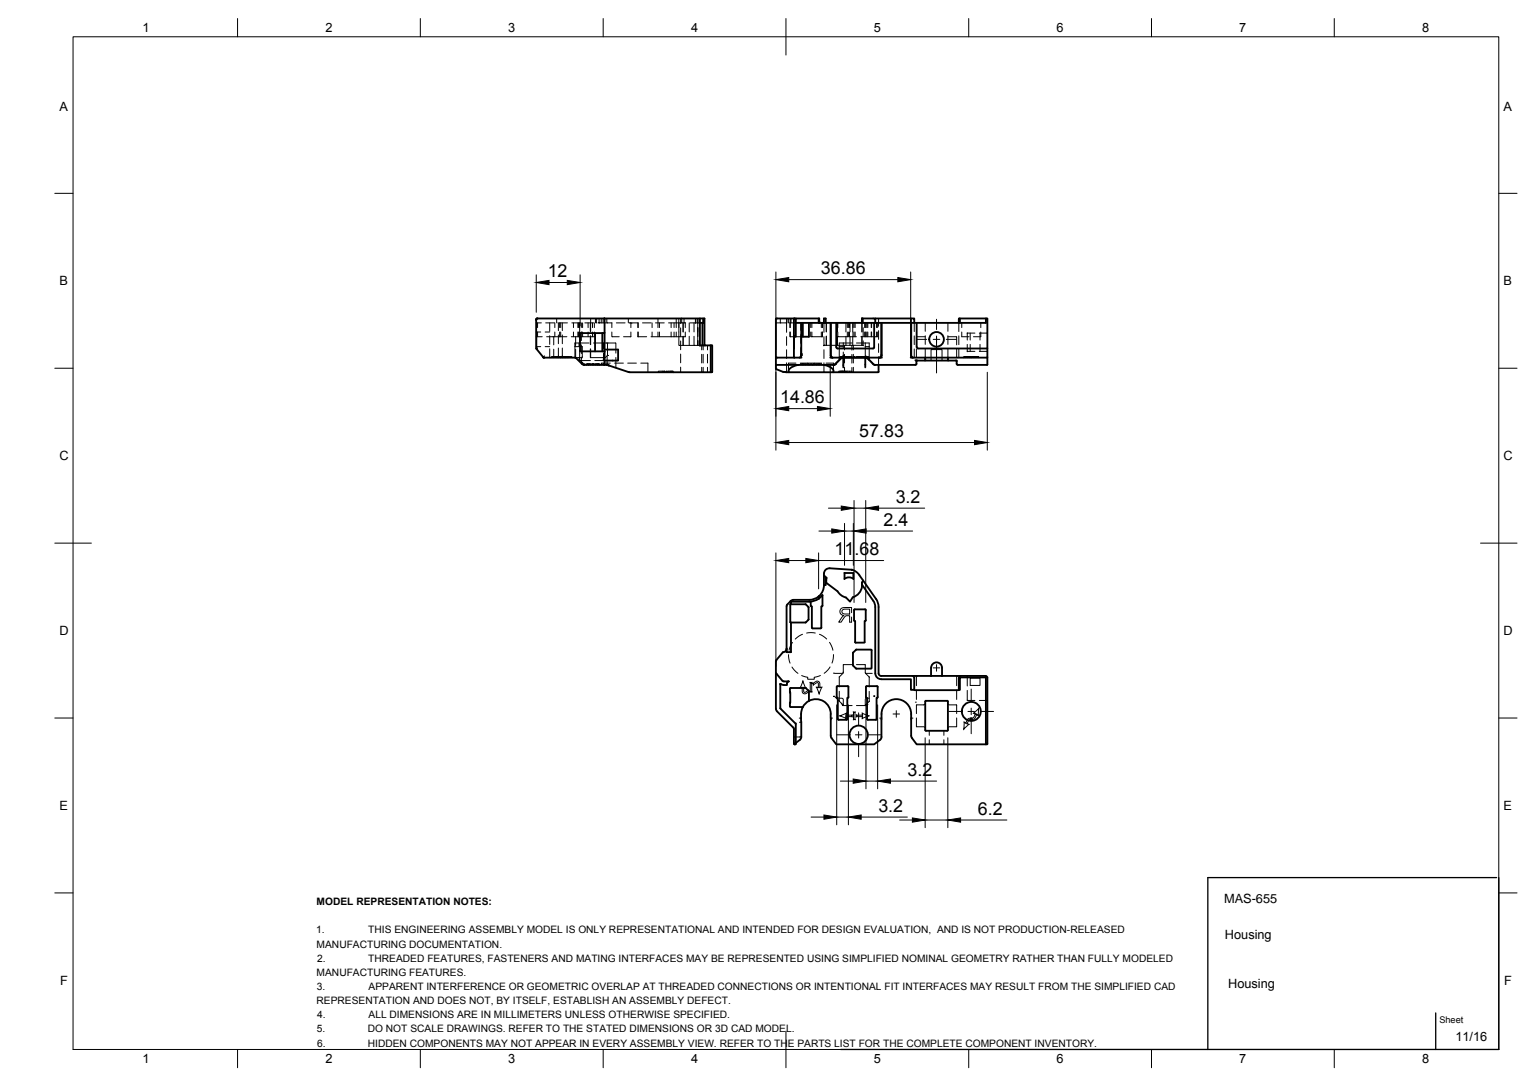
ISO-10303-21;
HEADER;
FILE_DESCRIPTION((''),'2;1');
FILE_NAME('Housing.step','2026-10-09T11:34:15-07:00',(''),(''),'','','');
FILE_SCHEMA (('AUTOMOTIVE_DESIGN { 1 0 10303 214 3 1 1 }'));
ENDSEC;
DATA;
#10=MECHANICAL_DESIGN_GEOMETRIC_PRESENTATION_REPRESENTATION('',(#643),#117170);
#97=(
BOUNDED_SURFACE()
B_SPLINE_SURFACE(2,2,((#90419,#90420,#90421),(#90422,#90423,#90424),(#90425,
#90426,#90427)),.UNSPECIFIED.,.F.,.F.,.F.)
B_SPLINE_SURFACE_WITH_KNOTS((3,3),(3,3),(-1.57079632679569,0.),(-3.14159265358917,
-1.57079632679587),.UNSPECIFIED.)
GEOMETRIC_REPRESENTATION_ITEM()
RATIONAL_B_SPLINE_SURFACE(((1.,0.707106781187113,1.),(0.707106781186163,
0.500000000000127,0.707106781186163),(1.,0.707106781187113,1.)))
REPRESENTATION_ITEM('')
SURFACE()
) ;
#98=(
BOUNDED_SURFACE()
B_SPLINE_SURFACE(2,2,((#90597,#90598,#90599),(#90600,#90601,#90602),(#90603,
#90604,#90605)),.UNSPECIFIED.,.F.,.F.,.F.)
B_SPLINE_SURFACE_WITH_KNOTS((3,3),(3,3),(-1.570796326795,2.27222014866972E-13),
(-1.57079632679441,-7.1054273575954E-13),.UNSPECIFIED.)
GEOMETRIC_REPRESENTATION_ITEM()
RATIONAL_B_SPLINE_SURFACE(((1.,0.707106781186971,1.),(0.70710678118641,
0.500000000000203,0.70710678118641),(1.,0.707106781186971,1.)))
REPRESENTATION_ITEM('')
SURFACE()
) ;
#99=(
BOUNDED_SURFACE()
B_SPLINE_SURFACE(2,2,((#92757,#92758,#92759),(#92760,#92761,#92762),(#92763,
#92764,#92765)),.UNSPECIFIED.,.F.,.F.,.F.)
B_SPLINE_SURFACE_WITH_KNOTS((3,3),(3,3),(-1.57079632680452,-1.25635394189736E-12),
(-2.44346095281043,-1.64859272029811),.UNSPECIFIED.)
GEOMETRIC_REPRESENTATION_ITEM()
RATIONAL_B_SPLINE_SURFACE(((1.,0.922057163080232,1.),(0.707106781183326,
0.651992872652692,0.707106781183326),(1.,0.922057163080232,1.)))
REPRESENTATION_ITEM('')
SURFACE()
) ;
#100=(
BOUNDED_SURFACE()
B_SPLINE_SURFACE(2,2,((#92794,#92795,#92796,#92797,#92798),(#92799,#92800,
#92801,#92802,#92803),(#92804,#92805,#92806,#92807,#92808)),
 .UNSPECIFIED.,.F.,.F.,.F.)
B_SPLINE_SURFACE_WITH_KNOTS((3,3),(3,2,3),(-3.14159265358979,-1.57079632679397),
(-0.795304873266846,0.,0.795304873266846),.UNSPECIFIED.)
GEOMETRIC_REPRESENTATION_ITEM()
RATIONAL_B_SPLINE_SURFACE(((1.,0.921972639390714,1.,0.921972639390714,1.),
(0.707106781186466,0.651933105381558,0.707106781186466,0.651933105381558,
0.707106781186466),(1.,0.921972639390714,1.,0.921972639390714,1.)))
REPRESENTATION_ITEM('')
SURFACE()
) ;
#101=(
BOUNDED_SURFACE()
B_SPLINE_SURFACE(2,2,((#97993,#97994,#97995),(#97996,#97997,#97998),(#97999,
#98000,#98001)),.UNSPECIFIED.,.F.,.F.,.F.)
B_SPLINE_SURFACE_WITH_KNOTS((3,3),(3,3),(-1.57079632673965,5.57007752630405E-11),
(4.19220214067588E-12,0.187132086721036),.UNSPECIFIED.)
GEOMETRIC_REPRESENTATION_ITEM()
RATIONAL_B_SPLINE_SURFACE(((1.,0.99562589029583,1.),(0.70710678118639,0.704013818552918,
0.70710678118639),(1.,0.99562589029583,1.)))
REPRESENTATION_ITEM('')
SURFACE()
) ;
#102=(
BOUNDED_SURFACE()
B_SPLINE_SURFACE(2,2,((#98044,#98045,#98046),(#98047,#98048,#98049),(#98050,
#98051,#98052)),.UNSPECIFIED.,.F.,.F.,.F.)
B_SPLINE_SURFACE_WITH_KNOTS((3,3),(3,3),(-1.57079632677152,2.35301000695734E-11),
(3.55271367856584E-13,0.187132086725463),.UNSPECIFIED.)
GEOMETRIC_REPRESENTATION_ITEM()
RATIONAL_B_SPLINE_SURFACE(((1.,0.995625890295444,1.),(0.707106781186499,
0.704013818552754,0.707106781186499),(1.,0.995625890295444,1.)))
REPRESENTATION_ITEM('')
SURFACE()
) ;
#395=ELLIPSE('',#52555,0.105759245252314,0.090533850109107) ;
#396=ELLIPSE('',#52556,0.105759245244956,0.0905338500956946) ;
#397=ELLIPSE('',#52573,0.634821045649877,0.44) ;
#398=ELLIPSE('',#52575,0.499397396869427,0.2) ;
#399=ELLIPSE('',#52590,0.335751501918208,0.111374721424487) ;
#400=ELLIPSE('',#52593,0.784766199683495,0.4) ;
#401=ELLIPSE('',#52594,24.8257930386904,0.4) ;
#402=ELLIPSE('',#52595,0.424264068711929,0.3) ;
#403=ELLIPSE('',#52596,6.4346717087976,4.55) ;
#404=ELLIPSE('',#52598,0.354400902933385,0.100000000000016) ;
#405=ELLIPSE('',#52599,0.354400902933385,0.100000000000016) ;
#406=ELLIPSE('',#52600,0.354400902933389,0.100000000000016) ;
#407=ELLIPSE('',#52601,0.354400902933389,0.100000000000016) ;
#408=ELLIPSE('',#52605,0.76367532368147,0.54) ;
#409=ELLIPSE('',#52606,0.617737808459213,0.299999999999998) ;
#410=ELLIPSE('',#52614,0.354400902933389,0.100000000000016) ;
#411=ELLIPSE('',#52615,0.354400902933389,0.100000000000016) ;
#412=ELLIPSE('',#52616,0.354400902933385,0.0999999999999801) ;
#413=ELLIPSE('',#52617,0.354400902933385,0.0999999999999801) ;
#414=ELLIPSE('',#52621,0.617737808459213,0.300000000000002) ;
#415=ELLIPSE('',#52622,0.76367532368147,0.54) ;
#416=ELLIPSE('',#52628,0.141421356237298,0.1) ;
#417=ELLIPSE('',#52631,0.277848879788995,0.239999999999938) ;
#418=ELLIPSE('',#52632,0.277848879788997,0.240000000000009) ;
#419=ELLIPSE('',#52639,0.141421356237298,0.1) ;
#420=ELLIPSE('',#52640,0.141421356237298,0.1) ;
#421=ELLIPSE('',#52647,0.339411254969547,0.24) ;
#422=ELLIPSE('',#52650,0.243578652595007,0.24) ;
#423=ELLIPSE('',#52652,0.0577110041499885,0.04) ;
#424=ELLIPSE('',#52655,0.577110041499878,0.399999999999996) ;
#425=ELLIPSE('',#52668,0.424264068711929,0.3) ;
#426=ELLIPSE('',#52700,0.344580851516853,0.222253203953467) ;
#427=ELLIPSE('',#52708,0.141421356237297,0.1) ;
#428=ELLIPSE('',#52747,0.141421356237322,0.1) ;
#429=ELLIPSE('',#52767,1.13357840487546,0.749999999999993) ;
#430=ELLIPSE('',#52768,1.20208152801713,0.85) ;
#431=ELLIPSE('',#52771,0.223606797749978,0.100000000000016) ;
#432=ELLIPSE('',#52772,0.282842712474619,0.2) ;
#433=ELLIPSE('',#52774,0.10069443430648,0.100017256319563) ;
#434=ELLIPSE('',#52805,0.282842712474618,0.2) ;
#435=ELLIPSE('',#52806,0.223606797749975,0.100000000000016) ;
#436=ELLIPSE('',#52810,0.70710678118655,0.5) ;
#437=ELLIPSE('',#52811,0.640312423743287,0.399999999999992) ;
#438=ELLIPSE('',#52813,0.846312901686476,0.400595643005874) ;
#439=ELLIPSE('',#52814,0.862858514657635,0.518233232113999) ;
#440=ELLIPSE('',#52815,0.640312423743287,0.399999999999992) ;
#441=ELLIPSE('',#52816,0.70710678118655,0.5) ;
#442=ELLIPSE('',#52818,0.412310562561758,0.4) ;
#443=ELLIPSE('',#52820,1.34350288425444,0.95) ;
#444=ELLIPSE('',#52825,0.141421356237322,0.1) ;
#445=ELLIPSE('',#52829,0.141421356237322,0.1) ;
#446=ELLIPSE('',#52836,0.223606797749974,0.0999999999999979) ;
#447=ELLIPSE('',#52837,0.223606797749986,0.0999999999999979) ;
#448=ELLIPSE('',#52967,0.258478364700829,0.0999999999999979) ;
#449=ELLIPSE('',#52969,0.311144765372046,0.199999999999998) ;
#450=ELLIPSE('',#52993,0.624999999999997,0.4) ;
#451=ELLIPSE('',#53004,0.51747248987523,0.4999999999999) ;
#452=ELLIPSE('',#53007,0.202758751010048,0.200000000000102) ;
#453=ELLIPSE('',#53010,1.06510302057801,0.999999999999996) ;
#454=ELLIPSE('',#53041,0.499999999999995,0.4) ;
#455=ELLIPSE('',#53084,0.499999999999995,0.4) ;
#456=ELLIPSE('',#53153,0.110950450383119,0.1) ;
#457=ELLIPSE('',#53155,0.693271231193088,0.499999999999992) ;
#458=ELLIPSE('',#53183,0.421637021355679,0.399999999999901) ;
#459=ELLIPSE('',#53187,0.105409255339058,0.100000000000106) ;
#460=ELLIPSE('',#53189,1.1595018087284,1.1) ;
#461=ELLIPSE('',#53225,0.141421356237293,0.1) ;
#462=ELLIPSE('',#53250,0.10597392847322,0.1) ;
#463=ELLIPSE('',#53279,0.800390529679108,0.5) ;
#464=ELLIPSE('',#53281,0.883883476483187,0.5) ;
#465=ELLIPSE('',#53287,0.210818510677909,0.200000000000016) ;
#466=ELLIPSE('',#53289,0.120185042515483,0.0999999999999979) ;
#467=ELLIPSE('',#53291,0.21081851067789,0.199999999999998) ;
#468=ELLIPSE('',#53293,0.120185042515479,0.0999999999999979) ;
#469=ELLIPSE('',#53311,0.316227766016838,0.3) ;
#470=ELLIPSE('',#53317,6.48266920334518,6.15) ;
#471=ELLIPSE('',#53320,1.21037184369102,0.749999999999993) ;
#472=ELLIPSE('',#53322,0.141421356237311,0.1) ;
#473=ELLIPSE('',#53323,0.112603250061041,0.1) ;
#474=ELLIPSE('',#53325,0.17320508075689,0.1) ;
#475=ELLIPSE('',#53326,0.173205080756888,0.1) ;
#476=ELLIPSE('',#53334,0.704171845621267,0.200000000000013) ;
#477=ELLIPSE('',#53337,24.8233760798141,0.2) ;
#478=ELLIPSE('',#53340,0.860232526704269,0.5) ;
#479=ELLIPSE('',#53341,0.18370348154524,0.0706876553262425) ;
#480=ELLIPSE('',#53343,0.989949493661167,0.7) ;
#481=ELLIPSE('',#53347,0.777817459305202,0.55) ;
#482=ELLIPSE('',#53348,0.930053761886906,0.75) ;
#483=ELLIPSE('',#53349,0.930053761886906,0.75) ;
#484=ELLIPSE('',#53358,0.675321117625136,0.479717269382621) ;
#485=ELLIPSE('',#53360,6.4346717087976,4.55) ;
#486=ELLIPSE('',#53363,0.461579895576042,0.2) ;
#487=ELLIPSE('',#53367,0.282842712474621,0.2) ;
#488=ELLIPSE('',#53373,0.565685424949227,0.399999999999992) ;
#489=ELLIPSE('',#53379,6.48266920334518,6.15) ;
#490=ELLIPSE('',#53401,0.100694440756805,0.100017263171969) ;
#491=ELLIPSE('',#53406,0.108636037740531,0.1) ;
#492=ELLIPSE('',#53416,0.179117445565849,0.1) ;
#493=ELLIPSE('',#53419,0.179117445565765,0.1) ;
#494=ELLIPSE('',#53421,0.265520995084799,0.1) ;
#495=ELLIPSE('',#53429,0.179117445565772,0.1) ;
#496=ELLIPSE('',#53431,0.265520995084877,0.1) ;
#497=ELLIPSE('',#53433,0.179117445565864,0.1) ;
#498=ELLIPSE('',#53440,0.179117445565776,0.1) ;
#499=ELLIPSE('',#53441,0.141421356237291,0.1) ;
#500=ELLIPSE('',#53443,0.265520995084917,0.1) ;
#501=ELLIPSE('',#53445,0.179117445565779,0.1) ;
#502=ELLIPSE('',#53447,0.141421356237298,0.1) ;
#503=ELLIPSE('',#53449,0.14142135623732,0.1) ;
#504=ELLIPSE('',#53451,0.141421356237322,0.1) ;
#505=ELLIPSE('',#53459,0.141421356237284,0.1) ;
#506=ELLIPSE('',#53460,0.141421356237347,0.1) ;
#507=ELLIPSE('',#53462,0.141421356237322,0.1) ;
#508=ELLIPSE('',#53464,0.141421356237297,0.1) ;
#509=ELLIPSE('',#53470,0.141421356237321,0.1) ;
#510=ELLIPSE('',#53471,0.17911744556577,0.1) ;
#511=ELLIPSE('',#53473,0.141421356237297,0.1) ;
#512=ELLIPSE('',#53475,0.141421356237325,0.1) ;
#513=ELLIPSE('',#53477,0.141421356237269,0.1) ;
#514=ELLIPSE('',#53479,0.17911744556575,0.1) ;
#515=ELLIPSE('',#53481,0.265520995084842,0.1) ;
#516=ELLIPSE('',#53489,0.141421356237322,0.1) ;
#517=ELLIPSE('',#53490,0.141421356237297,0.1) ;
#518=ELLIPSE('',#53492,0.141421356237297,0.1) ;
#519=ELLIPSE('',#53494,0.141421356237322,0.1) ;
#520=ELLIPSE('',#53500,0.179117445565841,0.1) ;
#521=ELLIPSE('',#53501,0.265520995084931,0.1) ;
#522=ELLIPSE('',#53503,0.141421356237301,0.1) ;
#523=ELLIPSE('',#53511,0.141421356237312,0.1) ;
#524=ELLIPSE('',#53513,0.141421356237306,0.1) ;
#525=ELLIPSE('',#53521,0.141421356237327,0.1) ;
#526=ELLIPSE('',#53523,0.179117445565764,0.1) ;
#527=ELLIPSE('',#53534,0.141421356237301,0.1) ;
#528=ELLIPSE('',#53535,0.179117445565841,0.1) ;
#529=ELLIPSE('',#53543,0.141421356237313,0.1) ;
#530=ELLIPSE('',#53545,0.141421356237306,0.1) ;
#531=ELLIPSE('',#53553,0.141421356237327,0.1) ;
#532=ELLIPSE('',#53555,0.179117445565764,0.1) ;
#533=ELLIPSE('',#53557,0.265520995084931,0.1) ;
#534=ELLIPSE('',#53569,0.179117445565845,0.1) ;
#535=ELLIPSE('',#53571,0.265520995084763,0.1) ;
#536=ELLIPSE('',#53573,0.179117445565757,0.1) ;
#537=ELLIPSE('',#53577,0.179117445565837,0.1) ;
#538=ELLIPSE('',#53579,0.179117445565763,0.1) ;
#539=ELLIPSE('',#53580,0.265520995084739,0.1) ;
#540=ELLIPSE('',#53587,0.179117445565766,0.1) ;
#541=ELLIPSE('',#53588,0.265520995084941,0.1) ;
#542=ELLIPSE('',#53590,0.179117445565779,0.1) ;
#543=ELLIPSE('',#53592,0.141421356237327,0.1) ;
#544=ELLIPSE('',#53594,0.141421356237297,0.1) ;
#545=ELLIPSE('',#53596,0.141421356237347,0.1) ;
#546=ELLIPSE('',#53598,0.141421356237294,0.1) ;
#547=ELLIPSE('',#53610,0.14142135623731,0.1) ;
#548=ELLIPSE('',#53611,0.141421356237284,0.1) ;
#549=ELLIPSE('',#53613,0.141421356237322,0.1) ;
#550=ELLIPSE('',#53615,0.141421356237297,0.1) ;
#551=ELLIPSE('',#53619,0.141421356237325,0.1) ;
#552=ELLIPSE('',#53620,0.141421356237319,0.1) ;
#553=ELLIPSE('',#53622,0.141421356237303,0.1) ;
#554=ELLIPSE('',#53624,0.179117445565787,0.1) ;
#555=ELLIPSE('',#53626,0.265520995084743,0.1) ;
#556=ELLIPSE('',#53628,0.179117445565783,0.1) ;
#557=ELLIPSE('',#53630,0.141421356237323,0.1) ;
#558=ELLIPSE('',#53635,0.141421356237297,0.1) ;
#559=ELLIPSE('',#53636,0.141421356237322,0.1) ;
#560=ELLIPSE('',#53638,0.141421356237322,0.1) ;
#561=ELLIPSE('',#53640,0.141421356237322,0.1) ;
#562=ELLIPSE('',#53644,0.141421356237324,0.1) ;
#563=ELLIPSE('',#53646,0.179117445565837,0.1) ;
#564=ELLIPSE('',#53648,0.265520995084907,0.1) ;
#565=ELLIPSE('',#53650,0.17911744556577,0.1) ;
#566=ELLIPSE('',#53652,0.141421356237293,0.1) ;
#567=ELLIPSE('',#53669,0.141421356237314,0.1) ;
#568=ELLIPSE('',#53670,0.141421356237323,0.1) ;
#569=ELLIPSE('',#53673,0.141421356237324,0.1) ;
#570=ELLIPSE('',#53675,0.179117445565837,0.1) ;
#571=ELLIPSE('',#53677,0.265520995084885,0.1) ;
#572=ELLIPSE('',#53679,0.179117445565777,0.1) ;
#573=ELLIPSE('',#53681,0.141421356237293,0.1) ;
#574=ELLIPSE('',#53750,0.554752251915545,0.5) ;
#575=ELLIPSE('',#53770,1.17924764150709,0.999999999999996) ;
#576=ELLIPSE('',#53781,6.09138736249799,4.05) ;
#577=ELLIPSE('',#53794,6.09138736249799,4.05) ;
#578=ELLIPSE('',#53808,1.04166666666667,0.5) ;
#579=ELLIPSE('',#53810,1.17924764150709,0.999999999999997) ;
#580=ELLIPSE('',#53811,0.800390529679107,0.5) ;
#581=ELLIPSE('',#53814,1.17924764150709,0.999999999999997) ;
#582=ELLIPSE('',#53815,0.800390529679107,0.5) ;
#583=ELLIPSE('',#53817,0.883883476483178,0.5) ;
#584=ELLIPSE('',#53821,1.17924764150709,0.999999999999996) ;
#585=ELLIPSE('',#53822,0.800390529679108,0.5) ;
#601=SHAPE_REPRESENTATION_RELATIONSHIP('SRR','None',#117256,#622) ;
#622=ADVANCED_BREP_SHAPE_REPRESENTATION('',(#664),#117164) ;
#643=STYLED_ITEM('',(#117355),#664) ;
#664=MANIFOLD_SOLID_BREP('Body1',#49072) ;
#738=FACE_BOUND('',#15575,.T.) ;
#739=FACE_BOUND('',#15577,.T.) ;
#740=FACE_BOUND('',#15578,.T.) ;
#741=FACE_BOUND('',#15718,.T.) ;
#742=FACE_BOUND('',#15719,.T.) ;
#743=FACE_BOUND('',#15720,.T.) ;
#744=FACE_BOUND('',#15721,.T.) ;
#745=FACE_BOUND('',#15722,.T.) ;
#746=FACE_BOUND('',#15723,.T.) ;
#747=FACE_BOUND('',#15724,.T.) ;
#748=FACE_BOUND('',#15886,.T.) ;
#749=FACE_BOUND('',#15887,.T.) ;
#750=FACE_BOUND('',#15891,.T.) ;
#751=FACE_BOUND('',#15930,.T.) ;
#752=FACE_BOUND('',#15931,.T.) ;
#753=FACE_BOUND('',#15932,.T.) ;
#754=FACE_BOUND('',#15963,.T.) ;
#755=FACE_BOUND('',#15973,.T.) ;
#756=FACE_BOUND('',#15976,.T.) ;
#757=FACE_BOUND('',#16106,.T.) ;
#758=FACE_BOUND('',#16107,.T.) ;
#759=FACE_BOUND('',#16108,.T.) ;
#760=FACE_BOUND('',#16262,.T.) ;
#1149=B_SPLINE_CURVE_WITH_KNOTS('',3,(#89080,#89081,#89082,#89083,#89084,
#89085,#89086,#89087,#89088,#89089,#89090,#89091,#89092),.UNSPECIFIED.,
 .F.,.F.,(4,1,1,1,1,1,1,1,1,1,4),(0.,0.1,0.2,0.3,0.4,0.5,0.6,0.7,0.8,0.9,
1.),.UNSPECIFIED.) ;
#1150=B_SPLINE_CURVE_WITH_KNOTS('',3,(#89094,#89095,#89096,#89097,#89098,
#89099),.UNSPECIFIED.,.F.,.F.,(4,1,1,4),(0.,0.333333333333333,0.666666666666667,
1.),.UNSPECIFIED.) ;
#1151=B_SPLINE_CURVE_WITH_KNOTS('',3,(#89101,#89102,#89103,#89104,#89105,
#89106,#89107,#89108,#89109,#89110,#89111,#89112,#89113,#89114,#89115,#89116,
#89117,#89118,#89119,#89120,#89121,#89122,#89123,#89124,#89125,#89126,#89127,
#89128,#89129,#89130,#89131,#89132,#89133,#89134,#89135,#89136,#89137,#89138,
#89139,#89140,#89141,#89142,#89143,#89144,#89145,#89146,#89147,#89148,#89149,
#89150,#89151,#89152,#89153,#89154,#89155,#89156,#89157,#89158,#89159,#89160,
#89161,#89162,#89163,#89164),.UNSPECIFIED.,.F.,.F.,(4,3,3,3,3,3,3,3,3,3,
3,3,3,3,3,3,3,3,3,3,3,4),(0.50000000000002,0.540931884362004,0.549999476969566,
0.57785534140829,0.599999449142665,0.630623423732254,0.650001938995543,
0.670121368703304,0.699999961337087,0.726319366023772,0.749998804879715,
0.764743070246695,0.800000000093043,0.800090168326521,0.850000141966713,
0.856761721866945,0.899999993071106,0.902358829665644,0.942091717824869,
0.950000243206862,0.977692918008602,1.),.UNSPECIFIED.) ;
#1152=B_SPLINE_CURVE_WITH_KNOTS('',3,(#89245,#89246,#89247,#89248,#89249,
#89250,#89251,#89252,#89253,#89254,#89255,#89256,#89257),.UNSPECIFIED.,
 .F.,.F.,(4,1,1,1,1,1,1,1,1,1,4),(0.,0.1,0.2,0.3,0.4,0.5,0.6,0.7,0.8,0.9,
1.),.UNSPECIFIED.) ;
#1153=B_SPLINE_CURVE_WITH_KNOTS('',3,(#89260,#89261,#89262,#89263,#89264,
#89265,#89266,#89267,#89268,#89269,#89270,#89271,#89272,#89273,#89274,#89275,
#89276,#89277,#89278,#89279,#89280,#89281,#89282,#89283,#89284,#89285,#89286,
#89287,#89288,#89289,#89290,#89291,#89292,#89293,#89294,#89295,#89296,#89297,
#89298,#89299,#89300,#89301,#89302,#89303,#89304,#89305,#89306,#89307,#89308,
#89309,#89310,#89311,#89312,#89313,#89314,#89315,#89316,#89317,#89318,#89319,
#89320,#89321,#89322,#89323,#89324,#89325,#89326),.UNSPECIFIED.,.F.,.F.,
(4,3,3,3,3,3,3,3,3,3,3,3,3,3,3,3,3,3,3,3,3,3,4),(0.,0.029211291026702,0.0500008174088028,
0.060544943773545,0.0938972400757973,0.100000166665901,0.130378684246365,
0.15000088015134,0.174071006839537,0.199999777732466,0.221649421518731,
0.249999425571877,0.25898085613298,0.293770381915345,0.299999713862244,
0.331057161559401,0.350001769846541,0.368733440803518,0.400000309272562,
0.412905090819267,0.450000017037755,0.479639534628252,0.50000000000002),
 .UNSPECIFIED.) ;
#1154=B_SPLINE_CURVE_WITH_KNOTS('',3,(#89406,#89407,#89408,#89409,#89410,
#89411),.UNSPECIFIED.,.F.,.F.,(4,1,1,4),(0.,0.333333333333333,0.666666666666667,
0.999999901148969),.UNSPECIFIED.) ;
#1155=B_SPLINE_CURVE_WITH_KNOTS('',3,(#89413,#89414,#89415,#89416,#89417,
#89418,#89419,#89420,#89421,#89422,#89423,#89424,#89425,#89426,#89427,#89428,
#89429,#89430,#89431,#89432,#89433,#89434,#89435,#89436,#89437,#89438,#89439,
#89440,#89441,#89442,#89443,#89444,#89445,#89446,#89447,#89448,#89449,#89450,
#89451,#89452,#89453,#89454,#89455),.UNSPECIFIED.,.F.,.F.,(4,3,3,3,3,3,
3,3,3,3,3,3,3,3,4),(0.740046669567313,0.763099290859212,0.784481908360721,
0.811421669815631,0.819140541376942,0.832121780979733,0.85502513103706,
0.889660371947781,0.913260537792704,0.914933018320988,0.935388557500039,
0.955946024091937,0.975439020158076,0.993845115294604,0.999999999999939),
 .UNSPECIFIED.) ;
#1156=B_SPLINE_CURVE_WITH_KNOTS('',3,(#89457,#89458,#89459,#89460,#89461,
#89462,#89463,#89464,#89465,#89466,#89467,#89468,#89469,#89470,#89471,#89472,
#89473,#89474,#89475,#89476,#89477,#89478,#89479,#89480,#89481,#89482,#89483,
#89484,#89485,#89486,#89487,#89488,#89489,#89490,#89491,#89492,#89493,#89494,
#89495,#89496,#89497,#89498,#89499,#89500,#89501,#89502,#89503,#89504,#89505,
#89506,#89507,#89508,#89509,#89510,#89511,#89512,#89513,#89514,#89515,#89516,
#89517,#89518,#89519,#89520,#89521,#89522,#89523,#89524,#89525,#89526,#89527,
#89528,#89529,#89530,#89531,#89532,#89533,#89534,#89535,#89536,#89537,#89538,
#89539,#89540,#89541,#89542,#89543,#89544,#89545,#89546,#89547,#89548,#89549,
#89550,#89551,#89552,#89553,#89554,#89555,#89556),.UNSPECIFIED.,.F.,.F.,
(4,3,3,3,3,3,3,3,3,3,3,3,3,3,3,3,3,3,3,3,3,3,3,3,3,3,3,3,3,3,3,3,3,4),(9.43012544827459E-8,
0.031864058797589,0.0647840362122895,0.0990069909892971,0.125039338268755,
0.134916637559053,0.176959063913584,0.215046371604815,0.260170220267245,
0.265136830208005,0.318040825054938,0.360663273489004,0.363657546998835,
0.400621818895941,0.438082955214945,0.468825159061875,0.473202770514011,
0.511546102075598,0.546372378738656,0.578100024548857,0.583032295575111,
0.622265622394134,0.665621014897703,0.680754237084197,0.720780686822075,
0.771027763058629,0.790928228827376,0.813100495945339,0.85149915167859,
0.888624363758942,0.922410481952504,0.955205742315633,0.986814689647663,
1.),.UNSPECIFIED.) ;
#1157=B_SPLINE_CURVE_WITH_KNOTS('',3,(#89625,#89626,#89627,#89628,#89629,
#89630,#89631,#89632,#89633,#89634,#89635),.UNSPECIFIED.,.F.,.F.,(4,1,1,
1,1,1,1,1,4),(0.,0.125,0.25,0.375,0.5,0.625,0.75,0.875,1.),
 .UNSPECIFIED.) ;
#1158=B_SPLINE_CURVE_WITH_KNOTS('',3,(#89638,#89639,#89640,#89641,#89642,
#89643,#89644,#89645,#89646,#89647,#89648,#89649,#89650,#89651,#89652,#89653,
#89654,#89655,#89656,#89657,#89658,#89659,#89660,#89661,#89662,#89663,#89664,
#89665,#89666,#89667,#89668,#89669,#89670,#89671,#89672,#89673,#89674,#89675,
#89676,#89677,#89678,#89679,#89680,#89681,#89682,#89683,#89684,#89685,#89686,
#89687,#89688,#89689,#89690,#89691,#89692,#89693,#89694,#89695,#89696,#89697,
#89698,#89699,#89700,#89701,#89702,#89703,#89704,#89705,#89706,#89707,#89708,
#89709,#89710,#89711,#89712,#89713,#89714,#89715,#89716,#89717,#89718,#89719,
#89720,#89721,#89722,#89723,#89724,#89725,#89726,#89727,#89728,#89729,#89730,
#89731,#89732,#89733,#89734,#89735,#89736,#89737),.UNSPECIFIED.,.F.,.F.,
(4,3,3,3,3,3,3,3,3,3,3,3,3,3,3,3,3,3,3,3,3,3,3,3,3,3,3,3,3,3,3,3,3,4),(0.,
0.0234163840184272,0.0478392774354898,0.0735929525966121,0.101260672275236,
0.13215515581021,0.161611085696521,0.205091291829831,0.208484168145554,
0.238318416362703,0.265116005993426,0.265187074007494,0.29019218665116,
0.318308090975454,0.345050056035187,0.357100347629798,0.373722767756927,
0.405591170427141,0.433846469730387,0.445335557423208,0.48217444472529,
0.505617857135101,0.514408471114612,0.542613244205269,0.568369687650452,
0.581008652375286,0.593348553719565,0.615767486536519,0.638648003192484,
0.659516414041665,0.663954602269109,0.699207373791262,0.730123470459489,
0.740046655839865),.UNSPECIFIED.) ;
#1159=B_SPLINE_CURVE_WITH_KNOTS('',3,(#89805,#89806,#89807,#89808,#89809,
#89810),.UNSPECIFIED.,.F.,.F.,(4,1,1,4),(0.,0.333333333333333,0.666666666666667,
1.),.UNSPECIFIED.) ;
#1160=B_SPLINE_CURVE_WITH_KNOTS('',3,(#89812,#89813,#89814,#89815,#89816,
#89817,#89818,#89819,#89820,#89821,#89822,#89823,#89824,#89825,#89826,#89827,
#89828,#89829,#89830,#89831,#89832,#89833,#89834,#89835,#89836,#89837,#89838,
#89839,#89840,#89841,#89842,#89843,#89844,#89845,#89846,#89847,#89848,#89849,
#89850,#89851,#89852,#89853,#89854,#89855,#89856,#89857,#89858,#89859,#89860,
#89861,#89862,#89863,#89864,#89865,#89866,#89867,#89868,#89869,#89870,#89871,
#89872),.UNSPECIFIED.,.F.,.F.,(4,3,3,3,3,3,3,3,3,3,3,3,3,3,3,3,3,3,3,3,
4),(0.499999999999957,0.543426929556171,0.562498466595099,0.582529420733352,
0.623146114415814,0.624999981287924,0.663596929285891,0.687501639134093,
0.717594346195301,0.749999793833349,0.754935239198527,0.789630090278152,
0.812500138729425,0.825709594031802,0.866465848423957,0.875000628872866,
0.911531406767164,0.937498440919157,0.946944182542892,0.977771956059037,
1.),.UNSPECIFIED.) ;
#1161=B_SPLINE_CURVE_WITH_KNOTS('',3,(#89894,#89895,#89896,#89897,#89898),
 .UNSPECIFIED.,.F.,.F.,(4,1,4),(0.,0.0298071351389365,0.0685496713495228),
 .UNSPECIFIED.) ;
#1162=B_SPLINE_CURVE_WITH_KNOTS('',3,(#89901,#89902,#89903,#89904,#89905),
 .UNSPECIFIED.,.F.,.F.,(4,1,4),(0.,0.0298071351389365,0.0685496713495228),
 .UNSPECIFIED.) ;
#1163=B_SPLINE_CURVE_WITH_KNOTS('',3,(#89917,#89918,#89919,#89920,#89921),
 .UNSPECIFIED.,.F.,.F.,(4,1,4),(0.,0.0263673128827931,0.0523427870633456),
 .UNSPECIFIED.) ;
#1164=B_SPLINE_CURVE_WITH_KNOTS('',3,(#89924,#89925,#89926,#89927,#89928),
 .UNSPECIFIED.,.F.,.F.,(4,1,4),(0.,0.0263673128827931,0.0523427870633456),
 .UNSPECIFIED.) ;
#1165=B_SPLINE_CURVE_WITH_KNOTS('',3,(#89940,#89941,#89942,#89943,#89944),
 .UNSPECIFIED.,.F.,.F.,(4,1,4),(0.,0.0190758281807941,0.0379545209982657),
 .UNSPECIFIED.) ;
#1166=B_SPLINE_CURVE_WITH_KNOTS('',3,(#89947,#89948,#89949,#89950,#89951),
 .UNSPECIFIED.,.F.,.F.,(4,1,4),(0.,0.0190758281807941,0.0379545209982657),
 .UNSPECIFIED.) ;
#1167=B_SPLINE_CURVE_WITH_KNOTS('',3,(#89963,#89964,#89965,#89966,#89967),
 .UNSPECIFIED.,.F.,.F.,(4,1,4),(0.,0.0205128997765721,0.0398218276255599),
 .UNSPECIFIED.) ;
#1168=B_SPLINE_CURVE_WITH_KNOTS('',3,(#89970,#89971,#89972,#89973,#89974),
 .UNSPECIFIED.,.F.,.F.,(4,1,4),(0.,0.0205128997765721,0.0398218276255599),
 .UNSPECIFIED.) ;
#1169=B_SPLINE_CURVE_WITH_KNOTS('',3,(#89986,#89987,#89988,#89989,#89990),
 .UNSPECIFIED.,.F.,.F.,(4,1,4),(0.,0.0323852950215525,0.0574227556854303),
 .UNSPECIFIED.) ;
#1170=B_SPLINE_CURVE_WITH_KNOTS('',3,(#89993,#89994,#89995,#89996,#89997),
 .UNSPECIFIED.,.F.,.F.,(4,1,4),(0.,0.0323852950215525,0.0574227556854303),
 .UNSPECIFIED.) ;
#1171=B_SPLINE_CURVE_WITH_KNOTS('',3,(#90033,#90034,#90035,#90036,#90037),
 .UNSPECIFIED.,.F.,.F.,(4,1,4),(0.,0.011955158932918,0.0295605475166918),
 .UNSPECIFIED.) ;
#1172=B_SPLINE_CURVE_WITH_KNOTS('',3,(#90040,#90041,#90042,#90043,#90044),
 .UNSPECIFIED.,.F.,.F.,(4,1,4),(0.,0.011955158932918,0.0295605475166918),
 .UNSPECIFIED.) ;
#1173=B_SPLINE_CURVE_WITH_KNOTS('',3,(#90056,#90057,#90058,#90059,#90060),
 .UNSPECIFIED.,.F.,.F.,(4,1,4),(0.,0.0135228484064754,0.0263579081616444),
 .UNSPECIFIED.) ;
#1174=B_SPLINE_CURVE_WITH_KNOTS('',3,(#90063,#90064,#90065,#90066,#90067),
 .UNSPECIFIED.,.F.,.F.,(4,1,4),(0.,0.0135228484064754,0.0263579081616444),
 .UNSPECIFIED.) ;
#1175=B_SPLINE_CURVE_WITH_KNOTS('',3,(#90079,#90080,#90081,#90082,#90083),
 .UNSPECIFIED.,.F.,.F.,(4,1,4),(0.,0.0216058216755205,0.0381303842659523),
 .UNSPECIFIED.) ;
#1176=B_SPLINE_CURVE_WITH_KNOTS('',3,(#90086,#90087,#90088,#90089,#90090),
 .UNSPECIFIED.,.F.,.F.,(4,1,4),(0.,0.0216058216755205,0.0381303842659523),
 .UNSPECIFIED.) ;
#1177=B_SPLINE_CURVE_WITH_KNOTS('',3,(#90102,#90103,#90104,#90105,#90106),
 .UNSPECIFIED.,.F.,.F.,(4,1,4),(0.,0.0381782469542568,0.0670753371474822),
 .UNSPECIFIED.) ;
#1178=B_SPLINE_CURVE_WITH_KNOTS('',3,(#90109,#90110,#90111,#90112,#90113),
 .UNSPECIFIED.,.F.,.F.,(4,1,4),(0.,0.0381782469542568,0.0670753371474822),
 .UNSPECIFIED.) ;
#1179=B_SPLINE_CURVE_WITH_KNOTS('',3,(#90143,#90144,#90145,#90146,#90147),
 .UNSPECIFIED.,.F.,.F.,(4,1,4),(0.,0.0329095469988702,0.0691336974954879),
 .UNSPECIFIED.) ;
#1180=B_SPLINE_CURVE_WITH_KNOTS('',3,(#90150,#90151,#90152,#90153,#90154),
 .UNSPECIFIED.,.F.,.F.,(4,1,4),(0.,0.0329095469988702,0.0691336974954879),
 .UNSPECIFIED.) ;
#1181=B_SPLINE_CURVE_WITH_KNOTS('',3,(#90166,#90167,#90168,#90169,#90170),
 .UNSPECIFIED.,.F.,.F.,(4,1,4),(0.,0.0210301296927785,0.0377156586265697),
 .UNSPECIFIED.) ;
#1182=B_SPLINE_CURVE_WITH_KNOTS('',3,(#90173,#90174,#90175,#90176,#90177),
 .UNSPECIFIED.,.F.,.F.,(4,1,4),(0.,0.0210301296927785,0.0377156586265697),
 .UNSPECIFIED.) ;
#1183=B_SPLINE_CURVE_WITH_KNOTS('',3,(#90189,#90190,#90191,#90192,#90193),
 .UNSPECIFIED.,.F.,.F.,(4,1,4),(0.,0.0424180496051088,0.0942055476140892),
 .UNSPECIFIED.) ;
#1184=B_SPLINE_CURVE_WITH_KNOTS('',3,(#90196,#90197,#90198,#90199,#90200),
 .UNSPECIFIED.,.F.,.F.,(4,1,4),(0.,0.0424180496051088,0.0942055476140892),
 .UNSPECIFIED.) ;
#1185=B_SPLINE_CURVE_WITH_KNOTS('',3,(#90212,#90213,#90214,#90215,#90216),
 .UNSPECIFIED.,.F.,.F.,(4,1,4),(0.,0.0398228695438388,0.0783699334705556),
 .UNSPECIFIED.) ;
#1186=B_SPLINE_CURVE_WITH_KNOTS('',3,(#90219,#90220,#90221,#90222,#90223),
 .UNSPECIFIED.,.F.,.F.,(4,1,4),(0.,0.0398228695438388,0.0783699334705556),
 .UNSPECIFIED.) ;
#1187=B_SPLINE_CURVE_WITH_KNOTS('',3,(#90235,#90236,#90237,#90238,#90239),
 .UNSPECIFIED.,.F.,.F.,(4,1,4),(0.,0.0313133324080373,0.063168759987351),
 .UNSPECIFIED.) ;
#1188=B_SPLINE_CURVE_WITH_KNOTS('',3,(#90242,#90243,#90244,#90245,#90246),
 .UNSPECIFIED.,.F.,.F.,(4,1,4),(0.,0.0313133324080373,0.063168759987351),
 .UNSPECIFIED.) ;
#1189=B_SPLINE_CURVE_WITH_KNOTS('',3,(#90258,#90259,#90260,#90261,#90262),
 .UNSPECIFIED.,.F.,.F.,(4,1,4),(0.,0.0290828541577381,0.0592932101613289),
 .UNSPECIFIED.) ;
#1190=B_SPLINE_CURVE_WITH_KNOTS('',3,(#90265,#90266,#90267,#90268,#90269),
 .UNSPECIFIED.,.F.,.F.,(4,1,4),(0.,0.0290828541577381,0.0592932101613289),
 .UNSPECIFIED.) ;
#1191=B_SPLINE_CURVE_WITH_KNOTS('',3,(#90281,#90282,#90283,#90284,#90285),
 .UNSPECIFIED.,.F.,.F.,(4,1,4),(0.,0.0471458586470647,0.0823534588635132),
 .UNSPECIFIED.) ;
#1192=B_SPLINE_CURVE_WITH_KNOTS('',3,(#90288,#90289,#90290,#90291,#90292),
 .UNSPECIFIED.,.F.,.F.,(4,1,4),(0.,0.0471458586470647,0.0823534588635132),
 .UNSPECIFIED.) ;
#1193=B_SPLINE_CURVE_WITH_KNOTS('',3,(#90383,#90384,#90385,#90386,#90387,
#90388),.UNSPECIFIED.,.F.,.F.,(4,2,4),(-0.0646894582084791,-0.0581995466601206,
-0.0505532240038533),.UNSPECIFIED.) ;
#1194=B_SPLINE_CURVE_WITH_KNOTS('',3,(#90391,#90392,#90393,#90394,#90395,
#90396),.UNSPECIFIED.,.F.,.F.,(4,2,4),(-0.0279464003917075,-0.0162728575198495,
-0.00636479267613269),.UNSPECIFIED.) ;
#1195=B_SPLINE_CURVE_WITH_KNOTS('',3,(#90404,#90405,#90406,#90407,#90408,
#90409,#90410,#90411),.UNSPECIFIED.,.F.,.F.,(4,2,2,4),(-0.0463941724255825,
-0.0363335959367585,-0.0244739336232673,6.93889390390723E-18),
 .UNSPECIFIED.) ;
#1196=B_SPLINE_CURVE_WITH_KNOTS('',3,(#90438,#90439,#90440,#90441),
 .UNSPECIFIED.,.F.,.F.,(4,4),(-0.00233157716846821,0.),.UNSPECIFIED.) ;
#1197=B_SPLINE_CURVE_WITH_KNOTS('',3,(#90466,#90467,#90468,#90469,#90470,
#90471,#90472,#90473,#90474,#90475,#90476,#90477,#90478,#90479,#90480,#90481,
#90482,#90483,#90484,#90485,#90486,#90487,#90488,#90489,#90490,#90491,#90492,
#90493),.UNSPECIFIED.,.F.,.F.,(4,3,3,3,3,3,3,3,3,4),(3.21026029059551E-8,
0.00464707931025668,0.00929415862051336,0.0137678334300167,0.0156388310171345,
0.0187179653523303,0.0232666593299545,0.0251479586559353,0.0296888345732088,
0.0316724821582484),.UNSPECIFIED.) ;
#1198=B_SPLINE_CURVE_WITH_KNOTS('',3,(#90495,#90496,#90497,#90498),
 .UNSPECIFIED.,.F.,.F.,(4,4),(0.000498023522427242,0.00742046561384795),
 .UNSPECIFIED.) ;
#1199=B_SPLINE_CURVE_WITH_KNOTS('',3,(#90499,#90500,#90501,#90502,#90503,
#90504,#90505),.UNSPECIFIED.,.F.,.F.,(4,3,4),(0.00742046561384795,0.0146643599521495,
0.0162549092688308),.UNSPECIFIED.) ;
#1200=B_SPLINE_CURVE_WITH_KNOTS('',3,(#90552,#90553,#90554,#90555,#90556,
#90557),.UNSPECIFIED.,.F.,.F.,(4,2,4),(0.,0.00166959259478934,0.00333900921077541),
 .UNSPECIFIED.) ;
#1201=B_SPLINE_CURVE_WITH_KNOTS('',3,(#90565,#90566,#90567,#90568,#90569,
#90570,#90571,#90572,#90573,#90574,#90575,#90576,#90577),.UNSPECIFIED.,
 .F.,.F.,(4,3,3,3,4),(-0.0247314244030886,-0.0245013764734994,-0.0199768571653589,
-0.0156201260570807,-0.0140088579916689),.UNSPECIFIED.) ;
#1202=B_SPLINE_CURVE_WITH_KNOTS('',3,(#90579,#90580,#90581,#90582,#90583,
#90584),.UNSPECIFIED.,.F.,.F.,(4,2,4),(-0.00524067245577225,-0.00262950955895225,
0.),.UNSPECIFIED.) ;
#1203=B_SPLINE_CURVE_WITH_KNOTS('',3,(#90585,#90586,#90587,#90588,#90589,
#90590),.UNSPECIFIED.,.F.,.F.,(4,2,4),(-0.0208077196740842,-0.0103104127273635,
-0.000111699617630046),.UNSPECIFIED.) ;
#1204=B_SPLINE_CURVE_WITH_KNOTS('',3,(#90620,#90621,#90622,#90623,#90624,
#90625),.UNSPECIFIED.,.F.,.F.,(4,2,4),(-0.167893988576184,-0.139678911984281,
-0.12132773760924),.UNSPECIFIED.) ;
#1205=B_SPLINE_CURVE_WITH_KNOTS('',3,(#90711,#90712,#90713,#90714,#90715,
#90716,#90717,#90718,#90719,#90720,#90721,#90722),.UNSPECIFIED.,.F.,.F.,
(4,2,2,2,2,4),(-0.103468456759814,-0.102439814165996,-0.0469583320002097,
-0.0291854860033449,-0.010865621464627,0.),.UNSPECIFIED.) ;
#1206=B_SPLINE_CURVE_WITH_KNOTS('',3,(#90724,#90725,#90726,#90727,#90728,
#90729,#90730,#90731,#90732,#90733,#90734,#90735,#90736,#90737,#90738,#90739,
#90740,#90741,#90742,#90743,#90744,#90745,#90746,#90747,#90748,#90749,#90750,
#90751),.UNSPECIFIED.,.F.,.F.,(4,3,3,3,3,3,3,3,3,4),(-0.0929261016547975,
-0.0912735545557092,-0.0896210074566209,-0.0863159132584443,-0.0797057248620911,
-0.073095536465738,-0.0532649712766785,-0.0268242176912658,-0.0234862530524168,
-0.00123315546009042),.UNSPECIFIED.) ;
#1207=B_SPLINE_CURVE_WITH_KNOTS('',3,(#90757,#90758,#90759,#90760,#90761,
#90762),.UNSPECIFIED.,.F.,.F.,(4,2,4),(-0.0160009459236279,-0.00787429008612065,
-7.73645268326029E-6),.UNSPECIFIED.) ;
#1208=B_SPLINE_CURVE_WITH_KNOTS('',3,(#90764,#90765,#90766,#90767,#90768,
#90769,#90770,#90771),.UNSPECIFIED.,.F.,.F.,(4,2,2,4),(2.69755551674642E-5,
0.0275748103794202,0.0564582935792714,0.0567967509721843),.UNSPECIFIED.) ;
#1209=B_SPLINE_CURVE_WITH_KNOTS('',3,(#90777,#90778,#90779,#90780,#90781),
 .UNSPECIFIED.,.F.,.F.,(4,1,4),(-0.0267801877362277,-0.0114772233155261,
0.),.UNSPECIFIED.) ;
#1210=B_SPLINE_CURVE_WITH_KNOTS('',3,(#90890,#90891,#90892,#90893,#90894,
#90895),.UNSPECIFIED.,.F.,.F.,(4,2,4),(0.,0.0518624644373431,0.0522283064773341),
 .UNSPECIFIED.) ;
#1211=B_SPLINE_CURVE_WITH_KNOTS('',3,(#90896,#90897,#90898,#90899,#90900,
#90901),.UNSPECIFIED.,.F.,.F.,(4,2,4),(-0.0522283064773341,-0.0518624644373431,
0.),.UNSPECIFIED.) ;
#1212=B_SPLINE_CURVE_WITH_KNOTS('',3,(#91009,#91010,#91011,#91012),
 .UNSPECIFIED.,.F.,.F.,(4,4),(-0.051862464436985,-0.00040498540622502),
 .UNSPECIFIED.) ;
#1213=B_SPLINE_CURVE_WITH_KNOTS('',3,(#91013,#91014,#91015,#91016,#91017,
#91018),.UNSPECIFIED.,.F.,.F.,(4,2,4),(-0.00040498540622502,0.,0.000365842040355155),
 .UNSPECIFIED.) ;
#1214=B_SPLINE_CURVE_WITH_KNOTS('',3,(#91020,#91021,#91022,#91023,#91024,
#91025),.UNSPECIFIED.,.F.,.F.,(4,2,4),(-0.000365842040355155,0.,0.000404915206456683),
 .UNSPECIFIED.) ;
#1215=B_SPLINE_CURVE_WITH_KNOTS('',3,(#91026,#91027,#91028,#91029),
 .UNSPECIFIED.,.F.,.F.,(4,4),(0.000404915206456683,0.051862464436985),
 .UNSPECIFIED.) ;
#1216=B_SPLINE_CURVE_WITH_KNOTS('',3,(#91099,#91100,#91101,#91102,#91103,
#91104,#91105,#91106,#91107,#91108),.UNSPECIFIED.,.F.,.F.,(4,2,2,2,4),(-0.0248690759606685,
-0.024715611553566,-0.0142883199095518,-0.00605736591428742,0.),
 .UNSPECIFIED.) ;
#1217=B_SPLINE_CURVE_WITH_KNOTS('',3,(#91148,#91149,#91150,#91151,#91152,
#91153),.UNSPECIFIED.,.F.,.F.,(4,2,4),(-0.0617997712808834,-0.0284087068830499,
0.),.UNSPECIFIED.) ;
#1218=B_SPLINE_CURVE_WITH_KNOTS('',3,(#91310,#91311,#91312,#91313,#91314),
 .UNSPECIFIED.,.F.,.F.,(4,1,4),(0.0402140666257685,0.0595744748887569,0.0856917518795941),
 .UNSPECIFIED.) ;
#1219=B_SPLINE_CURVE_WITH_KNOTS('',3,(#91315,#91316,#91317,#91318),
 .UNSPECIFIED.,.F.,.F.,(4,4),(-0.00119196920320868,0.00853666604048891),
 .UNSPECIFIED.) ;
#1220=B_SPLINE_CURVE_WITH_KNOTS('',3,(#91335,#91336,#91337,#91338,#91339,
#91340,#91341,#91342,#91343,#91344,#91345,#91346,#91347,#91348,#91349,#91350),
 .UNSPECIFIED.,.F.,.F.,(4,2,2,2,2,2,2,4),(0.0209336302119049,0.0225603262737206,
0.0248958150254002,0.0295087749195171,0.0344155207767142,0.0391677058630032,
0.0437345723765867,0.0438833919350602),.UNSPECIFIED.) ;
#1221=B_SPLINE_CURVE_WITH_KNOTS('',3,(#91398,#91399,#91400,#91401,#91402,
#91403),.UNSPECIFIED.,.F.,.F.,(4,2,4),(-0.0194026045695604,-0.0117562819132907,
0.),.UNSPECIFIED.) ;
#1222=B_SPLINE_CURVE_WITH_KNOTS('',3,(#91489,#91490,#91491,#91492,#91493,
#91494,#91495,#91496,#91497,#91498,#91499,#91500),.UNSPECIFIED.,.F.,.F.,
(4,2,2,2,2,4),(-0.029993636019315,-0.0220228924152891,-0.0132531560003494,
-0.00562260137335941,1.54323775980458E-12,7.5349547761283E-5),
 .UNSPECIFIED.) ;
#1223=B_SPLINE_CURVE_WITH_KNOTS('',3,(#91501,#91502,#91503,#91504,#91505,
#91506),.UNSPECIFIED.,.F.,.F.,(4,1,1,4),(-0.184560397797916,-0.166722152241299,
-0.156528869066089,-0.148883906684682),.UNSPECIFIED.) ;
#1224=B_SPLINE_CURVE_WITH_KNOTS('',3,(#91507,#91508,#91509,#91510,#91511),
 .UNSPECIFIED.,.F.,.F.,(4,1,4),(0.148883906684682,0.156528869066089,0.159545911357215),
 .UNSPECIFIED.) ;
#1225=B_SPLINE_CURVE_WITH_KNOTS('',3,(#91555,#91556,#91557,#91558,#91559,
#91560),.UNSPECIFIED.,.F.,.F.,(4,2,4),(-0.0663145530984604,0.,0.000424263177439857),
 .UNSPECIFIED.) ;
#1226=B_SPLINE_CURVE_WITH_KNOTS('',3,(#91562,#91563,#91564,#91565,#91566,
#91567),.UNSPECIFIED.,.F.,.F.,(4,2,4),(-0.000424263177439857,0.,0.00584465807886479),
 .UNSPECIFIED.) ;
#1227=B_SPLINE_CURVE_WITH_KNOTS('',3,(#91568,#91569,#91570,#91571),
 .UNSPECIFIED.,.F.,.F.,(4,4),(0.00584465807886479,0.0663145530984604),
 .UNSPECIFIED.) ;
#1228=B_SPLINE_CURVE_WITH_KNOTS('',3,(#91617,#91618,#91619,#91620),
 .UNSPECIFIED.,.F.,.F.,(4,4),(-0.0254449718282482,0.),.UNSPECIFIED.) ;
#1229=B_SPLINE_CURVE_WITH_KNOTS('',3,(#91623,#91624,#91625,#91626),
 .UNSPECIFIED.,.F.,.F.,(4,4),(0.,0.0254449718282482),.UNSPECIFIED.) ;
#1230=B_SPLINE_CURVE_WITH_KNOTS('',3,(#91685,#91686,#91687,#91688,#91689,
#91690,#91691,#91692,#91693,#91694),.UNSPECIFIED.,.F.,.F.,(4,2,2,2,4),(0.,
0.00873255283564249,0.0137119265240959,0.0174485463463235,0.0174926355298175),
 .UNSPECIFIED.) ;
#1231=B_SPLINE_CURVE_WITH_KNOTS('',3,(#91698,#91699,#91700,#91701,#91702,
#91703),.UNSPECIFIED.,.F.,.F.,(4,2,4),(-0.00554349508612338,-0.00278303954230401,
-7.86527024303811E-6),.UNSPECIFIED.) ;
#1232=B_SPLINE_CURVE_WITH_KNOTS('',3,(#91793,#91794,#91795,#91796,#91797,
#91798,#91799,#91800,#91801,#91802,#91803,#91804,#91805,#91806,#91807,#91808,
#91809,#91810,#91811),.UNSPECIFIED.,.F.,.F.,(4,3,3,3,3,3,4),(0.,0.00467491259865511,
0.00948510350195526,0.0145483091112081,0.0197594621886094,0.025280122058927,
0.0297379259389668),.UNSPECIFIED.) ;
#1233=B_SPLINE_CURVE_WITH_KNOTS('',3,(#91813,#91814,#91815,#91816,#91817,
#91818,#91819),.UNSPECIFIED.,.F.,.F.,(4,3,4),(0.0297379259389668,0.0299720828361244,
0.0300731157523127),.UNSPECIFIED.) ;
#1234=B_SPLINE_CURVE_WITH_KNOTS('',3,(#91821,#91822,#91823,#91824,#91825,
#91826),.UNSPECIFIED.,.F.,.F.,(4,2,4),(-0.0300731157523127,-0.0299720828361244,
-0.0297216886550733),.UNSPECIFIED.) ;
#1235=B_SPLINE_CURVE_WITH_KNOTS('',3,(#91827,#91828,#91829,#91830),
 .UNSPECIFIED.,.F.,.F.,(4,4),(-0.0297216886550733,0.),.UNSPECIFIED.) ;
#1236=B_SPLINE_CURVE_WITH_KNOTS('',3,(#91931,#91932,#91933,#91934,#91935,
#91936,#91937,#91938,#91939,#91940),.UNSPECIFIED.,.F.,.F.,(4,2,2,2,4),(-0.0174676169376883,
-0.0173982625003064,-0.00856749914223533,-0.00158802779347854,0.),
 .UNSPECIFIED.) ;
#1237=B_SPLINE_CURVE_WITH_KNOTS('',3,(#91946,#91947,#91948,#91949),
 .UNSPECIFIED.,.F.,.F.,(4,4),(1.33431567541952E-15,0.0171168860941288),
 .UNSPECIFIED.) ;
#1238=B_SPLINE_CURVE_WITH_KNOTS('',3,(#91961,#91962,#91963,#91964,#91965,
#91966,#91967,#91968),.UNSPECIFIED.,.F.,.F.,(4,2,2,4),(-0.0256452708673575,
-0.0124292433503726,-0.00476507154092581,-9.48509615022065E-6),
 .UNSPECIFIED.) ;
#1239=B_SPLINE_CURVE_WITH_KNOTS('',3,(#91983,#91984,#91985,#91986,#91987,
#91988,#91989,#91990,#91991,#91992,#91993,#91994,#91995,#91996),
 .UNSPECIFIED.,.F.,.F.,(4,2,2,2,2,2,4),(0.0354537163355204,0.0383240848475325,
0.0418682032589909,0.0476210418726295,0.057789083784607,0.0709074326710473,
0.0712608101152448),.UNSPECIFIED.) ;
#1240=B_SPLINE_CURVE_WITH_KNOTS('',3,(#92000,#92001,#92002,#92003,#92004,
#92005,#92006,#92007,#92008,#92009,#92010,#92011,#92012,#92013),
 .UNSPECIFIED.,.F.,.F.,(4,2,2,2,2,2,4),(-0.0354537163167348,-0.0325833478064478,
-0.0290392293972437,-0.0232863907872553,-0.013118348881858,0.,0.000353377444176431),
 .UNSPECIFIED.) ;
#1241=B_SPLINE_CURVE_WITH_KNOTS('',3,(#92066,#92067,#92068,#92069,#92070,
#92071,#92072,#92073,#92074,#92075,#92076,#92077,#92078,#92079,#92080,#92081,
#92082,#92083,#92084,#92085,#92086,#92087),.UNSPECIFIED.,.F.,.F.,(4,3,3,
3,3,3,3,4),(-0.0477209576750425,-0.0468497353395086,-0.0434194841369138,
-0.0391915106912518,-0.0334700977178844,-0.0309360218424187,-0.0293311245511305,
-0.0287682560648015),.UNSPECIFIED.) ;
#1242=B_SPLINE_CURVE_WITH_KNOTS('',3,(#92227,#92228,#92229,#92230,#92231,
#92232),.UNSPECIFIED.,.F.,.F.,(4,2,4),(0.,0.0117562819132905,0.0194026045695574),
 .UNSPECIFIED.) ;
#1243=B_SPLINE_CURVE_WITH_KNOTS('',3,(#92236,#92237,#92238,#92239,#92240,
#92241),.UNSPECIFIED.,.F.,.F.,(4,2,4),(0.0505532240038504,0.0581995466601177,
0.0699558285734079),.UNSPECIFIED.) ;
#1244=B_SPLINE_CURVE_WITH_KNOTS('',3,(#92268,#92269,#92270,#92271,#92272,
#92273,#92274),.UNSPECIFIED.,.F.,.F.,(4,3,4),(-0.129427938726121,-0.00760184093280492,
-9.99999994838463E-7),.UNSPECIFIED.) ;
#1245=B_SPLINE_CURVE_WITH_KNOTS('',3,(#92411,#92412,#92413,#92414,#92415,
#92416),.UNSPECIFIED.,.F.,.F.,(4,2,4),(-0.0699558285734104,-0.0581995466601188,
-0.0505532240038526),.UNSPECIFIED.) ;
#1246=B_SPLINE_CURVE_WITH_KNOTS('',3,(#92435,#92436,#92437,#92438,#92439,
#92440),.UNSPECIFIED.,.F.,.F.,(4,2,4),(-0.0194026045695577,-0.0117562819132915,
0.),.UNSPECIFIED.) ;
#1247=B_SPLINE_CURVE_WITH_KNOTS('',3,(#92443,#92444,#92445,#92446,#92447,
#92448),.UNSPECIFIED.,.F.,.F.,(4,2,4),(-0.0194026045695576,-0.01175628191329,
0.),.UNSPECIFIED.) ;
#1248=B_SPLINE_CURVE_WITH_KNOTS('',3,(#92558,#92559,#92560,#92561,#92562,
#92563,#92564,#92565),.UNSPECIFIED.,.F.,.F.,(4,1,1,1,1,4),(-0.0400607966507765,
-0.0286148547505547,-0.0171689128503328,-0.0114459419002219,-0.00572297095011093,
-9.19824141439016E-31),.UNSPECIFIED.) ;
#1249=B_SPLINE_CURVE_WITH_KNOTS('',3,(#92568,#92569,#92570,#92571,#92572,
#92573,#92574,#92575),.UNSPECIFIED.,.F.,.F.,(4,1,1,1,1,4),(9.19824141439016E-31,
0.00572297095011093,0.0114459419002219,0.0171689128503328,0.0286148547505547,
0.0400607966507765),.UNSPECIFIED.) ;
#1250=B_SPLINE_CURVE_WITH_KNOTS('',3,(#92582,#92583,#92584,#92585,#92586,
#92587,#92588,#92589,#92590,#92591,#92592,#92593,#92594,#92595,#92596,#92597,
#92598,#92599,#92600),.UNSPECIFIED.,.F.,.F.,(4,3,3,3,3,3,4),(0.0252869589686981,
0.0279002827276299,0.0312075970894694,0.0359392781305207,0.0430930520183015,
0.0490510238207101,0.049573752749312),.UNSPECIFIED.) ;
#1251=B_SPLINE_CURVE_WITH_KNOTS('',3,(#92669,#92670,#92671,#92672,#92673,
#92674,#92675,#92676,#92677,#92678,#92679,#92680,#92681,#92682),
 .UNSPECIFIED.,.F.,.F.,(4,2,2,2,2,2,4),(-0.0293717278535513,-0.0114851593454505,
-0.00300187054344729,-0.00150093527172364,-0.00075046763586182,-0.000375233817930908,
3.46944695195361E-18),.UNSPECIFIED.) ;
#1252=B_SPLINE_CURVE_WITH_KNOTS('',3,(#92810,#92811,#92812,#92813,#92814,
#92815,#92816,#92817,#92818,#92819,#92820,#92821,#92822,#92823,#92824,#92825,
#92826,#92827,#92828,#92829,#92830,#92831,#92832,#92833,#92834),
 .UNSPECIFIED.,.F.,.F.,(4,3,3,3,3,3,3,3,4),(6.85291849789822E-5,0.00224825149847016,
0.00410846025809801,0.00699382185291758,0.00799199065054034,0.0109464436869959,
0.0118449474474184,0.014171090431278,0.0157080392133692),.UNSPECIFIED.) ;
#1253=B_SPLINE_CURVE_WITH_KNOTS('',3,(#92835,#92836,#92837,#92838),
 .UNSPECIFIED.,.F.,.F.,(4,4),(-7.29056287534871E-5,6.85291849789822E-5),
 .UNSPECIFIED.) ;
#1254=B_SPLINE_CURVE_WITH_KNOTS('',3,(#92897,#92898,#92899,#92900),
 .UNSPECIFIED.,.F.,.F.,(4,4),(2.15310365171961E-15,0.0294983491188769),
 .UNSPECIFIED.) ;
#1255=B_SPLINE_CURVE_WITH_KNOTS('',3,(#92936,#92937,#92938,#92939,#92940,
#92941,#92942,#92943,#92944,#92945,#92946,#92947,#92948,#92949,#92950,#92951,
#92952,#92953,#92954,#92955,#92956,#92957,#92958,#92959,#92960),
 .UNSPECIFIED.,.F.,.F.,(4,3,3,3,3,3,3,3,4),(8.270742692011E-19,0.0056026191517687,
0.0117794878631444,0.0162039536314463,0.0221619695143852,0.0231485051877804,
0.0273176591774019,0.0314713233612342,0.0324079072628925),.UNSPECIFIED.) ;
#1256=B_SPLINE_CURVE_WITH_KNOTS('',3,(#92963,#92964,#92965,#92966,#92967,
#92968),.UNSPECIFIED.,.F.,.F.,(4,1,1,4),(-0.0324079072628925,-0.0231485051877804,
-0.0162039536314463,-8.270742692011E-19),.UNSPECIFIED.) ;
#1257=B_SPLINE_CURVE_WITH_KNOTS('',3,(#93034,#93035,#93036,#93037,#93038,
#93039,#93040,#93041,#93042,#93043,#93044,#93045,#93046,#93047,#93048,#93049,
#93050,#93051,#93052,#93053,#93054,#93055,#93056,#93057,#93058),
 .UNSPECIFIED.,.F.,.F.,(4,3,3,3,3,3,3,3,4),(0.,0.00415188905280238,0.00832027739506051,
0.00925932038092611,0.0152172958024042,0.0162038106666207,0.0224596241657163,
0.0281435224497628,0.032407621333235),.UNSPECIFIED.) ;
#1258=B_SPLINE_CURVE_WITH_KNOTS('',3,(#93062,#93063,#93064,#93065,#93066,
#93067),.UNSPECIFIED.,.F.,.F.,(4,1,1,4),(-0.0324076213332414,-0.0162038106666207,
-0.00925932038092611,0.),.UNSPECIFIED.) ;
#1259=B_SPLINE_CURVE_WITH_KNOTS('',3,(#93111,#93112,#93113,#93114,#93115),
 .UNSPECIFIED.,.F.,.F.,(4,1,4),(-0.0294932405228361,-0.0126399602240726,
0.),.UNSPECIFIED.) ;
#1260=B_SPLINE_CURVE_WITH_KNOTS('',3,(#93116,#93117,#93118,#93119,#93120),
 .UNSPECIFIED.,.F.,.F.,(4,1,4),(0.,0.0126399602240726,0.0294932405228361),
 .UNSPECIFIED.) ;
#1261=B_SPLINE_CURVE_WITH_KNOTS('',3,(#93255,#93256,#93257,#93258,#93259),
 .UNSPECIFIED.,.F.,.F.,(4,1,4),(-0.0294932405474481,-0.0168532803128275,
0.),.UNSPECIFIED.) ;
#1262=B_SPLINE_CURVE_WITH_KNOTS('',3,(#93261,#93262,#93263,#93264,#93265),
 .UNSPECIFIED.,.F.,.F.,(4,1,4),(0.,0.0168532803128275,0.0294932405474481),
 .UNSPECIFIED.) ;
#1263=B_SPLINE_CURVE_WITH_KNOTS('',3,(#93300,#93301,#93302,#93303),
 .UNSPECIFIED.,.F.,.F.,(4,4),(0.,0.0936141811972385),.UNSPECIFIED.) ;
#1264=B_SPLINE_CURVE_WITH_KNOTS('',3,(#93679,#93680,#93681,#93682),
 .UNSPECIFIED.,.F.,.F.,(4,4),(-0.0294983491188769,-2.15310365171961E-15),
 .UNSPECIFIED.) ;
#1265=B_SPLINE_CURVE_WITH_KNOTS('',3,(#93820,#93821,#93822,#93823,#93824,
#93825,#93826,#93827,#93828,#93829,#93830,#93831,#93832,#93833,#93834,#93835,
#93836,#93837,#93838,#93839,#93840,#93841,#93842),.UNSPECIFIED.,.F.,.F.,
(4,2,1,1,1,1,1,1,1,1,1,1,1,1,1,1,1,1,1,4),(-0.158000078699635,-0.148000078699544,
-0.12685721031389,-0.116285776121063,-0.105714341928236,-0.105053627291185,
-0.104392912654133,-0.100428624831823,-0.0951429077354094,-0.0845714735425825,
-0.079285756446169,-0.0766428978979623,-0.0759821832609106,-0.0753214686238589,
-0.0746607539868073,-0.0740000393497556,-0.0634286051569287,-0.0422857367712749,
-0.0211428683856211,-0.0100909341248642),.UNSPECIFIED.) ;
#1266=B_SPLINE_CURVE_WITH_KNOTS('',3,(#93846,#93847,#93848,#93849,#93850,
#93851,#93852,#93853,#93854,#93855,#93856),.UNSPECIFIED.,.F.,.F.,(4,1,1,
1,1,1,2,4),(-0.208459662581221,-0.179372878146882,-0.155976415779898,-0.124781132623918,
-0.0935858494679386,-0.062390566311959,0.,0.0100000000000179),
 .UNSPECIFIED.) ;
#1267=B_SPLINE_CURVE_WITH_KNOTS('',3,(#93872,#93873,#93874,#93875,#93876,
#93877,#93878,#93879,#93880,#93881,#93882,#93883,#93884,#93885,#93886,#93887),
 .UNSPECIFIED.,.F.,.F.,(4,2,1,1,1,1,1,1,1,1,1,1,4),(-0.168369812149447,
-0.158369812149344,-0.135745553270846,-0.113121294392348,-0.107465229672724,
-0.101809164953099,-0.0961531002334749,-0.0904970355138505,-0.084840970794226,
-0.0791849060746015,-0.0678727766353526,-0.0226242588783568,-0.0102825850151437),
 .UNSPECIFIED.) ;
#1268=B_SPLINE_CURVE_WITH_KNOTS('',3,(#93891,#93892,#93893,#93894,#93895,
#93896,#93897,#93898,#93899,#93900,#93901),.UNSPECIFIED.,.F.,.F.,(4,1,1,
1,1,1,2,4),(-0.206302611384505,-0.177449514196477,-0.154303925388241,-0.123443140310593,
-0.0925823552329445,-0.0617215701552963,0.,0.0100000000001109),
 .UNSPECIFIED.) ;
#1269=B_SPLINE_CURVE_WITH_KNOTS('',3,(#94047,#94048,#94049,#94050,#94051),
 .UNSPECIFIED.,.F.,.F.,(4,1,4),(-0.045647970439003,-0.0195634159024299,
0.),.UNSPECIFIED.) ;
#1270=B_SPLINE_CURVE_WITH_KNOTS('',3,(#94052,#94053,#94054,#94055,#94056,
#94057,#94058,#94059,#94060,#94061,#94062,#94063,#94064,#94065,#94066,#94067,
#94068,#94069,#94070,#94071,#94072,#94073,#94074,#94075,#94076,#94077,#94078,
#94079),.UNSPECIFIED.,.F.,.F.,(4,3,3,3,3,3,3,3,3,4),(0.,0.00537990329643797,
0.0110107587247129,0.017075331585266,0.0195634159024299,0.0256456020000555,
0.0315029066657429,0.0371776636413155,0.0425892624415814,0.045647970439003),
 .UNSPECIFIED.) ;
#1271=B_SPLINE_CURVE_WITH_KNOTS('',3,(#94152,#94153,#94154,#94155),
 .UNSPECIFIED.,.F.,.F.,(4,4),(-0.0171168860941288,-1.33431567541952E-15),
 .UNSPECIFIED.) ;
#1272=B_SPLINE_CURVE_WITH_KNOTS('',3,(#94179,#94180,#94181,#94182,#94183,
#94184,#94185,#94186,#94187,#94188,#94189,#94190,#94191),.UNSPECIFIED.,
 .F.,.F.,(4,3,3,3,4),(0.530502305869095,0.542967004358727,0.555197283003313,
0.567168185545784,0.569716944924395),.UNSPECIFIED.) ;
#1273=B_SPLINE_CURVE_WITH_KNOTS('',3,(#94243,#94244,#94245,#94246),
 .UNSPECIFIED.,.F.,.F.,(4,4),(0.0564440131838686,0.109806780005479),
 .UNSPECIFIED.) ;
#1274=B_SPLINE_CURVE_WITH_KNOTS('',3,(#94317,#94318,#94319,#94320,#94321,
#94322,#94323,#94324,#94325,#94326,#94327,#94328,#94329,#94330,#94331,#94332,
#94333,#94334,#94335,#94336,#94337,#94338,#94339,#94340,#94341,#94342,#94343,
#94344),.UNSPECIFIED.,.F.,.F.,(4,3,3,3,3,3,3,3,3,4),(1.1236943236576E-6,
0.00317388582283794,0.00628350468964704,0.00935335072246934,0.0114772233155261,
0.0148928133883393,0.0183304301194573,0.0217988007428664,0.0253473022429601,
0.0267801877362277),.UNSPECIFIED.) ;
#1275=B_SPLINE_CURVE_WITH_KNOTS('',3,(#94412,#94413,#94414,#94415,#94416,
#94417,#94418,#94419,#94420,#94421,#94422,#94423),.UNSPECIFIED.,.F.,.F.,
(4,2,2,2,2,4),(0.,0.00818348889632409,0.0162723371528994,0.0205125633057343,
0.0248544226127729,0.0249813220785652),.UNSPECIFIED.) ;
#1276=B_SPLINE_CURVE_WITH_KNOTS('',3,(#94424,#94425,#94426,#94427,#94428),
 .UNSPECIFIED.,.F.,.F.,(4,1,4),(-0.0856917518795941,-0.0595744748887569,
-0.0334715043589776),.UNSPECIFIED.) ;
#1277=B_SPLINE_CURVE_WITH_KNOTS('',3,(#94433,#94434,#94435,#94436),
 .UNSPECIFIED.,.F.,.F.,(4,4),(0.,0.0936131112963941),.UNSPECIFIED.) ;
#1278=B_SPLINE_CURVE_WITH_KNOTS('',3,(#94440,#94441,#94442,#94443),
 .UNSPECIFIED.,.F.,.F.,(4,4),(0.,0.0936141814749616),.UNSPECIFIED.) ;
#1279=B_SPLINE_CURVE_WITH_KNOTS('',3,(#94541,#94542,#94543,#94544,#94545,
#94546,#94547,#94548,#94549,#94550,#94551,#94552,#94553,#94554,#94555,#94556,
#94557,#94558),.UNSPECIFIED.,.F.,.F.,(4,2,2,2,2,2,2,2,4),(-0.0223129172590684,
-0.0168544066118854,-0.0114714787709719,-0.0065572365263978,-0.00563951438992895,
-0.0049148380277049,-0.00389243501027995,-0.00207747054762647,-9.5473990429501E-7),
 .UNSPECIFIED.) ;
#1280=B_SPLINE_CURVE_WITH_KNOTS('',3,(#94673,#94674,#94675,#94676,#94677,
#94678,#94679,#94680,#94681,#94682),.UNSPECIFIED.,.F.,.F.,(4,2,2,2,4),(-0.0146631250948371,
-0.00714591699534451,-0.00307413779860312,-0.00137081844245783,-2.36480237567184E-5),
 .UNSPECIFIED.) ;
#1281=B_SPLINE_CURVE_WITH_KNOTS('',3,(#94794,#94795,#94796,#94797),
 .UNSPECIFIED.,.F.,.F.,(4,4),(-0.341768486244514,-0.318230893672861),
 .UNSPECIFIED.) ;
#1282=B_SPLINE_CURVE_WITH_KNOTS('',3,(#94800,#94801,#94802,#94803),
 .UNSPECIFIED.,.F.,.F.,(4,4),(0.318228890765255,0.341768504405115),
 .UNSPECIFIED.) ;
#1283=B_SPLINE_CURVE_WITH_KNOTS('',3,(#94810,#94811,#94812,#94813,#94814,
#94815,#94816,#94817,#94818,#94819,#94820,#94821,#94822),.UNSPECIFIED.,
 .F.,.F.,(4,3,3,3,4),(0.110165078811181,0.122187579457333,0.134390211284239,
0.146912945246986,0.149379717866476),.UNSPECIFIED.) ;
#1284=B_SPLINE_CURVE_WITH_KNOTS('',3,(#94880,#94881,#94882,#94883,#94884,
#94885,#94886),.UNSPECIFIED.,.F.,.F.,(4,3,4),(-0.143004044169051,-0.0211094711173082,
-9.99999994338863E-7),.UNSPECIFIED.) ;
#1285=B_SPLINE_CURVE_WITH_KNOTS('',3,(#94957,#94958,#94959,#94960,#94961,
#94962,#94963,#94964,#94965,#94966,#94967,#94968,#94969,#94970),
 .UNSPECIFIED.,.F.,.F.,(4,2,2,2,2,2,4),(-0.000104155204377971,-3.86217593415514E-11,
0.00490122913929789,0.009484123212302,0.014276465079669,0.0171575682197624,
0.0199062496531735),.UNSPECIFIED.) ;
#1286=B_SPLINE_CURVE_WITH_KNOTS('',3,(#95025,#95026,#95027,#95028,#95029,
#95030,#95031,#95032,#95033,#95034),.UNSPECIFIED.,.F.,.F.,(4,1,1,1,1,1,
1,4),(-0.0100926828333812,0.0417412101282966,0.0676581566091356,0.0935751030899745,
0.106533576330394,0.119492049570813,0.132450522811233,0.161355759040101),
 .UNSPECIFIED.) ;
#1287=B_SPLINE_CURVE_WITH_KNOTS('',3,(#95036,#95037,#95038,#95039,#95040,
#95041,#95042,#95043,#95044,#95045,#95046,#95047,#95048,#95049),
 .UNSPECIFIED.,.F.,.F.,(4,2,2,2,2,2,4),(-0.00010162007045407,0.,0.00486299775130735,
0.00944029817878617,0.014181595291943,0.0169882395959943,0.0196725193024137),
 .UNSPECIFIED.) ;
#1288=B_SPLINE_CURVE_WITH_KNOTS('',3,(#95050,#95051,#95052,#95053,#95054,
#95055,#95056,#95057,#95058,#95059,#95060,#95061,#95062,#95063,#95064,#95065,
#95066,#95067,#95068,#95069,#95070,#95071,#95072,#95073,#95074,#95075,#95076,
#95077,#95078,#95079,#95080,#95081,#95082,#95083,#95084,#95085,#95086,#95087,
#95088,#95089,#95090,#95091,#95092,#95093,#95094,#95095,#95096,#95097,#95098,
#95099,#95100,#95101,#95102,#95103,#95104,#95105,#95106,#95107,#95108,#95109,
#95110,#95111,#95112,#95113,#95114,#95115,#95116,#95117,#95118,#95119,#95120,
#95121,#95122,#95123,#95124,#95125,#95126,#95127,#95128,#95129,#95130,#95131,
#95132,#95133,#95134,#95135,#95136,#95137,#95138,#95139,#95140,#95141,#95142,
#95143,#95144,#95145,#95146,#95147,#95148,#95149,#95150,#95151,#95152,#95153,
#95154,#95155),.UNSPECIFIED.,.F.,.F.,(4,3,3,3,3,3,3,3,3,3,3,3,3,3,3,3,3,
3,3,3,3,3,3,3,3,3,3,3,3,3,3,3,3,3,3,4),(-0.171325942532491,-0.165652411514985,
-0.160023962991389,-0.154439365331305,-0.148893369077348,-0.143356525209383,
-0.137846834510568,-0.132450522811233,-0.128972714613851,-0.125830929486734,
-0.12198716027631,-0.119492049570813,-0.114252996717646,-0.109668825471125,
-0.107349770539937,-0.105445902026418,-0.101635560910071,-0.097921982835525,
-0.0947866325002212,-0.0930504505530208,-0.0883568045689103,-0.0833681805307477,
-0.0778844727423146,-0.0775796267454788,-0.0727306918766619,-0.068184815437146,
-0.0667474756601821,-0.0611266349681567,-0.0551249595064378,-0.0486421623061817,
-0.04256147562346,-0.0393563002552848,-0.0299724411047558,-0.0185906216435956,
-0.000936915493295949,3.33115559203421E-6),.UNSPECIFIED.) ;
#1289=B_SPLINE_CURVE_WITH_KNOTS('',3,(#95160,#95161,#95162,#95163,#95164,
#95165,#95166,#95167,#95168,#95169,#95170,#95171,#95172,#95173),
 .UNSPECIFIED.,.F.,.F.,(4,2,2,2,2,2,4),(-0.0178788923403474,-0.0177845502863682,
-0.0133934732125181,-0.00931791430816039,-0.00505589452225569,-0.00246766909513425,
0.),.UNSPECIFIED.) ;
#1290=B_SPLINE_CURVE_WITH_KNOTS('',3,(#95231,#95232,#95233,#95234,#95235,
#95236,#95237,#95238,#95239,#95240,#95241),.UNSPECIFIED.,.F.,.F.,(4,1,1,
1,1,1,1,1,4),(-0.195028884511668,-0.161022259696524,-0.146383872451384,
-0.117107097961104,-0.0878303234708248,-0.073191936225685,-0.0585535489805452,
-0.0292767744902657,1.38391897109284E-14),.UNSPECIFIED.) ;
#1291=B_SPLINE_CURVE_WITH_KNOTS('',3,(#95243,#95244,#95245,#95246,#95247,
#95248,#95249,#95250,#95251,#95252,#95253),.UNSPECIFIED.,.F.,.F.,(4,1,1,
1,1,1,1,1,4),(0.0100076242561881,0.0292767744902657,0.0585535489805452,
0.073191936225685,0.0878303234708248,0.117107097961104,0.146383872451384,
0.161022259696524,0.204937421431943),.UNSPECIFIED.) ;
#1292=B_SPLINE_CURVE_WITH_KNOTS('',3,(#95254,#95255,#95256,#95257,#95258,
#95259,#95260,#95261,#95262,#95263,#95264,#95265,#95266,#95267),
 .UNSPECIFIED.,.F.,.F.,(4,2,2,2,2,2,4),(-0.017736256622245,-0.0176440568681958,
-0.0132953764850671,-0.00922540700529897,-0.00498067116082595,-0.0024336851353481,
0.),.UNSPECIFIED.) ;
#1293=B_SPLINE_CURVE_WITH_KNOTS('',3,(#95384,#95385,#95386,#95387,#95388,
#95389,#95390,#95391,#95392,#95393,#95394,#95395,#95396,#95397,#95398,#95399),
 .UNSPECIFIED.,.F.,.F.,(4,1,1,1,1,1,1,1,1,1,1,1,1,4),(0.01000334021752,
0.0295575519591679,0.059115103918338,0.088672655877508,0.118230207836678,
0.119153881335402,0.120077554834126,0.121924901831574,0.125619595826471,
0.133008983816263,0.140398371806056,0.144093065800952,0.147787759795848,
0.206902863714188),.UNSPECIFIED.) ;
#1294=B_SPLINE_CURVE_WITH_KNOTS('',3,(#95401,#95402,#95403,#95404,#95405,
#95406,#95407,#95408,#95409,#95410,#95411,#95412,#95413,#95414),
 .UNSPECIFIED.,.F.,.F.,(4,2,2,2,2,2,4),(-0.0176827121873784,-0.0175909062599249,
-0.0132508379959276,-0.00918624532464143,-0.00495893130814665,-0.0024252092698044,
0.),.UNSPECIFIED.) ;
#1295=B_SPLINE_CURVE_WITH_KNOTS('',3,(#95416,#95417,#95418,#95419,#95420,
#95421,#95422,#95423,#95424,#95425,#95426,#95427,#95428,#95429,#95430,#95431,
#95432,#95433,#95434,#95435,#95436,#95437,#95438,#95439,#95440,#95441,#95442,
#95443,#95444,#95445,#95446,#95447,#95448,#95449,#95450,#95451,#95452,#95453,
#95454,#95455,#95456,#95457,#95458,#95459,#95460,#95461,#95462,#95463,#95464,
#95465,#95466,#95467,#95468,#95469,#95470,#95471,#95472,#95473,#95474,#95475,
#95476,#95477,#95478,#95479,#95480,#95481,#95482,#95483,#95484,#95485,#95486,
#95487,#95488,#95489,#95490,#95491,#95492,#95493,#95494,#95495,#95496,#95497,
#95498,#95499,#95500,#95501,#95502,#95503,#95504,#95505,#95506,#95507,#95508,
#95509,#95510,#95511,#95512,#95513,#95514,#95515,#95516,#95517,#95518,#95519,
#95520,#95521),.UNSPECIFIED.,.F.,.F.,(4,3,3,3,3,3,3,3,3,3,3,3,3,3,3,3,3,
3,3,3,3,3,3,3,3,3,3,3,3,3,3,3,3,3,3,4),(-0.197162523347665,-0.185428221805325,
-0.172815072988371,-0.162883491013023,-0.154392034322415,-0.147787759795848,
-0.144093065800952,-0.140386955559284,-0.137815595832713,-0.133734101190473,
-0.130078332958677,-0.123836669195403,-0.121279913284718,-0.119931182187908,
-0.118936648793649,-0.117861366913671,-0.111884404652618,-0.105224027606823,
-0.0981642867190361,-0.0928694810531958,-0.0898789028134254,-0.0874314612044946,
-0.0809167123108539,-0.0769850640556748,-0.0673619310487152,-0.0631518103581704,
-0.0595014740038858,-0.0579656444507446,-0.0507199388944013,-0.0432381492298856,
-0.0354523555092146,-0.0296634974360258,-0.0257462330660413,-0.0158461536836325,
-0.00541231684862231,2.12204013797473E-15),.UNSPECIFIED.) ;
#1296=B_SPLINE_CURVE_WITH_KNOTS('',3,(#95522,#95523,#95524,#95525,#95526,
#95527,#95528,#95529,#95530,#95531,#95532,#95533,#95534,#95535),
 .UNSPECIFIED.,.F.,.F.,(4,2,2,2,2,2,4),(-0.0178405879764861,-0.0177469544214278,
-0.0133665397468608,-0.00928874858233894,-0.00503211426553545,-0.00245657296492195,
0.),.UNSPECIFIED.) ;
#1297=B_SPLINE_CURVE_WITH_KNOTS('',3,(#95559,#95560,#95561,#95562,#95563,
#95564,#95565,#95566,#95567,#95568,#95569,#95570,#95571,#95572),
 .UNSPECIFIED.,.F.,.F.,(4,2,2,2,2,2,4),(-0.000105117782515234,0.,0.00493324992095991,
0.00954507006010922,0.0143873118328074,0.0173002157143566,0.0200732442869903),
 .UNSPECIFIED.) ;
#1298=B_SPLINE_CURVE_WITH_KNOTS('',3,(#95639,#95640,#95641,#95642,#95643,
#95644,#95645,#95646,#95647,#95648,#95649,#95650,#95651,#95652,#95653,#95654,
#95655,#95656,#95657,#95658,#95659,#95660,#95661,#95662,#95663,#95664,#95665,
#95666,#95667,#95668,#95669,#95670,#95671,#95672,#95673,#95674,#95675,#95676,
#95677,#95678,#95679,#95680,#95681,#95682,#95683,#95684,#95685,#95686,#95687,
#95688,#95689,#95690,#95691,#95692,#95693,#95694,#95695,#95696,#95697,#95698,
#95699,#95700,#95701,#95702,#95703,#95704,#95705,#95706,#95707,#95708,#95709,
#95710,#95711,#95712,#95713,#95714,#95715,#95716,#95717,#95718,#95719,#95720,
#95721,#95722,#95723,#95724,#95725,#95726,#95727,#95728,#95729,#95730,#95731,
#95732,#95733,#95734,#95735,#95736,#95737,#95738,#95739,#95740,#95741,#95742,
#95743,#95744,#95745,#95746,#95747,#95748,#95749,#95750,#95751,#95752,#95753),
 .UNSPECIFIED.,.F.,.F.,(4,3,3,3,3,3,3,3,3,3,3,3,3,3,3,3,3,3,3,3,3,3,3,3,
3,3,3,3,3,3,3,3,3,3,3,3,3,3,4),(-0.177215824581903,-0.17030695155021,-0.163618926693659,
-0.157169053165717,-0.152969641660887,-0.150909770118349,-0.149305581657313,
-0.143934851050869,-0.138734177892587,-0.133779971680493,-0.131601954446486,
-0.126404873939755,-0.124975937434575,-0.123838209813924,-0.123095140176218,
-0.119886853024125,-0.116610406055776,-0.113180338591535,-0.109502458713641,
-0.105676366361172,-0.102113043504167,-0.0987197845521641,-0.0967028274534084,
-0.0925150665588207,-0.0881219492072544,-0.0833340779411559,-0.0809205515762085,
-0.080118735865623,-0.0767815667188522,-0.0723071648618782,-0.0689908285233252,
-0.0628516389877999,-0.0566815075547967,-0.0496779741197332,-0.0422255974286259,
-0.0327088895574629,-0.0209856075626229,-0.00903256831842716,8.12739771206159E-6),
 .UNSPECIFIED.) ;
#1299=B_SPLINE_CURVE_WITH_KNOTS('',3,(#95755,#95756,#95757,#95758,#95759,
#95760,#95761,#95762,#95763,#95764,#95765,#95766,#95767),.UNSPECIFIED.,
 .F.,.F.,(4,1,1,1,1,1,1,1,1,1,4),(-0.010282001904707,0.043288805662896,
0.0566815075547967,0.0633778585007471,0.0700742094466975,0.0767705603926478,
0.080118735865623,0.0968596132304989,0.1236450170143,0.150430420798102,
0.167188433543675),.UNSPECIFIED.) ;
#1300=B_SPLINE_CURVE_WITH_KNOTS('',3,(#95768,#95769,#95770,#95771,#95772,
#95773,#95774,#95775,#95776,#95777,#95778,#95779,#95780,#95781),
 .UNSPECIFIED.,.F.,.F.,(4,2,2,2,2,2,4),(-0.000101449588089462,0.,0.00483514941605568,
0.00939524326714808,0.0141515681069081,0.0169776746522734,0.0196788154735788),
 .UNSPECIFIED.) ;
#1301=B_SPLINE_CURVE_WITH_KNOTS('',3,(#95813,#95814,#95815,#95816,#95817,
#95818,#95819,#95820,#95821,#95822,#95823,#95824,#95825,#95826,#95827,#95828,
#95829,#95830,#95831,#95832,#95833,#95834,#95835,#95836,#95837,#95838,#95839,
#95840,#95841,#95842,#95843,#95844,#95845,#95846,#95847,#95848,#95849,#95850,
#95851,#95852,#95853,#95854,#95855,#95856,#95857,#95858,#95859,#95860,#95861,
#95862,#95863,#95864,#95865,#95866,#95867,#95868,#95869,#95870,#95871,#95872,
#95873,#95874,#95875,#95876,#95877,#95878,#95879,#95880,#95881,#95882,#95883,
#95884,#95885,#95886,#95887,#95888,#95889,#95890,#95891,#95892,#95893,#95894,
#95895,#95896,#95897,#95898,#95899,#95900,#95901,#95902,#95903,#95904,#95905,
#95906,#95907,#95908,#95909,#95910,#95911,#95912,#95913,#95914,#95915,#95916,
#95917,#95918,#95919,#95920,#95921,#95922,#95923,#95924,#95925,#95926,#95927,
#95928,#95929,#95930,#95931,#95932,#95933,#95934,#95935,#95936,#95937,#95938,
#95939,#95940,#95941,#95942,#95943,#95944,#95945,#95946,#95947,#95948,#95949,
#95950,#95951,#95952,#95953,#95954,#95955,#95956,#95957,#95958,#95959,#95960,
#95961,#95962,#95963),.UNSPECIFIED.,.F.,.F.,(4,3,3,3,3,3,3,3,3,3,3,3,3,
3,3,3,3,3,3,3,3,3,3,3,3,3,3,3,3,3,3,3,3,3,3,3,3,3,3,3,3,3,3,3,3,3,3,3,3,
3,4),(-1.41081590854242E-13,0.0103491921525447,0.0211841901626651,0.0241620336586163,
0.0346906689700701,0.043243695236957,0.0509049151551453,0.0579592044052852,
0.0640311579531103,0.0672167264441228,0.0701609156160853,0.074589955199646,
0.0784184868981158,0.080000656512071,0.0822470185965856,0.0846286186319091,
0.0882902149729238,0.0901096689174299,0.0910088738799008,0.0929106796275256,
0.094767296982211,0.0956149406062722,0.0964897141933299,0.0980072157210099,
0.0995495458830169,0.101158309464652,0.101720958003161,0.102190952996405,
0.103858756677589,0.10544844525405,0.106942574357921,0.107537144758825,
0.109524324640222,0.111493613001422,0.11271545936729,0.113638792421966,
0.117087933645678,0.117401478085021,0.120526599485897,0.123807081707708,
0.127250293897731,0.13085310602188,0.134301105123365,0.135464756099362,
0.136301990452286,0.142360570616147,0.148621853955712,0.153529476394735,
0.155984145694832,0.157726358513963,0.158437098833759),.UNSPECIFIED.) ;
#1302=B_SPLINE_CURVE_WITH_KNOTS('',3,(#95990,#95991,#95992,#95993,#95994,
#95995,#95996,#95997,#95998,#95999,#96000,#96001,#96002,#96003,#96004,#96005,
#96006,#96007,#96008,#96009,#96010,#96011,#96012,#96013,#96014,#96015,#96016,
#96017,#96018,#96019,#96020,#96021,#96022,#96023,#96024,#96025,#96026,#96027,
#96028,#96029,#96030,#96031,#96032,#96033,#96034,#96035,#96036,#96037,#96038,
#96039,#96040,#96041,#96042,#96043,#96044,#96045,#96046,#96047,#96048,#96049,
#96050,#96051,#96052,#96053,#96054,#96055,#96056,#96057,#96058,#96059,#96060,
#96061,#96062,#96063,#96064,#96065,#96066,#96067,#96068,#96069,#96070,#96071,
#96072,#96073,#96074),.UNSPECIFIED.,.F.,.F.,(4,3,3,3,3,3,3,3,3,3,3,3,3,
3,3,3,3,3,3,3,3,3,3,3,3,3,3,3,4),(7.39226184629487E-5,0.0136598058106041,
0.0271262719666971,0.0405296849046172,0.0524208783693001,0.0614937185449666,
0.0634789335509413,0.0767258083011943,0.0880944587633485,0.0913698481542741,
0.0927499368255514,0.100385237169618,0.108120428760434,0.115978104732835,
0.121432471043905,0.126347332023278,0.134910688538487,0.143620005971135,
0.151284213182461,0.153901104284404,0.155875512280353,0.15796612950932,
0.16550652664177,0.171821397754491,0.177387753248743,0.180427948441218,
0.190045700231785,0.202346657648098,0.216025495543537),.UNSPECIFIED.) ;
#1303=B_SPLINE_CURVE_WITH_KNOTS('',3,(#96592,#96593,#96594,#96595,#96596,
#96597,#96598,#96599,#96600,#96601,#96602,#96603,#96604,#96605),
 .UNSPECIFIED.,.F.,.F.,(4,2,2,2,2,2,4),(-0.0176214355467283,-0.017530501859727,
-0.0132488502937593,-0.00923793408389468,-0.00503892175603895,-0.00245939376250771,
0.),.UNSPECIFIED.) ;
#1304=B_SPLINE_CURVE_WITH_KNOTS('',3,(#96607,#96608,#96609,#96610,#96611,
#96612,#96613,#96614,#96615,#96616,#96617,#96618,#96619,#96620,#96621,#96622,
#96623,#96624,#96625,#96626,#96627,#96628,#96629,#96630,#96631,#96632,#96633,
#96634,#96635,#96636,#96637,#96638,#96639,#96640,#96641,#96642,#96643,#96644,
#96645,#96646,#96647,#96648,#96649,#96650,#96651,#96652,#96653,#96654,#96655,
#96656,#96657,#96658,#96659,#96660,#96661,#96662,#96663,#96664,#96665,#96666,
#96667,#96668,#96669,#96670,#96671,#96672,#96673,#96674,#96675,#96676,#96677,
#96678,#96679,#96680,#96681,#96682,#96683,#96684,#96685,#96686,#96687,#96688,
#96689,#96690,#96691,#96692,#96693,#96694,#96695,#96696,#96697,#96698,#96699,
#96700,#96701,#96702,#96703,#96704,#96705,#96706,#96707,#96708,#96709,#96710,
#96711,#96712,#96713,#96714,#96715,#96716,#96717,#96718,#96719,#96720,#96721,
#96722,#96723,#96724,#96725,#96726,#96727,#96728,#96729,#96730,#96731,#96732,
#96733,#96734,#96735,#96736,#96737,#96738,#96739,#96740,#96741,#96742),
 .UNSPECIFIED.,.F.,.F.,(4,3,3,3,3,3,3,3,3,3,3,3,3,3,3,3,3,3,3,3,3,3,3,3,
3,3,3,3,3,3,3,3,3,3,3,3,3,3,3,3,3,3,3,3,3,4),(-3.27226604903845E-14,0.0160117966439575,
0.0211428683856211,0.031714302578448,0.0407823893134045,0.0422857367712749,
0.0492754087599505,0.0557982959251203,0.0617950682355224,0.0634286051569287,
0.0681480760224011,0.0725110490107089,0.0740000393497556,0.0746607539868073,
0.0766428978979623,0.0778912092473952,0.079285756446169,0.0837839956329802,
0.0845714735425825,0.088007436305928,0.091295323036963,0.0942668433925865,
0.0951429077354094,0.0974554089650903,0.0994724153333818,0.100919062094076,
0.103024026638316,0.104392912654133,0.105053627291185,0.105714341928236,
0.107788014864766,0.110048891466238,0.112101300019925,0.114621057440101,
0.116285776121063,0.118457056421753,0.120715341329924,0.123028442844287,
0.125415872099653,0.12685721031389,0.131314440274099,0.135828076616338,
0.140391856397832,0.145055869455185,0.148000078699544,0.148109584576875),
 .UNSPECIFIED.) ;
#1305=B_SPLINE_CURVE_WITH_KNOTS('',3,(#96743,#96744,#96745,#96746,#96747,
#96748,#96749,#96750,#96751,#96752,#96753,#96754,#96755,#96756),
 .UNSPECIFIED.,.F.,.F.,(4,2,2,2,2,2,4),(-0.0175852662160816,-0.0174945942492549,
-0.0132202758144662,-0.00921513953873651,-0.00502788279858528,-0.00245503564383476,
0.),.UNSPECIFIED.) ;
#1306=B_SPLINE_CURVE_WITH_KNOTS('',3,(#96760,#96761,#96762,#96763,#96764,
#96765,#96766,#96767,#96768,#96769,#96770,#96771,#96772,#96773),
 .UNSPECIFIED.,.F.,.F.,(4,2,2,2,2,2,4),(-0.0199785618144753,-0.0171739150053981,
-0.0142340627298171,-0.00945030384531014,-0.0048741475451923,0.,0.000102743923195659),
 .UNSPECIFIED.) ;
#1307=B_SPLINE_CURVE_WITH_KNOTS('',3,(#96781,#96782,#96783,#96784,#96785,
#96786,#96787,#96788,#96789,#96790,#96791,#96792,#96793,#96794),
 .UNSPECIFIED.,.F.,.F.,(4,2,2,2,2,2,4),(-0.000102391965205721,0.,0.00486346247839452,
0.00942960119761456,0.0141914129216922,0.0171211331600819,0.019918128305216),
 .UNSPECIFIED.) ;
#1308=B_SPLINE_CURVE_WITH_KNOTS('',3,(#96872,#96873,#96874,#96875,#96876,
#96877,#96878,#96879,#96880),.UNSPECIFIED.,.F.,.F.,(4,1,1,1,1,1,4),(0.000114312075647494,
0.062390566311959,0.0935858494679386,0.124781132623918,0.155976415779898,
0.179372878146882,0.218366982091857),.UNSPECIFIED.) ;
#1309=B_SPLINE_CURVE_WITH_KNOTS('',3,(#97020,#97021,#97022,#97023,#97024,
#97025,#97026,#97027,#97028,#97029,#97030,#97031,#97032,#97033),
 .UNSPECIFIED.,.F.,.F.,(4,2,2,2,2,2,4),(-0.0176806146939217,-0.0175891900945432,
-0.0132974964292661,-0.00928060348132365,-0.00506273387556004,-0.00246851070493003,
0.),.UNSPECIFIED.) ;
#1310=B_SPLINE_CURVE_WITH_KNOTS('',3,(#97034,#97035,#97036,#97037,#97038,
#97039,#97040,#97041,#97042,#97043,#97044,#97045,#97046,#97047),
 .UNSPECIFIED.,.F.,.F.,(4,2,2,2,2,2,4),(-0.0175931989203968,-0.0175024032743514,
-0.0132245503122902,-0.00921679814022863,-0.00502740345754487,-0.00245476268172447,
0.),.UNSPECIFIED.) ;
#1311=B_SPLINE_CURVE_WITH_KNOTS('',3,(#97058,#97059,#97060,#97061,#97062,
#97063,#97064,#97065,#97066,#97067,#97068,#97069,#97070,#97071),
 .UNSPECIFIED.,.F.,.F.,(4,2,2,2,2,2,4),(-0.000101340840706905,0.,0.00484233032281562,
0.0094210889116318,0.0145740257047924,0.0180441794667034,0.02136133766618),
 .UNSPECIFIED.) ;
#1312=B_SPLINE_CURVE_WITH_KNOTS('',3,(#97173,#97174,#97175,#97176,#97177,
#97178,#97179,#97180,#97181,#97182,#97183,#97184,#97185,#97186),
 .UNSPECIFIED.,.F.,.F.,(4,2,2,2,2,2,4),(-0.000102734018361801,0.,0.00489034565378813,
0.00951254000304755,0.0146727528261873,0.0181007070879955,0.0213700605851311),
 .UNSPECIFIED.) ;
#1313=B_SPLINE_CURVE_WITH_KNOTS('',3,(#97247,#97248,#97249,#97250,#97251,
#97252,#97253,#97254,#97255,#97256,#97257,#97258,#97259,#97260,#97261,#97262,
#97263,#97264,#97265,#97266,#97267,#97268,#97269,#97270,#97271,#97272,#97273,
#97274,#97275,#97276,#97277,#97278,#97279,#97280,#97281,#97282,#97283,#97284,
#97285,#97286,#97287,#97288,#97289,#97290,#97291,#97292,#97293,#97294,#97295),
 .UNSPECIFIED.,.F.,.F.,(4,3,3,3,3,3,3,3,3,3,3,3,3,3,3,3,4),(0.,0.032673883783352,
0.0500024738644771,0.0672069534204982,0.104457829903168,0.14643552926833,
0.209150107398444,0.250248878590514,0.289222712534637,0.299999453075335,
0.329665056211051,0.350002030405379,0.370262793003315,0.400000667676969,
0.418641417258019,0.450001086263869,0.499999999999957),.UNSPECIFIED.) ;
#1314=B_SPLINE_CURVE_WITH_KNOTS('',3,(#97573,#97574,#97575,#97576,#97577,
#97578,#97579,#97580,#97581,#97582,#97583,#97584,#97585,#97586,#97587,#97588),
 .UNSPECIFIED.,.F.,.F.,(4,3,3,3,3,4),(-0.0789300037689148,-0.0785665817449109,
-0.0585416501678468,-0.0389601328135845,-0.0194590440039062,0.),
 .UNSPECIFIED.) ;
#1315=B_SPLINE_CURVE_WITH_KNOTS('',3,(#97600,#97601,#97602,#97603,#97604,
#97605,#97606,#97607,#97608,#97609,#97610,#97611,#97612,#97613,#97614,#97615),
 .UNSPECIFIED.,.F.,.F.,(4,3,3,3,3,4),(-0.000440517445296823,0.,0.0197956662855006,
0.0393399095404366,0.0588657095784546,0.0783818325119316),.UNSPECIFIED.) ;
#1316=B_SPLINE_CURVE_WITH_KNOTS('',3,(#97720,#97721,#97722,#97723),
 .UNSPECIFIED.,.F.,.F.,(4,4),(-0.0936131112963942,0.),.UNSPECIFIED.) ;
#1317=B_SPLINE_CURVE_WITH_KNOTS('',3,(#97725,#97726,#97727,#97728),
 .UNSPECIFIED.,.F.,.F.,(4,4),(0.,0.0936131112963942),.UNSPECIFIED.) ;
#1318=B_SPLINE_CURVE_WITH_KNOTS('',3,(#97771,#97772,#97773,#97774,#97775,
#97776,#97777,#97778,#97779,#97780,#97781,#97782,#97783,#97784,#97785,#97786),
 .UNSPECIFIED.,.F.,.F.,(4,3,3,3,3,4),(-0.000440517445296842,0.,0.0197956662855012,
0.0393399095404381,0.0588657095784568,0.0783818325119346),.UNSPECIFIED.) ;
#1319=B_SPLINE_CURVE_WITH_KNOTS('',3,(#97810,#97811,#97812,#97813),
 .UNSPECIFIED.,.F.,.F.,(4,4),(-0.0936141814749616,0.),.UNSPECIFIED.) ;
#1320=B_SPLINE_CURVE_WITH_KNOTS('',3,(#97820,#97821,#97822,#97823,#97824,
#97825,#97826,#97827,#97828,#97829,#97830,#97831,#97832,#97833,#97834,#97835),
 .UNSPECIFIED.,.F.,.F.,(4,3,3,3,3,4),(-0.0788196095195842,-0.0783791073898761,
-0.0585841293455798,-0.0390405655905564,-0.019515444411231,0.),
 .UNSPECIFIED.) ;
#1321=B_SPLINE_CURVE_WITH_KNOTS('',3,(#97891,#97892,#97893,#97894),
 .UNSPECIFIED.,.F.,.F.,(4,4),(-0.0936131112963941,0.),.UNSPECIFIED.) ;
#1322=B_SPLINE_CURVE_WITH_KNOTS('',3,(#97926,#97927,#97928,#97929),
 .UNSPECIFIED.,.F.,.F.,(4,4),(-0.0936141811972385,0.),.UNSPECIFIED.) ;
#1323=B_SPLINE_CURVE_WITH_KNOTS('',3,(#97936,#97937,#97938,#97939,#97940,
#97941,#97942,#97943,#97944,#97945,#97946,#97947,#97948,#97949,#97950,#97951),
 .UNSPECIFIED.,.F.,.F.,(4,3,3,3,3,4),(-0.0788196095195841,-0.0783791073898759,
-0.0585841293455797,-0.0390405655905564,-0.019515444411231,0.),
 .UNSPECIFIED.) ;
#1324=B_SPLINE_CURVE_WITH_KNOTS('',3,(#98190,#98191,#98192,#98193,#98194,
#98195),.UNSPECIFIED.,.F.,.F.,(4,2,4),(-0.0699558285734079,-0.0581995466601182,
-0.0505532240038504),.UNSPECIFIED.) ;
#1325=B_SPLINE_CURVE_WITH_KNOTS('',3,(#98212,#98213,#98214,#98215,#98216,
#98217),.UNSPECIFIED.,.F.,.F.,(4,2,4),(-0.0194026045695574,-0.0117562819132905,
0.),.UNSPECIFIED.) ;
#1326=B_SPLINE_CURVE_WITH_KNOTS('',3,(#98320,#98321,#98322,#98323,#98324,
#98325),.UNSPECIFIED.,.F.,.F.,(4,2,4),(-0.0279464003916688,-0.0169330751594897,
0.),.UNSPECIFIED.) ;
#1327=B_SPLINE_CURVE_WITH_KNOTS('',3,(#98446,#98447,#98448,#98449,#98450,
#98451),.UNSPECIFIED.,.F.,.F.,(4,2,4),(-0.0161351759984767,-0.00635867011347371,
0.),.UNSPECIFIED.) ;
#1328=B_SPLINE_CURVE_WITH_KNOTS('',3,(#98481,#98482,#98483,#98484,#98485,
#98486),.UNSPECIFIED.,.F.,.F.,(4,2,4),(-0.0161351760106074,-0.00635867011825523,
0.),.UNSPECIFIED.) ;
#2005=B_SPLINE_SURFACE_WITH_KNOTS('',3,3,((#89000,#89001,#89002,#89003,
#89004,#89005,#89006,#89007,#89008,#89009,#89010,#89011,#89012),(#89013,
#89014,#89015,#89016,#89017,#89018,#89019,#89020,#89021,#89022,#89023,#89024,
#89025),(#89026,#89027,#89028,#89029,#89030,#89031,#89032,#89033,#89034,
#89035,#89036,#89037,#89038),(#89039,#89040,#89041,#89042,#89043,#89044,
#89045,#89046,#89047,#89048,#89049,#89050,#89051),(#89052,#89053,#89054,
#89055,#89056,#89057,#89058,#89059,#89060,#89061,#89062,#89063,#89064),
(#89065,#89066,#89067,#89068,#89069,#89070,#89071,#89072,#89073,#89074,
#89075,#89076,#89077)),.UNSPECIFIED.,.F.,.F.,.F.,(4,1,1,4),(4,1,1,1,1,1,
1,1,1,1,4),(0.,0.333333333333333,0.666666666666667,1.),(0.,0.1,0.2,0.3,
0.4,0.5,0.6,0.7,0.8,0.9,1.),.UNSPECIFIED.) ;
#2006=B_SPLINE_SURFACE_WITH_KNOTS('',3,3,((#89166,#89167,#89168,#89169,
#89170,#89171),(#89172,#89173,#89174,#89175,#89176,#89177),(#89178,#89179,
#89180,#89181,#89182,#89183),(#89184,#89185,#89186,#89187,#89188,#89189),
(#89190,#89191,#89192,#89193,#89194,#89195),(#89196,#89197,#89198,#89199,
#89200,#89201),(#89202,#89203,#89204,#89205,#89206,#89207),(#89208,#89209,
#89210,#89211,#89212,#89213),(#89214,#89215,#89216,#89217,#89218,#89219),
(#89220,#89221,#89222,#89223,#89224,#89225),(#89226,#89227,#89228,#89229,
#89230,#89231),(#89232,#89233,#89234,#89235,#89236,#89237),(#89238,#89239,
#89240,#89241,#89242,#89243)),.UNSPECIFIED.,.F.,.F.,.F.,(4,1,1,1,1,1,1,
1,1,1,4),(4,1,1,4),(0.,0.1,0.2,0.3,0.4,0.5,0.6,0.7,0.8,0.9,1.),(0.,0.333333333333333,
0.666666666666667,1.),.UNSPECIFIED.) ;
#2007=B_SPLINE_SURFACE_WITH_KNOTS('',3,3,((#89327,#89328,#89329,#89330,
#89331,#89332,#89333,#89334,#89335,#89336,#89337,#89338,#89339),(#89340,
#89341,#89342,#89343,#89344,#89345,#89346,#89347,#89348,#89349,#89350,#89351,
#89352),(#89353,#89354,#89355,#89356,#89357,#89358,#89359,#89360,#89361,
#89362,#89363,#89364,#89365),(#89366,#89367,#89368,#89369,#89370,#89371,
#89372,#89373,#89374,#89375,#89376,#89377,#89378),(#89379,#89380,#89381,
#89382,#89383,#89384,#89385,#89386,#89387,#89388,#89389,#89390,#89391),
(#89392,#89393,#89394,#89395,#89396,#89397,#89398,#89399,#89400,#89401,
#89402,#89403,#89404)),.UNSPECIFIED.,.F.,.F.,.F.,(4,1,1,4),(4,1,1,1,1,1,
1,1,1,1,4),(0.,0.333333333333333,0.666666666666667,1.),(0.,0.1,0.2,0.3,
0.4,0.5,0.6,0.7,0.8,0.9,1.),.UNSPECIFIED.) ;
#2008=B_SPLINE_SURFACE_WITH_KNOTS('',3,3,((#89558,#89559,#89560,#89561,
#89562,#89563),(#89564,#89565,#89566,#89567,#89568,#89569),(#89570,#89571,
#89572,#89573,#89574,#89575),(#89576,#89577,#89578,#89579,#89580,#89581),
(#89582,#89583,#89584,#89585,#89586,#89587),(#89588,#89589,#89590,#89591,
#89592,#89593),(#89594,#89595,#89596,#89597,#89598,#89599),(#89600,#89601,
#89602,#89603,#89604,#89605),(#89606,#89607,#89608,#89609,#89610,#89611),
(#89612,#89613,#89614,#89615,#89616,#89617),(#89618,#89619,#89620,#89621,
#89622,#89623)),.UNSPECIFIED.,.F.,.F.,.F.,(4,1,1,1,1,1,1,1,4),(4,1,1,4),
(0.,0.125,0.25,0.375,0.5,0.625,0.75,0.875,1.),(0.,0.333333333333333,0.666666666666667,
1.),.UNSPECIFIED.) ;
#2009=B_SPLINE_SURFACE_WITH_KNOTS('',3,3,((#89738,#89739,#89740,#89741,
#89742,#89743,#89744,#89745,#89746,#89747,#89748),(#89749,#89750,#89751,
#89752,#89753,#89754,#89755,#89756,#89757,#89758,#89759),(#89760,#89761,
#89762,#89763,#89764,#89765,#89766,#89767,#89768,#89769,#89770),(#89771,
#89772,#89773,#89774,#89775,#89776,#89777,#89778,#89779,#89780,#89781),
(#89782,#89783,#89784,#89785,#89786,#89787,#89788,#89789,#89790,#89791,
#89792),(#89793,#89794,#89795,#89796,#89797,#89798,#89799,#89800,#89801,
#89802,#89803)),.UNSPECIFIED.,.F.,.F.,.F.,(4,1,1,4),(4,1,1,1,1,1,1,1,4),
(0.,0.333333333333333,0.666666666666667,1.),(0.,0.125,0.25,0.375,0.5,0.625,
0.75,0.875,1.),.UNSPECIFIED.) ;
#2010=B_SPLINE_SURFACE_WITH_KNOTS('',3,1,((#89883,#89884),(#89885,#89886),
(#89887,#89888),(#89889,#89890),(#89891,#89892)),.UNSPECIFIED.,.F.,.F.,
 .F.,(4,1,4),(2,2),(0.,0.0298071351389365,0.0685496713495228),(0.,0.0359999999999998),
 .UNSPECIFIED.) ;
#2011=B_SPLINE_SURFACE_WITH_KNOTS('',3,1,((#89906,#89907),(#89908,#89909),
(#89910,#89911),(#89912,#89913),(#89914,#89915)),.UNSPECIFIED.,.F.,.F.,
 .F.,(4,1,4),(2,2),(0.,0.0263673128827931,0.0523427870633456),(0.,0.0359999999999998),
 .UNSPECIFIED.) ;
#2012=B_SPLINE_SURFACE_WITH_KNOTS('',3,1,((#89929,#89930),(#89931,#89932),
(#89933,#89934),(#89935,#89936),(#89937,#89938)),.UNSPECIFIED.,.F.,.F.,
 .F.,(4,1,4),(2,2),(0.,0.0190758281807941,0.0379545209982657),(0.,0.0359999999999998),
 .UNSPECIFIED.) ;
#2013=B_SPLINE_SURFACE_WITH_KNOTS('',3,1,((#89952,#89953),(#89954,#89955),
(#89956,#89957),(#89958,#89959),(#89960,#89961)),.UNSPECIFIED.,.F.,.F.,
 .F.,(4,1,4),(2,2),(0.,0.0205128997765721,0.0398218276255599),(0.,0.0359999999999998),
 .UNSPECIFIED.) ;
#2014=B_SPLINE_SURFACE_WITH_KNOTS('',3,1,((#89975,#89976),(#89977,#89978),
(#89979,#89980),(#89981,#89982),(#89983,#89984)),.UNSPECIFIED.,.F.,.F.,
 .F.,(4,1,4),(2,2),(0.,0.0323852950215525,0.0574227556854303),(0.,0.0359999999999998),
 .UNSPECIFIED.) ;
#2015=B_SPLINE_SURFACE_WITH_KNOTS('',3,1,((#90022,#90023),(#90024,#90025),
(#90026,#90027),(#90028,#90029),(#90030,#90031)),.UNSPECIFIED.,.F.,.F.,
 .F.,(4,1,4),(2,2),(0.,0.011955158932918,0.0295605475166918),(0.,0.0359999999999998),
 .UNSPECIFIED.) ;
#2016=B_SPLINE_SURFACE_WITH_KNOTS('',3,1,((#90045,#90046),(#90047,#90048),
(#90049,#90050),(#90051,#90052),(#90053,#90054)),.UNSPECIFIED.,.F.,.F.,
 .F.,(4,1,4),(2,2),(0.,0.0135228484064754,0.0263579081616444),(0.,0.0359999999999998),
 .UNSPECIFIED.) ;
#2017=B_SPLINE_SURFACE_WITH_KNOTS('',3,1,((#90068,#90069),(#90070,#90071),
(#90072,#90073),(#90074,#90075),(#90076,#90077)),.UNSPECIFIED.,.F.,.F.,
 .F.,(4,1,4),(2,2),(0.,0.0216058216755205,0.0381303842659523),(0.,0.0359999999999998),
 .UNSPECIFIED.) ;
#2018=B_SPLINE_SURFACE_WITH_KNOTS('',3,1,((#90091,#90092),(#90093,#90094),
(#90095,#90096),(#90097,#90098),(#90099,#90100)),.UNSPECIFIED.,.F.,.F.,
 .F.,(4,1,4),(2,2),(0.,0.0381782469542568,0.0670753371474822),(0.,0.0359999999999998),
 .UNSPECIFIED.) ;
#2019=B_SPLINE_SURFACE_WITH_KNOTS('',3,1,((#90132,#90133),(#90134,#90135),
(#90136,#90137),(#90138,#90139),(#90140,#90141)),.UNSPECIFIED.,.F.,.F.,
 .F.,(4,1,4),(2,2),(0.,0.0329095469988702,0.0691336974954879),(0.,0.0359999999999998),
 .UNSPECIFIED.) ;
#2020=B_SPLINE_SURFACE_WITH_KNOTS('',3,1,((#90155,#90156),(#90157,#90158),
(#90159,#90160),(#90161,#90162),(#90163,#90164)),.UNSPECIFIED.,.F.,.F.,
 .F.,(4,1,4),(2,2),(0.,0.0210301296927785,0.0377156586265697),(0.,0.0359999999999998),
 .UNSPECIFIED.) ;
#2021=B_SPLINE_SURFACE_WITH_KNOTS('',3,1,((#90178,#90179),(#90180,#90181),
(#90182,#90183),(#90184,#90185),(#90186,#90187)),.UNSPECIFIED.,.F.,.F.,
 .F.,(4,1,4),(2,2),(0.,0.0424180496051088,0.0942055476140892),(0.,0.0359999999999998),
 .UNSPECIFIED.) ;
#2022=B_SPLINE_SURFACE_WITH_KNOTS('',3,1,((#90201,#90202),(#90203,#90204),
(#90205,#90206),(#90207,#90208),(#90209,#90210)),.UNSPECIFIED.,.F.,.F.,
 .F.,(4,1,4),(2,2),(0.,0.0398228695438388,0.0783699334705556),(0.,0.0359999999999998),
 .UNSPECIFIED.) ;
#2023=B_SPLINE_SURFACE_WITH_KNOTS('',3,1,((#90224,#90225),(#90226,#90227),
(#90228,#90229),(#90230,#90231),(#90232,#90233)),.UNSPECIFIED.,.F.,.F.,
 .F.,(4,1,4),(2,2),(0.,0.0313133324080373,0.063168759987351),(0.,0.0359999999999998),
 .UNSPECIFIED.) ;
#2024=B_SPLINE_SURFACE_WITH_KNOTS('',3,1,((#90247,#90248),(#90249,#90250),
(#90251,#90252),(#90253,#90254),(#90255,#90256)),.UNSPECIFIED.,.F.,.F.,
 .F.,(4,1,4),(2,2),(0.,0.0290828541577381,0.0592932101613289),(0.,0.0359999999999998),
 .UNSPECIFIED.) ;
#2025=B_SPLINE_SURFACE_WITH_KNOTS('',3,1,((#90270,#90271),(#90272,#90273),
(#90274,#90275),(#90276,#90277),(#90278,#90279)),.UNSPECIFIED.,.F.,.F.,
 .F.,(4,1,4),(2,2),(0.,0.0471458586470647,0.0823534588635132),(0.,0.0359999999999998),
 .UNSPECIFIED.) ;
#2026=B_SPLINE_SURFACE_WITH_KNOTS('',3,1,((#90354,#90355),(#90356,#90357),
(#90358,#90359),(#90360,#90361)),.UNSPECIFIED.,.F.,.F.,.F.,(4,4),(2,2),
(0.,1.),(0.,0.456),.UNSPECIFIED.) ;
#2027=B_SPLINE_SURFACE_WITH_KNOTS('',3,1,((#90370,#90371),(#90372,#90373),
(#90374,#90375),(#90376,#90377),(#90378,#90379),(#90380,#90381)),
 .UNSPECIFIED.,.F.,.F.,.F.,(4,2,4),(2,2),(-0.0699558285734109,-0.0581995466601206,
-0.0505532240038533),(0.,1.14),.UNSPECIFIED.) ;
#2028=B_SPLINE_SURFACE_WITH_KNOTS('',3,3,((#90444,#90445,#90446,#90447),
(#90448,#90449,#90450,#90451),(#90452,#90453,#90454,#90455),(#90456,#90457,
#90458,#90459),(#90460,#90461,#90462,#90463)),.UNSPECIFIED.,.F.,.F.,.F.,
(4,1,4),(4,4),(0.,0.5,1.),(-0.156907118032788,-0.139899380964935),
 .UNSPECIFIED.) ;
#2029=B_SPLINE_SURFACE_WITH_KNOTS('',3,3,((#90525,#90526,#90527,#90528,
#90529),(#90530,#90531,#90532,#90533,#90534),(#90535,#90536,#90537,#90538,
#90539),(#90540,#90541,#90542,#90543,#90544),(#90545,#90546,#90547,#90548,
#90549)),.UNSPECIFIED.,.F.,.F.,.F.,(4,1,4),(4,1,4),(0.,0.5,1.00016791794751),
(4.71222106243701,5.16843353557162,5.77649294248775),.UNSPECIFIED.) ;
#2030=B_SPLINE_SURFACE_WITH_KNOTS('',3,3,((#90642,#90643,#90644,#90645,
#90646,#90647,#90648,#90649,#90650,#90651,#90652),(#90653,#90654,#90655,
#90656,#90657,#90658,#90659,#90660,#90661,#90662,#90663),(#90664,#90665,
#90666,#90667,#90668,#90669,#90670,#90671,#90672,#90673,#90674),(#90675,
#90676,#90677,#90678,#90679,#90680,#90681,#90682,#90683,#90684,#90685),
(#90686,#90687,#90688,#90689,#90690,#90691,#90692,#90693,#90694,#90695,
#90696),(#90697,#90698,#90699,#90700,#90701,#90702,#90703,#90704,#90705,
#90706,#90707)),.UNSPECIFIED.,.F.,.F.,.F.,(4,1,1,4),(4,1,1,1,1,1,1,1,4),
(0.,0.285714285714286,0.571428571428571,1.55420651718688),(0.000383464105853098,
0.0268242176912658,0.0532649712766785,0.073095536465738,0.0797057248620911,
0.0863159132584443,0.0896210074566209,0.0912735545557092,0.0929261016547975),
 .UNSPECIFIED.) ;
#2031=B_SPLINE_SURFACE_WITH_KNOTS('',3,3,((#90799,#90800,#90801,#90802,
#90803),(#90804,#90805,#90806,#90807,#90808),(#90809,#90810,#90811,#90812,
#90813),(#90814,#90815,#90816,#90817,#90818),(#90819,#90820,#90821,#90822,
#90823)),.UNSPECIFIED.,.F.,.F.,.F.,(4,1,4),(4,1,4),(-0.000290474503729989,
0.5,1.00029047450393),(-0.000290474503928144,0.897597901025654,1.5707963267949),
 .UNSPECIFIED.) ;
#2032=B_SPLINE_SURFACE_WITH_KNOTS('',3,3,((#90840,#90841,#90842,#90843),
(#90844,#90845,#90846,#90847),(#90848,#90849,#90850,#90851),(#90852,#90853,
#90854,#90855),(#90856,#90857,#90858,#90859)),.UNSPECIFIED.,.F.,.F.,.F.,
(4,1,4),(4,4),(-0.000506016721647412,0.5,1.),(-5.54544584248221,-4.71188296366304),
 .UNSPECIFIED.) ;
#2033=B_SPLINE_SURFACE_WITH_KNOTS('',3,3,((#90865,#90866,#90867,#90868,
#90869,#90870),(#90871,#90872,#90873,#90874,#90875,#90876),(#90877,#90878,
#90879,#90880,#90881,#90882),(#90883,#90884,#90885,#90886,#90887,#90888)),
 .UNSPECIFIED.,.F.,.F.,.F.,(4,4),(4,2,4),(0.,1.),(0.,0.0518624644373431,
0.0522283064773341),.UNSPECIFIED.) ;
#2034=B_SPLINE_SURFACE_WITH_KNOTS('',3,3,((#90918,#90919,#90920,#90921,
#90922),(#90923,#90924,#90925,#90926,#90927),(#90928,#90929,#90930,#90931,
#90932),(#90933,#90934,#90935,#90936,#90937),(#90938,#90939,#90940,#90941,
#90942)),.UNSPECIFIED.,.F.,.F.,.F.,(4,1,4),(4,1,4),(-0.000419225650178164,
0.5,1.00041922565031),(-1.5707963267949,-0.67319842576924,0.0004192256503168),
 .UNSPECIFIED.) ;
#2035=B_SPLINE_SURFACE_WITH_KNOTS('',3,3,((#90959,#90960,#90961,#90962),
(#90963,#90964,#90965,#90966),(#90967,#90968,#90969,#90970),(#90971,#90972,
#90973,#90974),(#90975,#90976,#90977,#90978)),.UNSPECIFIED.,.F.,.F.,.F.,
(4,1,4),(4,4),(-0.000506016735097035,0.5,1.),(-1.57130234353,-0.737739464683826),
 .UNSPECIFIED.) ;
#2036=B_SPLINE_SURFACE_WITH_KNOTS('',3,3,((#90984,#90985,#90986,#90987,
#90988,#90989),(#90990,#90991,#90992,#90993,#90994,#90995),(#90996,#90997,
#90998,#90999,#91000,#91001),(#91002,#91003,#91004,#91005,#91006,#91007)),
 .UNSPECIFIED.,.F.,.F.,.F.,(4,4),(4,2,4),(0.,1.),(-0.000365842040355155,
0.,0.051862464436985),.UNSPECIFIED.) ;
#2037=B_SPLINE_SURFACE_WITH_KNOTS('',3,3,((#91063,#91064,#91065,#91066),
(#91067,#91068,#91069,#91070),(#91071,#91072,#91073,#91074),(#91075,#91076,
#91077,#91078),(#91079,#91080,#91081,#91082)),.UNSPECIFIED.,.F.,.F.,.F.,
(4,1,4),(4,4),(-0.0189222038896959,0.571428571428571,1.01886279511128),
(-0.0189222038896219,1.5707963267949),.UNSPECIFIED.) ;
#2038=B_SPLINE_SURFACE_WITH_KNOTS('',3,3,((#91155,#91156,#91157,#91158,
#91159),(#91160,#91161,#91162,#91163,#91164),(#91165,#91166,#91167,#91168,
#91169),(#91170,#91171,#91172,#91173,#91174),(#91175,#91176,#91177,#91178,
#91179)),.UNSPECIFIED.,.F.,.F.,.F.,(4,1,4),(4,1,4),(0.,0.5,1.00066906930274),
(-0.000669069302958659,0.785398163397612,1.57146539609819),
 .UNSPECIFIED.) ;
#2039=B_SPLINE_SURFACE_WITH_KNOTS('',3,3,((#91445,#91446,#91447,#91448,
#91449,#91450),(#91451,#91452,#91453,#91454,#91455,#91456),(#91457,#91458,
#91459,#91460,#91461,#91462),(#91463,#91464,#91465,#91466,#91467,#91468),
(#91469,#91470,#91471,#91472,#91473,#91474),(#91475,#91476,#91477,#91478,
#91479,#91480),(#91481,#91482,#91483,#91484,#91485,#91486)),
 .UNSPECIFIED.,.F.,.F.,.F.,(4,1,1,1,4),(4,1,1,4),(0.,0.285714285714286,
0.5,0.785714285714286,1.),(0.148883906684682,0.156528869066089,0.166722152241299,
0.184560397797916),.UNSPECIFIED.) ;
#2040=B_SPLINE_SURFACE_WITH_KNOTS('',3,3,((#91524,#91525,#91526,#91527,
#91528,#91529),(#91530,#91531,#91532,#91533,#91534,#91535),(#91536,#91537,
#91538,#91539,#91540,#91541),(#91542,#91543,#91544,#91545,#91546,#91547),
(#91548,#91549,#91550,#91551,#91552,#91553)),.UNSPECIFIED.,.F.,.F.,.F.,
(4,1,4),(4,2,4),(0.,0.571428571428571,1.),(-0.0663145530984604,0.,0.000424263177439857),
 .UNSPECIFIED.) ;
#2041=B_SPLINE_SURFACE_WITH_KNOTS('',3,3,((#91596,#91597,#91598,#91599),
(#91600,#91601,#91602,#91603),(#91604,#91605,#91606,#91607),(#91608,#91609,
#91610,#91611),(#91612,#91613,#91614,#91615)),.UNSPECIFIED.,.F.,.F.,.F.,
(4,1,4),(4,4),(0.,0.571428571428571,1.),(0.,0.0254449718282482),
 .UNSPECIFIED.) ;
#2042=B_SPLINE_SURFACE_WITH_KNOTS('',3,3,((#91627,#91628,#91629,#91630),
(#91631,#91632,#91633,#91634),(#91635,#91636,#91637,#91638),(#91639,#91640,
#91641,#91642),(#91643,#91644,#91645,#91646)),.UNSPECIFIED.,.F.,.F.,.F.,
(4,1,4),(4,4),(-0.00104348049004246,0.571428571428571,1.),(0.861856499795871,
1.57183980728496),.UNSPECIFIED.) ;
#2043=B_SPLINE_SURFACE_WITH_KNOTS('',3,3,((#91658,#91659,#91660,#91661,
#91662),(#91663,#91664,#91665,#91666,#91667),(#91668,#91669,#91670,#91671,
#91672),(#91673,#91674,#91675,#91676,#91677),(#91678,#91679,#91680,#91681,
#91682)),.UNSPECIFIED.,.F.,.F.,.F.,(4,1,4),(4,1,4),(-0.000590521380405756,
0.571428571428571,1.),(-1.57138684817531,-1.12581647705762,-0.531919489361454),
 .UNSPECIFIED.) ;
#2044=B_SPLINE_SURFACE_WITH_KNOTS('',3,3,((#91765,#91766,#91767,#91768,
#91769,#91770),(#91771,#91772,#91773,#91774,#91775,#91776),(#91777,#91778,
#91779,#91780,#91781,#91782),(#91783,#91784,#91785,#91786,#91787,#91788)),
 .UNSPECIFIED.,.F.,.F.,.F.,(4,4),(4,2,4),(-0.000170891015070361,1.),(-0.0300731157523127,
-0.0299720828361244,0.000170254829587993),.UNSPECIFIED.) ;
#2045=B_SPLINE_SURFACE_WITH_KNOTS('',3,3,((#91831,#91832,#91833,#91834),
(#91835,#91836,#91837,#91838),(#91839,#91840,#91841,#91842),(#91843,#91844,
#91845,#91846),(#91847,#91848,#91849,#91850)),.UNSPECIFIED.,.F.,.F.,.F.,
(4,1,4),(4,4),(0.,0.571428571428571,1.),(1.13982531580781,1.57079632679494),
 .UNSPECIFIED.) ;
#2046=B_SPLINE_SURFACE_WITH_KNOTS('',3,3,((#91862,#91863,#91864,#91865),
(#91866,#91867,#91868,#91869),(#91870,#91871,#91872,#91873),(#91874,#91875,
#91876,#91877),(#91878,#91879,#91880,#91881)),.UNSPECIFIED.,.F.,.F.,.F.,
(4,1,4),(4,4),(0.,0.571428571428571,1.0003523080326),(-1.57114863482751,
-0.92694290996995),.UNSPECIFIED.) ;
#2047=B_SPLINE_SURFACE_WITH_KNOTS('',3,3,((#91887,#91888,#91889,#91890),
(#91891,#91892,#91893,#91894),(#91895,#91896,#91897,#91898),(#91899,#91900,
#91901,#91902),(#91903,#91904,#91905,#91906)),.UNSPECIFIED.,.F.,.F.,.F.,
(4,1,4),(4,4),(0.,0.571428571428571,1.),(4.14247343901052E-16,0.0173725716234068),
 .UNSPECIFIED.) ;
#2048=B_SPLINE_SURFACE_WITH_KNOTS('',3,3,((#91912,#91913,#91914,#91915),
(#91916,#91917,#91918,#91919),(#91920,#91921,#91922,#91923),(#91924,#91925,
#91926,#91927)),.UNSPECIFIED.,.F.,.F.,.F.,(4,4),(4,4),(0.,1.00246533549981),
(-0.64596644429237,0.00246533549982144),.UNSPECIFIED.) ;
#2049=B_SPLINE_SURFACE_WITH_KNOTS('',3,3,((#92031,#92032,#92033,#92034),
(#92035,#92036,#92037,#92038),(#92039,#92040,#92041,#92042),(#92043,#92044,
#92045,#92046),(#92047,#92048,#92049,#92050)),.UNSPECIFIED.,.F.,.F.,.F.,
(4,1,4),(4,4),(0.,0.571428571428571,1.),(-1.57079632679486,1.0162123752053E-13),
 .UNSPECIFIED.) ;
#2050=B_SPLINE_SURFACE_WITH_KNOTS('',3,3,((#92500,#92501,#92502,#92503,
#92504,#92505,#92506,#92507),(#92508,#92509,#92510,#92511,#92512,#92513,
#92514,#92515),(#92516,#92517,#92518,#92519,#92520,#92521,#92522,#92523),
(#92524,#92525,#92526,#92527,#92528,#92529,#92530,#92531),(#92532,#92533,
#92534,#92535,#92536,#92537,#92538,#92539),(#92540,#92541,#92542,#92543,
#92544,#92545,#92546,#92547),(#92548,#92549,#92550,#92551,#92552,#92553,
#92554,#92555)),.UNSPECIFIED.,.F.,.F.,.F.,(4,1,1,1,4),(4,1,1,1,1,4),(0.,
0.285714285714286,0.5,0.785714285714286,1.),(9.19824141439016E-31,0.00572297095011093,
0.0114459419002219,0.0171689128503328,0.0286148547505547,0.0400607966507765),
 .UNSPECIFIED.) ;
#2051=B_SPLINE_SURFACE_WITH_KNOTS('',3,3,((#92697,#92698,#92699,#92700,
#92701,#92702,#92703),(#92704,#92705,#92706,#92707,#92708,#92709,#92710),
(#92711,#92712,#92713,#92714,#92715,#92716,#92717),(#92718,#92719,#92720,
#92721,#92722,#92723,#92724),(#92725,#92726,#92727,#92728,#92729,#92730,
#92731),(#92732,#92733,#92734,#92735,#92736,#92737,#92738),(#92739,#92740,
#92741,#92742,#92743,#92744,#92745)),.UNSPECIFIED.,.F.,.F.,.F.,(4,1,1,1,
4),(4,1,1,1,4),(0.,0.285714285714286,0.5,0.785714285714286,1.),(-8.67361737988406E-17,
0.224399475256413,0.448798950512826,0.897597901025653,1.57079632679489),
 .UNSPECIFIED.) ;
#2052=B_SPLINE_SURFACE_WITH_KNOTS('',3,3,((#92902,#92903,#92904,#92905,
#92906,#92907),(#92908,#92909,#92910,#92911,#92912,#92913),(#92914,#92915,
#92916,#92917,#92918,#92919),(#92920,#92921,#92922,#92923,#92924,#92925),
(#92926,#92927,#92928,#92929,#92930,#92931)),.UNSPECIFIED.,.F.,.F.,.F.,
(4,1,4),(4,1,1,4),(0.,0.571428571428571,1.),(8.270742692011E-19,0.0162039536314463,
0.0231485051877804,0.0324079072628925),.UNSPECIFIED.) ;
#2053=B_SPLINE_SURFACE_WITH_KNOTS('',3,3,((#93002,#93003,#93004,#93005,
#93006,#93007),(#93008,#93009,#93010,#93011,#93012,#93013),(#93014,#93015,
#93016,#93017,#93018,#93019),(#93020,#93021,#93022,#93023,#93024,#93025),
(#93026,#93027,#93028,#93029,#93030,#93031)),.UNSPECIFIED.,.F.,.F.,.F.,
(4,1,4),(4,1,1,4),(0.,0.571428571428571,1.),(0.,0.00925932038092611,0.0162038106666207,
0.0324076213332414),.UNSPECIFIED.) ;
#2054=B_SPLINE_SURFACE_WITH_KNOTS('',3,3,((#93084,#93085,#93086,#93087,
#93088),(#93089,#93090,#93091,#93092,#93093),(#93094,#93095,#93096,#93097,
#93098),(#93099,#93100,#93101,#93102,#93103),(#93104,#93105,#93106,#93107,
#93108)),.UNSPECIFIED.,.F.,.F.,.F.,(4,1,4),(4,1,4),(0.,0.571428571428571,
1.),(0.,0.0126399602240726,0.0294932405228361),.UNSPECIFIED.) ;
#2055=B_SPLINE_SURFACE_WITH_KNOTS('',3,3,((#93121,#93122,#93123,#93124),
(#93125,#93126,#93127,#93128),(#93129,#93130,#93131,#93132),(#93133,#93134,
#93135,#93136),(#93137,#93138,#93139,#93140)),.UNSPECIFIED.,.F.,.F.,.F.,
(4,1,4),(4,4),(-0.00114393799377549,0.571428571428571,1.),(0.914253278585075,
1.57194026478868),.UNSPECIFIED.) ;
#2056=B_SPLINE_SURFACE_WITH_KNOTS('',3,3,((#93229,#93230,#93231,#93232,
#93233),(#93234,#93235,#93236,#93237,#93238),(#93239,#93240,#93241,#93242,
#93243),(#93244,#93245,#93246,#93247,#93248),(#93249,#93250,#93251,#93252,
#93253)),.UNSPECIFIED.,.F.,.F.,.F.,(4,1,4),(4,1,4),(0.,0.571428571428571,
1.),(0.,0.0168532803128275,0.0294932405474481),.UNSPECIFIED.) ;
#2057=B_SPLINE_SURFACE_WITH_KNOTS('',3,3,((#93266,#93267,#93268,#93269),
(#93270,#93271,#93272,#93273),(#93274,#93275,#93276,#93277),(#93278,#93279,
#93280,#93281),(#93282,#93283,#93284,#93285)),.UNSPECIFIED.,.F.,.F.,.F.,
(4,1,4),(4,4),(-0.00114393799175905,0.571428571428571,1.),(-1.57194026478668,
-0.914253278587085),.UNSPECIFIED.) ;
#2058=B_SPLINE_SURFACE_WITH_KNOTS('',3,3,((#93481,#93482,#93483,#93484,
#93485),(#93486,#93487,#93488,#93489,#93490),(#93491,#93492,#93493,#93494,
#93495),(#93496,#93497,#93498,#93499,#93500),(#93501,#93502,#93503,#93504,
#93505),(#93506,#93507,#93508,#93509,#93510),(#93511,#93512,#93513,#93514,
#93515)),.UNSPECIFIED.,.F.,.F.,.F.,(4,1,1,1,4),(4,1,4),(-0.000276284474482355,
0.285714285714286,0.5,0.785714285714286,1.00025438918361),(0.67448655303988,
1.05876467846844,1.57107261127047),.UNSPECIFIED.) ;
#2059=B_SPLINE_SURFACE_WITH_KNOTS('',3,3,((#93561,#93562,#93563,#93564),
(#93565,#93566,#93567,#93568),(#93569,#93570,#93571,#93572),(#93573,#93574,
#93575,#93576),(#93577,#93578,#93579,#93580),(#93581,#93582,#93583,#93584)),
 .UNSPECIFIED.,.F.,.F.,.F.,(4,1,1,4),(4,4),(-0.000163798824285399,0.285714285714286,
0.571428571428571,1.00148567620286),(-1.57228200299773,-0.871178949794101),
 .UNSPECIFIED.) ;
#2060=B_SPLINE_SURFACE_WITH_KNOTS('',3,3,((#93592,#93593,#93594,#93595),
(#93596,#93597,#93598,#93599),(#93600,#93601,#93602,#93603),(#93604,#93605,
#93606,#93607),(#93608,#93609,#93610,#93611),(#93612,#93613,#93614,#93615),
(#93616,#93617,#93618,#93619)),.UNSPECIFIED.,.F.,.F.,.F.,(4,1,1,1,4),(4,
4),(-0.000162614260257949,0.285714285714286,0.5,0.714285714285714,1.0005808683447),
(-0.873245494341663,-0.0772155251815629),.UNSPECIFIED.) ;
#2061=B_SPLINE_SURFACE_WITH_KNOTS('',3,3,((#93623,#93624,#93625,#93626),
(#93627,#93628,#93629,#93630),(#93631,#93632,#93633,#93634),(#93635,#93636,
#93637,#93638),(#93639,#93640,#93641,#93642),(#93643,#93644,#93645,#93646),
(#93647,#93648,#93649,#93650)),.UNSPECIFIED.,.F.,.F.,.F.,(4,1,1,1,4),(4,
4),(0.,0.285714285714286,0.5,0.714285714285714,1.),(0.0777963935263006,
0.648820263581669),.UNSPECIFIED.) ;
#2062=B_SPLINE_SURFACE_WITH_KNOTS('',3,3,((#93654,#93655,#93656,#93657),
(#93658,#93659,#93660,#93661),(#93662,#93663,#93664,#93665),(#93666,#93667,
#93668,#93669),(#93670,#93671,#93672,#93673),(#93674,#93675,#93676,#93677)),
 .UNSPECIFIED.,.F.,.F.,.F.,(4,1,1,4),(4,4),(0.,0.285714285714286,0.571428571428571,
1.),(2.15310365171961E-15,0.0294983491188769),.UNSPECIFIED.) ;
#2063=B_SPLINE_SURFACE_WITH_KNOTS('',3,3,((#93937,#93938,#93939,#93940,
#93941,#93942),(#93943,#93944,#93945,#93946,#93947,#93948),(#93949,#93950,
#93951,#93952,#93953,#93954),(#93955,#93956,#93957,#93958,#93959,#93960),
(#93961,#93962,#93963,#93964,#93965,#93966)),.UNSPECIFIED.,.F.,.F.,.F.,
(4,1,4),(4,1,1,4),(-0.00069658220300701,0.571428571428571,1.),(-0.00069658220300276,
0.673198425769244,1.12199737628207,1.57149290899785),.UNSPECIFIED.) ;
#2064=B_SPLINE_SURFACE_WITH_KNOTS('',3,3,((#93975,#93976,#93977,#93978,
#93979,#93980),(#93981,#93982,#93983,#93984,#93985,#93986),(#93987,#93988,
#93989,#93990,#93991,#93992),(#93993,#93994,#93995,#93996,#93997,#93998),
(#93999,#94000,#94001,#94002,#94003,#94004)),.UNSPECIFIED.,.F.,.F.,.F.,
(4,1,4),(4,1,1,4),(-0.00069647979888005,0.571428571428571,1.),(-1.57149280659377,
-1.12199737628207,-0.673198425769238,0.000696479798882929),
 .UNSPECIFIED.) ;
#2065=B_SPLINE_SURFACE_WITH_KNOTS('',3,3,((#94019,#94020,#94021,#94022,
#94023),(#94024,#94025,#94026,#94027,#94028),(#94029,#94030,#94031,#94032,
#94033),(#94034,#94035,#94036,#94037,#94038),(#94039,#94040,#94041,#94042,
#94043)),.UNSPECIFIED.,.F.,.F.,.F.,(4,1,4),(4,1,4),(-0.00194122259541691,
0.571428571428571,1.),(-0.00194122259541691,0.0195634159024299,0.0475891930344199),
 .UNSPECIFIED.) ;
#2066=B_SPLINE_SURFACE_WITH_KNOTS('',3,3,((#94109,#94110,#94111,#94112),
(#94113,#94114,#94115,#94116),(#94117,#94118,#94119,#94120),(#94121,#94122,
#94123,#94124),(#94125,#94126,#94127,#94128)),.UNSPECIFIED.,.F.,.F.,.F.,
(4,1,4),(4,4),(-0.00567875718055857,0.571428571428571,1.),(0.562190624368961,
1.57647508397548),.UNSPECIFIED.) ;
#2067=B_SPLINE_SURFACE_WITH_KNOTS('',3,3,((#94132,#94133,#94134,#94135),
(#94136,#94137,#94138,#94139),(#94140,#94141,#94142,#94143),(#94144,#94145,
#94146,#94147),(#94148,#94149,#94150,#94151)),.UNSPECIFIED.,.F.,.F.,.F.,
(4,1,4),(4,4),(0.,0.571428571428571,1.),(1.33431567541952E-15,0.0171168860941288),
 .UNSPECIFIED.) ;
#2068=B_SPLINE_SURFACE_WITH_KNOTS('',3,3,((#94222,#94223,#94224,#94225),
(#94226,#94227,#94228,#94229),(#94230,#94231,#94232,#94233),(#94234,#94235,
#94236,#94237),(#94238,#94239,#94240,#94241)),.UNSPECIFIED.,.F.,.F.,.F.,
(4,1,4),(4,4),(0.,0.5,1.),(0.0461307304951755,0.109806780005479),
 .UNSPECIFIED.) ;
#2069=B_SPLINE_SURFACE_WITH_KNOTS('',3,3,((#94251,#94252,#94253,#94254),
(#94255,#94256,#94257,#94258),(#94259,#94260,#94261,#94262),(#94263,#94264,
#94265,#94266),(#94267,#94268,#94269,#94270),(#94271,#94272,#94273,#94274),
(#94275,#94276,#94277,#94278)),.UNSPECIFIED.,.F.,.F.,.F.,(4,1,1,1,4),(4,
4),(0.,0.285714285714286,0.5,0.785714285714286,1.),(-2.1768822796151,-1.66773041364303),
 .UNSPECIFIED.) ;
#2070=B_SPLINE_SURFACE_WITH_KNOTS('',3,3,((#94280,#94281,#94282,#94283,
#94284),(#94285,#94286,#94287,#94288,#94289),(#94290,#94291,#94292,#94293,
#94294),(#94295,#94296,#94297,#94298,#94299),(#94300,#94301,#94302,#94303,
#94304),(#94305,#94306,#94307,#94308,#94309),(#94310,#94311,#94312,#94313,
#94314)),.UNSPECIFIED.,.F.,.F.,.F.,(4,1,1,1,4),(4,1,4),(-0.000518096114479414,
0.285714285714286,0.5,0.785714285714286,1.),(-0.00050344375524984,0.0114772233155261,
0.0272982838507071),.UNSPECIFIED.) ;
#2071=B_SPLINE_SURFACE_WITH_KNOTS('',3,3,((#94345,#94346,#94347,#94348),
(#94349,#94350,#94351,#94352),(#94353,#94354,#94355,#94356),(#94357,#94358,
#94359,#94360),(#94361,#94362,#94363,#94364),(#94365,#94366,#94367,#94368),
(#94369,#94370,#94371,#94372)),.UNSPECIFIED.,.F.,.F.,.F.,(4,1,1,1,4),(4,
4),(0.,0.285714285714286,0.5,0.785714285714286,1.),(-1.27744058344438,-1.20367640622073),
 .UNSPECIFIED.) ;
#2072=B_SPLINE_SURFACE_WITH_KNOTS('',3,3,((#94376,#94377,#94378,#94379,
#94380),(#94381,#94382,#94383,#94384,#94385),(#94386,#94387,#94388,#94389,
#94390),(#94391,#94392,#94393,#94394,#94395),(#94396,#94397,#94398,#94399,
#94400),(#94401,#94402,#94403,#94404,#94405),(#94406,#94407,#94408,#94409,
#94410)),.UNSPECIFIED.,.F.,.F.,.F.,(4,1,1,1,4),(4,1,4),(0.,0.285714285714286,
0.5,0.785714285714286,1.),(0.0334571978979197,0.0595744748887569,0.0856917518795941),
 .UNSPECIFIED.) ;
#2073=B_SPLINE_SURFACE_WITH_KNOTS('',3,3,((#94449,#94450,#94451,#94452),
(#94453,#94454,#94455,#94456),(#94457,#94458,#94459,#94460),(#94461,#94462,
#94463,#94464),(#94465,#94466,#94467,#94468),(#94469,#94470,#94471,#94472),
(#94473,#94474,#94475,#94476)),.UNSPECIFIED.,.F.,.F.,.F.,(4,1,1,1,4),(4,
4),(0.,0.285714285714286,0.5,0.785714285714286,1.),(-1.56238538892354,-0.785398163397404),
 .UNSPECIFIED.) ;
#2074=B_SPLINE_SURFACE_WITH_KNOTS('',3,3,((#94487,#94488,#94489,#94490),
(#94491,#94492,#94493,#94494),(#94495,#94496,#94497,#94498),(#94499,#94500,
#94501,#94502),(#94503,#94504,#94505,#94506),(#94507,#94508,#94509,#94510),
(#94511,#94512,#94513,#94514)),.UNSPECIFIED.,.F.,.F.,.F.,(4,1,1,1,4),(4,
4),(-0.000154725634345458,0.285714285714286,0.5,0.785714285714286,1.00006609114655),
(-1.2305075083907,-0.785243437762843),.UNSPECIFIED.) ;
#2075=B_SPLINE_SURFACE_WITH_KNOTS('',3,3,((#94519,#94520,#94521,#94522),
(#94523,#94524,#94525,#94526),(#94527,#94528,#94529,#94530),(#94531,#94532,
#94533,#94534),(#94535,#94536,#94537,#94538)),.UNSPECIFIED.,.F.,.F.,.F.,
(4,1,4),(4,4),(0.,0.5,1.),(1.2303527827561,1.54388796055314),
 .UNSPECIFIED.) ;
#2076=B_SPLINE_SURFACE_WITH_KNOTS('',3,3,((#94635,#94636,#94637,#94638),
(#94639,#94640,#94641,#94642),(#94643,#94644,#94645,#94646),(#94647,#94648,
#94649,#94650)),.UNSPECIFIED.,.F.,.F.,.F.,(4,4),(4,4),(0.,1.),(-0.263885209381218,
-1.85090356762827E-14),.UNSPECIFIED.) ;
#2077=B_SPLINE_SURFACE_WITH_KNOTS('',3,3,((#94651,#94652,#94653,#94654),
(#94655,#94656,#94657,#94658),(#94659,#94660,#94661,#94662),(#94663,#94664,
#94665,#94666)),.UNSPECIFIED.,.F.,.F.,.F.,(4,4),(4,4),(0.,1.00201261903925),
(-0.00201261903924553,0.787410782436316),.UNSPECIFIED.) ;
#2078=B_SPLINE_SURFACE_WITH_KNOTS('',3,3,((#94688,#94689,#94690,#94691,
#94692,#94693,#94694,#94695,#94696),(#94697,#94698,#94699,#94700,#94701,
#94702,#94703,#94704,#94705),(#94706,#94707,#94708,#94709,#94710,#94711,
#94712,#94713,#94714),(#94715,#94716,#94717,#94718,#94719,#94720,#94721,
#94722,#94723),(#94724,#94725,#94726,#94727,#94728,#94729,#94730,#94731,
#94732)),.UNSPECIFIED.,.F.,.F.,.F.,(4,1,4),(4,1,1,1,1,1,4),(0.,0.5,1.),
(-0.0334031852475255,-0.0321676440171422,-0.0309321027867588,-0.0284610203259921,
-0.0161056080221584,-0.00869236063985824,0.00119196920320868),
 .UNSPECIFIED.) ;
#2079=B_SPLINE_SURFACE_WITH_KNOTS('',3,3,((#94736,#94737,#94738,#94739,
#94740,#94741,#94742,#94743,#94744,#94745),(#94746,#94747,#94748,#94749,
#94750,#94751,#94752,#94753,#94754,#94755),(#94756,#94757,#94758,#94759,
#94760,#94761,#94762,#94763,#94764,#94765),(#94766,#94767,#94768,#94769,
#94770,#94771,#94772,#94773,#94774,#94775)),.UNSPECIFIED.,.F.,.F.,.F.,(4,
4),(4,1,1,1,1,1,1,4),(0.,1.00026349704058),(0.047946162077175,0.048285659180944,
0.048625156284713,0.0493041504922509,0.0506621389073269,0.0513411331148649,
0.0520201273224029,0.0577155780232905),.UNSPECIFIED.) ;
#2080=B_SPLINE_SURFACE_WITH_KNOTS('',5,1,((#94850,#94851),(#94852,#94853),
(#94854,#94855),(#94856,#94857),(#94858,#94859),(#94860,#94861),(#94862,
#94863),(#94864,#94865),(#94866,#94867),(#94868,#94869),(#94870,#94871),
(#94872,#94873),(#94874,#94875),(#94876,#94877),(#94878,#94879)),
 .UNSPECIFIED.,.F.,.F.,.F.,(6,1,1,1,1,1,1,1,1,1,6),(2,2),(-1.,-0.9,-0.8,
-0.7,-0.6,-0.5,-0.4,-0.3,-0.2,-0.1,0.),(0.,0.7668),.UNSPECIFIED.) ;
#2081=B_SPLINE_SURFACE_WITH_KNOTS('',3,3,((#94974,#94975,#94976,#94977,
#94978,#94979,#94980,#94981,#94982,#94983),(#94984,#94985,#94986,#94987,
#94988,#94989,#94990,#94991,#94992,#94993),(#94994,#94995,#94996,#94997,
#94998,#94999,#95000,#95001,#95002,#95003),(#95004,#95005,#95006,#95007,
#95008,#95009,#95010,#95011,#95012,#95013),(#95014,#95015,#95016,#95017,
#95018,#95019,#95020,#95021,#95022,#95023)),.UNSPECIFIED.,.F.,.F.,.F.,(4,
1,4),(4,1,1,1,1,1,1,4),(0.,0.571428571428571,1.),(-0.0100926828333812,0.0417412101282966,
0.0676581566091356,0.0935751030899745,0.106533576330394,0.119492049570813,
0.132450522811233,0.171325942532491),.UNSPECIFIED.) ;
#2082=B_SPLINE_SURFACE_WITH_KNOTS('',3,3,((#95175,#95176,#95177,#95178,
#95179,#95180,#95181,#95182,#95183,#95184,#95185),(#95186,#95187,#95188,
#95189,#95190,#95191,#95192,#95193,#95194,#95195,#95196),(#95197,#95198,
#95199,#95200,#95201,#95202,#95203,#95204,#95205,#95206,#95207),(#95208,
#95209,#95210,#95211,#95212,#95213,#95214,#95215,#95216,#95217,#95218),
(#95219,#95220,#95221,#95222,#95223,#95224,#95225,#95226,#95227,#95228,
#95229)),.UNSPECIFIED.,.F.,.F.,.F.,(4,1,4),(4,1,1,1,1,1,1,1,4),(0.,0.571428571428571,
1.),(-1.38391897109284E-14,0.0292767744902657,0.0585535489805452,0.073191936225685,
0.0878303234708248,0.117107097961104,0.146383872451384,0.161022259696524,
0.204937421431943),.UNSPECIFIED.) ;
#2083=B_SPLINE_SURFACE_WITH_KNOTS('',3,3,((#95302,#95303,#95304,#95305,
#95306,#95307,#95308,#95309,#95310,#95311,#95312,#95313,#95314,#95315,#95316,
#95317),(#95318,#95319,#95320,#95321,#95322,#95323,#95324,#95325,#95326,
#95327,#95328,#95329,#95330,#95331,#95332,#95333),(#95334,#95335,#95336,
#95337,#95338,#95339,#95340,#95341,#95342,#95343,#95344,#95345,#95346,#95347,
#95348,#95349),(#95350,#95351,#95352,#95353,#95354,#95355,#95356,#95357,
#95358,#95359,#95360,#95361,#95362,#95363,#95364,#95365),(#95366,#95367,
#95368,#95369,#95370,#95371,#95372,#95373,#95374,#95375,#95376,#95377,#95378,
#95379,#95380,#95381)),.UNSPECIFIED.,.F.,.F.,.F.,(4,1,4),(4,1,1,1,1,1,1,
1,1,1,1,1,1,4),(0.,0.571428571428571,1.),(-2.12204013797473E-15,0.0295575519591679,
0.059115103918338,0.088672655877508,0.118230207836678,0.119153881335402,
0.120077554834126,0.121924901831574,0.125619595826471,0.133008983816263,
0.140398371806056,0.144093065800952,0.147787759795848,0.206902863714188),
 .UNSPECIFIED.) ;
#2084=B_SPLINE_SURFACE_WITH_KNOTS('',3,3,((#95573,#95574,#95575,#95576,
#95577,#95578,#95579,#95580,#95581,#95582,#95583,#95584,#95585),(#95586,
#95587,#95588,#95589,#95590,#95591,#95592,#95593,#95594,#95595,#95596,#95597,
#95598),(#95599,#95600,#95601,#95602,#95603,#95604,#95605,#95606,#95607,
#95608,#95609,#95610,#95611),(#95612,#95613,#95614,#95615,#95616,#95617,
#95618,#95619,#95620,#95621,#95622,#95623,#95624),(#95625,#95626,#95627,
#95628,#95629,#95630,#95631,#95632,#95633,#95634,#95635,#95636,#95637)),
 .UNSPECIFIED.,.F.,.F.,.F.,(4,1,4),(4,1,1,1,1,1,1,1,1,1,4),(0.,0.571428571428571,
1.),(-0.010282001904707,0.043288805662896,0.0566815075547967,0.0633778585007471,
0.0700742094466975,0.0767705603926478,0.080118735865623,0.0968596132304989,
0.1236450170143,0.150430420798102,0.177215824581903),.UNSPECIFIED.) ;
#2085=B_SPLINE_SURFACE_WITH_KNOTS('',3,1,((#95791,#95792),(#95793,#95794),
(#95795,#95796),(#95797,#95798),(#95799,#95800),(#95801,#95802),(#95803,
#95804),(#95805,#95806),(#95807,#95808),(#95809,#95810)),.UNSPECIFIED.,
 .F.,.F.,.F.,(4,3,3,4),(2,2),(0.158459382483081,0.476662334259652,0.810817235783357,
1.),(0.,0.0359999999999998),.UNSPECIFIED.) ;
#2086=B_SPLINE_SURFACE_WITH_KNOTS('',3,1,((#95968,#95969),(#95970,#95971),
(#95972,#95973),(#95974,#95975),(#95976,#95977),(#95978,#95979),(#95980,
#95981),(#95982,#95983),(#95984,#95985),(#95986,#95987)),.UNSPECIFIED.,
 .F.,.F.,.F.,(4,3,3,4),(2,2),(-1.,-0.68247429487388,-0.37617247715991,-0.15436867748257),
(0.,0.0359999999999998),.UNSPECIFIED.) ;
#2087=B_SPLINE_SURFACE_WITH_KNOTS('',3,3,((#96454,#96455,#96456,#96457,
#96458,#96459,#96460,#96461,#96462,#96463,#96464,#96465,#96466,#96467,#96468,
#96469,#96470,#96471,#96472,#96473,#96474,#96475,#96476),(#96477,#96478,
#96479,#96480,#96481,#96482,#96483,#96484,#96485,#96486,#96487,#96488,#96489,
#96490,#96491,#96492,#96493,#96494,#96495,#96496,#96497,#96498,#96499),
(#96500,#96501,#96502,#96503,#96504,#96505,#96506,#96507,#96508,#96509,
#96510,#96511,#96512,#96513,#96514,#96515,#96516,#96517,#96518,#96519,#96520,
#96521,#96522),(#96523,#96524,#96525,#96526,#96527,#96528,#96529,#96530,
#96531,#96532,#96533,#96534,#96535,#96536,#96537,#96538,#96539,#96540,#96541,
#96542,#96543,#96544,#96545),(#96546,#96547,#96548,#96549,#96550,#96551,
#96552,#96553,#96554,#96555,#96556,#96557,#96558,#96559,#96560,#96561,#96562,
#96563,#96564,#96565,#96566,#96567,#96568),(#96569,#96570,#96571,#96572,
#96573,#96574,#96575,#96576,#96577,#96578,#96579,#96580,#96581,#96582,#96583,
#96584,#96585,#96586,#96587,#96588,#96589,#96590,#96591)),.UNSPECIFIED.,
 .F.,.F.,.F.,(4,1,1,4),(4,1,1,1,1,1,1,1,1,1,1,1,1,1,1,1,1,1,2,4),(0.,0.285714285714286,
0.571428571428571,1.),(-3.27226604903845E-14,0.0211428683856211,0.0422857367712749,
0.0634286051569287,0.0740000393497556,0.0746607539868073,0.0753214686238589,
0.0759821832609106,0.0766428978979623,0.079285756446169,0.0845714735425825,
0.0951429077354094,0.100428624831823,0.104392912654133,0.105053627291185,
0.105714341928236,0.116285776121063,0.12685721031389,0.148000078699544,
0.158000078699635),.UNSPECIFIED.) ;
#2088=B_SPLINE_SURFACE_WITH_KNOTS('',3,3,((#96795,#96796,#96797,#96798,
#96799,#96800,#96801,#96802,#96803,#96804,#96805),(#96806,#96807,#96808,
#96809,#96810,#96811,#96812,#96813,#96814,#96815,#96816),(#96817,#96818,
#96819,#96820,#96821,#96822,#96823,#96824,#96825,#96826,#96827),(#96828,
#96829,#96830,#96831,#96832,#96833,#96834,#96835,#96836,#96837,#96838),
(#96839,#96840,#96841,#96842,#96843,#96844,#96845,#96846,#96847,#96848,
#96849),(#96850,#96851,#96852,#96853,#96854,#96855,#96856,#96857,#96858,
#96859,#96860),(#96861,#96862,#96863,#96864,#96865,#96866,#96867,#96868,
#96869,#96870,#96871)),.UNSPECIFIED.,.F.,.F.,.F.,(4,1,1,1,4),(4,2,1,1,1,
1,1,4),(0.,0.285714285714286,0.571428571428571,0.857142857142857,1.),(-0.0100000000000179,
0.,0.062390566311959,0.0935858494679386,0.124781132623918,0.155976415779898,
0.179372878146882,0.218366982091857),.UNSPECIFIED.) ;
#2089=B_SPLINE_SURFACE_WITH_KNOTS('',3,1,((#96881,#96882),(#96883,#96884),
(#96885,#96886),(#96887,#96888),(#96889,#96890),(#96891,#96892),(#96893,
#96894),(#96895,#96896),(#96897,#96898),(#96899,#96900)),.UNSPECIFIED.,
 .F.,.F.,.F.,(4,3,3,4),(2,2),(-1.,-0.727595954149532,-0.403941852861304,
-0.18399442225235),(0.,0.0359999999999998),.UNSPECIFIED.) ;
#2090=B_SPLINE_SURFACE_WITH_KNOTS('',3,1,((#96904,#96905),(#96906,#96907),
(#96908,#96909),(#96910,#96911),(#96912,#96913),(#96914,#96915),(#96916,
#96917),(#96918,#96919),(#96920,#96921),(#96922,#96923)),.UNSPECIFIED.,
 .F.,.F.,.F.,(4,3,3,4),(2,2),(0.185322868216722,0.499244287262782,0.821195447612718,
1.),(0.,0.0359999999999998),.UNSPECIFIED.) ;
#2091=B_SPLINE_SURFACE_WITH_KNOTS('',3,3,((#96924,#96925,#96926,#96927,
#96928,#96929,#96930,#96931,#96932,#96933,#96934,#96935,#96936,#96937,#96938,
#96939),(#96940,#96941,#96942,#96943,#96944,#96945,#96946,#96947,#96948,
#96949,#96950,#96951,#96952,#96953,#96954,#96955),(#96956,#96957,#96958,
#96959,#96960,#96961,#96962,#96963,#96964,#96965,#96966,#96967,#96968,#96969,
#96970,#96971),(#96972,#96973,#96974,#96975,#96976,#96977,#96978,#96979,
#96980,#96981,#96982,#96983,#96984,#96985,#96986,#96987),(#96988,#96989,
#96990,#96991,#96992,#96993,#96994,#96995,#96996,#96997,#96998,#96999,#97000,
#97001,#97002,#97003),(#97004,#97005,#97006,#97007,#97008,#97009,#97010,
#97011,#97012,#97013,#97014,#97015,#97016,#97017,#97018,#97019)),
 .UNSPECIFIED.,.F.,.F.,.F.,(4,1,1,4),(4,1,1,1,1,1,1,1,1,1,1,2,4),(0.,0.285714285714286,
0.571428571428571,1.),(-1.41081590854242E-13,0.0226242588783568,0.0678727766353526,
0.0791849060746015,0.084840970794226,0.0904970355138505,0.0961531002334749,
0.101809164953099,0.107465229672724,0.113121294392348,0.135745553270846,
0.158369812149344,0.168369812149447),.UNSPECIFIED.) ;
#2092=B_SPLINE_SURFACE_WITH_KNOTS('',3,3,((#97074,#97075,#97076,#97077,
#97078,#97079,#97080,#97081,#97082,#97083,#97084),(#97085,#97086,#97087,
#97088,#97089,#97090,#97091,#97092,#97093,#97094,#97095),(#97096,#97097,
#97098,#97099,#97100,#97101,#97102,#97103,#97104,#97105,#97106),(#97107,
#97108,#97109,#97110,#97111,#97112,#97113,#97114,#97115,#97116,#97117),
(#97118,#97119,#97120,#97121,#97122,#97123,#97124,#97125,#97126,#97127,
#97128),(#97129,#97130,#97131,#97132,#97133,#97134,#97135,#97136,#97137,
#97138,#97139),(#97140,#97141,#97142,#97143,#97144,#97145,#97146,#97147,
#97148,#97149,#97150),(#97151,#97152,#97153,#97154,#97155,#97156,#97157,
#97158,#97159,#97160,#97161),(#97162,#97163,#97164,#97165,#97166,#97167,
#97168,#97169,#97170,#97171,#97172)),.UNSPECIFIED.,.F.,.F.,.F.,(4,1,1,1,
1,1,4),(4,2,1,1,1,1,1,4),(0.,0.285714285714286,0.5,0.785714285714286,0.857142857142857,
0.928571428571429,1.),(-0.0100000000001109,0.,0.0617215701552963,0.0925823552329445,
0.123443140310593,0.154303925388241,0.177449514196477,0.216025495543537),
 .UNSPECIFIED.) ;
#2093=B_SPLINE_SURFACE_WITH_KNOTS('',3,3,((#97617,#97618,#97619,#97620,
#97621,#97622),(#97623,#97624,#97625,#97626,#97627,#97628),(#97629,#97630,
#97631,#97632,#97633,#97634),(#97635,#97636,#97637,#97638,#97639,#97640),
(#97641,#97642,#97643,#97644,#97645,#97646),(#97647,#97648,#97649,#97650,
#97651,#97652),(#97653,#97654,#97655,#97656,#97657,#97658),(#97659,#97660,
#97661,#97662,#97663,#97664),(#97665,#97666,#97667,#97668,#97669,#97670),
(#97671,#97672,#97673,#97674,#97675,#97676),(#97677,#97678,#97679,#97680,
#97681,#97682),(#97683,#97684,#97685,#97686,#97687,#97688),(#97689,#97690,
#97691,#97692,#97693,#97694)),.UNSPECIFIED.,.F.,.F.,.F.,(4,1,1,1,1,1,1,
1,1,1,4),(4,1,1,4),(0.,0.1,0.2,0.3,0.4,0.5,0.6,0.7,0.8,0.9,1.),(0.,0.333333333333333,
0.666666666666667,1.),.UNSPECIFIED.) ;
#2094=B_SPLINE_SURFACE_WITH_KNOTS('',3,3,((#97698,#97699,#97700,#97701),
(#97702,#97703,#97704,#97705),(#97706,#97707,#97708,#97709),(#97710,#97711,
#97712,#97713),(#97714,#97715,#97716,#97717)),.UNSPECIFIED.,.F.,.F.,.F.,
(4,1,4),(4,4),(0.,0.5,1.),(0.,0.0936131112963942),.UNSPECIFIED.) ;
#2095=B_SPLINE_SURFACE_WITH_KNOTS('',3,3,((#97741,#97742,#97743,#97744),
(#97745,#97746,#97747,#97748),(#97749,#97750,#97751,#97752),(#97753,#97754,
#97755,#97756),(#97757,#97758,#97759,#97760)),.UNSPECIFIED.,.F.,.F.,.F.,
(4,1,4),(4,4),(-9.85495485568073E-5,0.5,1.),(-1.38376278961886,-0.927196668453033),
 .UNSPECIFIED.) ;
#2096=B_SPLINE_SURFACE_WITH_KNOTS('',3,3,((#97787,#97788,#97789,#97790),
(#97791,#97792,#97793,#97794),(#97795,#97796,#97797,#97798),(#97799,#97800,
#97801,#97802),(#97803,#97804,#97805,#97806)),.UNSPECIFIED.,.F.,.F.,.F.,
(4,1,4),(4,4),(0.,0.5,1.),(0.,0.0936141814749616),.UNSPECIFIED.) ;
#2097=B_SPLINE_SURFACE_WITH_KNOTS('',3,3,((#97838,#97839,#97840,#97841,
#97842,#97843),(#97844,#97845,#97846,#97847,#97848,#97849),(#97850,#97851,
#97852,#97853,#97854,#97855),(#97856,#97857,#97858,#97859,#97860,#97861),
(#97862,#97863,#97864,#97865,#97866,#97867)),.UNSPECIFIED.,.F.,.F.,.F.,
(4,1,4),(4,1,1,4),(-0.00794987368555094,0.571428571428571,1.),(-0.858804741536017,
-0.12155069540721,0.364652086221628,0.858804741536017),.UNSPECIFIED.) ;
#2098=B_SPLINE_SURFACE_WITH_KNOTS('',3,3,((#97869,#97870,#97871,#97872),
(#97873,#97874,#97875,#97876),(#97877,#97878,#97879,#97880),(#97881,#97882,
#97883,#97884),(#97885,#97886,#97887,#97888)),.UNSPECIFIED.,.F.,.F.,.F.,
(4,1,4),(4,4),(0.,0.5,1.),(0.,0.0936131112963941),.UNSPECIFIED.) ;
#2099=B_SPLINE_SURFACE_WITH_KNOTS('',3,3,((#97903,#97904,#97905,#97906),
(#97907,#97908,#97909,#97910),(#97911,#97912,#97913,#97914),(#97915,#97916,
#97917,#97918),(#97919,#97920,#97921,#97922)),.UNSPECIFIED.,.F.,.F.,.F.,
(4,1,4),(4,4),(0.,0.5,1.),(0.,0.0936141811972385),.UNSPECIFIED.) ;
#2100=B_SPLINE_SURFACE_WITH_KNOTS('',3,3,((#97954,#97955,#97956,#97957,
#97958,#97959),(#97960,#97961,#97962,#97963,#97964,#97965),(#97966,#97967,
#97968,#97969,#97970,#97971),(#97972,#97973,#97974,#97975,#97976,#97977),
(#97978,#97979,#97980,#97981,#97982,#97983)),.UNSPECIFIED.,.F.,.F.,.F.,
(4,1,4),(4,1,1,4),(-0.00795694173847245,0.571428571428571,1.),(-0.858811809588939,
-0.12155069540721,0.364652086221628,0.858811809588939),.UNSPECIFIED.) ;
#2101=B_SPLINE_SURFACE_WITH_KNOTS('',3,3,((#98022,#98023,#98024,#98025),
(#98026,#98027,#98028,#98029),(#98030,#98031,#98032,#98033),(#98034,#98035,
#98036,#98037),(#98038,#98039,#98040,#98041)),.UNSPECIFIED.,.F.,.F.,.F.,
(4,1,4),(4,4),(-0.00025082614922299,0.5,1.),(0.643250282643994,1.18620111781914),
 .UNSPECIFIED.) ;
#2102=B_SPLINE_SURFACE_WITH_KNOTS('',3,3,((#98054,#98055,#98056,#98057),
(#98058,#98059,#98060,#98061),(#98062,#98063,#98064,#98065),(#98066,#98067,
#98068,#98069),(#98070,#98071,#98072,#98073)),.UNSPECIFIED.,.F.,.F.,.F.,
(4,1,4),(4,4),(-9.85495485873771E-5,0.5,1.),(-1.38376278961876,-0.927196668453042),
 .UNSPECIFIED.) ;
#2103=B_SPLINE_SURFACE_WITH_KNOTS('',3,3,((#98091,#98092,#98093,#98094),
(#98095,#98096,#98097,#98098),(#98099,#98100,#98101,#98102),(#98103,#98104,
#98105,#98106),(#98107,#98108,#98109,#98110)),.UNSPECIFIED.,.F.,.F.,.F.,
(4,1,4),(4,4),(-0.0018031252703055,0.5,1.),(0.641697983523243,1.57259945206521),
 .UNSPECIFIED.) ;
#2104=B_SPLINE_SURFACE_WITH_KNOTS('',3,1,((#98176,#98177),(#98178,#98179),
(#98180,#98181),(#98182,#98183),(#98184,#98185),(#98186,#98187)),
 .UNSPECIFIED.,.F.,.F.,.F.,(4,2,4),(2,2),(-0.0699558285734079,-0.0581995466601177,
-0.0505532240038504),(0.,1.14),.UNSPECIFIED.) ;
#2105=B_SPLINE_SURFACE_WITH_KNOTS('',3,1,((#98200,#98201),(#98202,#98203),
(#98204,#98205),(#98206,#98207),(#98208,#98209),(#98210,#98211)),
 .UNSPECIFIED.,.F.,.F.,.F.,(4,2,4),(2,2),(-0.0194026045695574,-0.0117562819132905,
0.),(0.,1.14),.UNSPECIFIED.) ;
#2106=B_SPLINE_SURFACE_WITH_KNOTS('',3,1,((#98307,#98308),(#98309,#98310),
(#98311,#98312),(#98313,#98314),(#98315,#98316),(#98317,#98318)),
 .UNSPECIFIED.,.F.,.F.,.F.,(4,2,4),(2,2),(-0.0699558285734104,-0.0581995466601188,
-0.0505532240038526),(0.,1.14),.UNSPECIFIED.) ;
#2107=B_SPLINE_SURFACE_WITH_KNOTS('',3,1,((#98433,#98434),(#98435,#98436),
(#98437,#98438),(#98439,#98440),(#98441,#98442),(#98443,#98444)),
 .UNSPECIFIED.,.F.,.F.,.F.,(4,2,4),(2,2),(-0.0194026045695577,-0.0117562819132915,
0.),(0.,1.14),.UNSPECIFIED.) ;
#2108=B_SPLINE_SURFACE_WITH_KNOTS('',3,1,((#98468,#98469),(#98470,#98471),
(#98472,#98473),(#98474,#98475),(#98476,#98477),(#98478,#98479)),
 .UNSPECIFIED.,.F.,.F.,.F.,(4,2,4),(2,2),(-0.0194026045695576,-0.0117562819132903,
0.),(0.,1.14),.UNSPECIFIED.) ;
#2211=SPHERICAL_SURFACE('',#52703,0.0999999999999979) ;
#2212=SPHERICAL_SURFACE('',#52848,0.0999999999999979) ;
#2213=SPHERICAL_SURFACE('',#52943,0.0999999999999979) ;
#2214=SPHERICAL_SURFACE('',#53751,0.500000000000009) ;
#2215=SPHERICAL_SURFACE('',#53766,0.500000000000009) ;
#2563=PLANE('',#52532) ;
#2564=PLANE('',#52533) ;
#2565=PLANE('',#52534) ;
#2566=PLANE('',#52535) ;
#2567=PLANE('',#52536) ;
#2568=PLANE('',#52537) ;
#2569=PLANE('',#52538) ;
#2570=PLANE('',#52539) ;
#2571=PLANE('',#52540) ;
#2572=PLANE('',#52541) ;
#2573=PLANE('',#52542) ;
#2574=PLANE('',#52543) ;
#2575=PLANE('',#52544) ;
#2576=PLANE('',#52569) ;
#2577=PLANE('',#52572) ;
#2578=PLANE('',#52586) ;
#2579=PLANE('',#52589) ;
#2580=PLANE('',#52591) ;
#2581=PLANE('',#52592) ;
#2582=PLANE('',#52609) ;
#2583=PLANE('',#52623) ;
#2584=PLANE('',#52638) ;
#2585=PLANE('',#52641) ;
#2586=PLANE('',#52642) ;
#2587=PLANE('',#52648) ;
#2588=PLANE('',#52654) ;
#2589=PLANE('',#52658) ;
#2590=PLANE('',#52667) ;
#2591=PLANE('',#52696) ;
#2592=PLANE('',#52699) ;
#2593=PLANE('',#52735) ;
#2594=PLANE('',#52743) ;
#2595=PLANE('',#52753) ;
#2596=PLANE('',#52795) ;
#2597=PLANE('',#52798) ;
#2598=PLANE('',#52819) ;
#2599=PLANE('',#52821) ;
#2600=PLANE('',#52833) ;
#2601=PLANE('',#52834) ;
#2602=PLANE('',#52843) ;
#2603=PLANE('',#52862) ;
#2604=PLANE('',#52927) ;
#2605=PLANE('',#52941) ;
#2606=PLANE('',#52942) ;
#2607=PLANE('',#52990) ;
#2608=PLANE('',#52992) ;
#2609=PLANE('',#52996) ;
#2610=PLANE('',#52999) ;
#2611=PLANE('',#53005) ;
#2612=PLANE('',#53093) ;
#2613=PLANE('',#53097) ;
#2614=PLANE('',#53098) ;
#2615=PLANE('',#53099) ;
#2616=PLANE('',#53100) ;
#2617=PLANE('',#53101) ;
#2618=PLANE('',#53106) ;
#2619=PLANE('',#53143) ;
#2620=PLANE('',#53150) ;
#2621=PLANE('',#53214) ;
#2622=PLANE('',#53217) ;
#2623=PLANE('',#53220) ;
#2624=PLANE('',#53269) ;
#2625=PLANE('',#53270) ;
#2626=PLANE('',#53272) ;
#2627=PLANE('',#53278) ;
#2628=PLANE('',#53280) ;
#2629=PLANE('',#53285) ;
#2630=PLANE('',#53286) ;
#2631=PLANE('',#53314) ;
#2632=PLANE('',#53316) ;
#2633=PLANE('',#53327) ;
#2634=PLANE('',#53328) ;
#2635=PLANE('',#53329) ;
#2636=PLANE('',#53350) ;
#2637=PLANE('',#53359) ;
#2638=PLANE('',#53368) ;
#2639=PLANE('',#53372) ;
#2640=PLANE('',#53374) ;
#2641=PLANE('',#53375) ;
#2642=PLANE('',#53380) ;
#2643=PLANE('',#53382) ;
#2644=PLANE('',#53384) ;
#2645=PLANE('',#53387) ;
#2646=PLANE('',#53393) ;
#2647=PLANE('',#53394) ;
#2648=PLANE('',#53395) ;
#2649=PLANE('',#53396) ;
#2650=PLANE('',#53407) ;
#2651=PLANE('',#53408) ;
#2652=PLANE('',#53409) ;
#2653=PLANE('',#53410) ;
#2654=PLANE('',#53411) ;
#2655=PLANE('',#53412) ;
#2656=PLANE('',#53413) ;
#2657=PLANE('',#53414) ;
#2658=PLANE('',#53423) ;
#2659=PLANE('',#53424) ;
#2660=PLANE('',#53425) ;
#2661=PLANE('',#53426) ;
#2662=PLANE('',#53427) ;
#2663=PLANE('',#53436) ;
#2664=PLANE('',#53437) ;
#2665=PLANE('',#53438) ;
#2666=PLANE('',#53453) ;
#2667=PLANE('',#53454) ;
#2668=PLANE('',#53455) ;
#2669=PLANE('',#53456) ;
#2670=PLANE('',#53457) ;
#2671=PLANE('',#53466) ;
#2672=PLANE('',#53467) ;
#2673=PLANE('',#53468) ;
#2674=PLANE('',#53483) ;
#2675=PLANE('',#53484) ;
#2676=PLANE('',#53485) ;
#2677=PLANE('',#53486) ;
#2678=PLANE('',#53487) ;
#2679=PLANE('',#53496) ;
#2680=PLANE('',#53497) ;
#2681=PLANE('',#53498) ;
#2682=PLANE('',#53525) ;
#2683=PLANE('',#53528) ;
#2684=PLANE('',#53529) ;
#2685=PLANE('',#53530) ;
#2686=PLANE('',#53531) ;
#2687=PLANE('',#53532) ;
#2688=PLANE('',#53561) ;
#2689=PLANE('',#53562) ;
#2690=PLANE('',#53563) ;
#2691=PLANE('',#53564) ;
#2692=PLANE('',#53565) ;
#2693=PLANE('',#53566) ;
#2694=PLANE('',#53575) ;
#2695=PLANE('',#53584) ;
#2696=PLANE('',#53585) ;
#2697=PLANE('',#53600) ;
#2698=PLANE('',#53601) ;
#2699=PLANE('',#53602) ;
#2700=PLANE('',#53603) ;
#2701=PLANE('',#53617) ;
#2702=PLANE('',#53632) ;
#2703=PLANE('',#53633) ;
#2704=PLANE('',#53664) ;
#2705=PLANE('',#53666) ;
#2706=PLANE('',#53667) ;
#2707=PLANE('',#53691) ;
#2708=PLANE('',#53692) ;
#2709=PLANE('',#53693) ;
#2710=PLANE('',#53695) ;
#2711=PLANE('',#53696) ;
#2712=PLANE('',#53697) ;
#2713=PLANE('',#53698) ;
#2714=PLANE('',#53699) ;
#2715=PLANE('',#53700) ;
#2716=PLANE('',#53701) ;
#2717=PLANE('',#53702) ;
#2718=PLANE('',#53703) ;
#2719=PLANE('',#53706) ;
#2720=PLANE('',#53709) ;
#2721=PLANE('',#53712) ;
#2722=PLANE('',#53713) ;
#2723=PLANE('',#53714) ;
#2724=PLANE('',#53715) ;
#2725=PLANE('',#53719) ;
#2726=PLANE('',#53720) ;
#2727=PLANE('',#53721) ;
#2728=PLANE('',#53722) ;
#2729=PLANE('',#53723) ;
#2730=PLANE('',#53724) ;
#2731=PLANE('',#53725) ;
#2732=PLANE('',#53726) ;
#2733=PLANE('',#53727) ;
#2734=PLANE('',#53730) ;
#2735=PLANE('',#53731) ;
#2736=PLANE('',#53732) ;
#2737=PLANE('',#53735) ;
#2738=PLANE('',#53736) ;
#2739=PLANE('',#53737) ;
#2740=PLANE('',#53738) ;
#2741=PLANE('',#53739) ;
#2742=PLANE('',#53742) ;
#2743=PLANE('',#53744) ;
#2744=PLANE('',#53745) ;
#2745=PLANE('',#53746) ;
#2746=PLANE('',#53747) ;
#2747=PLANE('',#53748) ;
#2748=PLANE('',#53824) ;
#2749=PLANE('',#53826) ;
#2750=PLANE('',#53828) ;
#2751=PLANE('',#53829) ;
#2752=PLANE('',#53834) ;
#2753=PLANE('',#53837) ;
#2754=PLANE('',#53838) ;
#2755=PLANE('',#53841) ;
#2756=PLANE('',#53844) ;
#2757=PLANE('',#53845) ;
#2758=PLANE('',#53846) ;
#2759=PLANE('',#53848) ;
#2760=PLANE('',#53853) ;
#2761=PLANE('',#53856) ;
#2762=PLANE('',#53859) ;
#2763=PLANE('',#53862) ;
#2764=PLANE('',#53865) ;
#2765=PLANE('',#53866) ;
#2766=PLANE('',#53869) ;
#2767=PLANE('',#53872) ;
#2768=PLANE('',#53875) ;
#2769=PLANE('',#53878) ;
#2770=PLANE('',#53881) ;
#2771=PLANE('',#53884) ;
#2772=PLANE('',#53885) ;
#2773=PLANE('',#53886) ;
#2774=PLANE('',#53889) ;
#2775=PLANE('',#53892) ;
#2776=PLANE('',#53897) ;
#2777=PLANE('',#53900) ;
#2778=PLANE('',#53901) ;
#2779=PLANE('',#53904) ;
#2780=PLANE('',#53907) ;
#2781=PLANE('',#53908) ;
#2782=PLANE('',#53911) ;
#2783=PLANE('',#53914) ;
#2784=PLANE('',#53915) ;
#2785=PLANE('',#53916) ;
#2786=PLANE('',#53917) ;
#2787=PLANE('',#53920) ;
#2788=PLANE('',#53923) ;
#2789=PLANE('',#53924) ;
#2790=PLANE('',#53925) ;
#2791=PLANE('',#53928) ;
#2792=PLANE('',#53931) ;
#2793=PLANE('',#53932) ;
#2794=PLANE('',#53935) ;
#2795=PLANE('',#53936) ;
#2796=PLANE('',#53937) ;
#2797=PLANE('',#53938) ;
#2798=PLANE('',#53939) ;
#2799=PLANE('',#53942) ;
#2800=PLANE('',#53946) ;
#2801=PLANE('',#53947) ;
#2802=PLANE('',#53950) ;
#2803=PLANE('',#53953) ;
#2804=PLANE('',#53954) ;
#2805=PLANE('',#53957) ;
#2806=PLANE('',#53960) ;
#2807=PLANE('',#53963) ;
#2808=PLANE('',#53964) ;
#2809=PLANE('',#53965) ;
#2810=PLANE('',#53968) ;
#2811=PLANE('',#53969) ;
#2812=PLANE('',#53970) ;
#2813=PLANE('',#53971) ;
#2814=PLANE('',#53972) ;
#2815=PLANE('',#53973) ;
#2816=PLANE('',#53974) ;
#2817=PLANE('',#53975) ;
#2818=PLANE('',#53976) ;
#2819=PLANE('',#53978) ;
#2820=PLANE('',#53980) ;
#2821=PLANE('',#53981) ;
#2822=PLANE('',#53985) ;
#2823=PLANE('',#53987) ;
#2824=PLANE('',#53988) ;
#2825=PLANE('',#53989) ;
#2826=PLANE('',#53990) ;
#2827=PLANE('',#53991) ;
#2828=PLANE('',#53993) ;
#2829=PLANE('',#53995) ;
#2830=PLANE('',#53996) ;
#2831=PLANE('',#53999) ;
#2832=PLANE('',#54001) ;
#2833=PLANE('',#54003) ;
#2834=PLANE('',#54004) ;
#2835=PLANE('',#54006) ;
#2836=PLANE('',#54007) ;
#2837=PLANE('',#54008) ;
#2838=PLANE('',#54009) ;
#2839=PLANE('',#54010) ;
#4592=LINE('',#89877,#7806) ;
#4593=LINE('',#89879,#7807) ;
#4594=LINE('',#89881,#7808) ;
#4595=LINE('',#89882,#7809) ;
#4596=LINE('',#89900,#7810) ;
#4597=LINE('',#89923,#7811) ;
#4598=LINE('',#89946,#7812) ;
#4599=LINE('',#89969,#7813) ;
#4600=LINE('',#89992,#7814) ;
#4601=LINE('',#90000,#7815) ;
#4602=LINE('',#90002,#7816) ;
#4603=LINE('',#90003,#7817) ;
#4604=LINE('',#90005,#7818) ;
#4605=LINE('',#90006,#7819) ;
#4606=LINE('',#90010,#7820) ;
#4607=LINE('',#90012,#7821) ;
#4608=LINE('',#90014,#7822) ;
#4609=LINE('',#90015,#7823) ;
#4610=LINE('',#90018,#7824) ;
#4611=LINE('',#90020,#7825) ;
#4612=LINE('',#90021,#7826) ;
#4613=LINE('',#90039,#7827) ;
#4614=LINE('',#90062,#7828) ;
#4615=LINE('',#90085,#7829) ;
#4616=LINE('',#90108,#7830) ;
#4617=LINE('',#90116,#7831) ;
#4618=LINE('',#90118,#7832) ;
#4619=LINE('',#90119,#7833) ;
#4620=LINE('',#90122,#7834) ;
#4621=LINE('',#90124,#7835) ;
#4622=LINE('',#90125,#7836) ;
#4623=LINE('',#90128,#7837) ;
#4624=LINE('',#90130,#7838) ;
#4625=LINE('',#90131,#7839) ;
#4626=LINE('',#90149,#7840) ;
#4627=LINE('',#90172,#7841) ;
#4628=LINE('',#90195,#7842) ;
#4629=LINE('',#90218,#7843) ;
#4630=LINE('',#90241,#7844) ;
#4631=LINE('',#90264,#7845) ;
#4632=LINE('',#90287,#7846) ;
#4633=LINE('',#90295,#7847) ;
#4634=LINE('',#90297,#7848) ;
#4635=LINE('',#90298,#7849) ;
#4636=LINE('',#90301,#7850) ;
#4637=LINE('',#90303,#7851) ;
#4638=LINE('',#90304,#7852) ;
#4639=LINE('',#90306,#7853) ;
#4640=LINE('',#90307,#7854) ;
#4641=LINE('',#90312,#7855) ;
#4642=LINE('',#90314,#7856) ;
#4643=LINE('',#90318,#7857) ;
#4644=LINE('',#90322,#7858) ;
#4645=LINE('',#90326,#7859) ;
#4646=LINE('',#90332,#7860) ;
#4647=LINE('',#90336,#7861) ;
#4648=LINE('',#90340,#7862) ;
#4649=LINE('',#90344,#7863) ;
#4650=LINE('',#90348,#7864) ;
#4651=LINE('',#90352,#7865) ;
#4652=LINE('',#90353,#7866) ;
#4653=LINE('',#90366,#7867) ;
#4654=LINE('',#90369,#7868) ;
#4655=LINE('',#90390,#7869) ;
#4656=LINE('',#90417,#7870) ;
#4657=LINE('',#90418,#7871) ;
#4658=LINE('',#90442,#7872) ;
#4659=LINE('',#90443,#7873) ;
#4660=LINE('',#90509,#7874) ;
#4661=LINE('',#90511,#7875) ;
#4662=LINE('',#90513,#7876) ;
#4663=LINE('',#90515,#7877) ;
#4664=LINE('',#90516,#7878) ;
#4665=LINE('',#90519,#7879) ;
#4666=LINE('',#90523,#7880) ;
#4667=LINE('',#90524,#7881) ;
#4668=LINE('',#90595,#7882) ;
#4669=LINE('',#90596,#7883) ;
#4670=LINE('',#90615,#7884) ;
#4671=LINE('',#90616,#7885) ;
#4672=LINE('',#90630,#7886) ;
#4673=LINE('',#90632,#7887) ;
#4674=LINE('',#90633,#7888) ;
#4675=LINE('',#90636,#7889) ;
#4676=LINE('',#90640,#7890) ;
#4677=LINE('',#90641,#7891) ;
#4678=LINE('',#90709,#7892) ;
#4679=LINE('',#90754,#7893) ;
#4680=LINE('',#90775,#7894) ;
#4681=LINE('',#90785,#7895) ;
#4682=LINE('',#90787,#7896) ;
#4683=LINE('',#90789,#7897) ;
#4684=LINE('',#90791,#7898) ;
#4685=LINE('',#90795,#7899) ;
#4686=LINE('',#90798,#7900) ;
#4687=LINE('',#90838,#7901) ;
#4688=LINE('',#90839,#7902) ;
#4689=LINE('',#90904,#7903) ;
#4690=LINE('',#90907,#7904) ;
#4691=LINE('',#90910,#7905) ;
#4692=LINE('',#90912,#7906) ;
#4693=LINE('',#90916,#7907) ;
#4694=LINE('',#90957,#7908) ;
#4695=LINE('',#90958,#7909) ;
#4696=LINE('',#91032,#7910) ;
#4697=LINE('',#91034,#7911) ;
#4698=LINE('',#91038,#7912) ;
#4699=LINE('',#91042,#7913) ;
#4700=LINE('',#91043,#7914) ;
#4701=LINE('',#91045,#7915) ;
#4702=LINE('',#91047,#7916) ;
#4703=LINE('',#91051,#7917) ;
#4704=LINE('',#91052,#7918) ;
#4705=LINE('',#91055,#7919) ;
#4706=LINE('',#91059,#7920) ;
#4707=LINE('',#91062,#7921) ;
#4708=LINE('',#91091,#7922) ;
#4709=LINE('',#91094,#7923) ;
#4710=LINE('',#91097,#7924) ;
#4711=LINE('',#91110,#7925) ;
#4712=LINE('',#91113,#7926) ;
#4713=LINE('',#91116,#7927) ;
#4714=LINE('',#91118,#7928) ;
#4715=LINE('',#91120,#7929) ;
#4716=LINE('',#91122,#7930) ;
#4717=LINE('',#91126,#7931) ;
#4718=LINE('',#91129,#7932) ;
#4719=LINE('',#91131,#7933) ;
#4720=LINE('',#91135,#7934) ;
#4721=LINE('',#91139,#7935) ;
#4722=LINE('',#91142,#7936) ;
#4723=LINE('',#91145,#7937) ;
#4724=LINE('',#91154,#7938) ;
#4725=LINE('',#91189,#7939) ;
#4726=LINE('',#91190,#7940) ;
#4727=LINE('',#91193,#7941) ;
#4728=LINE('',#91197,#7942) ;
#4729=LINE('',#91198,#7943) ;
#4730=LINE('',#91201,#7944) ;
#4731=LINE('',#91205,#7945) ;
#4732=LINE('',#91207,#7946) ;
#4733=LINE('',#91209,#7947) ;
#4734=LINE('',#91211,#7948) ;
#4735=LINE('',#91212,#7949) ;
#4736=LINE('',#91222,#7950) ;
#4737=LINE('',#91225,#7951) ;
#4738=LINE('',#91228,#7952) ;
#4739=LINE('',#91231,#7953) ;
#4740=LINE('',#91233,#7954) ;
#4741=LINE('',#91235,#7955) ;
#4742=LINE('',#91248,#7956) ;
#4743=LINE('',#91260,#7957) ;
#4744=LINE('',#91271,#7958) ;
#4745=LINE('',#91272,#7959) ;
#4746=LINE('',#91279,#7960) ;
#4747=LINE('',#91282,#7961) ;
#4748=LINE('',#91284,#7962) ;
#4749=LINE('',#91286,#7963) ;
#4750=LINE('',#91288,#7964) ;
#4751=LINE('',#91290,#7965) ;
#4752=LINE('',#91291,#7966) ;
#4753=LINE('',#91294,#7967) ;
#4754=LINE('',#91298,#7968) ;
#4755=LINE('',#91302,#7969) ;
#4756=LINE('',#91304,#7970) ;
#4757=LINE('',#91306,#7971) ;
#4758=LINE('',#91330,#7972) ;
#4759=LINE('',#91331,#7973) ;
#4760=LINE('',#91360,#7974) ;
#4761=LINE('',#91361,#7975) ;
#4762=LINE('',#91378,#7976) ;
#4763=LINE('',#91379,#7977) ;
#4764=LINE('',#91387,#7978) ;
#4765=LINE('',#91388,#7979) ;
#4766=LINE('',#91393,#7980) ;
#4767=LINE('',#91394,#7981) ;
#4768=LINE('',#91408,#7982) ;
#4769=LINE('',#91412,#7983) ;
#4770=LINE('',#91416,#7984) ;
#4771=LINE('',#91418,#7985) ;
#4772=LINE('',#91420,#7986) ;
#4773=LINE('',#91428,#7987) ;
#4774=LINE('',#91432,#7988) ;
#4775=LINE('',#91433,#7989) ;
#4776=LINE('',#91439,#7990) ;
#4777=LINE('',#91443,#7991) ;
#4778=LINE('',#91516,#7992) ;
#4779=LINE('',#91520,#7993) ;
#4780=LINE('',#91523,#7994) ;
#4781=LINE('',#91574,#7995) ;
#4782=LINE('',#91576,#7996) ;
#4783=LINE('',#91577,#7997) ;
#4784=LINE('',#91589,#7998) ;
#4785=LINE('',#91595,#7999) ;
#4786=LINE('',#91656,#8000) ;
#4787=LINE('',#91657,#8001) ;
#4788=LINE('',#91713,#8002) ;
#4789=LINE('',#91721,#8003) ;
#4790=LINE('',#91732,#8004) ;
#4791=LINE('',#91733,#8005) ;
#4792=LINE('',#91739,#8006) ;
#4793=LINE('',#91743,#8007) ;
#4794=LINE('',#91744,#8008) ;
#4795=LINE('',#91747,#8009) ;
#4796=LINE('',#91751,#8010) ;
#4797=LINE('',#91753,#8011) ;
#4798=LINE('',#91755,#8012) ;
#4799=LINE('',#91756,#8013) ;
#4800=LINE('',#91759,#8014) ;
#4801=LINE('',#91764,#8015) ;
#4802=LINE('',#91860,#8016) ;
#4803=LINE('',#91861,#8017) ;
#4804=LINE('',#91944,#8018) ;
#4805=LINE('',#91952,#8019) ;
#4806=LINE('',#91955,#8020) ;
#4807=LINE('',#91957,#8021) ;
#4808=LINE('',#91959,#8022) ;
#4809=LINE('',#91970,#8023) ;
#4810=LINE('',#91973,#8024) ;
#4811=LINE('',#91976,#8025) ;
#4812=LINE('',#91982,#8026) ;
#4813=LINE('',#92016,#8027) ;
#4814=LINE('',#92019,#8028) ;
#4815=LINE('',#92022,#8029) ;
#4816=LINE('',#92025,#8030) ;
#4817=LINE('',#92028,#8031) ;
#4818=LINE('',#92029,#8032) ;
#4819=LINE('',#92088,#8033) ;
#4820=LINE('',#92089,#8034) ;
#4821=LINE('',#92092,#8035) ;
#4822=LINE('',#92094,#8036) ;
#4823=LINE('',#92096,#8037) ;
#4824=LINE('',#92098,#8038) ;
#4825=LINE('',#92099,#8039) ;
#4826=LINE('',#92102,#8040) ;
#4827=LINE('',#92106,#8041) ;
#4828=LINE('',#92109,#8042) ;
#4829=LINE('',#92118,#8043) ;
#4830=LINE('',#92119,#8044) ;
#4831=LINE('',#92121,#8045) ;
#4832=LINE('',#92122,#8046) ;
#4833=LINE('',#92133,#8047) ;
#4834=LINE('',#92134,#8048) ;
#4835=LINE('',#92136,#8049) ;
#4836=LINE('',#92137,#8050) ;
#4837=LINE('',#92139,#8051) ;
#4838=LINE('',#92140,#8052) ;
#4839=LINE('',#92143,#8053) ;
#4840=LINE('',#92147,#8054) ;
#4841=LINE('',#92151,#8055) ;
#4842=LINE('',#92155,#8056) ;
#4843=LINE('',#92159,#8057) ;
#4844=LINE('',#92161,#8058) ;
#4845=LINE('',#92163,#8059) ;
#4846=LINE('',#92165,#8060) ;
#4847=LINE('',#92167,#8061) ;
#4848=LINE('',#92171,#8062) ;
#4849=LINE('',#92175,#8063) ;
#4850=LINE('',#92179,#8064) ;
#4851=LINE('',#92183,#8065) ;
#4852=LINE('',#92187,#8066) ;
#4853=LINE('',#92191,#8067) ;
#4854=LINE('',#92193,#8068) ;
#4855=LINE('',#92195,#8069) ;
#4856=LINE('',#92199,#8070) ;
#4857=LINE('',#92203,#8071) ;
#4858=LINE('',#92207,#8072) ;
#4859=LINE('',#92211,#8073) ;
#4860=LINE('',#92215,#8074) ;
#4861=LINE('',#92217,#8075) ;
#4862=LINE('',#92219,#8076) ;
#4863=LINE('',#92221,#8077) ;
#4864=LINE('',#92223,#8078) ;
#4865=LINE('',#92225,#8079) ;
#4866=LINE('',#92234,#8080) ;
#4867=LINE('',#92243,#8081) ;
#4868=LINE('',#92245,#8082) ;
#4869=LINE('',#92247,#8083) ;
#4870=LINE('',#92251,#8084) ;
#4871=LINE('',#92255,#8085) ;
#4872=LINE('',#92257,#8086) ;
#4873=LINE('',#92261,#8087) ;
#4874=LINE('',#92263,#8088) ;
#4875=LINE('',#92267,#8089) ;
#4876=LINE('',#92276,#8090) ;
#4877=LINE('',#92278,#8091) ;
#4878=LINE('',#92280,#8092) ;
#4879=LINE('',#92290,#8093) ;
#4880=LINE('',#92294,#8094) ;
#4881=LINE('',#92296,#8095) ;
#4882=LINE('',#92300,#8096) ;
#4883=LINE('',#92304,#8097) ;
#4884=LINE('',#92306,#8098) ;
#4885=LINE('',#92310,#8099) ;
#4886=LINE('',#92314,#8100) ;
#4887=LINE('',#92316,#8101) ;
#4888=LINE('',#92318,#8102) ;
#4889=LINE('',#92322,#8103) ;
#4890=LINE('',#92326,#8104) ;
#4891=LINE('',#92330,#8105) ;
#4892=LINE('',#92334,#8106) ;
#4893=LINE('',#92335,#8107) ;
#4894=LINE('',#92341,#8108) ;
#4895=LINE('',#92345,#8109) ;
#4896=LINE('',#92347,#8110) ;
#4897=LINE('',#92351,#8111) ;
#4898=LINE('',#92357,#8112) ;
#4899=LINE('',#92358,#8113) ;
#4900=LINE('',#92363,#8114) ;
#4901=LINE('',#92367,#8115) ;
#4902=LINE('',#92371,#8116) ;
#4903=LINE('',#92374,#8117) ;
#4904=LINE('',#92381,#8118) ;
#4905=LINE('',#92385,#8119) ;
#4906=LINE('',#92387,#8120) ;
#4907=LINE('',#92391,#8121) ;
#4908=LINE('',#92395,#8122) ;
#4909=LINE('',#92399,#8123) ;
#4910=LINE('',#92403,#8124) ;
#4911=LINE('',#92404,#8125) ;
#4912=LINE('',#92409,#8126) ;
#4913=LINE('',#92418,#8127) ;
#4914=LINE('',#92422,#8128) ;
#4915=LINE('',#92426,#8129) ;
#4916=LINE('',#92430,#8130) ;
#4917=LINE('',#92434,#8131) ;
#4918=LINE('',#92449,#8132) ;
#4919=LINE('',#92451,#8133) ;
#4920=LINE('',#92453,#8134) ;
#4921=LINE('',#92457,#8135) ;
#4922=LINE('',#92461,#8136) ;
#4923=LINE('',#92465,#8137) ;
#4924=LINE('',#92469,#8138) ;
#4925=LINE('',#92470,#8139) ;
#4926=LINE('',#92475,#8140) ;
#4927=LINE('',#92479,#8141) ;
#4928=LINE('',#92481,#8142) ;
#4929=LINE('',#92485,#8143) ;
#4930=LINE('',#92489,#8144) ;
#4931=LINE('',#92493,#8145) ;
#4932=LINE('',#92497,#8146) ;
#4933=LINE('',#92498,#8147) ;
#4934=LINE('',#92578,#8148) ;
#4935=LINE('',#92579,#8149) ;
#4936=LINE('',#92609,#8150) ;
#4937=LINE('',#92611,#8151) ;
#4938=LINE('',#92614,#8152) ;
#4939=LINE('',#92617,#8153) ;
#4940=LINE('',#92620,#8154) ;
#4941=LINE('',#92621,#8155) ;
#4942=LINE('',#92623,#8156) ;
#4943=LINE('',#92624,#8157) ;
#4944=LINE('',#92626,#8158) ;
#4945=LINE('',#92628,#8159) ;
#4946=LINE('',#92630,#8160) ;
#4947=LINE('',#92631,#8161) ;
#4948=LINE('',#92641,#8162) ;
#4949=LINE('',#92644,#8163) ;
#4950=LINE('',#92655,#8164) ;
#4951=LINE('',#92656,#8165) ;
#4952=LINE('',#92664,#8166) ;
#4953=LINE('',#92665,#8167) ;
#4954=LINE('',#92684,#8168) ;
#4955=LINE('',#92687,#8169) ;
#4956=LINE('',#92695,#8170) ;
#4957=LINE('',#92696,#8171) ;
#4958=LINE('',#92772,#8172) ;
#4959=LINE('',#92778,#8173) ;
#4960=LINE('',#92780,#8174) ;
#4961=LINE('',#92781,#8175) ;
#4962=LINE('',#92785,#8176) ;
#4963=LINE('',#92793,#8177) ;
#4964=LINE('',#92841,#8178) ;
#4965=LINE('',#92843,#8179) ;
#4966=LINE('',#92847,#8180) ;
#4967=LINE('',#92849,#8181) ;
#4968=LINE('',#92851,#8182) ;
#4969=LINE('',#92855,#8183) ;
#4970=LINE('',#92859,#8184) ;
#4971=LINE('',#92860,#8185) ;
#4972=LINE('',#92863,#8186) ;
#4973=LINE('',#92867,#8187) ;
#4974=LINE('',#92869,#8188) ;
#4975=LINE('',#92873,#8189) ;
#4976=LINE('',#92877,#8190) ;
#4977=LINE('',#92880,#8191) ;
#4978=LINE('',#92883,#8192) ;
#4979=LINE('',#92887,#8193) ;
#4980=LINE('',#92888,#8194) ;
#4981=LINE('',#92891,#8195) ;
#4982=LINE('',#92973,#8196) ;
#4983=LINE('',#92974,#8197) ;
#4984=LINE('',#92988,#8198) ;
#4985=LINE('',#92989,#8199) ;
#4986=LINE('',#93076,#8200) ;
#4987=LINE('',#93077,#8201) ;
#4988=LINE('',#93082,#8202) ;
#4989=LINE('',#93083,#8203) ;
#4990=LINE('',#93145,#8204) ;
#4991=LINE('',#93150,#8205) ;
#4992=LINE('',#93151,#8206) ;
#4993=LINE('',#93159,#8207) ;
#4994=LINE('',#93165,#8208) ;
#4995=LINE('',#93170,#8209) ;
#4996=LINE('',#93171,#8210) ;
#4997=LINE('',#93176,#8211) ;
#4998=LINE('',#93177,#8212) ;
#4999=LINE('',#93188,#8213) ;
#5000=LINE('',#93189,#8214) ;
#5001=LINE('',#93200,#8215) ;
#5002=LINE('',#93201,#8216) ;
#5003=LINE('',#93212,#8217) ;
#5004=LINE('',#93213,#8218) ;
#5005=LINE('',#93221,#8219) ;
#5006=LINE('',#93222,#8220) ;
#5007=LINE('',#93227,#8221) ;
#5008=LINE('',#93228,#8222) ;
#5009=LINE('',#93291,#8223) ;
#5010=LINE('',#93292,#8224) ;
#5011=LINE('',#93296,#8225) ;
#5012=LINE('',#93299,#8226) ;
#5013=LINE('',#93306,#8227) ;
#5014=LINE('',#93309,#8228) ;
#5015=LINE('',#93311,#8229) ;
#5016=LINE('',#93312,#8230) ;
#5017=LINE('',#93314,#8231) ;
#5018=LINE('',#93316,#8232) ;
#5019=LINE('',#93319,#8233) ;
#5020=LINE('',#93322,#8234) ;
#5021=LINE('',#93324,#8235) ;
#5022=LINE('',#93326,#8236) ;
#5023=LINE('',#93327,#8237) ;
#5024=LINE('',#93329,#8238) ;
#5025=LINE('',#93332,#8239) ;
#5026=LINE('',#93333,#8240) ;
#5027=LINE('',#93334,#8241) ;
#5028=LINE('',#93336,#8242) ;
#5029=LINE('',#93339,#8243) ;
#5030=LINE('',#93346,#8244) ;
#5031=LINE('',#93349,#8245) ;
#5032=LINE('',#93352,#8246) ;
#5033=LINE('',#93354,#8247) ;
#5034=LINE('',#93355,#8248) ;
#5035=LINE('',#93361,#8249) ;
#5036=LINE('',#93381,#8250) ;
#5037=LINE('',#93382,#8251) ;
#5038=LINE('',#93388,#8252) ;
#5039=LINE('',#93391,#8253) ;
#5040=LINE('',#93399,#8254) ;
#5041=LINE('',#93400,#8255) ;
#5042=LINE('',#93405,#8256) ;
#5043=LINE('',#93406,#8257) ;
#5044=LINE('',#93411,#8258) ;
#5045=LINE('',#93412,#8259) ;
#5046=LINE('',#93417,#8260) ;
#5047=LINE('',#93418,#8261) ;
#5048=LINE('',#93429,#8262) ;
#5049=LINE('',#93430,#8263) ;
#5050=LINE('',#93433,#8264) ;
#5051=LINE('',#93436,#8265) ;
#5052=LINE('',#93439,#8266) ;
#5053=LINE('',#93441,#8267) ;
#5054=LINE('',#93445,#8268) ;
#5055=LINE('',#93447,#8269) ;
#5056=LINE('',#93451,#8270) ;
#5057=LINE('',#93455,#8271) ;
#5058=LINE('',#93458,#8272) ;
#5059=LINE('',#93461,#8273) ;
#5060=LINE('',#93465,#8274) ;
#5061=LINE('',#93467,#8275) ;
#5062=LINE('',#93469,#8276) ;
#5063=LINE('',#93471,#8277) ;
#5064=LINE('',#93472,#8278) ;
#5065=LINE('',#93473,#8279) ;
#5066=LINE('',#93474,#8280) ;
#5067=LINE('',#93479,#8281) ;
#5068=LINE('',#93520,#8282) ;
#5069=LINE('',#93528,#8283) ;
#5070=LINE('',#93536,#8284) ;
#5071=LINE('',#93544,#8285) ;
#5072=LINE('',#93552,#8286) ;
#5073=LINE('',#93560,#8287) ;
#5074=LINE('',#93591,#8288) ;
#5075=LINE('',#93694,#8289) ;
#5076=LINE('',#93705,#8290) ;
#5077=LINE('',#93714,#8291) ;
#5078=LINE('',#93715,#8292) ;
#5079=LINE('',#93719,#8293) ;
#5080=LINE('',#93721,#8294) ;
#5081=LINE('',#93723,#8295) ;
#5082=LINE('',#93725,#8296) ;
#5083=LINE('',#93730,#8297) ;
#5084=LINE('',#93735,#8298) ;
#5085=LINE('',#93742,#8299) ;
#5086=LINE('',#93750,#8300) ;
#5087=LINE('',#93761,#8301) ;
#5088=LINE('',#93768,#8302) ;
#5089=LINE('',#93775,#8303) ;
#5090=LINE('',#93778,#8304) ;
#5091=LINE('',#93787,#8305) ;
#5092=LINE('',#93795,#8306) ;
#5093=LINE('',#93801,#8307) ;
#5094=LINE('',#93804,#8308) ;
#5095=LINE('',#93808,#8309) ;
#5096=LINE('',#93812,#8310) ;
#5097=LINE('',#93816,#8311) ;
#5098=LINE('',#93844,#8312) ;
#5099=LINE('',#93858,#8313) ;
#5100=LINE('',#93860,#8314) ;
#5101=LINE('',#93862,#8315) ;
#5102=LINE('',#93863,#8316) ;
#5103=LINE('',#93866,#8317) ;
#5104=LINE('',#93868,#8318) ;
#5105=LINE('',#93870,#8319) ;
#5106=LINE('',#93889,#8320) ;
#5107=LINE('',#93902,#8321) ;
#5108=LINE('',#93905,#8322) ;
#5109=LINE('',#93909,#8323) ;
#5110=LINE('',#93911,#8324) ;
#5111=LINE('',#93915,#8325) ;
#5112=LINE('',#93916,#8326) ;
#5113=LINE('',#93918,#8327) ;
#5114=LINE('',#93924,#8328) ;
#5115=LINE('',#93928,#8329) ;
#5116=LINE('',#93930,#8330) ;
#5117=LINE('',#93932,#8331) ;
#5118=LINE('',#93933,#8332) ;
#5119=LINE('',#93935,#8333) ;
#5120=LINE('',#93936,#8334) ;
#5121=LINE('',#94015,#8335) ;
#5122=LINE('',#94018,#8336) ;
#5123=LINE('',#94087,#8337) ;
#5124=LINE('',#94088,#8338) ;
#5125=LINE('',#94093,#8339) ;
#5126=LINE('',#94094,#8340) ;
#5127=LINE('',#94096,#8341) ;
#5128=LINE('',#94097,#8342) ;
#5129=LINE('',#94102,#8343) ;
#5130=LINE('',#94103,#8344) ;
#5131=LINE('',#94107,#8345) ;
#5132=LINE('',#94108,#8346) ;
#5133=LINE('',#94158,#8347) ;
#5134=LINE('',#94161,#8348) ;
#5135=LINE('',#94163,#8349) ;
#5136=LINE('',#94165,#8350) ;
#5137=LINE('',#94168,#8351) ;
#5138=LINE('',#94171,#8352) ;
#5139=LINE('',#94178,#8353) ;
#5140=LINE('',#94195,#8354) ;
#5141=LINE('',#94200,#8355) ;
#5142=LINE('',#94204,#8356) ;
#5143=LINE('',#94207,#8357) ;
#5144=LINE('',#94209,#8358) ;
#5145=LINE('',#94211,#8359) ;
#5146=LINE('',#94213,#8360) ;
#5147=LINE('',#94214,#8361) ;
#5148=LINE('',#94217,#8362) ;
#5149=LINE('',#94218,#8363) ;
#5150=LINE('',#94220,#8364) ;
#5151=LINE('',#94221,#8365) ;
#5152=LINE('',#94430,#8366) ;
#5153=LINE('',#94438,#8367) ;
#5154=LINE('',#94445,#8368) ;
#5155=LINE('',#94448,#8369) ;
#5156=LINE('',#94485,#8370) ;
#5157=LINE('',#94486,#8371) ;
#5158=LINE('',#94561,#8372) ;
#5159=LINE('',#94565,#8373) ;
#5160=LINE('',#94567,#8374) ;
#5161=LINE('',#94569,#8375) ;
#5162=LINE('',#94572,#8376) ;
#5163=LINE('',#94573,#8377) ;
#5164=LINE('',#94576,#8378) ;
#5165=LINE('',#94580,#8379) ;
#5166=LINE('',#94582,#8380) ;
#5167=LINE('',#94584,#8381) ;
#5168=LINE('',#94588,#8382) ;
#5169=LINE('',#94590,#8383) ;
#5170=LINE('',#94592,#8384) ;
#5171=LINE('',#94594,#8385) ;
#5172=LINE('',#94595,#8386) ;
#5173=LINE('',#94598,#8387) ;
#5174=LINE('',#94600,#8388) ;
#5175=LINE('',#94604,#8389) ;
#5176=LINE('',#94606,#8390) ;
#5177=LINE('',#94608,#8391) ;
#5178=LINE('',#94610,#8392) ;
#5179=LINE('',#94612,#8393) ;
#5180=LINE('',#94614,#8394) ;
#5181=LINE('',#94617,#8395) ;
#5182=LINE('',#94620,#8396) ;
#5183=LINE('',#94622,#8397) ;
#5184=LINE('',#94624,#8398) ;
#5185=LINE('',#94625,#8399) ;
#5186=LINE('',#94628,#8400) ;
#5187=LINE('',#94632,#8401) ;
#5188=LINE('',#94672,#8402) ;
#5189=LINE('',#94686,#8403) ;
#5190=LINE('',#94734,#8404) ;
#5191=LINE('',#94778,#8405) ;
#5192=LINE('',#94780,#8406) ;
#5193=LINE('',#94783,#8407) ;
#5194=LINE('',#94787,#8408) ;
#5195=LINE('',#94788,#8409) ;
#5196=LINE('',#94790,#8410) ;
#5197=LINE('',#94791,#8411) ;
#5198=LINE('',#94798,#8412) ;
#5199=LINE('',#94805,#8413) ;
#5200=LINE('',#94808,#8414) ;
#5201=LINE('',#94826,#8415) ;
#5202=LINE('',#94828,#8416) ;
#5203=LINE('',#94833,#8417) ;
#5204=LINE('',#94835,#8418) ;
#5205=LINE('',#94837,#8419) ;
#5206=LINE('',#94838,#8420) ;
#5207=LINE('',#94839,#8421) ;
#5208=LINE('',#94843,#8422) ;
#5209=LINE('',#94846,#8423) ;
#5210=LINE('',#94848,#8424) ;
#5211=LINE('',#94849,#8425) ;
#5212=LINE('',#94891,#8426) ;
#5213=LINE('',#94895,#8427) ;
#5214=LINE('',#94899,#8428) ;
#5215=LINE('',#94900,#8429) ;
#5216=LINE('',#94903,#8430) ;
#5217=LINE('',#94904,#8431) ;
#5218=LINE('',#94906,#8432) ;
#5219=LINE('',#94909,#8433) ;
#5220=LINE('',#94911,#8434) ;
#5221=LINE('',#94915,#8435) ;
#5222=LINE('',#94918,#8436) ;
#5223=LINE('',#94919,#8437) ;
#5224=LINE('',#94929,#8438) ;
#5225=LINE('',#94932,#8439) ;
#5226=LINE('',#94934,#8440) ;
#5227=LINE('',#94935,#8441) ;
#5228=LINE('',#94938,#8442) ;
#5229=LINE('',#94940,#8443) ;
#5230=LINE('',#94941,#8444) ;
#5231=LINE('',#94943,#8445) ;
#5232=LINE('',#94944,#8446) ;
#5233=LINE('',#94946,#8447) ;
#5234=LINE('',#94948,#8448) ;
#5235=LINE('',#94950,#8449) ;
#5236=LINE('',#94955,#8450) ;
#5237=LINE('',#94972,#8451) ;
#5238=LINE('',#95158,#8452) ;
#5239=LINE('',#95174,#8453) ;
#5240=LINE('',#95270,#8454) ;
#5241=LINE('',#95272,#8455) ;
#5242=LINE('',#95276,#8456) ;
#5243=LINE('',#95278,#8457) ;
#5244=LINE('',#95281,#8458) ;
#5245=LINE('',#95282,#8459) ;
#5246=LINE('',#95285,#8460) ;
#5247=LINE('',#95287,#8461) ;
#5248=LINE('',#95288,#8462) ;
#5249=LINE('',#95291,#8463) ;
#5250=LINE('',#95292,#8464) ;
#5251=LINE('',#95295,#8465) ;
#5252=LINE('',#95296,#8466) ;
#5253=LINE('',#95299,#8467) ;
#5254=LINE('',#95300,#8468) ;
#5255=LINE('',#95538,#8469) ;
#5256=LINE('',#95541,#8470) ;
#5257=LINE('',#95544,#8471) ;
#5258=LINE('',#95547,#8472) ;
#5259=LINE('',#95550,#8473) ;
#5260=LINE('',#95552,#8474) ;
#5261=LINE('',#95556,#8475) ;
#5262=LINE('',#95558,#8476) ;
#5263=LINE('',#95783,#8477) ;
#5264=LINE('',#95784,#8478) ;
#5265=LINE('',#95787,#8479) ;
#5266=LINE('',#95789,#8480) ;
#5267=LINE('',#95790,#8481) ;
#5268=LINE('',#95812,#8482) ;
#5269=LINE('',#95966,#8483) ;
#5270=LINE('',#95967,#8484) ;
#5271=LINE('',#95989,#8485) ;
#5272=LINE('',#96079,#8486) ;
#5273=LINE('',#96083,#8487) ;
#5274=LINE('',#96087,#8488) ;
#5275=LINE('',#96090,#8489) ;
#5276=LINE('',#96093,#8490) ;
#5277=LINE('',#96096,#8491) ;
#5278=LINE('',#96099,#8492) ;
#5279=LINE('',#96101,#8493) ;
#5280=LINE('',#96105,#8494) ;
#5281=LINE('',#96107,#8495) ;
#5282=LINE('',#96111,#8496) ;
#5283=LINE('',#96113,#8497) ;
#5284=LINE('',#96116,#8498) ;
#5285=LINE('',#96117,#8499) ;
#5286=LINE('',#96120,#8500) ;
#5287=LINE('',#96122,#8501) ;
#5288=LINE('',#96123,#8502) ;
#5289=LINE('',#96126,#8503) ;
#5290=LINE('',#96127,#8504) ;
#5291=LINE('',#96130,#8505) ;
#5292=LINE('',#96131,#8506) ;
#5293=LINE('',#96134,#8507) ;
#5294=LINE('',#96135,#8508) ;
#5295=LINE('',#96140,#8509) ;
#5296=LINE('',#96144,#8510) ;
#5297=LINE('',#96148,#8511) ;
#5298=LINE('',#96150,#8512) ;
#5299=LINE('',#96154,#8513) ;
#5300=LINE('',#96156,#8514) ;
#5301=LINE('',#96159,#8515) ;
#5302=LINE('',#96160,#8516) ;
#5303=LINE('',#96163,#8517) ;
#5304=LINE('',#96165,#8518) ;
#5305=LINE('',#96166,#8519) ;
#5306=LINE('',#96169,#8520) ;
#5307=LINE('',#96170,#8521) ;
#5308=LINE('',#96175,#8522) ;
#5309=LINE('',#96179,#8523) ;
#5310=LINE('',#96183,#8524) ;
#5311=LINE('',#96186,#8525) ;
#5312=LINE('',#96189,#8526) ;
#5313=LINE('',#96192,#8527) ;
#5314=LINE('',#96195,#8528) ;
#5315=LINE('',#96197,#8529) ;
#5316=LINE('',#96201,#8530) ;
#5317=LINE('',#96203,#8531) ;
#5318=LINE('',#96207,#8532) ;
#5319=LINE('',#96209,#8533) ;
#5320=LINE('',#96212,#8534) ;
#5321=LINE('',#96213,#8535) ;
#5322=LINE('',#96216,#8536) ;
#5323=LINE('',#96218,#8537) ;
#5324=LINE('',#96219,#8538) ;
#5325=LINE('',#96222,#8539) ;
#5326=LINE('',#96223,#8540) ;
#5327=LINE('',#96226,#8541) ;
#5328=LINE('',#96227,#8542) ;
#5329=LINE('',#96230,#8543) ;
#5330=LINE('',#96231,#8544) ;
#5331=LINE('',#96236,#8545) ;
#5332=LINE('',#96240,#8546) ;
#5333=LINE('',#96244,#8547) ;
#5334=LINE('',#96246,#8548) ;
#5335=LINE('',#96250,#8549) ;
#5336=LINE('',#96252,#8550) ;
#5337=LINE('',#96255,#8551) ;
#5338=LINE('',#96256,#8552) ;
#5339=LINE('',#96259,#8553) ;
#5340=LINE('',#96261,#8554) ;
#5341=LINE('',#96262,#8555) ;
#5342=LINE('',#96265,#8556) ;
#5343=LINE('',#96266,#8557) ;
#5344=LINE('',#96271,#8558) ;
#5345=LINE('',#96275,#8559) ;
#5346=LINE('',#96279,#8560) ;
#5347=LINE('',#96282,#8561) ;
#5348=LINE('',#96285,#8562) ;
#5349=LINE('',#96288,#8563) ;
#5350=LINE('',#96297,#8564) ;
#5351=LINE('',#96299,#8565) ;
#5352=LINE('',#96303,#8566) ;
#5353=LINE('',#96305,#8567) ;
#5354=LINE('',#96309,#8568) ;
#5355=LINE('',#96312,#8569) ;
#5356=LINE('',#96321,#8570) ;
#5357=LINE('',#96323,#8571) ;
#5358=LINE('',#96327,#8572) ;
#5359=LINE('',#96329,#8573) ;
#5360=LINE('',#96332,#8574) ;
#5361=LINE('',#96333,#8575) ;
#5362=LINE('',#96336,#8576) ;
#5363=LINE('',#96338,#8577) ;
#5364=LINE('',#96339,#8578) ;
#5365=LINE('',#96342,#8579) ;
#5366=LINE('',#96346,#8580) ;
#5367=LINE('',#96347,#8581) ;
#5368=LINE('',#96350,#8582) ;
#5369=LINE('',#96351,#8583) ;
#5370=LINE('',#96354,#8584) ;
#5371=LINE('',#96355,#8585) ;
#5372=LINE('',#96358,#8586) ;
#5373=LINE('',#96359,#8587) ;
#5374=LINE('',#96364,#8588) ;
#5375=LINE('',#96368,#8589) ;
#5376=LINE('',#96372,#8590) ;
#5377=LINE('',#96375,#8591) ;
#5378=LINE('',#96384,#8592) ;
#5379=LINE('',#96386,#8593) ;
#5380=LINE('',#96390,#8594) ;
#5381=LINE('',#96393,#8595) ;
#5382=LINE('',#96396,#8596) ;
#5383=LINE('',#96399,#8597) ;
#5384=LINE('',#96408,#8598) ;
#5385=LINE('',#96410,#8599) ;
#5386=LINE('',#96414,#8600) ;
#5387=LINE('',#96416,#8601) ;
#5388=LINE('',#96420,#8602) ;
#5389=LINE('',#96422,#8603) ;
#5390=LINE('',#96425,#8604) ;
#5391=LINE('',#96426,#8605) ;
#5392=LINE('',#96429,#8606) ;
#5393=LINE('',#96432,#8607) ;
#5394=LINE('',#96435,#8608) ;
#5395=LINE('',#96436,#8609) ;
#5396=LINE('',#96439,#8610) ;
#5397=LINE('',#96440,#8611) ;
#5398=LINE('',#96443,#8612) ;
#5399=LINE('',#96444,#8613) ;
#5400=LINE('',#96447,#8614) ;
#5401=LINE('',#96448,#8615) ;
#5402=LINE('',#96451,#8616) ;
#5403=LINE('',#96452,#8617) ;
#5404=LINE('',#96759,#8618) ;
#5405=LINE('',#96901,#8619) ;
#5406=LINE('',#96903,#8620) ;
#5407=LINE('',#97054,#8621) ;
#5408=LINE('',#97057,#8622) ;
#5409=LINE('',#97073,#8623) ;
#5410=LINE('',#97189,#8624) ;
#5411=LINE('',#97191,#8625) ;
#5412=LINE('',#97195,#8626) ;
#5413=LINE('',#97198,#8627) ;
#5414=LINE('',#97202,#8628) ;
#5415=LINE('',#97205,#8629) ;
#5416=LINE('',#97208,#8630) ;
#5417=LINE('',#97212,#8631) ;
#5418=LINE('',#97216,#8632) ;
#5419=LINE('',#97220,#8633) ;
#5420=LINE('',#97223,#8634) ;
#5421=LINE('',#97224,#8635) ;
#5422=LINE('',#97226,#8636) ;
#5423=LINE('',#97228,#8637) ;
#5424=LINE('',#97233,#8638) ;
#5425=LINE('',#97237,#8639) ;
#5426=LINE('',#97242,#8640) ;
#5427=LINE('',#97245,#8641) ;
#5428=LINE('',#97297,#8642) ;
#5429=LINE('',#97301,#8643) ;
#5430=LINE('',#97303,#8644) ;
#5431=LINE('',#97305,#8645) ;
#5432=LINE('',#97306,#8646) ;
#5433=LINE('',#97309,#8647) ;
#5434=LINE('',#97311,#8648) ;
#5435=LINE('',#97313,#8649) ;
#5436=LINE('',#97315,#8650) ;
#5437=LINE('',#97317,#8651) ;
#5438=LINE('',#97319,#8652) ;
#5439=LINE('',#97320,#8653) ;
#5440=LINE('',#97328,#8654) ;
#5441=LINE('',#97331,#8655) ;
#5442=LINE('',#97333,#8656) ;
#5443=LINE('',#97338,#8657) ;
#5444=LINE('',#97342,#8658) ;
#5445=LINE('',#97352,#8659) ;
#5446=LINE('',#97354,#8660) ;
#5447=LINE('',#97356,#8661) ;
#5448=LINE('',#97363,#8662) ;
#5449=LINE('',#97367,#8663) ;
#5450=LINE('',#97371,#8664) ;
#5451=LINE('',#97376,#8665) ;
#5452=LINE('',#97396,#8666) ;
#5453=LINE('',#97398,#8667) ;
#5454=LINE('',#97399,#8668) ;
#5455=LINE('',#97401,#8669) ;
#5456=LINE('',#97403,#8670) ;
#5457=LINE('',#97409,#8671) ;
#5458=LINE('',#97413,#8672) ;
#5459=LINE('',#97429,#8673) ;
#5460=LINE('',#97431,#8674) ;
#5461=LINE('',#97437,#8675) ;
#5462=LINE('',#97439,#8676) ;
#5463=LINE('',#97441,#8677) ;
#5464=LINE('',#97443,#8678) ;
#5465=LINE('',#97447,#8679) ;
#5466=LINE('',#97454,#8680) ;
#5467=LINE('',#97455,#8681) ;
#5468=LINE('',#97458,#8682) ;
#5469=LINE('',#97462,#8683) ;
#5470=LINE('',#97466,#8684) ;
#5471=LINE('',#97467,#8685) ;
#5472=LINE('',#97469,#8686) ;
#5473=LINE('',#97472,#8687) ;
#5474=LINE('',#97476,#8688) ;
#5475=LINE('',#97477,#8689) ;
#5476=LINE('',#97480,#8690) ;
#5477=LINE('',#97484,#8691) ;
#5478=LINE('',#97485,#8692) ;
#5479=LINE('',#97488,#8693) ;
#5480=LINE('',#97489,#8694) ;
#5481=LINE('',#97492,#8695) ;
#5482=LINE('',#97493,#8696) ;
#5483=LINE('',#97496,#8697) ;
#5484=LINE('',#97500,#8698) ;
#5485=LINE('',#97504,#8699) ;
#5486=LINE('',#97505,#8700) ;
#5487=LINE('',#97507,#8701) ;
#5488=LINE('',#97511,#8702) ;
#5489=LINE('',#97513,#8703) ;
#5490=LINE('',#97514,#8704) ;
#5491=LINE('',#97517,#8705) ;
#5492=LINE('',#97518,#8706) ;
#5493=LINE('',#97521,#8707) ;
#5494=LINE('',#97522,#8708) ;
#5495=LINE('',#97524,#8709) ;
#5496=LINE('',#97527,#8710) ;
#5497=LINE('',#97529,#8711) ;
#5498=LINE('',#97531,#8712) ;
#5499=LINE('',#97532,#8713) ;
#5500=LINE('',#97535,#8714) ;
#5501=LINE('',#97538,#8715) ;
#5502=LINE('',#97540,#8716) ;
#5503=LINE('',#97542,#8717) ;
#5504=LINE('',#97546,#8718) ;
#5505=LINE('',#97551,#8719) ;
#5506=LINE('',#97553,#8720) ;
#5507=LINE('',#97554,#8721) ;
#5508=LINE('',#97555,#8722) ;
#5509=LINE('',#97559,#8723) ;
#5510=LINE('',#97562,#8724) ;
#5511=LINE('',#97564,#8725) ;
#5512=LINE('',#97567,#8726) ;
#5513=LINE('',#97590,#8727) ;
#5514=LINE('',#97697,#8728) ;
#5515=LINE('',#97735,#8729) ;
#5516=LINE('',#97765,#8730) ;
#5517=LINE('',#97818,#8731) ;
#5518=LINE('',#97902,#8732) ;
#5519=LINE('',#97934,#8733) ;
#5520=LINE('',#97989,#8734) ;
#5521=LINE('',#98004,#8735) ;
#5522=LINE('',#98009,#8736) ;
#5523=LINE('',#98018,#8737) ;
#5524=LINE('',#98021,#8738) ;
#5525=LINE('',#98083,#8739) ;
#5526=LINE('',#98084,#8740) ;
#5527=LINE('',#98087,#8741) ;
#5528=LINE('',#98090,#8742) ;
#5529=LINE('',#98117,#8743) ;
#5530=LINE('',#98118,#8744) ;
#5531=LINE('',#98120,#8745) ;
#5532=LINE('',#98121,#8746) ;
#5533=LINE('',#98123,#8747) ;
#5534=LINE('',#98125,#8748) ;
#5535=LINE('',#98127,#8749) ;
#5536=LINE('',#98133,#8750) ;
#5537=LINE('',#98134,#8751) ;
#5538=LINE('',#98136,#8752) ;
#5539=LINE('',#98137,#8753) ;
#5540=LINE('',#98140,#8754) ;
#5541=LINE('',#98142,#8755) ;
#5542=LINE('',#98143,#8756) ;
#5543=LINE('',#98147,#8757) ;
#5544=LINE('',#98150,#8758) ;
#5545=LINE('',#98151,#8759) ;
#5546=LINE('',#98154,#8760) ;
#5547=LINE('',#98155,#8761) ;
#5548=LINE('',#98159,#8762) ;
#5549=LINE('',#98162,#8763) ;
#5550=LINE('',#98163,#8764) ;
#5551=LINE('',#98167,#8765) ;
#5552=LINE('',#98170,#8766) ;
#5553=LINE('',#98171,#8767) ;
#5554=LINE('',#98174,#8768) ;
#5555=LINE('',#98175,#8769) ;
#5556=LINE('',#98189,#8770) ;
#5557=LINE('',#98198,#8771) ;
#5558=LINE('',#98199,#8772) ;
#5559=LINE('',#98219,#8773) ;
#5560=LINE('',#98221,#8774) ;
#5561=LINE('',#98227,#8775) ;
#5562=LINE('',#98231,#8776) ;
#5563=LINE('',#98233,#8777) ;
#5564=LINE('',#98234,#8778) ;
#5565=LINE('',#98238,#8779) ;
#5566=LINE('',#98241,#8780) ;
#5567=LINE('',#98242,#8781) ;
#5568=LINE('',#98246,#8782) ;
#5569=LINE('',#98249,#8783) ;
#5570=LINE('',#98250,#8784) ;
#5571=LINE('',#98255,#8785) ;
#5572=LINE('',#98256,#8786) ;
#5573=LINE('',#98259,#8787) ;
#5574=LINE('',#98260,#8788) ;
#5575=LINE('',#98264,#8789) ;
#5576=LINE('',#98267,#8790) ;
#5577=LINE('',#98268,#8791) ;
#5578=LINE('',#98271,#8792) ;
#5579=LINE('',#98272,#8793) ;
#5580=LINE('',#98276,#8794) ;
#5581=LINE('',#98279,#8795) ;
#5582=LINE('',#98280,#8796) ;
#5583=LINE('',#98283,#8797) ;
#5584=LINE('',#98288,#8798) ;
#5585=LINE('',#98289,#8799) ;
#5586=LINE('',#98290,#8800) ;
#5587=LINE('',#98294,#8801) ;
#5588=LINE('',#98297,#8802) ;
#5589=LINE('',#98298,#8803) ;
#5590=LINE('',#98302,#8804) ;
#5591=LINE('',#98305,#8805) ;
#5592=LINE('',#98306,#8806) ;
#5593=LINE('',#98326,#8807) ;
#5594=LINE('',#98331,#8808) ;
#5595=LINE('',#98332,#8809) ;
#5596=LINE('',#98335,#8810) ;
#5597=LINE('',#98336,#8811) ;
#5598=LINE('',#98340,#8812) ;
#5599=LINE('',#98343,#8813) ;
#5600=LINE('',#98344,#8814) ;
#5601=LINE('',#98346,#8815) ;
#5602=LINE('',#98349,#8816) ;
#5603=LINE('',#98350,#8817) ;
#5604=LINE('',#98355,#8818) ;
#5605=LINE('',#98356,#8819) ;
#5606=LINE('',#98359,#8820) ;
#5607=LINE('',#98360,#8821) ;
#5608=LINE('',#98361,#8822) ;
#5609=LINE('',#98365,#8823) ;
#5610=LINE('',#98368,#8824) ;
#5611=LINE('',#98369,#8825) ;
#5612=LINE('',#98376,#8826) ;
#5613=LINE('',#98377,#8827) ;
#5614=LINE('',#98380,#8828) ;
#5615=LINE('',#98381,#8829) ;
#5616=LINE('',#98385,#8830) ;
#5617=LINE('',#98388,#8831) ;
#5618=LINE('',#98389,#8832) ;
#5619=LINE('',#98392,#8833) ;
#5620=LINE('',#98393,#8834) ;
#5621=LINE('',#98397,#8835) ;
#5622=LINE('',#98400,#8836) ;
#5623=LINE('',#98401,#8837) ;
#5624=LINE('',#98405,#8838) ;
#5625=LINE('',#98408,#8839) ;
#5626=LINE('',#98409,#8840) ;
#5627=LINE('',#98412,#8841) ;
#5628=LINE('',#98413,#8842) ;
#5629=LINE('',#98417,#8843) ;
#5630=LINE('',#98420,#8844) ;
#5631=LINE('',#98421,#8845) ;
#5632=LINE('',#98425,#8846) ;
#5633=LINE('',#98427,#8847) ;
#5634=LINE('',#98431,#8848) ;
#5635=LINE('',#98432,#8849) ;
#5636=LINE('',#98452,#8850) ;
#5637=LINE('',#98455,#8851) ;
#5638=LINE('',#98456,#8852) ;
#5639=LINE('',#98460,#8853) ;
#5640=LINE('',#98463,#8854) ;
#5641=LINE('',#98464,#8855) ;
#5642=LINE('',#98487,#8856) ;
#5643=LINE('',#98490,#8857) ;
#5644=LINE('',#98491,#8858) ;
#5645=LINE('',#98494,#8859) ;
#5646=LINE('',#98495,#8860) ;
#5647=LINE('',#98499,#8861) ;
#5648=LINE('',#98502,#8862) ;
#5649=LINE('',#98503,#8863) ;
#5650=LINE('',#98507,#8864) ;
#5651=LINE('',#98509,#8865) ;
#5652=LINE('',#98514,#8866) ;
#5653=LINE('',#98517,#8867) ;
#5654=LINE('',#98518,#8868) ;
#5655=LINE('',#98521,#8869) ;
#5656=LINE('',#98522,#8870) ;
#5657=LINE('',#98525,#8871) ;
#5658=LINE('',#98526,#8872) ;
#5659=LINE('',#98529,#8873) ;
#5660=LINE('',#98530,#8874) ;
#5661=LINE('',#98533,#8875) ;
#5662=LINE('',#98534,#8876) ;
#5663=LINE('',#98538,#8877) ;
#5664=LINE('',#98542,#8878) ;
#5665=LINE('',#98546,#8879) ;
#5666=LINE('',#98549,#8880) ;
#5667=LINE('',#98550,#8881) ;
#5668=LINE('',#98553,#8882) ;
#5669=LINE('',#98554,#8883) ;
#5670=LINE('',#98558,#8884) ;
#5671=LINE('',#98561,#8885) ;
#5672=LINE('',#98562,#8886) ;
#5673=LINE('',#98566,#8887) ;
#5674=LINE('',#98568,#8888) ;
#5675=LINE('',#98573,#8889) ;
#5676=LINE('',#98576,#8890) ;
#5677=LINE('',#98577,#8891) ;
#5678=LINE('',#98581,#8892) ;
#5679=LINE('',#98584,#8893) ;
#5680=LINE('',#98585,#8894) ;
#5681=LINE('',#98589,#8895) ;
#5682=LINE('',#98591,#8896) ;
#5683=LINE('',#98597,#8897) ;
#5684=LINE('',#98600,#8898) ;
#5685=LINE('',#98601,#8899) ;
#5686=LINE('',#98604,#8900) ;
#5687=LINE('',#98605,#8901) ;
#5688=LINE('',#98607,#8902) ;
#5689=LINE('',#98608,#8903) ;
#5690=LINE('',#98610,#8904) ;
#5691=LINE('',#98612,#8905) ;
#5692=LINE('',#98613,#8906) ;
#5693=LINE('',#98616,#8907) ;
#5694=LINE('',#98618,#8908) ;
#5695=LINE('',#98620,#8909) ;
#5696=LINE('',#98622,#8910) ;
#5697=LINE('',#98624,#8911) ;
#5698=LINE('',#98631,#8912) ;
#5699=LINE('',#98634,#8913) ;
#5700=LINE('',#98636,#8914) ;
#5701=LINE('',#98639,#8915) ;
#5702=LINE('',#98642,#8916) ;
#5703=LINE('',#98645,#8917) ;
#5704=LINE('',#98649,#8918) ;
#5705=LINE('',#98652,#8919) ;
#5706=LINE('',#98654,#8920) ;
#5707=LINE('',#98656,#8921) ;
#5708=LINE('',#98658,#8922) ;
#5709=LINE('',#98660,#8923) ;
#5710=LINE('',#98663,#8924) ;
#5711=LINE('',#98666,#8925) ;
#5712=LINE('',#98667,#8926) ;
#7806=VECTOR('',#63103,10.) ;
#7807=VECTOR('',#63104,10.) ;
#7808=VECTOR('',#63105,10.) ;
#7809=VECTOR('',#63106,10.) ;
#7810=VECTOR('',#63107,10.) ;
#7811=VECTOR('',#63108,10.) ;
#7812=VECTOR('',#63109,10.) ;
#7813=VECTOR('',#63110,10.) ;
#7814=VECTOR('',#63111,10.) ;
#7815=VECTOR('',#63114,10.) ;
#7816=VECTOR('',#63115,10.) ;
#7817=VECTOR('',#63116,10.) ;
#7818=VECTOR('',#63119,10.) ;
#7819=VECTOR('',#63120,10.) ;
#7820=VECTOR('',#63123,10.) ;
#7821=VECTOR('',#63124,10.) ;
#7822=VECTOR('',#63125,10.) ;
#7823=VECTOR('',#63126,10.) ;
#7824=VECTOR('',#63129,10.) ;
#7825=VECTOR('',#63130,10.) ;
#7826=VECTOR('',#63131,10.) ;
#7827=VECTOR('',#63132,10.) ;
#7828=VECTOR('',#63133,10.) ;
#7829=VECTOR('',#63134,10.) ;
#7830=VECTOR('',#63135,10.) ;
#7831=VECTOR('',#63138,10.) ;
#7832=VECTOR('',#63139,10.) ;
#7833=VECTOR('',#63140,10.) ;
#7834=VECTOR('',#63143,10.) ;
#7835=VECTOR('',#63144,10.) ;
#7836=VECTOR('',#63145,10.) ;
#7837=VECTOR('',#63148,10.) ;
#7838=VECTOR('',#63149,10.) ;
#7839=VECTOR('',#63150,9.99999999999999) ;
#7840=VECTOR('',#63151,10.) ;
#7841=VECTOR('',#63152,10.) ;
#7842=VECTOR('',#63153,10.) ;
#7843=VECTOR('',#63154,10.) ;
#7844=VECTOR('',#63155,10.) ;
#7845=VECTOR('',#63156,10.) ;
#7846=VECTOR('',#63157,10.) ;
#7847=VECTOR('',#63160,10.) ;
#7848=VECTOR('',#63161,10.) ;
#7849=VECTOR('',#63162,10.) ;
#7850=VECTOR('',#63165,10.) ;
#7851=VECTOR('',#63166,10.) ;
#7852=VECTOR('',#63167,10.) ;
#7853=VECTOR('',#63170,10.) ;
#7854=VECTOR('',#63171,10.) ;
#7855=VECTOR('',#63176,10.) ;
#7856=VECTOR('',#63177,10.) ;
#7857=VECTOR('',#63180,10.) ;
#7858=VECTOR('',#63183,10.) ;
#7859=VECTOR('',#63186,10.) ;
#7860=VECTOR('',#63191,10.) ;
#7861=VECTOR('',#63194,10.) ;
#7862=VECTOR('',#63197,10.) ;
#7863=VECTOR('',#63200,10.) ;
#7864=VECTOR('',#63203,10.) ;
#7865=VECTOR('',#63206,10.) ;
#7866=VECTOR('',#63207,10.) ;
#7867=VECTOR('',#63210,10.) ;
#7868=VECTOR('',#63213,10.) ;
#7869=VECTOR('',#63214,10.) ;
#7870=VECTOR('',#63227,10.) ;
#7871=VECTOR('',#63228,10.) ;
#7872=VECTOR('',#63239,10.) ;
#7873=VECTOR('',#63240,10.) ;
#7874=VECTOR('',#63245,10.) ;
#7875=VECTOR('',#63246,10.) ;
#7876=VECTOR('',#63247,10.) ;
#7877=VECTOR('',#63248,10.) ;
#7878=VECTOR('',#63249,10.) ;
#7879=VECTOR('',#63252,10.) ;
#7880=VECTOR('',#63257,10.) ;
#7881=VECTOR('',#63258,10.) ;
#7882=VECTOR('',#63269,10.) ;
#7883=VECTOR('',#63270,10.) ;
#7884=VECTOR('',#63281,10.) ;
#7885=VECTOR('',#63282,10.) ;
#7886=VECTOR('',#63291,10.) ;
#7887=VECTOR('',#63292,10.) ;
#7888=VECTOR('',#63293,10.) ;
#7889=VECTOR('',#63296,10.) ;
#7890=VECTOR('',#63301,10.) ;
#7891=VECTOR('',#63302,10.) ;
#7892=VECTOR('',#63303,10.) ;
#7893=VECTOR('',#63308,10.) ;
#7894=VECTOR('',#63313,10.) ;
#7895=VECTOR('',#63316,10.) ;
#7896=VECTOR('',#63317,10.) ;
#7897=VECTOR('',#63318,10.) ;
#7898=VECTOR('',#63319,10.) ;
#7899=VECTOR('',#63322,10.) ;
#7900=VECTOR('',#63325,10.) ;
#7901=VECTOR('',#63340,10.) ;
#7902=VECTOR('',#63341,10.) ;
#7903=VECTOR('',#63350,10.) ;
#7904=VECTOR('',#63353,10.) ;
#7905=VECTOR('',#63356,10.) ;
#7906=VECTOR('',#63357,10.) ;
#7907=VECTOR('',#63362,10.) ;
#7908=VECTOR('',#63379,10.) ;
#7909=VECTOR('',#63380,10.) ;
#7910=VECTOR('',#63389,10.) ;
#7911=VECTOR('',#63390,10.) ;
#7912=VECTOR('',#63393,10.) ;
#7913=VECTOR('',#63396,10.) ;
#7914=VECTOR('',#63397,10.) ;
#7915=VECTOR('',#63398,10.) ;
#7916=VECTOR('',#63399,10.) ;
#7917=VECTOR('',#63402,10.) ;
#7918=VECTOR('',#63403,10.) ;
#7919=VECTOR('',#63406,10.) ;
#7920=VECTOR('',#63411,10.) ;
#7921=VECTOR('',#63414,10.) ;
#7922=VECTOR('',#63423,10.) ;
#7923=VECTOR('',#63426,10.) ;
#7924=VECTOR('',#63429,10.) ;
#7925=VECTOR('',#63430,10.) ;
#7926=VECTOR('',#63433,10.) ;
#7927=VECTOR('',#63436,10.) ;
#7928=VECTOR('',#63437,10.) ;
#7929=VECTOR('',#63438,10.) ;
#7930=VECTOR('',#63439,10.) ;
#7931=VECTOR('',#63442,10.) ;
#7932=VECTOR('',#63445,10.) ;
#7933=VECTOR('',#63448,10.) ;
#7934=VECTOR('',#63453,10.) ;
#7935=VECTOR('',#63458,10.) ;
#7936=VECTOR('',#63461,10.) ;
#7937=VECTOR('',#63464,10.) ;
#7938=VECTOR('',#63467,10.) ;
#7939=VECTOR('',#63478,10.) ;
#7940=VECTOR('',#63479,10.) ;
#7941=VECTOR('',#63482,10.) ;
#7942=VECTOR('',#63485,10.) ;
#7943=VECTOR('',#63486,10.) ;
#7944=VECTOR('',#63489,10.) ;
#7945=VECTOR('',#63494,10.) ;
#7946=VECTOR('',#63495,10.) ;
#7947=VECTOR('',#63496,10.) ;
#7948=VECTOR('',#63497,10.) ;
#7949=VECTOR('',#63498,10.) ;
#7950=VECTOR('',#63511,10.) ;
#7951=VECTOR('',#63514,10.) ;
#7952=VECTOR('',#63517,10.) ;
#7953=VECTOR('',#63520,10.) ;
#7954=VECTOR('',#63521,10.) ;
#7955=VECTOR('',#63522,10.) ;
#7956=VECTOR('',#63541,10.) ;
#7957=VECTOR('',#63558,10.) ;
#7958=VECTOR('',#63571,10.) ;
#7959=VECTOR('',#63572,10.) ;
#7960=VECTOR('',#63583,10.) ;
#7961=VECTOR('',#63586,10.) ;
#7962=VECTOR('',#63587,10.) ;
#7963=VECTOR('',#63588,10.) ;
#7964=VECTOR('',#63589,10.) ;
#7965=VECTOR('',#63590,10.) ;
#7966=VECTOR('',#63591,10.) ;
#7967=VECTOR('',#63594,10.) ;
#7968=VECTOR('',#63599,10.) ;
#7969=VECTOR('',#63602,10.) ;
#7970=VECTOR('',#63603,10.) ;
#7971=VECTOR('',#63604,10.) ;
#7972=VECTOR('',#63621,10.) ;
#7973=VECTOR('',#63622,10.) ;
#7974=VECTOR('',#63635,10.) ;
#7975=VECTOR('',#63636,10.) ;
#7976=VECTOR('',#63657,10.) ;
#7977=VECTOR('',#63658,10.) ;
#7978=VECTOR('',#63669,10.) ;
#7979=VECTOR('',#63670,10.) ;
#7980=VECTOR('',#63675,10.) ;
#7981=VECTOR('',#63676,10.) ;
#7982=VECTOR('',#63685,10.) ;
#7983=VECTOR('',#63688,10.) ;
#7984=VECTOR('',#63691,10.) ;
#7985=VECTOR('',#63692,10.) ;
#7986=VECTOR('',#63693,10.) ;
#7987=VECTOR('',#63702,10.) ;
#7988=VECTOR('',#63707,10.) ;
#7989=VECTOR('',#63708,10.) ;
#7990=VECTOR('',#63713,10.) ;
#7991=VECTOR('',#63716,10.) ;
#7992=VECTOR('',#63723,10.) ;
#7993=VECTOR('',#63728,10.) ;
#7994=VECTOR('',#63731,10.) ;
#7995=VECTOR('',#63734,10.) ;
#7996=VECTOR('',#63735,10.) ;
#7997=VECTOR('',#63736,0.999999999999996) ;
#7998=VECTOR('',#63751,10.) ;
#7999=VECTOR('',#63760,10.) ;
#8000=VECTOR('',#63773,10.) ;
#8001=VECTOR('',#63774,10.) ;
#8002=VECTOR('',#63791,10.) ;
#8003=VECTOR('',#63802,10.) ;
#8004=VECTOR('',#63815,9.99999999999999) ;
#8005=VECTOR('',#63816,9.99999999999999) ;
#8006=VECTOR('',#63825,10.) ;
#8007=VECTOR('',#63830,10.) ;
#8008=VECTOR('',#63831,10.) ;
#8009=VECTOR('',#63834,10.) ;
#8010=VECTOR('',#63839,10.) ;
#8011=VECTOR('',#63840,10.) ;
#8012=VECTOR('',#63841,10.) ;
#8013=VECTOR('',#63842,10.) ;
#8014=VECTOR('',#63845,10.) ;
#8015=VECTOR('',#63852,10.) ;
#8016=VECTOR('',#63865,10.) ;
#8017=VECTOR('',#63866,10.) ;
#8018=VECTOR('',#63885,10.) ;
#8019=VECTOR('',#63888,10.) ;
#8020=VECTOR('',#63891,10.) ;
#8021=VECTOR('',#63892,10.) ;
#8022=VECTOR('',#63893,10.) ;
#8023=VECTOR('',#63894,10.) ;
#8024=VECTOR('',#63899,10.) ;
#8025=VECTOR('',#63902,10.) ;
#8026=VECTOR('',#63909,10.) ;
#8027=VECTOR('',#63916,10.) ;
#8028=VECTOR('',#63921,10.) ;
#8029=VECTOR('',#63924,10.) ;
#8030=VECTOR('',#63927,10.) ;
#8031=VECTOR('',#63930,10.) ;
#8032=VECTOR('',#63931,10.) ;
#8033=VECTOR('',#63950,10.) ;
#8034=VECTOR('',#63951,10.) ;
#8035=VECTOR('',#63954,10.) ;
#8036=VECTOR('',#63955,10.) ;
#8037=VECTOR('',#63956,10.) ;
#8038=VECTOR('',#63957,10.) ;
#8039=VECTOR('',#63958,10.) ;
#8040=VECTOR('',#63961,10.) ;
#8041=VECTOR('',#63966,10.) ;
#8042=VECTOR('',#63969,10.) ;
#8043=VECTOR('',#63980,10.) ;
#8044=VECTOR('',#63981,10.) ;
#8045=VECTOR('',#63984,10.) ;
#8046=VECTOR('',#63985,10.) ;
#8047=VECTOR('',#63998,10.) ;
#8048=VECTOR('',#63999,10.) ;
#8049=VECTOR('',#64002,10.) ;
#8050=VECTOR('',#64003,10.) ;
#8051=VECTOR('',#64006,10.) ;
#8052=VECTOR('',#64007,10.) ;
#8053=VECTOR('',#64010,10.) ;
#8054=VECTOR('',#64013,10.) ;
#8055=VECTOR('',#64016,10.) ;
#8056=VECTOR('',#64019,10.) ;
#8057=VECTOR('',#64022,10.) ;
#8058=VECTOR('',#64023,10.) ;
#8059=VECTOR('',#64024,10.) ;
#8060=VECTOR('',#64025,10.) ;
#8061=VECTOR('',#64026,10.) ;
#8062=VECTOR('',#64029,10.) ;
#8063=VECTOR('',#64032,10.) ;
#8064=VECTOR('',#64035,10.) ;
#8065=VECTOR('',#64038,10.) ;
#8066=VECTOR('',#64041,10.) ;
#8067=VECTOR('',#64044,10.) ;
#8068=VECTOR('',#64045,10.) ;
#8069=VECTOR('',#64046,10.) ;
#8070=VECTOR('',#64049,10.) ;
#8071=VECTOR('',#64052,10.) ;
#8072=VECTOR('',#64055,10.) ;
#8073=VECTOR('',#64058,10.) ;
#8074=VECTOR('',#64061,10.) ;
#8075=VECTOR('',#64062,10.) ;
#8076=VECTOR('',#64063,10.) ;
#8077=VECTOR('',#64064,10.) ;
#8078=VECTOR('',#64065,10.) ;
#8079=VECTOR('',#64066,10.) ;
#8080=VECTOR('',#64067,10.) ;
#8081=VECTOR('',#64068,10.) ;
#8082=VECTOR('',#64069,10.) ;
#8083=VECTOR('',#64070,10.) ;
#8084=VECTOR('',#64073,10.) ;
#8085=VECTOR('',#64076,10.) ;
#8086=VECTOR('',#64077,10.) ;
#8087=VECTOR('',#64080,9.99999999999999) ;
#8088=VECTOR('',#64081,10.) ;
#8089=VECTOR('',#64084,10.) ;
#8090=VECTOR('',#64085,10.) ;
#8091=VECTOR('',#64086,10.) ;
#8092=VECTOR('',#64087,10.) ;
#8093=VECTOR('',#64096,10.) ;
#8094=VECTOR('',#64099,10.) ;
#8095=VECTOR('',#64100,10.) ;
#8096=VECTOR('',#64103,10.) ;
#8097=VECTOR('',#64106,10.) ;
#8098=VECTOR('',#64107,10.) ;
#8099=VECTOR('',#64110,10.) ;
#8100=VECTOR('',#64113,10.) ;
#8101=VECTOR('',#64114,10.) ;
#8102=VECTOR('',#64115,10.) ;
#8103=VECTOR('',#64118,10.) ;
#8104=VECTOR('',#64121,10.) ;
#8105=VECTOR('',#64124,10.) ;
#8106=VECTOR('',#64127,10.) ;
#8107=VECTOR('',#64128,10.) ;
#8108=VECTOR('',#64133,10.) ;
#8109=VECTOR('',#64136,10.) ;
#8110=VECTOR('',#64137,10.) ;
#8111=VECTOR('',#64140,10.) ;
#8112=VECTOR('',#64145,10.) ;
#8113=VECTOR('',#64146,10.) ;
#8114=VECTOR('',#64149,10.) ;
#8115=VECTOR('',#64152,10.) ;
#8116=VECTOR('',#64155,10.) ;
#8117=VECTOR('',#64158,10.) ;
#8118=VECTOR('',#64163,10.) ;
#8119=VECTOR('',#64166,10.) ;
#8120=VECTOR('',#64167,10.) ;
#8121=VECTOR('',#64170,10.) ;
#8122=VECTOR('',#64173,10.) ;
#8123=VECTOR('',#64176,10.) ;
#8124=VECTOR('',#64179,10.) ;
#8125=VECTOR('',#64180,10.) ;
#8126=VECTOR('',#64183,10.) ;
#8127=VECTOR('',#64184,10.) ;
#8128=VECTOR('',#64187,10.) ;
#8129=VECTOR('',#64190,10.) ;
#8130=VECTOR('',#64193,10.) ;
#8131=VECTOR('',#64196,10.) ;
#8132=VECTOR('',#64197,10.) ;
#8133=VECTOR('',#64198,10.) ;
#8134=VECTOR('',#64199,10.) ;
#8135=VECTOR('',#64202,10.) ;
#8136=VECTOR('',#64205,10.) ;
#8137=VECTOR('',#64208,10.) ;
#8138=VECTOR('',#64211,10.) ;
#8139=VECTOR('',#64212,10.) ;
#8140=VECTOR('',#64215,10.) ;
#8141=VECTOR('',#64218,10.) ;
#8142=VECTOR('',#64219,10.) ;
#8143=VECTOR('',#64222,10.) ;
#8144=VECTOR('',#64225,10.) ;
#8145=VECTOR('',#64228,10.) ;
#8146=VECTOR('',#64231,10.) ;
#8147=VECTOR('',#64232,10.) ;
#8148=VECTOR('',#64241,10.) ;
#8149=VECTOR('',#64242,10.) ;
#8150=VECTOR('',#64257,10.) ;
#8151=VECTOR('',#64260,10.) ;
#8152=VECTOR('',#64263,10.) ;
#8153=VECTOR('',#64266,10.) ;
#8154=VECTOR('',#64269,10.) ;
#8155=VECTOR('',#64270,10.) ;
#8156=VECTOR('',#64271,10.) ;
#8157=VECTOR('',#64272,10.) ;
#8158=VECTOR('',#64275,10.) ;
#8159=VECTOR('',#64276,10.) ;
#8160=VECTOR('',#64277,10.) ;
#8161=VECTOR('',#64278,10.) ;
#8162=VECTOR('',#64289,10.) ;
#8163=VECTOR('',#64292,10.) ;
#8164=VECTOR('',#64305,10.) ;
#8165=VECTOR('',#64306,10.) ;
#8166=VECTOR('',#64317,10.) ;
#8167=VECTOR('',#64318,10.) ;
#8168=VECTOR('',#64321,10.) ;
#8169=VECTOR('',#64324,10.) ;
#8170=VECTOR('',#64335,10.) ;
#8171=VECTOR('',#64336,10.) ;
#8172=VECTOR('',#64359,10.) ;
#8173=VECTOR('',#64368,10.) ;
#8174=VECTOR('',#64371,10.) ;
#8175=VECTOR('',#64372,10.) ;
#8176=VECTOR('',#64377,10.) ;
#8177=VECTOR('',#64388,10.) ;
#8178=VECTOR('',#64391,10.) ;
#8179=VECTOR('',#64392,10.) ;
#8180=VECTOR('',#64397,10.) ;
#8181=VECTOR('',#64398,10.) ;
#8182=VECTOR('',#64399,10.) ;
#8183=VECTOR('',#64404,10.) ;
#8184=VECTOR('',#64409,10.) ;
#8185=VECTOR('',#64410,10.) ;
#8186=VECTOR('',#64413,10.) ;
#8187=VECTOR('',#64418,10.) ;
#8188=VECTOR('',#64419,9.99999999999999) ;
#8189=VECTOR('',#64422,10.) ;
#8190=VECTOR('',#64425,10.) ;
#8191=VECTOR('',#64428,10.) ;
#8192=VECTOR('',#64431,10.) ;
#8193=VECTOR('',#64436,10.) ;
#8194=VECTOR('',#64437,10.) ;
#8195=VECTOR('',#64440,0.999999999999996) ;
#8196=VECTOR('',#64457,10.) ;
#8197=VECTOR('',#64458,10.) ;
#8198=VECTOR('',#64473,10.) ;
#8199=VECTOR('',#64474,10.) ;
#8200=VECTOR('',#64505,10.) ;
#8201=VECTOR('',#64506,10.) ;
#8202=VECTOR('',#64511,10.) ;
#8203=VECTOR('',#64512,10.) ;
#8204=VECTOR('',#64521,10.) ;
#8205=VECTOR('',#64526,10.) ;
#8206=VECTOR('',#64527,10.) ;
#8207=VECTOR('',#64538,10.) ;
#8208=VECTOR('',#64547,10.) ;
#8209=VECTOR('',#64552,10.) ;
#8210=VECTOR('',#64553,10.) ;
#8211=VECTOR('',#64558,10.) ;
#8212=VECTOR('',#64559,10.) ;
#8213=VECTOR('',#64572,10.) ;
#8214=VECTOR('',#64573,10.) ;
#8215=VECTOR('',#64586,10.) ;
#8216=VECTOR('',#64587,10.) ;
#8217=VECTOR('',#64600,10.) ;
#8218=VECTOR('',#64601,10.) ;
#8219=VECTOR('',#64612,10.) ;
#8220=VECTOR('',#64613,10.) ;
#8221=VECTOR('',#64618,10.) ;
#8222=VECTOR('',#64619,10.) ;
#8223=VECTOR('',#64628,10.) ;
#8224=VECTOR('',#64629,10.) ;
#8225=VECTOR('',#64634,10.) ;
#8226=VECTOR('',#64637,10.) ;
#8227=VECTOR('',#64640,10.) ;
#8228=VECTOR('',#64643,10.) ;
#8229=VECTOR('',#64646,10.) ;
#8230=VECTOR('',#64647,10.) ;
#8231=VECTOR('',#64650,10.) ;
#8232=VECTOR('',#64653,10.) ;
#8233=VECTOR('',#64656,10.) ;
#8234=VECTOR('',#64659,10.) ;
#8235=VECTOR('',#64662,10.) ;
#8236=VECTOR('',#64663,10.) ;
#8237=VECTOR('',#64664,10.) ;
#8238=VECTOR('',#64667,10.) ;
#8239=VECTOR('',#64670,10.) ;
#8240=VECTOR('',#64671,10.) ;
#8241=VECTOR('',#64672,10.) ;
#8242=VECTOR('',#64675,10.) ;
#8243=VECTOR('',#64678,10.) ;
#8244=VECTOR('',#64685,10.) ;
#8245=VECTOR('',#64688,10.) ;
#8246=VECTOR('',#64691,10.) ;
#8247=VECTOR('',#64692,10.) ;
#8248=VECTOR('',#64693,10.) ;
#8249=VECTOR('',#64700,10.) ;
#8250=VECTOR('',#64723,10.) ;
#8251=VECTOR('',#64724,10.) ;
#8252=VECTOR('',#64729,10.) ;
#8253=VECTOR('',#64732,10.) ;
#8254=VECTOR('',#64743,10.) ;
#8255=VECTOR('',#64744,10.) ;
#8256=VECTOR('',#64749,10.) ;
#8257=VECTOR('',#64750,10.) ;
#8258=VECTOR('',#64755,10.) ;
#8259=VECTOR('',#64756,10.) ;
#8260=VECTOR('',#64761,10.) ;
#8261=VECTOR('',#64762,10.) ;
#8262=VECTOR('',#64775,10.) ;
#8263=VECTOR('',#64776,10.) ;
#8264=VECTOR('',#64779,10.) ;
#8265=VECTOR('',#64782,10.) ;
#8266=VECTOR('',#64785,10.) ;
#8267=VECTOR('',#64786,10.) ;
#8268=VECTOR('',#64789,10.) ;
#8269=VECTOR('',#64790,10.) ;
#8270=VECTOR('',#64793,10.) ;
#8271=VECTOR('',#64796,10.) ;
#8272=VECTOR('',#64799,10.) ;
#8273=VECTOR('',#64802,10.) ;
#8274=VECTOR('',#64807,10.) ;
#8275=VECTOR('',#64808,10.) ;
#8276=VECTOR('',#64809,10.) ;
#8277=VECTOR('',#64810,10.) ;
#8278=VECTOR('',#64811,10.) ;
#8279=VECTOR('',#64812,10.) ;
#8280=VECTOR('',#64813,10.) ;
#8281=VECTOR('',#64818,10.) ;
#8282=VECTOR('',#64827,10.) ;
#8283=VECTOR('',#64838,10.) ;
#8284=VECTOR('',#64849,10.) ;
#8285=VECTOR('',#64860,10.) ;
#8286=VECTOR('',#64871,10.) ;
#8287=VECTOR('',#64882,9.99999999999999) ;
#8288=VECTOR('',#64891,10.) ;
#8289=VECTOR('',#64920,10.) ;
#8290=VECTOR('',#64937,10.) ;
#8291=VECTOR('',#64952,10.) ;
#8292=VECTOR('',#64953,10.) ;
#8293=VECTOR('',#64960,10.) ;
#8294=VECTOR('',#64963,10.) ;
#8295=VECTOR('',#64966,10.) ;
#8296=VECTOR('',#64969,10.) ;
#8297=VECTOR('',#64976,10.) ;
#8298=VECTOR('',#64983,10.) ;
#8299=VECTOR('',#64994,10.) ;
#8300=VECTOR('',#65005,10.) ;
#8301=VECTOR('',#65024,10.) ;
#8302=VECTOR('',#65033,10.) ;
#8303=VECTOR('',#65040,10.) ;
#8304=VECTOR('',#65043,10.) ;
#8305=VECTOR('',#65056,10.) ;
#8306=VECTOR('',#65067,10.) ;
#8307=VECTOR('',#65076,10.) ;
#8308=VECTOR('',#65081,10.) ;
#8309=VECTOR('',#65086,10.) ;
#8310=VECTOR('',#65089,10.) ;
#8311=VECTOR('',#65092,10.) ;
#8312=VECTOR('',#65095,10.) ;
#8313=VECTOR('',#65096,10.) ;
#8314=VECTOR('',#65097,10.) ;
#8315=VECTOR('',#65098,10.) ;
#8316=VECTOR('',#65099,10.) ;
#8317=VECTOR('',#65100,10.) ;
#8318=VECTOR('',#65101,10.) ;
#8319=VECTOR('',#65102,10.) ;
#8320=VECTOR('',#65103,10.) ;
#8321=VECTOR('',#65104,10.) ;
#8322=VECTOR('',#65107,10.) ;
#8323=VECTOR('',#65112,10.) ;
#8324=VECTOR('',#65113,10.) ;
#8325=VECTOR('',#65118,10.) ;
#8326=VECTOR('',#65119,10.) ;
#8327=VECTOR('',#65120,10.) ;
#8328=VECTOR('',#65127,10.) ;
#8329=VECTOR('',#65132,10.) ;
#8330=VECTOR('',#65133,10.) ;
#8331=VECTOR('',#65134,10.) ;
#8332=VECTOR('',#65135,10.) ;
#8333=VECTOR('',#65138,10.) ;
#8334=VECTOR('',#65139,10.) ;
#8335=VECTOR('',#65158,10.) ;
#8336=VECTOR('',#65161,10.) ;
#8337=VECTOR('',#65174,9.99999999999999) ;
#8338=VECTOR('',#65175,9.99999999999999) ;
#8339=VECTOR('',#65180,10.) ;
#8340=VECTOR('',#65181,10.) ;
#8341=VECTOR('',#65184,10.) ;
#8342=VECTOR('',#65185,10.) ;
#8343=VECTOR('',#65190,10.) ;
#8344=VECTOR('',#65191,10.) ;
#8345=VECTOR('',#65196,9.99999999999999) ;
#8346=VECTOR('',#65197,10.) ;
#8347=VECTOR('',#65204,10.) ;
#8348=VECTOR('',#65207,10.) ;
#8349=VECTOR('',#65210,10.) ;
#8350=VECTOR('',#65213,10.) ;
#8351=VECTOR('',#65216,10.) ;
#8352=VECTOR('',#65219,10.) ;
#8353=VECTOR('',#65226,10.) ;
#8354=VECTOR('',#65229,10.) ;
#8355=VECTOR('',#65236,10.) ;
#8356=VECTOR('',#65239,10.) ;
#8357=VECTOR('',#65244,10.) ;
#8358=VECTOR('',#65245,10.) ;
#8359=VECTOR('',#65246,10.) ;
#8360=VECTOR('',#65247,10.) ;
#8361=VECTOR('',#65248,10.) ;
#8362=VECTOR('',#65251,10.) ;
#8363=VECTOR('',#65252,10.) ;
#8364=VECTOR('',#65255,10.) ;
#8365=VECTOR('',#65256,10.) ;
#8366=VECTOR('',#65275,10.) ;
#8367=VECTOR('',#65278,10.) ;
#8368=VECTOR('',#65279,10.) ;
#8369=VECTOR('',#65282,10.) ;
#8370=VECTOR('',#65293,10.) ;
#8371=VECTOR('',#65294,10.) ;
#8372=VECTOR('',#65305,10.) ;
#8373=VECTOR('',#65308,10.) ;
#8374=VECTOR('',#65309,10.) ;
#8375=VECTOR('',#65310,10.) ;
#8376=VECTOR('',#65313,10.) ;
#8377=VECTOR('',#65314,10.) ;
#8378=VECTOR('',#65315,10.) ;
#8379=VECTOR('',#65318,10.) ;
#8380=VECTOR('',#65319,10.) ;
#8381=VECTOR('',#65320,10.) ;
#8382=VECTOR('',#65323,10.) ;
#8383=VECTOR('',#65324,10.) ;
#8384=VECTOR('',#65325,10.) ;
#8385=VECTOR('',#65326,9.99999999999999) ;
#8386=VECTOR('',#65327,10.) ;
#8387=VECTOR('',#65328,10.) ;
#8388=VECTOR('',#65329,10.) ;
#8389=VECTOR('',#65332,10.) ;
#8390=VECTOR('',#65333,10.) ;
#8391=VECTOR('',#65334,10.) ;
#8392=VECTOR('',#65335,9.99999999999999) ;
#8393=VECTOR('',#65336,10.) ;
#8394=VECTOR('',#65337,10.) ;
#8395=VECTOR('',#65340,10.) ;
#8396=VECTOR('',#65341,10.) ;
#8397=VECTOR('',#65342,10.) ;
#8398=VECTOR('',#65343,10.) ;
#8399=VECTOR('',#65344,10.) ;
#8400=VECTOR('',#65349,10.) ;
#8401=VECTOR('',#65354,10.) ;
#8402=VECTOR('',#65365,9.99999999999999) ;
#8403=VECTOR('',#65370,10.) ;
#8404=VECTOR('',#65373,10.) ;
#8405=VECTOR('',#65378,10.) ;
#8406=VECTOR('',#65381,10.) ;
#8407=VECTOR('',#65384,10.) ;
#8408=VECTOR('',#65389,10.) ;
#8409=VECTOR('',#65390,10.) ;
#8410=VECTOR('',#65393,10.) ;
#8411=VECTOR('',#65394,10.) ;
#8412=VECTOR('',#65397,10.) ;
#8413=VECTOR('',#65400,10.) ;
#8414=VECTOR('',#65403,10.) ;
#8415=VECTOR('',#65410,10.) ;
#8416=VECTOR('',#65413,10.) ;
#8417=VECTOR('',#65418,10.) ;
#8418=VECTOR('',#65419,10.) ;
#8419=VECTOR('',#65420,10.) ;
#8420=VECTOR('',#65421,10.) ;
#8421=VECTOR('',#65422,10.) ;
#8422=VECTOR('',#65427,10.) ;
#8423=VECTOR('',#65430,10.) ;
#8424=VECTOR('',#65431,10.) ;
#8425=VECTOR('',#65432,10.) ;
#8426=VECTOR('',#65437,10.) ;
#8427=VECTOR('',#65442,10.) ;
#8428=VECTOR('',#65447,10.) ;
#8429=VECTOR('',#65448,10.) ;
#8430=VECTOR('',#65451,10.) ;
#8431=VECTOR('',#65452,10.) ;
#8432=VECTOR('',#65455,9.99999999999999) ;
#8433=VECTOR('',#65458,9.99999999999999) ;
#8434=VECTOR('',#65459,10.) ;
#8435=VECTOR('',#65462,10.) ;
#8436=VECTOR('',#65465,10.) ;
#8437=VECTOR('',#65466,10.) ;
#8438=VECTOR('',#65485,9.99999999999999) ;
#8439=VECTOR('',#65488,10.) ;
#8440=VECTOR('',#65489,10.) ;
#8441=VECTOR('',#65490,10.) ;
#8442=VECTOR('',#65493,10.) ;
#8443=VECTOR('',#65494,10.) ;
#8444=VECTOR('',#65495,10.) ;
#8445=VECTOR('',#65498,10.) ;
#8446=VECTOR('',#65499,10.) ;
#8447=VECTOR('',#65502,10.) ;
#8448=VECTOR('',#65505,10.) ;
#8449=VECTOR('',#65508,10.) ;
#8450=VECTOR('',#65513,10.) ;
#8451=VECTOR('',#65514,10.) ;
#8452=VECTOR('',#65519,10.) ;
#8453=VECTOR('',#65520,10.) ;
#8454=VECTOR('',#65523,10.) ;
#8455=VECTOR('',#65524,10.) ;
#8456=VECTOR('',#65529,10.) ;
#8457=VECTOR('',#65530,10.) ;
#8458=VECTOR('',#65535,10.) ;
#8459=VECTOR('',#65536,10.) ;
#8460=VECTOR('',#65539,10.) ;
#8461=VECTOR('',#65540,10.) ;
#8462=VECTOR('',#65541,10.) ;
#8463=VECTOR('',#65544,10.) ;
#8464=VECTOR('',#65545,10.) ;
#8465=VECTOR('',#65548,10.) ;
#8466=VECTOR('',#65549,10.) ;
#8467=VECTOR('',#65552,10.) ;
#8468=VECTOR('',#65553,10.) ;
#8469=VECTOR('',#65558,10.) ;
#8470=VECTOR('',#65561,10.) ;
#8471=VECTOR('',#65564,10.) ;
#8472=VECTOR('',#65567,10.) ;
#8473=VECTOR('',#65570,10.) ;
#8474=VECTOR('',#65571,10.) ;
#8475=VECTOR('',#65576,10.) ;
#8476=VECTOR('',#65577,10.) ;
#8477=VECTOR('',#65580,10.) ;
#8478=VECTOR('',#65581,10.) ;
#8479=VECTOR('',#65584,10.) ;
#8480=VECTOR('',#65585,10.) ;
#8481=VECTOR('',#65586,10.) ;
#8482=VECTOR('',#65587,10.) ;
#8483=VECTOR('',#65590,10.) ;
#8484=VECTOR('',#65591,10.) ;
#8485=VECTOR('',#65592,10.) ;
#8486=VECTOR('',#65597,10.) ;
#8487=VECTOR('',#65600,10.) ;
#8488=VECTOR('',#65605,10.) ;
#8489=VECTOR('',#65608,10.) ;
#8490=VECTOR('',#65611,9.99999999999999) ;
#8491=VECTOR('',#65614,9.99999999999999) ;
#8492=VECTOR('',#65617,10.) ;
#8493=VECTOR('',#65618,10.) ;
#8494=VECTOR('',#65623,10.) ;
#8495=VECTOR('',#65624,10.) ;
#8496=VECTOR('',#65629,10.) ;
#8497=VECTOR('',#65630,10.) ;
#8498=VECTOR('',#65635,10.) ;
#8499=VECTOR('',#65636,10.) ;
#8500=VECTOR('',#65639,10.) ;
#8501=VECTOR('',#65640,10.) ;
#8502=VECTOR('',#65641,10.) ;
#8503=VECTOR('',#65644,10.) ;
#8504=VECTOR('',#65645,10.) ;
#8505=VECTOR('',#65648,10.) ;
#8506=VECTOR('',#65649,10.) ;
#8507=VECTOR('',#65652,10.) ;
#8508=VECTOR('',#65653,10.) ;
#8509=VECTOR('',#65658,10.) ;
#8510=VECTOR('',#65661,10.) ;
#8511=VECTOR('',#65666,10.) ;
#8512=VECTOR('',#65667,10.) ;
#8513=VECTOR('',#65672,10.) ;
#8514=VECTOR('',#65673,10.) ;
#8515=VECTOR('',#65678,10.) ;
#8516=VECTOR('',#65679,10.) ;
#8517=VECTOR('',#65682,10.) ;
#8518=VECTOR('',#65683,10.) ;
#8519=VECTOR('',#65684,10.) ;
#8520=VECTOR('',#65687,10.) ;
#8521=VECTOR('',#65688,10.) ;
#8522=VECTOR('',#65693,10.) ;
#8523=VECTOR('',#65696,10.) ;
#8524=VECTOR('',#65701,10.) ;
#8525=VECTOR('',#65704,10.) ;
#8526=VECTOR('',#65707,10.) ;
#8527=VECTOR('',#65710,10.) ;
#8528=VECTOR('',#65713,10.) ;
#8529=VECTOR('',#65714,10.) ;
#8530=VECTOR('',#65719,10.) ;
#8531=VECTOR('',#65720,10.) ;
#8532=VECTOR('',#65725,10.) ;
#8533=VECTOR('',#65726,10.) ;
#8534=VECTOR('',#65731,10.) ;
#8535=VECTOR('',#65732,10.) ;
#8536=VECTOR('',#65735,10.) ;
#8537=VECTOR('',#65736,10.) ;
#8538=VECTOR('',#65737,10.) ;
#8539=VECTOR('',#65740,10.) ;
#8540=VECTOR('',#65741,10.) ;
#8541=VECTOR('',#65744,10.) ;
#8542=VECTOR('',#65745,10.) ;
#8543=VECTOR('',#65748,10.) ;
#8544=VECTOR('',#65749,10.) ;
#8545=VECTOR('',#65754,10.) ;
#8546=VECTOR('',#65757,10.) ;
#8547=VECTOR('',#65762,10.) ;
#8548=VECTOR('',#65763,10.) ;
#8549=VECTOR('',#65768,10.) ;
#8550=VECTOR('',#65769,10.) ;
#8551=VECTOR('',#65774,10.) ;
#8552=VECTOR('',#65775,10.) ;
#8553=VECTOR('',#65778,10.) ;
#8554=VECTOR('',#65779,10.) ;
#8555=VECTOR('',#65780,10.) ;
#8556=VECTOR('',#65783,10.) ;
#8557=VECTOR('',#65784,10.) ;
#8558=VECTOR('',#65789,9.99999999999999) ;
#8559=VECTOR('',#65792,9.99999999999999) ;
#8560=VECTOR('',#65797,10.) ;
#8561=VECTOR('',#65800,10.) ;
#8562=VECTOR('',#65803,10.) ;
#8563=VECTOR('',#65806,10.) ;
#8564=VECTOR('',#65817,10.) ;
#8565=VECTOR('',#65818,10.) ;
#8566=VECTOR('',#65823,10.) ;
#8567=VECTOR('',#65824,10.) ;
#8568=VECTOR('',#65829,10.) ;
#8569=VECTOR('',#65832,10.) ;
#8570=VECTOR('',#65843,10.) ;
#8571=VECTOR('',#65844,10.) ;
#8572=VECTOR('',#65849,10.) ;
#8573=VECTOR('',#65850,10.) ;
#8574=VECTOR('',#65855,10.) ;
#8575=VECTOR('',#65856,10.) ;
#8576=VECTOR('',#65859,10.) ;
#8577=VECTOR('',#65860,10.) ;
#8578=VECTOR('',#65861,10.) ;
#8579=VECTOR('',#65864,10.) ;
#8580=VECTOR('',#65869,10.) ;
#8581=VECTOR('',#65870,10.) ;
#8582=VECTOR('',#65873,10.) ;
#8583=VECTOR('',#65874,10.) ;
#8584=VECTOR('',#65877,10.) ;
#8585=VECTOR('',#65878,10.) ;
#8586=VECTOR('',#65881,10.) ;
#8587=VECTOR('',#65882,9.99999999999999) ;
#8588=VECTOR('',#65887,10.) ;
#8589=VECTOR('',#65890,10.) ;
#8590=VECTOR('',#65895,10.) ;
#8591=VECTOR('',#65898,10.) ;
#8592=VECTOR('',#65909,10.) ;
#8593=VECTOR('',#65910,10.) ;
#8594=VECTOR('',#65915,10.) ;
#8595=VECTOR('',#65918,10.) ;
#8596=VECTOR('',#65921,10.) ;
#8597=VECTOR('',#65924,10.) ;
#8598=VECTOR('',#65935,10.) ;
#8599=VECTOR('',#65936,10.) ;
#8600=VECTOR('',#65941,10.) ;
#8601=VECTOR('',#65942,10.) ;
#8602=VECTOR('',#65947,10.) ;
#8603=VECTOR('',#65948,10.) ;
#8604=VECTOR('',#65953,9.99999999999999) ;
#8605=VECTOR('',#65954,9.99999999999999) ;
#8606=VECTOR('',#65957,10.) ;
#8607=VECTOR('',#65960,10.) ;
#8608=VECTOR('',#65963,10.) ;
#8609=VECTOR('',#65964,10.) ;
#8610=VECTOR('',#65967,10.) ;
#8611=VECTOR('',#65968,10.) ;
#8612=VECTOR('',#65971,10.) ;
#8613=VECTOR('',#65972,10.) ;
#8614=VECTOR('',#65975,10.) ;
#8615=VECTOR('',#65976,9.99999999999999) ;
#8616=VECTOR('',#65979,10.) ;
#8617=VECTOR('',#65980,10.) ;
#8618=VECTOR('',#65985,10.) ;
#8619=VECTOR('',#66000,10.) ;
#8620=VECTOR('',#66003,10.) ;
#8621=VECTOR('',#66012,10.) ;
#8622=VECTOR('',#66017,10.) ;
#8623=VECTOR('',#66020,10.) ;
#8624=VECTOR('',#66025,10.) ;
#8625=VECTOR('',#66028,10.) ;
#8626=VECTOR('',#66031,10.) ;
#8627=VECTOR('',#66034,10.) ;
#8628=VECTOR('',#66039,9.99999999999999) ;
#8629=VECTOR('',#66042,9.99999999999999) ;
#8630=VECTOR('',#66045,10.) ;
#8631=VECTOR('',#66050,10.) ;
#8632=VECTOR('',#66055,10.) ;
#8633=VECTOR('',#66060,10.) ;
#8634=VECTOR('',#66065,10.) ;
#8635=VECTOR('',#66066,10.) ;
#8636=VECTOR('',#66069,10.) ;
#8637=VECTOR('',#66072,10.) ;
#8638=VECTOR('',#66077,10.) ;
#8639=VECTOR('',#66080,10.) ;
#8640=VECTOR('',#66085,10.) ;
#8641=VECTOR('',#66088,10.) ;
#8642=VECTOR('',#66089,10.) ;
#8643=VECTOR('',#66092,10.) ;
#8644=VECTOR('',#66093,10.) ;
#8645=VECTOR('',#66094,10.) ;
#8646=VECTOR('',#66095,10.) ;
#8647=VECTOR('',#66096,10.) ;
#8648=VECTOR('',#66097,10.) ;
#8649=VECTOR('',#66098,10.) ;
#8650=VECTOR('',#66099,10.) ;
#8651=VECTOR('',#66100,10.) ;
#8652=VECTOR('',#66101,10.) ;
#8653=VECTOR('',#66102,10.) ;
#8654=VECTOR('',#66115,10.) ;
#8655=VECTOR('',#66120,10.) ;
#8656=VECTOR('',#66123,10.) ;
#8657=VECTOR('',#66128,10.) ;
#8658=VECTOR('',#66135,10.) ;
#8659=VECTOR('',#66154,10.) ;
#8660=VECTOR('',#66157,10.) ;
#8661=VECTOR('',#66160,10.) ;
#8662=VECTOR('',#66171,10.) ;
#8663=VECTOR('',#66178,10.) ;
#8664=VECTOR('',#66181,10.) ;
#8665=VECTOR('',#66190,10.) ;
#8666=VECTOR('',#66225,10.) ;
#8667=VECTOR('',#66228,10.) ;
#8668=VECTOR('',#66229,10.) ;
#8669=VECTOR('',#66232,10.) ;
#8670=VECTOR('',#66235,10.) ;
#8671=VECTOR('',#66242,10.) ;
#8672=VECTOR('',#66247,10.) ;
#8673=VECTOR('',#66276,10.) ;
#8674=VECTOR('',#66279,10.) ;
#8675=VECTOR('',#66290,10.) ;
#8676=VECTOR('',#66293,10.) ;
#8677=VECTOR('',#66296,10.) ;
#8678=VECTOR('',#66299,10.) ;
#8679=VECTOR('',#66306,10.) ;
#8680=VECTOR('',#66317,10.) ;
#8681=VECTOR('',#66318,10.) ;
#8682=VECTOR('',#66321,10.) ;
#8683=VECTOR('',#66324,10.) ;
#8684=VECTOR('',#66327,10.) ;
#8685=VECTOR('',#66328,10.) ;
#8686=VECTOR('',#66331,10.) ;
#8687=VECTOR('',#66334,10.) ;
#8688=VECTOR('',#66339,10.) ;
#8689=VECTOR('',#66340,10.) ;
#8690=VECTOR('',#66343,10.) ;
#8691=VECTOR('',#66348,10.) ;
#8692=VECTOR('',#66349,10.) ;
#8693=VECTOR('',#66352,10.) ;
#8694=VECTOR('',#66353,10.) ;
#8695=VECTOR('',#66356,10.) ;
#8696=VECTOR('',#66357,10.) ;
#8697=VECTOR('',#66360,10.) ;
#8698=VECTOR('',#66365,10.) ;
#8699=VECTOR('',#66370,10.) ;
#8700=VECTOR('',#66371,10.) ;
#8701=VECTOR('',#66374,10.) ;
#8702=VECTOR('',#66379,10.) ;
#8703=VECTOR('',#66380,10.) ;
#8704=VECTOR('',#66381,10.) ;
#8705=VECTOR('',#66384,10.) ;
#8706=VECTOR('',#66385,10.) ;
#8707=VECTOR('',#66388,10.) ;
#8708=VECTOR('',#66389,10.) ;
#8709=VECTOR('',#66392,10.) ;
#8710=VECTOR('',#66397,10.) ;
#8711=VECTOR('',#66398,10.) ;
#8712=VECTOR('',#66399,10.) ;
#8713=VECTOR('',#66400,10.) ;
#8714=VECTOR('',#66403,10.) ;
#8715=VECTOR('',#66406,10.) ;
#8716=VECTOR('',#66409,10.) ;
#8717=VECTOR('',#66412,10.) ;
#8718=VECTOR('',#66417,0.4) ;
#8719=VECTOR('',#66426,10.) ;
#8720=VECTOR('',#66429,10.) ;
#8721=VECTOR('',#66430,10.) ;
#8722=VECTOR('',#66431,10.) ;
#8723=VECTOR('',#66436,10.) ;
#8724=VECTOR('',#66441,10.) ;
#8725=VECTOR('',#66444,10.) ;
#8726=VECTOR('',#66449,10.) ;
#8727=VECTOR('',#66458,10.) ;
#8728=VECTOR('',#66477,10.) ;
#8729=VECTOR('',#66490,10.) ;
#8730=VECTOR('',#66505,10.) ;
#8731=VECTOR('',#66518,10.) ;
#8732=VECTOR('',#66539,10.) ;
#8733=VECTOR('',#66546,10.) ;
#8734=VECTOR('',#66559,10.) ;
#8735=VECTOR('',#66570,10.) ;
#8736=VECTOR('',#66575,10.) ;
#8737=VECTOR('',#66586,10.) ;
#8738=VECTOR('',#66589,10.) ;
#8739=VECTOR('',#66606,10.) ;
#8740=VECTOR('',#66607,10.) ;
#8741=VECTOR('',#66610,10.) ;
#8742=VECTOR('',#66613,10.) ;
#8743=VECTOR('',#66622,10.) ;
#8744=VECTOR('',#66623,10.) ;
#8745=VECTOR('',#66626,10.) ;
#8746=VECTOR('',#66627,10.) ;
#8747=VECTOR('',#66630,10.) ;
#8748=VECTOR('',#66633,10.) ;
#8749=VECTOR('',#66636,10.) ;
#8750=VECTOR('',#66647,10.) ;
#8751=VECTOR('',#66648,10.) ;
#8752=VECTOR('',#66651,10.) ;
#8753=VECTOR('',#66652,10.) ;
#8754=VECTOR('',#66655,10.) ;
#8755=VECTOR('',#66656,10.) ;
#8756=VECTOR('',#66657,10.) ;
#8757=VECTOR('',#66662,10.) ;
#8758=VECTOR('',#66665,10.) ;
#8759=VECTOR('',#66666,10.) ;
#8760=VECTOR('',#66669,10.) ;
#8761=VECTOR('',#66670,10.) ;
#8762=VECTOR('',#66675,10.) ;
#8763=VECTOR('',#66678,10.) ;
#8764=VECTOR('',#66679,10.) ;
#8765=VECTOR('',#66684,10.) ;
#8766=VECTOR('',#66687,10.) ;
#8767=VECTOR('',#66688,10.) ;
#8768=VECTOR('',#66691,10.) ;
#8769=VECTOR('',#66692,10.) ;
#8770=VECTOR('',#66693,10.) ;
#8771=VECTOR('',#66696,10.) ;
#8772=VECTOR('',#66697,10.) ;
#8773=VECTOR('',#66700,10.) ;
#8774=VECTOR('',#66703,10.) ;
#8775=VECTOR('',#66710,2.6) ;
#8776=VECTOR('',#66715,10.) ;
#8777=VECTOR('',#66716,10.) ;
#8778=VECTOR('',#66717,10.) ;
#8779=VECTOR('',#66722,10.) ;
#8780=VECTOR('',#66725,10.) ;
#8781=VECTOR('',#66726,10.) ;
#8782=VECTOR('',#66731,10.) ;
#8783=VECTOR('',#66734,10.) ;
#8784=VECTOR('',#66735,10.) ;
#8785=VECTOR('',#66740,10.) ;
#8786=VECTOR('',#66741,10.) ;
#8787=VECTOR('',#66744,10.) ;
#8788=VECTOR('',#66745,10.) ;
#8789=VECTOR('',#66750,10.) ;
#8790=VECTOR('',#66753,10.) ;
#8791=VECTOR('',#66754,10.) ;
#8792=VECTOR('',#66757,10.) ;
#8793=VECTOR('',#66758,10.) ;
#8794=VECTOR('',#66763,10.) ;
#8795=VECTOR('',#66766,10.) ;
#8796=VECTOR('',#66767,10.) ;
#8797=VECTOR('',#66770,2.49999999999999) ;
#8798=VECTOR('',#66775,10.) ;
#8799=VECTOR('',#66776,10.) ;
#8800=VECTOR('',#66777,10.) ;
#8801=VECTOR('',#66782,10.) ;
#8802=VECTOR('',#66785,10.) ;
#8803=VECTOR('',#66786,10.) ;
#8804=VECTOR('',#66791,10.) ;
#8805=VECTOR('',#66794,10.) ;
#8806=VECTOR('',#66795,10.) ;
#8807=VECTOR('',#66796,10.) ;
#8808=VECTOR('',#66801,10.) ;
#8809=VECTOR('',#66802,10.) ;
#8810=VECTOR('',#66805,10.) ;
#8811=VECTOR('',#66806,10.) ;
#8812=VECTOR('',#66811,10.) ;
#8813=VECTOR('',#66814,10.) ;
#8814=VECTOR('',#66815,10.) ;
#8815=VECTOR('',#66818,10.) ;
#8816=VECTOR('',#66821,10.) ;
#8817=VECTOR('',#66822,10.) ;
#8818=VECTOR('',#66827,10.) ;
#8819=VECTOR('',#66828,10.) ;
#8820=VECTOR('',#66831,10.) ;
#8821=VECTOR('',#66832,10.) ;
#8822=VECTOR('',#66833,10.) ;
#8823=VECTOR('',#66838,10.) ;
#8824=VECTOR('',#66841,10.) ;
#8825=VECTOR('',#66842,10.) ;
#8826=VECTOR('',#66851,10.) ;
#8827=VECTOR('',#66852,10.) ;
#8828=VECTOR('',#66855,10.) ;
#8829=VECTOR('',#66856,10.) ;
#8830=VECTOR('',#66861,10.) ;
#8831=VECTOR('',#66864,10.) ;
#8832=VECTOR('',#66865,10.) ;
#8833=VECTOR('',#66868,10.) ;
#8834=VECTOR('',#66869,10.) ;
#8835=VECTOR('',#66874,10.) ;
#8836=VECTOR('',#66877,10.) ;
#8837=VECTOR('',#66878,10.) ;
#8838=VECTOR('',#66883,10.) ;
#8839=VECTOR('',#66886,10.) ;
#8840=VECTOR('',#66887,10.) ;
#8841=VECTOR('',#66890,10.) ;
#8842=VECTOR('',#66891,10.) ;
#8843=VECTOR('',#66896,10.) ;
#8844=VECTOR('',#66899,10.) ;
#8845=VECTOR('',#66900,10.) ;
#8846=VECTOR('',#66905,10.) ;
#8847=VECTOR('',#66908,10.) ;
#8848=VECTOR('',#66913,10.) ;
#8849=VECTOR('',#66914,10.) ;
#8850=VECTOR('',#66915,10.) ;
#8851=VECTOR('',#66918,10.) ;
#8852=VECTOR('',#66919,10.) ;
#8853=VECTOR('',#66924,10.) ;
#8854=VECTOR('',#66927,10.) ;
#8855=VECTOR('',#66928,10.) ;
#8856=VECTOR('',#66935,10.) ;
#8857=VECTOR('',#66938,10.) ;
#8858=VECTOR('',#66939,10.) ;
#8859=VECTOR('',#66942,10.) ;
#8860=VECTOR('',#66943,10.) ;
#8861=VECTOR('',#66948,10.) ;
#8862=VECTOR('',#66951,10.) ;
#8863=VECTOR('',#66952,10.) ;
#8864=VECTOR('',#66957,10.) ;
#8865=VECTOR('',#66960,10.) ;
#8866=VECTOR('',#66967,10.) ;
#8867=VECTOR('',#66970,10.) ;
#8868=VECTOR('',#66971,10.) ;
#8869=VECTOR('',#66974,10.) ;
#8870=VECTOR('',#66975,10.) ;
#8871=VECTOR('',#66978,10.) ;
#8872=VECTOR('',#66979,10.) ;
#8873=VECTOR('',#66982,10.) ;
#8874=VECTOR('',#66983,10.) ;
#8875=VECTOR('',#66986,10.) ;
#8876=VECTOR('',#66987,10.) ;
#8877=VECTOR('',#66992,10.) ;
#8878=VECTOR('',#66997,10.) ;
#8879=VECTOR('',#67002,10.) ;
#8880=VECTOR('',#67005,10.) ;
#8881=VECTOR('',#67006,10.) ;
#8882=VECTOR('',#67009,10.) ;
#8883=VECTOR('',#67010,10.) ;
#8884=VECTOR('',#67015,10.) ;
#8885=VECTOR('',#67018,10.) ;
#8886=VECTOR('',#67019,10.) ;
#8887=VECTOR('',#67024,10.) ;
#8888=VECTOR('',#67027,10.) ;
#8889=VECTOR('',#67034,10.) ;
#8890=VECTOR('',#67037,10.) ;
#8891=VECTOR('',#67038,10.) ;
#8892=VECTOR('',#67043,10.) ;
#8893=VECTOR('',#67046,10.) ;
#8894=VECTOR('',#67047,10.) ;
#8895=VECTOR('',#67052,10.) ;
#8896=VECTOR('',#67055,10.) ;
#8897=VECTOR('',#67064,10.) ;
#8898=VECTOR('',#67067,10.) ;
#8899=VECTOR('',#67068,10.) ;
#8900=VECTOR('',#67073,10.) ;
#8901=VECTOR('',#67074,10.) ;
#8902=VECTOR('',#67077,10.) ;
#8903=VECTOR('',#67078,10.) ;
#8904=VECTOR('',#67081,10.) ;
#8905=VECTOR('',#67084,10.) ;
#8906=VECTOR('',#67085,10.) ;
#8907=VECTOR('',#67090,10.) ;
#8908=VECTOR('',#67093,10.) ;
#8909=VECTOR('',#67096,10.) ;
#8910=VECTOR('',#67099,10.) ;
#8911=VECTOR('',#67102,10.) ;
#8912=VECTOR('',#67113,10.) ;
#8913=VECTOR('',#67118,10.) ;
#8914=VECTOR('',#67121,10.) ;
#8915=VECTOR('',#67126,10.) ;
#8916=VECTOR('',#67131,10.) ;
#8917=VECTOR('',#67136,10.) ;
#8918=VECTOR('',#67143,10.) ;
#8919=VECTOR('',#67148,2.) ;
#8920=VECTOR('',#67151,10.) ;
#8921=VECTOR('',#67154,10.) ;
#8922=VECTOR('',#67157,10.) ;
#8923=VECTOR('',#67160,10.) ;
#8924=VECTOR('',#67165,10.) ;
#8925=VECTOR('',#67170,10.) ;
#8926=VECTOR('',#67171,10.) ;
#10134=CYLINDRICAL_SURFACE('',#52561,0.24) ;
#10135=CYLINDRICAL_SURFACE('',#52566,0.24) ;
#10136=CYLINDRICAL_SURFACE('',#52570,0.4) ;
#10137=CYLINDRICAL_SURFACE('',#52576,0.24) ;
#10138=CYLINDRICAL_SURFACE('',#52581,0.24) ;
#10139=CYLINDRICAL_SURFACE('',#52587,0.4) ;
#10140=CYLINDRICAL_SURFACE('',#52602,0.24) ;
#10141=CYLINDRICAL_SURFACE('',#52607,0.3) ;
#10142=CYLINDRICAL_SURFACE('',#52611,0.1) ;
#10143=CYLINDRICAL_SURFACE('',#52618,0.24) ;
#10144=CYLINDRICAL_SURFACE('',#52627,0.1) ;
#10145=CYLINDRICAL_SURFACE('',#52629,0.1) ;
#10146=CYLINDRICAL_SURFACE('',#52634,0.24) ;
#10147=CYLINDRICAL_SURFACE('',#52636,0.24) ;
#10148=CYLINDRICAL_SURFACE('',#52644,0.1) ;
#10149=CYLINDRICAL_SURFACE('',#52646,0.24) ;
#10150=CYLINDRICAL_SURFACE('',#52653,0.24) ;
#10151=CYLINDRICAL_SURFACE('',#52656,0.2) ;
#10152=CYLINDRICAL_SURFACE('',#52664,0.24) ;
#10153=CYLINDRICAL_SURFACE('',#52665,0.1) ;
#10154=CYLINDRICAL_SURFACE('',#52674,0.24) ;
#10155=CYLINDRICAL_SURFACE('',#52675,0.1) ;
#10156=CYLINDRICAL_SURFACE('',#52684,0.3) ;
#10157=CYLINDRICAL_SURFACE('',#52689,0.3) ;
#10158=CYLINDRICAL_SURFACE('',#52695,0.3) ;
#10159=CYLINDRICAL_SURFACE('',#52697,0.1) ;
#10160=CYLINDRICAL_SURFACE('',#52702,0.75) ;
#10161=CYLINDRICAL_SURFACE('',#52707,0.1) ;
#10162=CYLINDRICAL_SURFACE('',#52713,0.1) ;
#10163=CYLINDRICAL_SURFACE('',#52723,0.1) ;
#10164=CYLINDRICAL_SURFACE('',#52729,0.1) ;
#10165=CYLINDRICAL_SURFACE('',#52730,0.1) ;
#10166=CYLINDRICAL_SURFACE('',#52741,0.1) ;
#10167=CYLINDRICAL_SURFACE('',#52744,0.1) ;
#10168=CYLINDRICAL_SURFACE('',#52748,1.50000000000013) ;
#10169=CYLINDRICAL_SURFACE('',#52751,0.1) ;
#10170=CYLINDRICAL_SURFACE('',#52759,0.1) ;
#10171=CYLINDRICAL_SURFACE('',#52763,0.1) ;
#10172=CYLINDRICAL_SURFACE('',#52769,0.1) ;
#10173=CYLINDRICAL_SURFACE('',#52777,0.1) ;
#10174=CYLINDRICAL_SURFACE('',#52782,0.1) ;
#10175=CYLINDRICAL_SURFACE('',#52788,0.1) ;
#10176=CYLINDRICAL_SURFACE('',#52793,0.700000000000003) ;
#10177=CYLINDRICAL_SURFACE('',#52796,3.89999999999982) ;
#10178=CYLINDRICAL_SURFACE('',#52799,3.89999999999997) ;
#10179=CYLINDRICAL_SURFACE('',#52801,0.1) ;
#10180=CYLINDRICAL_SURFACE('',#52807,0.1) ;
#10181=CYLINDRICAL_SURFACE('',#52817,0.4) ;
#10182=CYLINDRICAL_SURFACE('',#52822,0.1) ;
#10183=CYLINDRICAL_SURFACE('',#52824,0.1) ;
#10184=CYLINDRICAL_SURFACE('',#52828,0.1) ;
#10185=CYLINDRICAL_SURFACE('',#52830,0.1) ;
#10186=CYLINDRICAL_SURFACE('',#52831,2.) ;
#10187=CYLINDRICAL_SURFACE('',#52842,0.1) ;
#10188=CYLINDRICAL_SURFACE('',#52844,0.1) ;
#10189=CYLINDRICAL_SURFACE('',#52846,0.1) ;
#10190=CYLINDRICAL_SURFACE('',#52852,0.1) ;
#10191=CYLINDRICAL_SURFACE('',#52853,0.1) ;
#10192=CYLINDRICAL_SURFACE('',#52859,0.1) ;
#10193=CYLINDRICAL_SURFACE('',#52860,0.1) ;
#10194=CYLINDRICAL_SURFACE('',#52861,0.1) ;
#10195=CYLINDRICAL_SURFACE('',#52930,0.1) ;
#10196=CYLINDRICAL_SURFACE('',#52936,0.1) ;
#10197=CYLINDRICAL_SURFACE('',#52938,2.9) ;
#10198=CYLINDRICAL_SURFACE('',#52939,3.99999999999997) ;
#10199=CYLINDRICAL_SURFACE('',#52947,0.1) ;
#10200=CYLINDRICAL_SURFACE('',#52953,0.1) ;
#10201=CYLINDRICAL_SURFACE('',#52959,0.1) ;
#10202=CYLINDRICAL_SURFACE('',#52960,0.1) ;
#10203=CYLINDRICAL_SURFACE('',#52966,0.1) ;
#10204=CYLINDRICAL_SURFACE('',#52976,0.1) ;
#10205=CYLINDRICAL_SURFACE('',#52981,0.1) ;
#10206=CYLINDRICAL_SURFACE('',#52982,0.1) ;
#10207=CYLINDRICAL_SURFACE('',#52983,0.1) ;
#10208=CYLINDRICAL_SURFACE('',#52988,0.1) ;
#10209=CYLINDRICAL_SURFACE('',#52994,0.599999999999915) ;
#10210=CYLINDRICAL_SURFACE('',#52997,1.) ;
#10211=CYLINDRICAL_SURFACE('',#53003,0.499999999999901) ;
#10212=CYLINDRICAL_SURFACE('',#53006,0.200000000000106) ;
#10213=CYLINDRICAL_SURFACE('',#53008,0.999999999999996) ;
#10214=CYLINDRICAL_SURFACE('',#53013,0.1) ;
#10215=CYLINDRICAL_SURFACE('',#53020,0.1) ;
#10216=CYLINDRICAL_SURFACE('',#53036,0.1) ;
#10217=CYLINDRICAL_SURFACE('',#53037,0.1) ;
#10218=CYLINDRICAL_SURFACE('',#53042,0.1) ;
#10219=CYLINDRICAL_SURFACE('',#53043,0.1) ;
#10220=CYLINDRICAL_SURFACE('',#53048,0.1) ;
#10221=CYLINDRICAL_SURFACE('',#53053,0.1) ;
#10222=CYLINDRICAL_SURFACE('',#53054,0.1) ;
#10223=CYLINDRICAL_SURFACE('',#53056,0.1) ;
#10224=CYLINDRICAL_SURFACE('',#53062,0.1) ;
#10225=CYLINDRICAL_SURFACE('',#53068,0.1) ;
#10226=CYLINDRICAL_SURFACE('',#53074,0.1) ;
#10227=CYLINDRICAL_SURFACE('',#53080,0.1) ;
#10228=CYLINDRICAL_SURFACE('',#53081,0.1) ;
#10229=CYLINDRICAL_SURFACE('',#53085,0.1) ;
#10230=CYLINDRICAL_SURFACE('',#53087,0.5) ;
#10231=CYLINDRICAL_SURFACE('',#53089,0.5) ;
#10232=CYLINDRICAL_SURFACE('',#53090,0.4) ;
#10233=CYLINDRICAL_SURFACE('',#53092,0.199999999999996) ;
#10234=CYLINDRICAL_SURFACE('',#53094,0.200000000000031) ;
#10235=CYLINDRICAL_SURFACE('',#53095,0.4) ;
#10236=CYLINDRICAL_SURFACE('',#53103,0.1) ;
#10237=CYLINDRICAL_SURFACE('',#53107,0.1) ;
#10238=CYLINDRICAL_SURFACE('',#53120,0.1) ;
#10239=CYLINDRICAL_SURFACE('',#53121,0.1) ;
#10240=CYLINDRICAL_SURFACE('',#53128,0.1) ;
#10241=CYLINDRICAL_SURFACE('',#53129,0.1) ;
#10242=CYLINDRICAL_SURFACE('',#53131,0.1) ;
#10243=CYLINDRICAL_SURFACE('',#53133,0.1) ;
#10244=CYLINDRICAL_SURFACE('',#53139,0.1) ;
#10245=CYLINDRICAL_SURFACE('',#53141,0.500000000000007) ;
#10246=CYLINDRICAL_SURFACE('',#53148,0.500000000000007) ;
#10247=CYLINDRICAL_SURFACE('',#53151,0.1) ;
#10248=CYLINDRICAL_SURFACE('',#53156,0.1) ;
#10249=CYLINDRICAL_SURFACE('',#53160,0.1) ;
#10250=CYLINDRICAL_SURFACE('',#53165,0.1) ;
#10251=CYLINDRICAL_SURFACE('',#53170,0.1) ;
#10252=CYLINDRICAL_SURFACE('',#53175,0.1) ;
#10253=CYLINDRICAL_SURFACE('',#53180,0.1) ;
#10254=CYLINDRICAL_SURFACE('',#53184,0.1) ;
#10255=CYLINDRICAL_SURFACE('',#53193,0.1) ;
#10256=CYLINDRICAL_SURFACE('',#53198,0.1) ;
#10257=CYLINDRICAL_SURFACE('',#53206,0.1) ;
#10258=CYLINDRICAL_SURFACE('',#53210,0.1) ;
#10259=CYLINDRICAL_SURFACE('',#53215,1.50000000000004) ;
#10260=CYLINDRICAL_SURFACE('',#53218,1.) ;
#10261=CYLINDRICAL_SURFACE('',#53219,0.600000000000129) ;
#10262=CYLINDRICAL_SURFACE('',#53221,0.600000000000129) ;
#10263=CYLINDRICAL_SURFACE('',#53222,0.1) ;
#10264=CYLINDRICAL_SURFACE('',#53224,0.1) ;
#10265=CYLINDRICAL_SURFACE('',#53226,0.1) ;
#10266=CYLINDRICAL_SURFACE('',#53231,0.1) ;
#10267=CYLINDRICAL_SURFACE('',#53235,0.1) ;
#10268=CYLINDRICAL_SURFACE('',#53240,0.1) ;
#10269=CYLINDRICAL_SURFACE('',#53244,0.1) ;
#10270=CYLINDRICAL_SURFACE('',#53249,0.1) ;
#10271=CYLINDRICAL_SURFACE('',#53251,0.1) ;
#10272=CYLINDRICAL_SURFACE('',#53258,0.1) ;
#10273=CYLINDRICAL_SURFACE('',#53263,0.1) ;
#10274=CYLINDRICAL_SURFACE('',#53268,0.1) ;
#10275=CYLINDRICAL_SURFACE('',#53271,0.75) ;
#10276=CYLINDRICAL_SURFACE('',#53276,0.5) ;
#10277=CYLINDRICAL_SURFACE('',#53283,0.4) ;
#10278=CYLINDRICAL_SURFACE('',#53295,0.1) ;
#10279=CYLINDRICAL_SURFACE('',#53302,0.1) ;
#10280=CYLINDRICAL_SURFACE('',#53303,0.1) ;
#10281=CYLINDRICAL_SURFACE('',#53305,0.1) ;
#10282=CYLINDRICAL_SURFACE('',#53306,0.1) ;
#10283=CYLINDRICAL_SURFACE('',#53308,0.1) ;
#10284=CYLINDRICAL_SURFACE('',#53312,0.4) ;
#10285=CYLINDRICAL_SURFACE('',#53315,0.75) ;
#10286=CYLINDRICAL_SURFACE('',#53318,0.75) ;
#10287=CYLINDRICAL_SURFACE('',#53321,0.1) ;
#10288=CYLINDRICAL_SURFACE('',#53324,0.1) ;
#10289=CYLINDRICAL_SURFACE('',#53331,0.2) ;
#10290=CYLINDRICAL_SURFACE('',#53338,0.2) ;
#10291=CYLINDRICAL_SURFACE('',#53339,0.5) ;
#10292=CYLINDRICAL_SURFACE('',#53344,0.2) ;
#10293=CYLINDRICAL_SURFACE('',#53357,0.75) ;
#10294=CYLINDRICAL_SURFACE('',#53361,0.2) ;
#10295=CYLINDRICAL_SURFACE('',#53365,0.2) ;
#10296=CYLINDRICAL_SURFACE('',#53366,0.2) ;
#10297=CYLINDRICAL_SURFACE('',#53371,0.2) ;
#10298=CYLINDRICAL_SURFACE('',#53376,0.75) ;
#10299=CYLINDRICAL_SURFACE('',#53377,6.15) ;
#10300=CYLINDRICAL_SURFACE('',#53381,0.75) ;
#10301=CYLINDRICAL_SURFACE('',#53383,0.75) ;
#10302=CYLINDRICAL_SURFACE('',#53385,3.6) ;
#10303=CYLINDRICAL_SURFACE('',#53388,3.6) ;
#10304=CYLINDRICAL_SURFACE('',#53391,3.6) ;
#10305=CYLINDRICAL_SURFACE('',#53402,0.1) ;
#10306=CYLINDRICAL_SURFACE('',#53405,0.1) ;
#10307=CYLINDRICAL_SURFACE('',#53415,0.1) ;
#10308=CYLINDRICAL_SURFACE('',#53417,0.1) ;
#10309=CYLINDRICAL_SURFACE('',#53418,0.1) ;
#10310=CYLINDRICAL_SURFACE('',#53420,0.1) ;
#10311=CYLINDRICAL_SURFACE('',#53422,0.1) ;
#10312=CYLINDRICAL_SURFACE('',#53428,0.1) ;
#10313=CYLINDRICAL_SURFACE('',#53430,0.1) ;
#10314=CYLINDRICAL_SURFACE('',#53432,0.1) ;
#10315=CYLINDRICAL_SURFACE('',#53434,0.1) ;
#10316=CYLINDRICAL_SURFACE('',#53435,0.1) ;
#10317=CYLINDRICAL_SURFACE('',#53439,0.1) ;
#10318=CYLINDRICAL_SURFACE('',#53442,0.1) ;
#10319=CYLINDRICAL_SURFACE('',#53444,0.1) ;
#10320=CYLINDRICAL_SURFACE('',#53446,0.1) ;
#10321=CYLINDRICAL_SURFACE('',#53448,0.1) ;
#10322=CYLINDRICAL_SURFACE('',#53450,0.1) ;
#10323=CYLINDRICAL_SURFACE('',#53452,0.1) ;
#10324=CYLINDRICAL_SURFACE('',#53458,0.1) ;
#10325=CYLINDRICAL_SURFACE('',#53461,0.1) ;
#10326=CYLINDRICAL_SURFACE('',#53463,0.1) ;
#10327=CYLINDRICAL_SURFACE('',#53465,0.1) ;
#10328=CYLINDRICAL_SURFACE('',#53469,0.1) ;
#10329=CYLINDRICAL_SURFACE('',#53472,0.1) ;
#10330=CYLINDRICAL_SURFACE('',#53474,0.1) ;
#10331=CYLINDRICAL_SURFACE('',#53476,0.1) ;
#10332=CYLINDRICAL_SURFACE('',#53478,0.1) ;
#10333=CYLINDRICAL_SURFACE('',#53480,0.1) ;
#10334=CYLINDRICAL_SURFACE('',#53482,0.1) ;
#10335=CYLINDRICAL_SURFACE('',#53488,0.1) ;
#10336=CYLINDRICAL_SURFACE('',#53491,0.1) ;
#10337=CYLINDRICAL_SURFACE('',#53493,0.1) ;
#10338=CYLINDRICAL_SURFACE('',#53495,0.1) ;
#10339=CYLINDRICAL_SURFACE('',#53499,0.1) ;
#10340=CYLINDRICAL_SURFACE('',#53502,0.1) ;
#10341=CYLINDRICAL_SURFACE('',#53504,0.1) ;
#10342=CYLINDRICAL_SURFACE('',#53510,0.1) ;
#10343=CYLINDRICAL_SURFACE('',#53512,0.1) ;
#10344=CYLINDRICAL_SURFACE('',#53514,0.1) ;
#10345=CYLINDRICAL_SURFACE('',#53520,0.1) ;
#10346=CYLINDRICAL_SURFACE('',#53522,0.1) ;
#10347=CYLINDRICAL_SURFACE('',#53524,0.1) ;
#10348=CYLINDRICAL_SURFACE('',#53526,0.299999999999963) ;
#10349=CYLINDRICAL_SURFACE('',#53533,0.1) ;
#10350=CYLINDRICAL_SURFACE('',#53536,0.1) ;
#10351=CYLINDRICAL_SURFACE('',#53542,0.1) ;
#10352=CYLINDRICAL_SURFACE('',#53544,0.1) ;
#10353=CYLINDRICAL_SURFACE('',#53546,0.1) ;
#10354=CYLINDRICAL_SURFACE('',#53552,0.1) ;
#10355=CYLINDRICAL_SURFACE('',#53554,0.1) ;
#10356=CYLINDRICAL_SURFACE('',#53556,0.1) ;
#10357=CYLINDRICAL_SURFACE('',#53558,0.1) ;
#10358=CYLINDRICAL_SURFACE('',#53559,0.299999999999963) ;
#10359=CYLINDRICAL_SURFACE('',#53567,0.1) ;
#10360=CYLINDRICAL_SURFACE('',#53568,0.1) ;
#10361=CYLINDRICAL_SURFACE('',#53570,0.1) ;
#10362=CYLINDRICAL_SURFACE('',#53572,0.1) ;
#10363=CYLINDRICAL_SURFACE('',#53574,0.1) ;
#10364=CYLINDRICAL_SURFACE('',#53576,0.1) ;
#10365=CYLINDRICAL_SURFACE('',#53578,0.1) ;
#10366=CYLINDRICAL_SURFACE('',#53581,0.1) ;
#10367=CYLINDRICAL_SURFACE('',#53582,0.1) ;
#10368=CYLINDRICAL_SURFACE('',#53583,0.1) ;
#10369=CYLINDRICAL_SURFACE('',#53586,0.1) ;
#10370=CYLINDRICAL_SURFACE('',#53589,0.1) ;
#10371=CYLINDRICAL_SURFACE('',#53591,0.1) ;
#10372=CYLINDRICAL_SURFACE('',#53593,0.1) ;
#10373=CYLINDRICAL_SURFACE('',#53595,0.1) ;
#10374=CYLINDRICAL_SURFACE('',#53597,0.1) ;
#10375=CYLINDRICAL_SURFACE('',#53599,0.1) ;
#10376=CYLINDRICAL_SURFACE('',#53609,0.1) ;
#10377=CYLINDRICAL_SURFACE('',#53612,0.1) ;
#10378=CYLINDRICAL_SURFACE('',#53614,0.1) ;
#10379=CYLINDRICAL_SURFACE('',#53616,0.1) ;
#10380=CYLINDRICAL_SURFACE('',#53618,0.1) ;
#10381=CYLINDRICAL_SURFACE('',#53621,0.1) ;
#10382=CYLINDRICAL_SURFACE('',#53623,0.1) ;
#10383=CYLINDRICAL_SURFACE('',#53625,0.1) ;
#10384=CYLINDRICAL_SURFACE('',#53627,0.1) ;
#10385=CYLINDRICAL_SURFACE('',#53629,0.1) ;
#10386=CYLINDRICAL_SURFACE('',#53631,0.1) ;
#10387=CYLINDRICAL_SURFACE('',#53634,0.1) ;
#10388=CYLINDRICAL_SURFACE('',#53637,0.1) ;
#10389=CYLINDRICAL_SURFACE('',#53639,0.1) ;
#10390=CYLINDRICAL_SURFACE('',#53641,0.1) ;
#10391=CYLINDRICAL_SURFACE('',#53642,0.1) ;
#10392=CYLINDRICAL_SURFACE('',#53645,0.1) ;
#10393=CYLINDRICAL_SURFACE('',#53647,0.1) ;
#10394=CYLINDRICAL_SURFACE('',#53649,0.1) ;
#10395=CYLINDRICAL_SURFACE('',#53651,0.1) ;
#10396=CYLINDRICAL_SURFACE('',#53653,0.1) ;
#10397=CYLINDRICAL_SURFACE('',#53658,0.1) ;
#10398=CYLINDRICAL_SURFACE('',#53662,0.1) ;
#10399=CYLINDRICAL_SURFACE('',#53665,0.699999999999972) ;
#10400=CYLINDRICAL_SURFACE('',#53668,0.1) ;
#10401=CYLINDRICAL_SURFACE('',#53671,0.1) ;
#10402=CYLINDRICAL_SURFACE('',#53674,0.1) ;
#10403=CYLINDRICAL_SURFACE('',#53676,0.1) ;
#10404=CYLINDRICAL_SURFACE('',#53678,0.1) ;
#10405=CYLINDRICAL_SURFACE('',#53680,0.1) ;
#10406=CYLINDRICAL_SURFACE('',#53685,0.1) ;
#10407=CYLINDRICAL_SURFACE('',#53686,0.1) ;
#10408=CYLINDRICAL_SURFACE('',#53690,0.1) ;
#10409=CYLINDRICAL_SURFACE('',#53694,0.699999999999972) ;
#10410=CYLINDRICAL_SURFACE('',#53707,2.99999999999998) ;
#10411=CYLINDRICAL_SURFACE('',#53710,1.60000000000004) ;
#10412=CYLINDRICAL_SURFACE('',#53717,0.500000000000043) ;
#10413=CYLINDRICAL_SURFACE('',#53728,1.5) ;
#10414=CYLINDRICAL_SURFACE('',#53733,0.399999999999992) ;
#10415=CYLINDRICAL_SURFACE('',#53740,0.4) ;
#10416=CYLINDRICAL_SURFACE('',#53743,0.4) ;
#10417=CYLINDRICAL_SURFACE('',#53749,0.5) ;
#10418=CYLINDRICAL_SURFACE('',#53758,0.5) ;
#10419=CYLINDRICAL_SURFACE('',#53764,0.5) ;
#10420=CYLINDRICAL_SURFACE('',#53765,0.5) ;
#10421=CYLINDRICAL_SURFACE('',#53771,0.5) ;
#10422=CYLINDRICAL_SURFACE('',#53777,0.5) ;
#10423=CYLINDRICAL_SURFACE('',#53787,0.5) ;
#10424=CYLINDRICAL_SURFACE('',#53790,0.5) ;
#10425=CYLINDRICAL_SURFACE('',#53795,0.5) ;
#10426=CYLINDRICAL_SURFACE('',#53801,0.5) ;
#10427=CYLINDRICAL_SURFACE('',#53802,0.5) ;
#10428=CYLINDRICAL_SURFACE('',#53807,0.5) ;
#10429=CYLINDRICAL_SURFACE('',#53816,0.5) ;
#10430=CYLINDRICAL_SURFACE('',#53818,0.5) ;
#10431=CYLINDRICAL_SURFACE('',#53823,0.5) ;
#10432=CYLINDRICAL_SURFACE('',#53825,4.06491106406736) ;
#10433=CYLINDRICAL_SURFACE('',#53827,1.) ;
#10434=CYLINDRICAL_SURFACE('',#53830,0.500000000000043) ;
#10435=CYLINDRICAL_SURFACE('',#53832,4.06491106406736) ;
#10436=CYLINDRICAL_SURFACE('',#53833,4.06491106406736) ;
#10437=CYLINDRICAL_SURFACE('',#53835,0.200000000000031) ;
#10438=CYLINDRICAL_SURFACE('',#53839,0.199999999999996) ;
#10439=CYLINDRICAL_SURFACE('',#53842,0.199999999999996) ;
#10440=CYLINDRICAL_SURFACE('',#53847,0.200000000000031) ;
#10441=CYLINDRICAL_SURFACE('',#53850,0.2) ;
#10442=CYLINDRICAL_SURFACE('',#53851,2.6) ;
#10443=CYLINDRICAL_SURFACE('',#53854,0.200000000000001) ;
#10444=CYLINDRICAL_SURFACE('',#53857,0.199999999999996) ;
#10445=CYLINDRICAL_SURFACE('',#53860,0.199999999999996) ;
#10446=CYLINDRICAL_SURFACE('',#53863,0.199999999999996) ;
#10447=CYLINDRICAL_SURFACE('',#53867,0.199999999999996) ;
#10448=CYLINDRICAL_SURFACE('',#53870,2.49999999999999) ;
#10449=CYLINDRICAL_SURFACE('',#53873,0.199999999999995) ;
#10450=CYLINDRICAL_SURFACE('',#53876,0.199999999999996) ;
#10451=CYLINDRICAL_SURFACE('',#53879,0.199999999999996) ;
#10452=CYLINDRICAL_SURFACE('',#53882,0.199999999999996) ;
#10453=CYLINDRICAL_SURFACE('',#53887,0.100000000000016) ;
#10454=CYLINDRICAL_SURFACE('',#53890,0.0999999999999979) ;
#10455=CYLINDRICAL_SURFACE('',#53893,0.100000000000051) ;
#10456=CYLINDRICAL_SURFACE('',#53895,0.199999999999996) ;
#10457=CYLINDRICAL_SURFACE('',#53898,0.199999999999996) ;
#10458=CYLINDRICAL_SURFACE('',#53902,0.199999999999996) ;
#10459=CYLINDRICAL_SURFACE('',#53905,0.199999999999996) ;
#10460=CYLINDRICAL_SURFACE('',#53909,0.199999999999996) ;
#10461=CYLINDRICAL_SURFACE('',#53912,0.199999999999996) ;
#10462=CYLINDRICAL_SURFACE('',#53918,0.199999999999995) ;
#10463=CYLINDRICAL_SURFACE('',#53921,0.199999999999996) ;
#10464=CYLINDRICAL_SURFACE('',#53926,0.199999999999996) ;
#10465=CYLINDRICAL_SURFACE('',#53929,0.200000000000031) ;
#10466=CYLINDRICAL_SURFACE('',#53933,0.199999999999996) ;
#10467=CYLINDRICAL_SURFACE('',#53940,0.200000000000031) ;
#10468=CYLINDRICAL_SURFACE('',#53944,0.199999999999996) ;
#10469=CYLINDRICAL_SURFACE('',#53948,0.199999999999996) ;
#10470=CYLINDRICAL_SURFACE('',#53951,0.199999999999996) ;
#10471=CYLINDRICAL_SURFACE('',#53955,0.0999999999999973) ;
#10472=CYLINDRICAL_SURFACE('',#53958,0.0999999999999979) ;
#10473=CYLINDRICAL_SURFACE('',#53961,0.100000000000004) ;
#10474=CYLINDRICAL_SURFACE('',#53966,0.199999999999996) ;
#10475=CYLINDRICAL_SURFACE('',#53977,0.500000000000114) ;
#10476=CYLINDRICAL_SURFACE('',#53979,0.500000000000025) ;
#10477=CYLINDRICAL_SURFACE('',#53984,0.199999999999996) ;
#10478=CYLINDRICAL_SURFACE('',#53986,4.49999999999997) ;
#10479=CYLINDRICAL_SURFACE('',#53992,1.) ;
#10480=CYLINDRICAL_SURFACE('',#53994,1.) ;
#10481=CYLINDRICAL_SURFACE('',#53997,1.) ;
#10482=CYLINDRICAL_SURFACE('',#53998,2.) ;
#10483=CYLINDRICAL_SURFACE('',#54000,4.06491106406736) ;
#10484=CYLINDRICAL_SURFACE('',#54002,4.05) ;
#10485=CYLINDRICAL_SURFACE('',#54005,4.05) ;
#12382=FACE_OUTER_BOUND('',#15542,.T.) ;
#12383=FACE_OUTER_BOUND('',#15543,.T.) ;
#12384=FACE_OUTER_BOUND('',#15544,.T.) ;
#12385=FACE_OUTER_BOUND('',#15545,.T.) ;
#12386=FACE_OUTER_BOUND('',#15546,.T.) ;
#12387=FACE_OUTER_BOUND('',#15547,.T.) ;
#12388=FACE_OUTER_BOUND('',#15548,.T.) ;
#12389=FACE_OUTER_BOUND('',#15549,.T.) ;
#12390=FACE_OUTER_BOUND('',#15550,.T.) ;
#12391=FACE_OUTER_BOUND('',#15551,.T.) ;
#12392=FACE_OUTER_BOUND('',#15552,.T.) ;
#12393=FACE_OUTER_BOUND('',#15553,.T.) ;
#12394=FACE_OUTER_BOUND('',#15554,.T.) ;
#12395=FACE_OUTER_BOUND('',#15555,.T.) ;
#12396=FACE_OUTER_BOUND('',#15556,.T.) ;
#12397=FACE_OUTER_BOUND('',#15557,.T.) ;
#12398=FACE_OUTER_BOUND('',#15558,.T.) ;
#12399=FACE_OUTER_BOUND('',#15559,.T.) ;
#12400=FACE_OUTER_BOUND('',#15560,.T.) ;
#12401=FACE_OUTER_BOUND('',#15561,.T.) ;
#12402=FACE_OUTER_BOUND('',#15562,.T.) ;
#12403=FACE_OUTER_BOUND('',#15563,.T.) ;
#12404=FACE_OUTER_BOUND('',#15564,.T.) ;
#12405=FACE_OUTER_BOUND('',#15565,.T.) ;
#12406=FACE_OUTER_BOUND('',#15566,.T.) ;
#12407=FACE_OUTER_BOUND('',#15567,.T.) ;
#12408=FACE_OUTER_BOUND('',#15568,.T.) ;
#12409=FACE_OUTER_BOUND('',#15569,.T.) ;
#12410=FACE_OUTER_BOUND('',#15570,.T.) ;
#12411=FACE_OUTER_BOUND('',#15571,.T.) ;
#12412=FACE_OUTER_BOUND('',#15572,.T.) ;
#12413=FACE_OUTER_BOUND('',#15573,.T.) ;
#12414=FACE_OUTER_BOUND('',#15574,.T.) ;
#12415=FACE_OUTER_BOUND('',#15576,.T.) ;
#12416=FACE_OUTER_BOUND('',#15579,.T.) ;
#12417=FACE_OUTER_BOUND('',#15580,.T.) ;
#12418=FACE_OUTER_BOUND('',#15581,.T.) ;
#12419=FACE_OUTER_BOUND('',#15582,.T.) ;
#12420=FACE_OUTER_BOUND('',#15583,.T.) ;
#12421=FACE_OUTER_BOUND('',#15584,.T.) ;
#12422=FACE_OUTER_BOUND('',#15585,.T.) ;
#12423=FACE_OUTER_BOUND('',#15586,.T.) ;
#12424=FACE_OUTER_BOUND('',#15587,.T.) ;
#12425=FACE_OUTER_BOUND('',#15588,.T.) ;
#12426=FACE_OUTER_BOUND('',#15589,.T.) ;
#12427=FACE_OUTER_BOUND('',#15590,.T.) ;
#12428=FACE_OUTER_BOUND('',#15591,.T.) ;
#12429=FACE_OUTER_BOUND('',#15592,.T.) ;
#12430=FACE_OUTER_BOUND('',#15593,.T.) ;
#12431=FACE_OUTER_BOUND('',#15594,.T.) ;
#12432=FACE_OUTER_BOUND('',#15595,.T.) ;
#12433=FACE_OUTER_BOUND('',#15596,.T.) ;
#12434=FACE_OUTER_BOUND('',#15597,.T.) ;
#12435=FACE_OUTER_BOUND('',#15598,.T.) ;
#12436=FACE_OUTER_BOUND('',#15599,.T.) ;
#12437=FACE_OUTER_BOUND('',#15600,.T.) ;
#12438=FACE_OUTER_BOUND('',#15601,.T.) ;
#12439=FACE_OUTER_BOUND('',#15602,.T.) ;
#12440=FACE_OUTER_BOUND('',#15603,.T.) ;
#12441=FACE_OUTER_BOUND('',#15604,.T.) ;
#12442=FACE_OUTER_BOUND('',#15605,.T.) ;
#12443=FACE_OUTER_BOUND('',#15606,.T.) ;
#12444=FACE_OUTER_BOUND('',#15607,.T.) ;
#12445=FACE_OUTER_BOUND('',#15608,.T.) ;
#12446=FACE_OUTER_BOUND('',#15609,.T.) ;
#12447=FACE_OUTER_BOUND('',#15610,.T.) ;
#12448=FACE_OUTER_BOUND('',#15611,.T.) ;
#12449=FACE_OUTER_BOUND('',#15612,.T.) ;
#12450=FACE_OUTER_BOUND('',#15613,.T.) ;
#12451=FACE_OUTER_BOUND('',#15614,.T.) ;
#12452=FACE_OUTER_BOUND('',#15615,.T.) ;
#12453=FACE_OUTER_BOUND('',#15616,.T.) ;
#12454=FACE_OUTER_BOUND('',#15617,.T.) ;
#12455=FACE_OUTER_BOUND('',#15618,.T.) ;
#12456=FACE_OUTER_BOUND('',#15619,.T.) ;
#12457=FACE_OUTER_BOUND('',#15620,.T.) ;
#12458=FACE_OUTER_BOUND('',#15621,.T.) ;
#12459=FACE_OUTER_BOUND('',#15622,.T.) ;
#12460=FACE_OUTER_BOUND('',#15623,.T.) ;
#12461=FACE_OUTER_BOUND('',#15624,.T.) ;
#12462=FACE_OUTER_BOUND('',#15625,.T.) ;
#12463=FACE_OUTER_BOUND('',#15626,.T.) ;
#12464=FACE_OUTER_BOUND('',#15627,.T.) ;
#12465=FACE_OUTER_BOUND('',#15628,.T.) ;
#12466=FACE_OUTER_BOUND('',#15629,.T.) ;
#12467=FACE_OUTER_BOUND('',#15630,.T.) ;
#12468=FACE_OUTER_BOUND('',#15631,.T.) ;
#12469=FACE_OUTER_BOUND('',#15632,.T.) ;
#12470=FACE_OUTER_BOUND('',#15633,.T.) ;
#12471=FACE_OUTER_BOUND('',#15634,.T.) ;
#12472=FACE_OUTER_BOUND('',#15635,.T.) ;
#12473=FACE_OUTER_BOUND('',#15636,.T.) ;
#12474=FACE_OUTER_BOUND('',#15637,.T.) ;
#12475=FACE_OUTER_BOUND('',#15638,.T.) ;
#12476=FACE_OUTER_BOUND('',#15639,.T.) ;
#12477=FACE_OUTER_BOUND('',#15640,.T.) ;
#12478=FACE_OUTER_BOUND('',#15641,.T.) ;
#12479=FACE_OUTER_BOUND('',#15642,.T.) ;
#12480=FACE_OUTER_BOUND('',#15643,.T.) ;
#12481=FACE_OUTER_BOUND('',#15644,.T.) ;
#12482=FACE_OUTER_BOUND('',#15645,.T.) ;
#12483=FACE_OUTER_BOUND('',#15646,.T.) ;
#12484=FACE_OUTER_BOUND('',#15647,.T.) ;
#12485=FACE_OUTER_BOUND('',#15648,.T.) ;
#12486=FACE_OUTER_BOUND('',#15649,.T.) ;
#12487=FACE_OUTER_BOUND('',#15650,.T.) ;
#12488=FACE_OUTER_BOUND('',#15651,.T.) ;
#12489=FACE_OUTER_BOUND('',#15652,.T.) ;
#12490=FACE_OUTER_BOUND('',#15653,.T.) ;
#12491=FACE_OUTER_BOUND('',#15654,.T.) ;
#12492=FACE_OUTER_BOUND('',#15655,.T.) ;
#12493=FACE_OUTER_BOUND('',#15656,.T.) ;
#12494=FACE_OUTER_BOUND('',#15657,.T.) ;
#12495=FACE_OUTER_BOUND('',#15658,.T.) ;
#12496=FACE_OUTER_BOUND('',#15659,.T.) ;
#12497=FACE_OUTER_BOUND('',#15660,.T.) ;
#12498=FACE_OUTER_BOUND('',#15661,.T.) ;
#12499=FACE_OUTER_BOUND('',#15662,.T.) ;
#12500=FACE_OUTER_BOUND('',#15663,.T.) ;
#12501=FACE_OUTER_BOUND('',#15664,.T.) ;
#12502=FACE_OUTER_BOUND('',#15665,.T.) ;
#12503=FACE_OUTER_BOUND('',#15666,.T.) ;
#12504=FACE_OUTER_BOUND('',#15667,.T.) ;
#12505=FACE_OUTER_BOUND('',#15668,.T.) ;
#12506=FACE_OUTER_BOUND('',#15669,.T.) ;
#12507=FACE_OUTER_BOUND('',#15670,.T.) ;
#12508=FACE_OUTER_BOUND('',#15671,.T.) ;
#12509=FACE_OUTER_BOUND('',#15672,.T.) ;
#12510=FACE_OUTER_BOUND('',#15673,.T.) ;
#12511=FACE_OUTER_BOUND('',#15674,.T.) ;
#12512=FACE_OUTER_BOUND('',#15675,.T.) ;
#12513=FACE_OUTER_BOUND('',#15676,.T.) ;
#12514=FACE_OUTER_BOUND('',#15677,.T.) ;
#12515=FACE_OUTER_BOUND('',#15678,.T.) ;
#12516=FACE_OUTER_BOUND('',#15679,.T.) ;
#12517=FACE_OUTER_BOUND('',#15680,.T.) ;
#12518=FACE_OUTER_BOUND('',#15681,.T.) ;
#12519=FACE_OUTER_BOUND('',#15682,.T.) ;
#12520=FACE_OUTER_BOUND('',#15683,.T.) ;
#12521=FACE_OUTER_BOUND('',#15684,.T.) ;
#12522=FACE_OUTER_BOUND('',#15685,.T.) ;
#12523=FACE_OUTER_BOUND('',#15686,.T.) ;
#12524=FACE_OUTER_BOUND('',#15687,.T.) ;
#12525=FACE_OUTER_BOUND('',#15688,.T.) ;
#12526=FACE_OUTER_BOUND('',#15689,.T.) ;
#12527=FACE_OUTER_BOUND('',#15690,.T.) ;
#12528=FACE_OUTER_BOUND('',#15691,.T.) ;
#12529=FACE_OUTER_BOUND('',#15692,.T.) ;
#12530=FACE_OUTER_BOUND('',#15693,.T.) ;
#12531=FACE_OUTER_BOUND('',#15694,.T.) ;
#12532=FACE_OUTER_BOUND('',#15695,.T.) ;
#12533=FACE_OUTER_BOUND('',#15696,.T.) ;
#12534=FACE_OUTER_BOUND('',#15697,.T.) ;
#12535=FACE_OUTER_BOUND('',#15698,.T.) ;
#12536=FACE_OUTER_BOUND('',#15699,.T.) ;
#12537=FACE_OUTER_BOUND('',#15700,.T.) ;
#12538=FACE_OUTER_BOUND('',#15701,.T.) ;
#12539=FACE_OUTER_BOUND('',#15702,.T.) ;
#12540=FACE_OUTER_BOUND('',#15703,.T.) ;
#12541=FACE_OUTER_BOUND('',#15704,.T.) ;
#12542=FACE_OUTER_BOUND('',#15705,.T.) ;
#12543=FACE_OUTER_BOUND('',#15706,.T.) ;
#12544=FACE_OUTER_BOUND('',#15707,.T.) ;
#12545=FACE_OUTER_BOUND('',#15708,.T.) ;
#12546=FACE_OUTER_BOUND('',#15709,.T.) ;
#12547=FACE_OUTER_BOUND('',#15710,.T.) ;
#12548=FACE_OUTER_BOUND('',#15711,.T.) ;
#12549=FACE_OUTER_BOUND('',#15712,.T.) ;
#12550=FACE_OUTER_BOUND('',#15713,.T.) ;
#12551=FACE_OUTER_BOUND('',#15714,.T.) ;
#12552=FACE_OUTER_BOUND('',#15715,.T.) ;
#12553=FACE_OUTER_BOUND('',#15716,.T.) ;
#12554=FACE_OUTER_BOUND('',#15717,.T.) ;
#12555=FACE_OUTER_BOUND('',#15725,.T.) ;
#12556=FACE_OUTER_BOUND('',#15726,.T.) ;
#12557=FACE_OUTER_BOUND('',#15727,.T.) ;
#12558=FACE_OUTER_BOUND('',#15728,.T.) ;
#12559=FACE_OUTER_BOUND('',#15729,.T.) ;
#12560=FACE_OUTER_BOUND('',#15730,.T.) ;
#12561=FACE_OUTER_BOUND('',#15731,.T.) ;
#12562=FACE_OUTER_BOUND('',#15732,.T.) ;
#12563=FACE_OUTER_BOUND('',#15733,.T.) ;
#12564=FACE_OUTER_BOUND('',#15734,.T.) ;
#12565=FACE_OUTER_BOUND('',#15735,.T.) ;
#12566=FACE_OUTER_BOUND('',#15736,.T.) ;
#12567=FACE_OUTER_BOUND('',#15737,.T.) ;
#12568=FACE_OUTER_BOUND('',#15738,.T.) ;
#12569=FACE_OUTER_BOUND('',#15739,.T.) ;
#12570=FACE_OUTER_BOUND('',#15740,.T.) ;
#12571=FACE_OUTER_BOUND('',#15741,.T.) ;
#12572=FACE_OUTER_BOUND('',#15742,.T.) ;
#12573=FACE_OUTER_BOUND('',#15743,.T.) ;
#12574=FACE_OUTER_BOUND('',#15744,.T.) ;
#12575=FACE_OUTER_BOUND('',#15745,.T.) ;
#12576=FACE_OUTER_BOUND('',#15746,.T.) ;
#12577=FACE_OUTER_BOUND('',#15747,.T.) ;
#12578=FACE_OUTER_BOUND('',#15748,.T.) ;
#12579=FACE_OUTER_BOUND('',#15749,.T.) ;
#12580=FACE_OUTER_BOUND('',#15750,.T.) ;
#12581=FACE_OUTER_BOUND('',#15751,.T.) ;
#12582=FACE_OUTER_BOUND('',#15752,.T.) ;
#12583=FACE_OUTER_BOUND('',#15753,.T.) ;
#12584=FACE_OUTER_BOUND('',#15754,.T.) ;
#12585=FACE_OUTER_BOUND('',#15755,.T.) ;
#12586=FACE_OUTER_BOUND('',#15756,.T.) ;
#12587=FACE_OUTER_BOUND('',#15757,.T.) ;
#12588=FACE_OUTER_BOUND('',#15758,.T.) ;
#12589=FACE_OUTER_BOUND('',#15759,.T.) ;
#12590=FACE_OUTER_BOUND('',#15760,.T.) ;
#12591=FACE_OUTER_BOUND('',#15761,.T.) ;
#12592=FACE_OUTER_BOUND('',#15762,.T.) ;
#12593=FACE_OUTER_BOUND('',#15763,.T.) ;
#12594=FACE_OUTER_BOUND('',#15764,.T.) ;
#12595=FACE_OUTER_BOUND('',#15765,.T.) ;
#12596=FACE_OUTER_BOUND('',#15766,.T.) ;
#12597=FACE_OUTER_BOUND('',#15767,.T.) ;
#12598=FACE_OUTER_BOUND('',#15768,.T.) ;
#12599=FACE_OUTER_BOUND('',#15769,.T.) ;
#12600=FACE_OUTER_BOUND('',#15770,.T.) ;
#12601=FACE_OUTER_BOUND('',#15771,.T.) ;
#12602=FACE_OUTER_BOUND('',#15772,.T.) ;
#12603=FACE_OUTER_BOUND('',#15773,.T.) ;
#12604=FACE_OUTER_BOUND('',#15774,.T.) ;
#12605=FACE_OUTER_BOUND('',#15775,.T.) ;
#12606=FACE_OUTER_BOUND('',#15776,.T.) ;
#12607=FACE_OUTER_BOUND('',#15777,.T.) ;
#12608=FACE_OUTER_BOUND('',#15778,.T.) ;
#12609=FACE_OUTER_BOUND('',#15779,.T.) ;
#12610=FACE_OUTER_BOUND('',#15780,.T.) ;
#12611=FACE_OUTER_BOUND('',#15781,.T.) ;
#12612=FACE_OUTER_BOUND('',#15782,.T.) ;
#12613=FACE_OUTER_BOUND('',#15783,.T.) ;
#12614=FACE_OUTER_BOUND('',#15784,.T.) ;
#12615=FACE_OUTER_BOUND('',#15785,.T.) ;
#12616=FACE_OUTER_BOUND('',#15786,.T.) ;
#12617=FACE_OUTER_BOUND('',#15787,.T.) ;
#12618=FACE_OUTER_BOUND('',#15788,.T.) ;
#12619=FACE_OUTER_BOUND('',#15789,.T.) ;
#12620=FACE_OUTER_BOUND('',#15790,.T.) ;
#12621=FACE_OUTER_BOUND('',#15791,.T.) ;
#12622=FACE_OUTER_BOUND('',#15792,.T.) ;
#12623=FACE_OUTER_BOUND('',#15793,.T.) ;
#12624=FACE_OUTER_BOUND('',#15794,.T.) ;
#12625=FACE_OUTER_BOUND('',#15795,.T.) ;
#12626=FACE_OUTER_BOUND('',#15796,.T.) ;
#12627=FACE_OUTER_BOUND('',#15797,.T.) ;
#12628=FACE_OUTER_BOUND('',#15798,.T.) ;
#12629=FACE_OUTER_BOUND('',#15799,.T.) ;
#12630=FACE_OUTER_BOUND('',#15800,.T.) ;
#12631=FACE_OUTER_BOUND('',#15801,.T.) ;
#12632=FACE_OUTER_BOUND('',#15802,.T.) ;
#12633=FACE_OUTER_BOUND('',#15803,.T.) ;
#12634=FACE_OUTER_BOUND('',#15804,.T.) ;
#12635=FACE_OUTER_BOUND('',#15805,.T.) ;
#12636=FACE_OUTER_BOUND('',#15806,.T.) ;
#12637=FACE_OUTER_BOUND('',#15807,.T.) ;
#12638=FACE_OUTER_BOUND('',#15808,.T.) ;
#12639=FACE_OUTER_BOUND('',#15809,.T.) ;
#12640=FACE_OUTER_BOUND('',#15810,.T.) ;
#12641=FACE_OUTER_BOUND('',#15811,.T.) ;
#12642=FACE_OUTER_BOUND('',#15812,.T.) ;
#12643=FACE_OUTER_BOUND('',#15813,.T.) ;
#12644=FACE_OUTER_BOUND('',#15814,.T.) ;
#12645=FACE_OUTER_BOUND('',#15815,.T.) ;
#12646=FACE_OUTER_BOUND('',#15816,.T.) ;
#12647=FACE_OUTER_BOUND('',#15817,.T.) ;
#12648=FACE_OUTER_BOUND('',#15818,.T.) ;
#12649=FACE_OUTER_BOUND('',#15819,.T.) ;
#12650=FACE_OUTER_BOUND('',#15820,.T.) ;
#12651=FACE_OUTER_BOUND('',#15821,.T.) ;
#12652=FACE_OUTER_BOUND('',#15822,.T.) ;
#12653=FACE_OUTER_BOUND('',#15823,.T.) ;
#12654=FACE_OUTER_BOUND('',#15824,.T.) ;
#12655=FACE_OUTER_BOUND('',#15825,.T.) ;
#12656=FACE_OUTER_BOUND('',#15826,.T.) ;
#12657=FACE_OUTER_BOUND('',#15827,.T.) ;
#12658=FACE_OUTER_BOUND('',#15828,.T.) ;
#12659=FACE_OUTER_BOUND('',#15829,.T.) ;
#12660=FACE_OUTER_BOUND('',#15830,.T.) ;
#12661=FACE_OUTER_BOUND('',#15831,.T.) ;
#12662=FACE_OUTER_BOUND('',#15832,.T.) ;
#12663=FACE_OUTER_BOUND('',#15833,.T.) ;
#12664=FACE_OUTER_BOUND('',#15834,.T.) ;
#12665=FACE_OUTER_BOUND('',#15835,.T.) ;
#12666=FACE_OUTER_BOUND('',#15836,.T.) ;
#12667=FACE_OUTER_BOUND('',#15837,.T.) ;
#12668=FACE_OUTER_BOUND('',#15838,.T.) ;
#12669=FACE_OUTER_BOUND('',#15839,.T.) ;
#12670=FACE_OUTER_BOUND('',#15840,.T.) ;
#12671=FACE_OUTER_BOUND('',#15841,.T.) ;
#12672=FACE_OUTER_BOUND('',#15842,.T.) ;
#12673=FACE_OUTER_BOUND('',#15843,.T.) ;
#12674=FACE_OUTER_BOUND('',#15844,.T.) ;
#12675=FACE_OUTER_BOUND('',#15845,.T.) ;
#12676=FACE_OUTER_BOUND('',#15846,.T.) ;
#12677=FACE_OUTER_BOUND('',#15847,.T.) ;
#12678=FACE_OUTER_BOUND('',#15848,.T.) ;
#12679=FACE_OUTER_BOUND('',#15849,.T.) ;
#12680=FACE_OUTER_BOUND('',#15850,.T.) ;
#12681=FACE_OUTER_BOUND('',#15851,.T.) ;
#12682=FACE_OUTER_BOUND('',#15852,.T.) ;
#12683=FACE_OUTER_BOUND('',#15853,.T.) ;
#12684=FACE_OUTER_BOUND('',#15854,.T.) ;
#12685=FACE_OUTER_BOUND('',#15855,.T.) ;
#12686=FACE_OUTER_BOUND('',#15856,.T.) ;
#12687=FACE_OUTER_BOUND('',#15857,.T.) ;
#12688=FACE_OUTER_BOUND('',#15858,.T.) ;
#12689=FACE_OUTER_BOUND('',#15859,.T.) ;
#12690=FACE_OUTER_BOUND('',#15860,.T.) ;
#12691=FACE_OUTER_BOUND('',#15861,.T.) ;
#12692=FACE_OUTER_BOUND('',#15862,.T.) ;
#12693=FACE_OUTER_BOUND('',#15863,.T.) ;
#12694=FACE_OUTER_BOUND('',#15864,.T.) ;
#12695=FACE_OUTER_BOUND('',#15865,.T.) ;
#12696=FACE_OUTER_BOUND('',#15866,.T.) ;
#12697=FACE_OUTER_BOUND('',#15867,.T.) ;
#12698=FACE_OUTER_BOUND('',#15868,.T.) ;
#12699=FACE_OUTER_BOUND('',#15869,.T.) ;
#12700=FACE_OUTER_BOUND('',#15870,.T.) ;
#12701=FACE_OUTER_BOUND('',#15871,.T.) ;
#12702=FACE_OUTER_BOUND('',#15872,.T.) ;
#12703=FACE_OUTER_BOUND('',#15873,.T.) ;
#12704=FACE_OUTER_BOUND('',#15874,.T.) ;
#12705=FACE_OUTER_BOUND('',#15875,.T.) ;
#12706=FACE_OUTER_BOUND('',#15876,.T.) ;
#12707=FACE_OUTER_BOUND('',#15877,.T.) ;
#12708=FACE_OUTER_BOUND('',#15878,.T.) ;
#12709=FACE_OUTER_BOUND('',#15879,.T.) ;
#12710=FACE_OUTER_BOUND('',#15880,.T.) ;
#12711=FACE_OUTER_BOUND('',#15881,.T.) ;
#12712=FACE_OUTER_BOUND('',#15882,.T.) ;
#12713=FACE_OUTER_BOUND('',#15883,.T.) ;
#12714=FACE_OUTER_BOUND('',#15884,.T.) ;
#12715=FACE_OUTER_BOUND('',#15885,.T.) ;
#12716=FACE_OUTER_BOUND('',#15888,.T.) ;
#12717=FACE_OUTER_BOUND('',#15889,.T.) ;
#12718=FACE_OUTER_BOUND('',#15890,.T.) ;
#12719=FACE_OUTER_BOUND('',#15892,.T.) ;
#12720=FACE_OUTER_BOUND('',#15893,.T.) ;
#12721=FACE_OUTER_BOUND('',#15894,.T.) ;
#12722=FACE_OUTER_BOUND('',#15895,.T.) ;
#12723=FACE_OUTER_BOUND('',#15896,.T.) ;
#12724=FACE_OUTER_BOUND('',#15897,.T.) ;
#12725=FACE_OUTER_BOUND('',#15898,.T.) ;
#12726=FACE_OUTER_BOUND('',#15899,.T.) ;
#12727=FACE_OUTER_BOUND('',#15900,.T.) ;
#12728=FACE_OUTER_BOUND('',#15901,.T.) ;
#12729=FACE_OUTER_BOUND('',#15902,.T.) ;
#12730=FACE_OUTER_BOUND('',#15903,.T.) ;
#12731=FACE_OUTER_BOUND('',#15904,.T.) ;
#12732=FACE_OUTER_BOUND('',#15905,.T.) ;
#12733=FACE_OUTER_BOUND('',#15906,.T.) ;
#12734=FACE_OUTER_BOUND('',#15907,.T.) ;
#12735=FACE_OUTER_BOUND('',#15908,.T.) ;
#12736=FACE_OUTER_BOUND('',#15909,.T.) ;
#12737=FACE_OUTER_BOUND('',#15910,.T.) ;
#12738=FACE_OUTER_BOUND('',#15911,.T.) ;
#12739=FACE_OUTER_BOUND('',#15912,.T.) ;
#12740=FACE_OUTER_BOUND('',#15913,.T.) ;
#12741=FACE_OUTER_BOUND('',#15914,.T.) ;
#12742=FACE_OUTER_BOUND('',#15915,.T.) ;
#12743=FACE_OUTER_BOUND('',#15916,.T.) ;
#12744=FACE_OUTER_BOUND('',#15917,.T.) ;
#12745=FACE_OUTER_BOUND('',#15918,.T.) ;
#12746=FACE_OUTER_BOUND('',#15919,.T.) ;
#12747=FACE_OUTER_BOUND('',#15920,.T.) ;
#12748=FACE_OUTER_BOUND('',#15921,.T.) ;
#12749=FACE_OUTER_BOUND('',#15922,.T.) ;
#12750=FACE_OUTER_BOUND('',#15923,.T.) ;
#12751=FACE_OUTER_BOUND('',#15924,.T.) ;
#12752=FACE_OUTER_BOUND('',#15925,.T.) ;
#12753=FACE_OUTER_BOUND('',#15926,.T.) ;
#12754=FACE_OUTER_BOUND('',#15927,.T.) ;
#12755=FACE_OUTER_BOUND('',#15928,.T.) ;
#12756=FACE_OUTER_BOUND('',#15929,.T.) ;
#12757=FACE_OUTER_BOUND('',#15933,.T.) ;
#12758=FACE_OUTER_BOUND('',#15934,.T.) ;
#12759=FACE_OUTER_BOUND('',#15935,.T.) ;
#12760=FACE_OUTER_BOUND('',#15936,.T.) ;
#12761=FACE_OUTER_BOUND('',#15937,.T.) ;
#12762=FACE_OUTER_BOUND('',#15938,.T.) ;
#12763=FACE_OUTER_BOUND('',#15939,.T.) ;
#12764=FACE_OUTER_BOUND('',#15940,.T.) ;
#12765=FACE_OUTER_BOUND('',#15941,.T.) ;
#12766=FACE_OUTER_BOUND('',#15942,.T.) ;
#12767=FACE_OUTER_BOUND('',#15943,.T.) ;
#12768=FACE_OUTER_BOUND('',#15944,.T.) ;
#12769=FACE_OUTER_BOUND('',#15945,.T.) ;
#12770=FACE_OUTER_BOUND('',#15946,.T.) ;
#12771=FACE_OUTER_BOUND('',#15947,.T.) ;
#12772=FACE_OUTER_BOUND('',#15948,.T.) ;
#12773=FACE_OUTER_BOUND('',#15949,.T.) ;
#12774=FACE_OUTER_BOUND('',#15950,.T.) ;
#12775=FACE_OUTER_BOUND('',#15951,.T.) ;
#12776=FACE_OUTER_BOUND('',#15952,.T.) ;
#12777=FACE_OUTER_BOUND('',#15953,.T.) ;
#12778=FACE_OUTER_BOUND('',#15954,.T.) ;
#12779=FACE_OUTER_BOUND('',#15955,.T.) ;
#12780=FACE_OUTER_BOUND('',#15956,.T.) ;
#12781=FACE_OUTER_BOUND('',#15957,.T.) ;
#12782=FACE_OUTER_BOUND('',#15958,.T.) ;
#12783=FACE_OUTER_BOUND('',#15959,.T.) ;
#12784=FACE_OUTER_BOUND('',#15960,.T.) ;
#12785=FACE_OUTER_BOUND('',#15961,.T.) ;
#12786=FACE_OUTER_BOUND('',#15962,.T.) ;
#12787=FACE_OUTER_BOUND('',#15964,.T.) ;
#12788=FACE_OUTER_BOUND('',#15965,.T.) ;
#12789=FACE_OUTER_BOUND('',#15966,.T.) ;
#12790=FACE_OUTER_BOUND('',#15967,.T.) ;
#12791=FACE_OUTER_BOUND('',#15968,.T.) ;
#12792=FACE_OUTER_BOUND('',#15969,.T.) ;
#12793=FACE_OUTER_BOUND('',#15970,.T.) ;
#12794=FACE_OUTER_BOUND('',#15971,.T.) ;
#12795=FACE_OUTER_BOUND('',#15972,.T.) ;
#12796=FACE_OUTER_BOUND('',#15974,.T.) ;
#12797=FACE_OUTER_BOUND('',#15975,.T.) ;
#12798=FACE_OUTER_BOUND('',#15977,.T.) ;
#12799=FACE_OUTER_BOUND('',#15978,.T.) ;
#12800=FACE_OUTER_BOUND('',#15979,.T.) ;
#12801=FACE_OUTER_BOUND('',#15980,.T.) ;
#12802=FACE_OUTER_BOUND('',#15981,.T.) ;
#12803=FACE_OUTER_BOUND('',#15982,.T.) ;
#12804=FACE_OUTER_BOUND('',#15983,.T.) ;
#12805=FACE_OUTER_BOUND('',#15984,.T.) ;
#12806=FACE_OUTER_BOUND('',#15985,.T.) ;
#12807=FACE_OUTER_BOUND('',#15986,.T.) ;
#12808=FACE_OUTER_BOUND('',#15987,.T.) ;
#12809=FACE_OUTER_BOUND('',#15988,.T.) ;
#12810=FACE_OUTER_BOUND('',#15989,.T.) ;
#12811=FACE_OUTER_BOUND('',#15990,.T.) ;
#12812=FACE_OUTER_BOUND('',#15991,.T.) ;
#12813=FACE_OUTER_BOUND('',#15992,.T.) ;
#12814=FACE_OUTER_BOUND('',#15993,.T.) ;
#12815=FACE_OUTER_BOUND('',#15994,.T.) ;
#12816=FACE_OUTER_BOUND('',#15995,.T.) ;
#12817=FACE_OUTER_BOUND('',#15996,.T.) ;
#12818=FACE_OUTER_BOUND('',#15997,.T.) ;
#12819=FACE_OUTER_BOUND('',#15998,.T.) ;
#12820=FACE_OUTER_BOUND('',#15999,.T.) ;
#12821=FACE_OUTER_BOUND('',#16000,.T.) ;
#12822=FACE_OUTER_BOUND('',#16001,.T.) ;
#12823=FACE_OUTER_BOUND('',#16002,.T.) ;
#12824=FACE_OUTER_BOUND('',#16003,.T.) ;
#12825=FACE_OUTER_BOUND('',#16004,.T.) ;
#12826=FACE_OUTER_BOUND('',#16005,.T.) ;
#12827=FACE_OUTER_BOUND('',#16006,.T.) ;
#12828=FACE_OUTER_BOUND('',#16007,.T.) ;
#12829=FACE_OUTER_BOUND('',#16008,.T.) ;
#12830=FACE_OUTER_BOUND('',#16009,.T.) ;
#12831=FACE_OUTER_BOUND('',#16010,.T.) ;
#12832=FACE_OUTER_BOUND('',#16011,.T.) ;
#12833=FACE_OUTER_BOUND('',#16012,.T.) ;
#12834=FACE_OUTER_BOUND('',#16013,.T.) ;
#12835=FACE_OUTER_BOUND('',#16014,.T.) ;
#12836=FACE_OUTER_BOUND('',#16015,.T.) ;
#12837=FACE_OUTER_BOUND('',#16016,.T.) ;
#12838=FACE_OUTER_BOUND('',#16017,.T.) ;
#12839=FACE_OUTER_BOUND('',#16018,.T.) ;
#12840=FACE_OUTER_BOUND('',#16019,.T.) ;
#12841=FACE_OUTER_BOUND('',#16020,.T.) ;
#12842=FACE_OUTER_BOUND('',#16021,.T.) ;
#12843=FACE_OUTER_BOUND('',#16022,.T.) ;
#12844=FACE_OUTER_BOUND('',#16023,.T.) ;
#12845=FACE_OUTER_BOUND('',#16024,.T.) ;
#12846=FACE_OUTER_BOUND('',#16025,.T.) ;
#12847=FACE_OUTER_BOUND('',#16026,.T.) ;
#12848=FACE_OUTER_BOUND('',#16027,.T.) ;
#12849=FACE_OUTER_BOUND('',#16028,.T.) ;
#12850=FACE_OUTER_BOUND('',#16029,.T.) ;
#12851=FACE_OUTER_BOUND('',#16030,.T.) ;
#12852=FACE_OUTER_BOUND('',#16031,.T.) ;
#12853=FACE_OUTER_BOUND('',#16032,.T.) ;
#12854=FACE_OUTER_BOUND('',#16033,.T.) ;
#12855=FACE_OUTER_BOUND('',#16034,.T.) ;
#12856=FACE_OUTER_BOUND('',#16035,.T.) ;
#12857=FACE_OUTER_BOUND('',#16036,.T.) ;
#12858=FACE_OUTER_BOUND('',#16037,.T.) ;
#12859=FACE_OUTER_BOUND('',#16038,.T.) ;
#12860=FACE_OUTER_BOUND('',#16039,.T.) ;
#12861=FACE_OUTER_BOUND('',#16040,.T.) ;
#12862=FACE_OUTER_BOUND('',#16041,.T.) ;
#12863=FACE_OUTER_BOUND('',#16042,.T.) ;
#12864=FACE_OUTER_BOUND('',#16043,.T.) ;
#12865=FACE_OUTER_BOUND('',#16044,.T.) ;
#12866=FACE_OUTER_BOUND('',#16045,.T.) ;
#12867=FACE_OUTER_BOUND('',#16046,.T.) ;
#12868=FACE_OUTER_BOUND('',#16047,.T.) ;
#12869=FACE_OUTER_BOUND('',#16048,.T.) ;
#12870=FACE_OUTER_BOUND('',#16049,.T.) ;
#12871=FACE_OUTER_BOUND('',#16050,.T.) ;
#12872=FACE_OUTER_BOUND('',#16051,.T.) ;
#12873=FACE_OUTER_BOUND('',#16052,.T.) ;
#12874=FACE_OUTER_BOUND('',#16053,.T.) ;
#12875=FACE_OUTER_BOUND('',#16054,.T.) ;
#12876=FACE_OUTER_BOUND('',#16055,.T.) ;
#12877=FACE_OUTER_BOUND('',#16056,.T.) ;
#12878=FACE_OUTER_BOUND('',#16057,.T.) ;
#12879=FACE_OUTER_BOUND('',#16058,.T.) ;
#12880=FACE_OUTER_BOUND('',#16059,.T.) ;
#12881=FACE_OUTER_BOUND('',#16060,.T.) ;
#12882=FACE_OUTER_BOUND('',#16061,.T.) ;
#12883=FACE_OUTER_BOUND('',#16062,.T.) ;
#12884=FACE_OUTER_BOUND('',#16063,.T.) ;
#12885=FACE_OUTER_BOUND('',#16064,.T.) ;
#12886=FACE_OUTER_BOUND('',#16065,.T.) ;
#12887=FACE_OUTER_BOUND('',#16066,.T.) ;
#12888=FACE_OUTER_BOUND('',#16067,.T.) ;
#12889=FACE_OUTER_BOUND('',#16068,.T.) ;
#12890=FACE_OUTER_BOUND('',#16069,.T.) ;
#12891=FACE_OUTER_BOUND('',#16070,.T.) ;
#12892=FACE_OUTER_BOUND('',#16071,.T.) ;
#12893=FACE_OUTER_BOUND('',#16072,.T.) ;
#12894=FACE_OUTER_BOUND('',#16073,.T.) ;
#12895=FACE_OUTER_BOUND('',#16074,.T.) ;
#12896=FACE_OUTER_BOUND('',#16075,.T.) ;
#12897=FACE_OUTER_BOUND('',#16076,.T.) ;
#12898=FACE_OUTER_BOUND('',#16077,.T.) ;
#12899=FACE_OUTER_BOUND('',#16078,.T.) ;
#12900=FACE_OUTER_BOUND('',#16079,.T.) ;
#12901=FACE_OUTER_BOUND('',#16080,.T.) ;
#12902=FACE_OUTER_BOUND('',#16081,.T.) ;
#12903=FACE_OUTER_BOUND('',#16082,.T.) ;
#12904=FACE_OUTER_BOUND('',#16083,.T.) ;
#12905=FACE_OUTER_BOUND('',#16084,.T.) ;
#12906=FACE_OUTER_BOUND('',#16085,.T.) ;
#12907=FACE_OUTER_BOUND('',#16086,.T.) ;
#12908=FACE_OUTER_BOUND('',#16087,.T.) ;
#12909=FACE_OUTER_BOUND('',#16088,.T.) ;
#12910=FACE_OUTER_BOUND('',#16089,.T.) ;
#12911=FACE_OUTER_BOUND('',#16090,.T.) ;
#12912=FACE_OUTER_BOUND('',#16091,.T.) ;
#12913=FACE_OUTER_BOUND('',#16092,.T.) ;
#12914=FACE_OUTER_BOUND('',#16093,.T.) ;
#12915=FACE_OUTER_BOUND('',#16094,.T.) ;
#12916=FACE_OUTER_BOUND('',#16095,.T.) ;
#12917=FACE_OUTER_BOUND('',#16096,.T.) ;
#12918=FACE_OUTER_BOUND('',#16097,.T.) ;
#12919=FACE_OUTER_BOUND('',#16098,.T.) ;
#12920=FACE_OUTER_BOUND('',#16099,.T.) ;
#12921=FACE_OUTER_BOUND('',#16100,.T.) ;
#12922=FACE_OUTER_BOUND('',#16101,.T.) ;
#12923=FACE_OUTER_BOUND('',#16102,.T.) ;
#12924=FACE_OUTER_BOUND('',#16103,.T.) ;
#12925=FACE_OUTER_BOUND('',#16104,.T.) ;
#12926=FACE_OUTER_BOUND('',#16105,.T.) ;
#12927=FACE_OUTER_BOUND('',#16109,.T.) ;
#12928=FACE_OUTER_BOUND('',#16110,.T.) ;
#12929=FACE_OUTER_BOUND('',#16111,.T.) ;
#12930=FACE_OUTER_BOUND('',#16112,.T.) ;
#12931=FACE_OUTER_BOUND('',#16113,.T.) ;
#12932=FACE_OUTER_BOUND('',#16114,.T.) ;
#12933=FACE_OUTER_BOUND('',#16115,.T.) ;
#12934=FACE_OUTER_BOUND('',#16116,.T.) ;
#12935=FACE_OUTER_BOUND('',#16117,.T.) ;
#12936=FACE_OUTER_BOUND('',#16118,.T.) ;
#12937=FACE_OUTER_BOUND('',#16119,.T.) ;
#12938=FACE_OUTER_BOUND('',#16120,.T.) ;
#12939=FACE_OUTER_BOUND('',#16121,.T.) ;
#12940=FACE_OUTER_BOUND('',#16122,.T.) ;
#12941=FACE_OUTER_BOUND('',#16123,.T.) ;
#12942=FACE_OUTER_BOUND('',#16124,.T.) ;
#12943=FACE_OUTER_BOUND('',#16125,.T.) ;
#12944=FACE_OUTER_BOUND('',#16126,.T.) ;
#12945=FACE_OUTER_BOUND('',#16127,.T.) ;
#12946=FACE_OUTER_BOUND('',#16128,.T.) ;
#12947=FACE_OUTER_BOUND('',#16129,.T.) ;
#12948=FACE_OUTER_BOUND('',#16130,.T.) ;
#12949=FACE_OUTER_BOUND('',#16131,.T.) ;
#12950=FACE_OUTER_BOUND('',#16132,.T.) ;
#12951=FACE_OUTER_BOUND('',#16133,.T.) ;
#12952=FACE_OUTER_BOUND('',#16134,.T.) ;
#12953=FACE_OUTER_BOUND('',#16135,.T.) ;
#12954=FACE_OUTER_BOUND('',#16136,.T.) ;
#12955=FACE_OUTER_BOUND('',#16137,.T.) ;
#12956=FACE_OUTER_BOUND('',#16138,.T.) ;
#12957=FACE_OUTER_BOUND('',#16139,.T.) ;
#12958=FACE_OUTER_BOUND('',#16140,.T.) ;
#12959=FACE_OUTER_BOUND('',#16141,.T.) ;
#12960=FACE_OUTER_BOUND('',#16142,.T.) ;
#12961=FACE_OUTER_BOUND('',#16143,.T.) ;
#12962=FACE_OUTER_BOUND('',#16144,.T.) ;
#12963=FACE_OUTER_BOUND('',#16145,.T.) ;
#12964=FACE_OUTER_BOUND('',#16146,.T.) ;
#12965=FACE_OUTER_BOUND('',#16147,.T.) ;
#12966=FACE_OUTER_BOUND('',#16148,.T.) ;
#12967=FACE_OUTER_BOUND('',#16149,.T.) ;
#12968=FACE_OUTER_BOUND('',#16150,.T.) ;
#12969=FACE_OUTER_BOUND('',#16151,.T.) ;
#12970=FACE_OUTER_BOUND('',#16152,.T.) ;
#12971=FACE_OUTER_BOUND('',#16153,.T.) ;
#12972=FACE_OUTER_BOUND('',#16154,.T.) ;
#12973=FACE_OUTER_BOUND('',#16155,.T.) ;
#12974=FACE_OUTER_BOUND('',#16156,.T.) ;
#12975=FACE_OUTER_BOUND('',#16157,.T.) ;
#12976=FACE_OUTER_BOUND('',#16158,.T.) ;
#12977=FACE_OUTER_BOUND('',#16159,.T.) ;
#12978=FACE_OUTER_BOUND('',#16160,.T.) ;
#12979=FACE_OUTER_BOUND('',#16161,.T.) ;
#12980=FACE_OUTER_BOUND('',#16162,.T.) ;
#12981=FACE_OUTER_BOUND('',#16163,.T.) ;
#12982=FACE_OUTER_BOUND('',#16164,.T.) ;
#12983=FACE_OUTER_BOUND('',#16165,.T.) ;
#12984=FACE_OUTER_BOUND('',#16166,.T.) ;
#12985=FACE_OUTER_BOUND('',#16167,.T.) ;
#12986=FACE_OUTER_BOUND('',#16168,.T.) ;
#12987=FACE_OUTER_BOUND('',#16169,.T.) ;
#12988=FACE_OUTER_BOUND('',#16170,.T.) ;
#12989=FACE_OUTER_BOUND('',#16171,.T.) ;
#12990=FACE_OUTER_BOUND('',#16172,.T.) ;
#12991=FACE_OUTER_BOUND('',#16173,.T.) ;
#12992=FACE_OUTER_BOUND('',#16174,.T.) ;
#12993=FACE_OUTER_BOUND('',#16175,.T.) ;
#12994=FACE_OUTER_BOUND('',#16176,.T.) ;
#12995=FACE_OUTER_BOUND('',#16177,.T.) ;
#12996=FACE_OUTER_BOUND('',#16178,.T.) ;
#12997=FACE_OUTER_BOUND('',#16179,.T.) ;
#12998=FACE_OUTER_BOUND('',#16180,.T.) ;
#12999=FACE_OUTER_BOUND('',#16181,.T.) ;
#13000=FACE_OUTER_BOUND('',#16182,.T.) ;
#13001=FACE_OUTER_BOUND('',#16183,.T.) ;
#13002=FACE_OUTER_BOUND('',#16184,.T.) ;
#13003=FACE_OUTER_BOUND('',#16185,.T.) ;
#13004=FACE_OUTER_BOUND('',#16186,.T.) ;
#13005=FACE_OUTER_BOUND('',#16187,.T.) ;
#13006=FACE_OUTER_BOUND('',#16188,.T.) ;
#13007=FACE_OUTER_BOUND('',#16189,.T.) ;
#13008=FACE_OUTER_BOUND('',#16190,.T.) ;
#13009=FACE_OUTER_BOUND('',#16191,.T.) ;
#13010=FACE_OUTER_BOUND('',#16192,.T.) ;
#13011=FACE_OUTER_BOUND('',#16193,.T.) ;
#13012=FACE_OUTER_BOUND('',#16194,.T.) ;
#13013=FACE_OUTER_BOUND('',#16195,.T.) ;
#13014=FACE_OUTER_BOUND('',#16196,.T.) ;
#13015=FACE_OUTER_BOUND('',#16197,.T.) ;
#13016=FACE_OUTER_BOUND('',#16198,.T.) ;
#13017=FACE_OUTER_BOUND('',#16199,.T.) ;
#13018=FACE_OUTER_BOUND('',#16200,.T.) ;
#13019=FACE_OUTER_BOUND('',#16201,.T.) ;
#13020=FACE_OUTER_BOUND('',#16202,.T.) ;
#13021=FACE_OUTER_BOUND('',#16203,.T.) ;
#13022=FACE_OUTER_BOUND('',#16204,.T.) ;
#13023=FACE_OUTER_BOUND('',#16205,.T.) ;
#13024=FACE_OUTER_BOUND('',#16206,.T.) ;
#13025=FACE_OUTER_BOUND('',#16207,.T.) ;
#13026=FACE_OUTER_BOUND('',#16208,.T.) ;
#13027=FACE_OUTER_BOUND('',#16209,.T.) ;
#13028=FACE_OUTER_BOUND('',#16210,.T.) ;
#13029=FACE_OUTER_BOUND('',#16211,.T.) ;
#13030=FACE_OUTER_BOUND('',#16212,.T.) ;
#13031=FACE_OUTER_BOUND('',#16213,.T.) ;
#13032=FACE_OUTER_BOUND('',#16214,.T.) ;
#13033=FACE_OUTER_BOUND('',#16215,.T.) ;
#13034=FACE_OUTER_BOUND('',#16216,.T.) ;
#13035=FACE_OUTER_BOUND('',#16217,.T.) ;
#13036=FACE_OUTER_BOUND('',#16218,.T.) ;
#13037=FACE_OUTER_BOUND('',#16219,.T.) ;
#13038=FACE_OUTER_BOUND('',#16220,.T.) ;
#13039=FACE_OUTER_BOUND('',#16221,.T.) ;
#13040=FACE_OUTER_BOUND('',#16222,.T.) ;
#13041=FACE_OUTER_BOUND('',#16223,.T.) ;
#13042=FACE_OUTER_BOUND('',#16224,.T.) ;
#13043=FACE_OUTER_BOUND('',#16225,.T.) ;
#13044=FACE_OUTER_BOUND('',#16226,.T.) ;
#13045=FACE_OUTER_BOUND('',#16227,.T.) ;
#13046=FACE_OUTER_BOUND('',#16228,.T.) ;
#13047=FACE_OUTER_BOUND('',#16229,.T.) ;
#13048=FACE_OUTER_BOUND('',#16230,.T.) ;
#13049=FACE_OUTER_BOUND('',#16231,.T.) ;
#13050=FACE_OUTER_BOUND('',#16232,.T.) ;
#13051=FACE_OUTER_BOUND('',#16233,.T.) ;
#13052=FACE_OUTER_BOUND('',#16234,.T.) ;
#13053=FACE_OUTER_BOUND('',#16235,.T.) ;
#13054=FACE_OUTER_BOUND('',#16236,.T.) ;
#13055=FACE_OUTER_BOUND('',#16237,.T.) ;
#13056=FACE_OUTER_BOUND('',#16238,.T.) ;
#13057=FACE_OUTER_BOUND('',#16239,.T.) ;
#13058=FACE_OUTER_BOUND('',#16240,.T.) ;
#13059=FACE_OUTER_BOUND('',#16241,.T.) ;
#13060=FACE_OUTER_BOUND('',#16242,.T.) ;
#13061=FACE_OUTER_BOUND('',#16243,.T.) ;
#13062=FACE_OUTER_BOUND('',#16244,.T.) ;
#13063=FACE_OUTER_BOUND('',#16245,.T.) ;
#13064=FACE_OUTER_BOUND('',#16246,.T.) ;
#13065=FACE_OUTER_BOUND('',#16247,.T.) ;
#13066=FACE_OUTER_BOUND('',#16248,.T.) ;
#13067=FACE_OUTER_BOUND('',#16249,.T.) ;
#13068=FACE_OUTER_BOUND('',#16250,.T.) ;
#13069=FACE_OUTER_BOUND('',#16251,.T.) ;
#13070=FACE_OUTER_BOUND('',#16252,.T.) ;
#13071=FACE_OUTER_BOUND('',#16253,.T.) ;
#13072=FACE_OUTER_BOUND('',#16254,.T.) ;
#13073=FACE_OUTER_BOUND('',#16255,.T.) ;
#13074=FACE_OUTER_BOUND('',#16256,.T.) ;
#13075=FACE_OUTER_BOUND('',#16257,.T.) ;
#13076=FACE_OUTER_BOUND('',#16258,.T.) ;
#13077=FACE_OUTER_BOUND('',#16259,.T.) ;
#13078=FACE_OUTER_BOUND('',#16260,.T.) ;
#13079=FACE_OUTER_BOUND('',#16261,.T.) ;
#13080=FACE_OUTER_BOUND('',#16263,.T.) ;
#13081=FACE_OUTER_BOUND('',#16264,.T.) ;
#13082=FACE_OUTER_BOUND('',#16265,.T.) ;
#13083=FACE_OUTER_BOUND('',#16266,.T.) ;
#13084=FACE_OUTER_BOUND('',#16267,.T.) ;
#13085=FACE_OUTER_BOUND('',#16268,.T.) ;
#13086=FACE_OUTER_BOUND('',#16269,.T.) ;
#13087=FACE_OUTER_BOUND('',#16270,.T.) ;
#13088=FACE_OUTER_BOUND('',#16271,.T.) ;
#13089=FACE_OUTER_BOUND('',#16272,.T.) ;
#13090=FACE_OUTER_BOUND('',#16273,.T.) ;
#13091=FACE_OUTER_BOUND('',#16274,.T.) ;
#13092=FACE_OUTER_BOUND('',#16275,.T.) ;
#13093=FACE_OUTER_BOUND('',#16276,.T.) ;
#13094=FACE_OUTER_BOUND('',#16277,.T.) ;
#13095=FACE_OUTER_BOUND('',#16278,.T.) ;
#13096=FACE_OUTER_BOUND('',#16279,.T.) ;
#13097=FACE_OUTER_BOUND('',#16280,.T.) ;
#13098=FACE_OUTER_BOUND('',#16281,.T.) ;
#13099=FACE_OUTER_BOUND('',#16282,.T.) ;
#13100=FACE_OUTER_BOUND('',#16283,.T.) ;
#13101=FACE_OUTER_BOUND('',#16284,.T.) ;
#13102=FACE_OUTER_BOUND('',#16285,.T.) ;
#13103=FACE_OUTER_BOUND('',#16286,.T.) ;
#13104=FACE_OUTER_BOUND('',#16287,.T.) ;
#13105=FACE_OUTER_BOUND('',#16288,.T.) ;
#13106=FACE_OUTER_BOUND('',#16289,.T.) ;
#13107=FACE_OUTER_BOUND('',#16290,.T.) ;
#13108=FACE_OUTER_BOUND('',#16291,.T.) ;
#13109=FACE_OUTER_BOUND('',#16292,.T.) ;
#13110=FACE_OUTER_BOUND('',#16293,.T.) ;
#13111=FACE_OUTER_BOUND('',#16294,.T.) ;
#13112=FACE_OUTER_BOUND('',#16295,.T.) ;
#13113=FACE_OUTER_BOUND('',#16296,.T.) ;
#13114=FACE_OUTER_BOUND('',#16297,.T.) ;
#13115=FACE_OUTER_BOUND('',#16298,.T.) ;
#13116=FACE_OUTER_BOUND('',#16299,.T.) ;
#13117=FACE_OUTER_BOUND('',#16300,.T.) ;
#13118=FACE_OUTER_BOUND('',#16301,.T.) ;
#13119=FACE_OUTER_BOUND('',#16302,.T.) ;
#13120=FACE_OUTER_BOUND('',#16303,.T.) ;
#13121=FACE_OUTER_BOUND('',#16304,.T.) ;
#13122=FACE_OUTER_BOUND('',#16305,.T.) ;
#13123=FACE_OUTER_BOUND('',#16306,.T.) ;
#13124=FACE_OUTER_BOUND('',#16307,.T.) ;
#13125=FACE_OUTER_BOUND('',#16308,.T.) ;
#13126=FACE_OUTER_BOUND('',#16309,.T.) ;
#13127=FACE_OUTER_BOUND('',#16310,.T.) ;
#13128=FACE_OUTER_BOUND('',#16311,.T.) ;
#13129=FACE_OUTER_BOUND('',#16312,.T.) ;
#13130=FACE_OUTER_BOUND('',#16313,.T.) ;
#13131=FACE_OUTER_BOUND('',#16314,.T.) ;
#13132=FACE_OUTER_BOUND('',#16315,.T.) ;
#13133=FACE_OUTER_BOUND('',#16316,.T.) ;
#13134=FACE_OUTER_BOUND('',#16317,.T.) ;
#13135=FACE_OUTER_BOUND('',#16318,.T.) ;
#13136=FACE_OUTER_BOUND('',#16319,.T.) ;
#13137=FACE_OUTER_BOUND('',#16320,.T.) ;
#13138=FACE_OUTER_BOUND('',#16321,.T.) ;
#13139=FACE_OUTER_BOUND('',#16322,.T.) ;
#13140=FACE_OUTER_BOUND('',#16323,.T.) ;
#13141=FACE_OUTER_BOUND('',#16324,.T.) ;
#13142=FACE_OUTER_BOUND('',#16325,.T.) ;
#13143=FACE_OUTER_BOUND('',#16326,.T.) ;
#13144=FACE_OUTER_BOUND('',#16327,.T.) ;
#13145=FACE_OUTER_BOUND('',#16328,.T.) ;
#13146=FACE_OUTER_BOUND('',#16329,.T.) ;
#13147=FACE_OUTER_BOUND('',#16330,.T.) ;
#13148=FACE_OUTER_BOUND('',#16331,.T.) ;
#13149=FACE_OUTER_BOUND('',#16332,.T.) ;
#13150=FACE_OUTER_BOUND('',#16333,.T.) ;
#13151=FACE_OUTER_BOUND('',#16334,.T.) ;
#13152=FACE_OUTER_BOUND('',#16335,.T.) ;
#13153=FACE_OUTER_BOUND('',#16336,.T.) ;
#13154=FACE_OUTER_BOUND('',#16337,.T.) ;
#13155=FACE_OUTER_BOUND('',#16338,.T.) ;
#13156=FACE_OUTER_BOUND('',#16339,.T.) ;
#13157=FACE_OUTER_BOUND('',#16340,.T.) ;
#13158=FACE_OUTER_BOUND('',#16341,.T.) ;
#13159=FACE_OUTER_BOUND('',#16342,.T.) ;
#13160=FACE_OUTER_BOUND('',#16343,.T.) ;
#13161=FACE_OUTER_BOUND('',#16344,.T.) ;
#13162=FACE_OUTER_BOUND('',#16345,.T.) ;
#13163=FACE_OUTER_BOUND('',#16346,.T.) ;
#13164=FACE_OUTER_BOUND('',#16347,.T.) ;
#13165=FACE_OUTER_BOUND('',#16348,.T.) ;
#13166=FACE_OUTER_BOUND('',#16349,.T.) ;
#13167=FACE_OUTER_BOUND('',#16350,.T.) ;
#13168=FACE_OUTER_BOUND('',#16351,.T.) ;
#13169=FACE_OUTER_BOUND('',#16352,.T.) ;
#13170=FACE_OUTER_BOUND('',#16353,.T.) ;
#13171=FACE_OUTER_BOUND('',#16354,.T.) ;
#13172=FACE_OUTER_BOUND('',#16355,.T.) ;
#13173=FACE_OUTER_BOUND('',#16356,.T.) ;
#13174=FACE_OUTER_BOUND('',#16357,.T.) ;
#13175=FACE_OUTER_BOUND('',#16358,.T.) ;
#13176=FACE_OUTER_BOUND('',#16359,.T.) ;
#13177=FACE_OUTER_BOUND('',#16360,.T.) ;
#13178=FACE_OUTER_BOUND('',#16361,.T.) ;
#13179=FACE_OUTER_BOUND('',#16362,.T.) ;
#13180=FACE_OUTER_BOUND('',#16363,.T.) ;
#13181=FACE_OUTER_BOUND('',#16364,.T.) ;
#13182=FACE_OUTER_BOUND('',#16365,.T.) ;
#13183=FACE_OUTER_BOUND('',#16366,.T.) ;
#13184=FACE_OUTER_BOUND('',#16367,.T.) ;
#13185=FACE_OUTER_BOUND('',#16368,.T.) ;
#13186=FACE_OUTER_BOUND('',#16369,.T.) ;
#13187=FACE_OUTER_BOUND('',#16370,.T.) ;
#13188=FACE_OUTER_BOUND('',#16371,.T.) ;
#13189=FACE_OUTER_BOUND('',#16372,.T.) ;
#13190=FACE_OUTER_BOUND('',#16373,.T.) ;
#13191=FACE_OUTER_BOUND('',#16374,.T.) ;
#13192=FACE_OUTER_BOUND('',#16375,.T.) ;
#13193=FACE_OUTER_BOUND('',#16376,.T.) ;
#13194=FACE_OUTER_BOUND('',#16377,.T.) ;
#13195=FACE_OUTER_BOUND('',#16378,.T.) ;
#13196=FACE_OUTER_BOUND('',#16379,.T.) ;
#13197=FACE_OUTER_BOUND('',#16380,.T.) ;
#13198=FACE_OUTER_BOUND('',#16381,.T.) ;
#13199=FACE_OUTER_BOUND('',#16382,.T.) ;
#13200=FACE_OUTER_BOUND('',#16383,.T.) ;
#13201=FACE_OUTER_BOUND('',#16384,.T.) ;
#13202=FACE_OUTER_BOUND('',#16385,.T.) ;
#13203=FACE_OUTER_BOUND('',#16386,.T.) ;
#13204=FACE_OUTER_BOUND('',#16387,.T.) ;
#13205=FACE_OUTER_BOUND('',#16388,.T.) ;
#13206=FACE_OUTER_BOUND('',#16389,.T.) ;
#13207=FACE_OUTER_BOUND('',#16390,.T.) ;
#15542=EDGE_LOOP('',(#38470,#38471,#38472,#38473)) ;
#15543=EDGE_LOOP('',(#38474,#38475,#38476,#38477)) ;
#15544=EDGE_LOOP('',(#38478,#38479,#38480,#38481,#38482)) ;
#15545=EDGE_LOOP('',(#38483,#38484,#38485,#38486)) ;
#15546=EDGE_LOOP('',(#38487,#38488,#38489,#38490)) ;
#15547=EDGE_LOOP('',(#38491,#38492,#38493,#38494)) ;
#15548=EDGE_LOOP('',(#38495,#38496,#38497,#38498)) ;
#15549=EDGE_LOOP('',(#38499,#38500,#38501,#38502)) ;
#15550=EDGE_LOOP('',(#38503,#38504,#38505,#38506)) ;
#15551=EDGE_LOOP('',(#38507,#38508,#38509,#38510)) ;
#15552=EDGE_LOOP('',(#38511,#38512,#38513,#38514)) ;
#15553=EDGE_LOOP('',(#38515,#38516,#38517,#38518)) ;
#15554=EDGE_LOOP('',(#38519,#38520,#38521,#38522)) ;
#15555=EDGE_LOOP('',(#38523,#38524,#38525,#38526)) ;
#15556=EDGE_LOOP('',(#38527,#38528,#38529,#38530)) ;
#15557=EDGE_LOOP('',(#38531,#38532,#38533,#38534)) ;
#15558=EDGE_LOOP('',(#38535,#38536,#38537,#38538)) ;
#15559=EDGE_LOOP('',(#38539,#38540,#38541,#38542)) ;
#15560=EDGE_LOOP('',(#38543,#38544,#38545,#38546)) ;
#15561=EDGE_LOOP('',(#38547,#38548,#38549,#38550)) ;
#15562=EDGE_LOOP('',(#38551,#38552,#38553,#38554)) ;
#15563=EDGE_LOOP('',(#38555,#38556,#38557,#38558)) ;
#15564=EDGE_LOOP('',(#38559,#38560,#38561,#38562)) ;
#15565=EDGE_LOOP('',(#38563,#38564,#38565,#38566)) ;
#15566=EDGE_LOOP('',(#38567,#38568,#38569,#38570)) ;
#15567=EDGE_LOOP('',(#38571,#38572,#38573,#38574)) ;
#15568=EDGE_LOOP('',(#38575,#38576,#38577,#38578)) ;
#15569=EDGE_LOOP('',(#38579,#38580,#38581,#38582)) ;
#15570=EDGE_LOOP('',(#38583,#38584,#38585,#38586)) ;
#15571=EDGE_LOOP('',(#38587,#38588,#38589,#38590)) ;
#15572=EDGE_LOOP('',(#38591,#38592,#38593,#38594)) ;
#15573=EDGE_LOOP('',(#38595,#38596,#38597,#38598)) ;
#15574=EDGE_LOOP('',(#38599,#38600,#38601,#38602,#38603,#38604,#38605,#38606,
#38607,#38608,#38609,#38610,#38611,#38612,#38613,#38614,#38615,#38616,#38617)) ;
#15575=EDGE_LOOP('',(#38618,#38619,#38620,#38621,#38622,#38623,#38624,#38625)) ;
#15576=EDGE_LOOP('',(#38626,#38627,#38628,#38629,#38630,#38631,#38632,#38633,
#38634,#38635,#38636,#38637,#38638,#38639,#38640,#38641,#38642,#38643)) ;
#15577=EDGE_LOOP('',(#38644,#38645,#38646,#38647)) ;
#15578=EDGE_LOOP('',(#38648,#38649,#38650,#38651,#38652,#38653,#38654,#38655,
#38656,#38657,#38658,#38659,#38660,#38661,#38662,#38663,#38664,#38665,#38666)) ;
#15579=EDGE_LOOP('',(#38667,#38668,#38669,#38670)) ;
#15580=EDGE_LOOP('',(#38671,#38672,#38673,#38674)) ;
#15581=EDGE_LOOP('',(#38675,#38676,#38677,#38678)) ;
#15582=EDGE_LOOP('',(#38679,#38680,#38681,#38682)) ;
#15583=EDGE_LOOP('',(#38683,#38684,#38685,#38686)) ;
#15584=EDGE_LOOP('',(#38687,#38688,#38689,#38690,#38691)) ;
#15585=EDGE_LOOP('',(#38692,#38693,#38694,#38695,#38696)) ;
#15586=EDGE_LOOP('',(#38697,#38698,#38699,#38700,#38701,#38702,#38703)) ;
#15587=EDGE_LOOP('',(#38704,#38705,#38706,#38707)) ;
#15588=EDGE_LOOP('',(#38708,#38709,#38710,#38711,#38712)) ;
#15589=EDGE_LOOP('',(#38713,#38714,#38715,#38716,#38717,#38718,#38719)) ;
#15590=EDGE_LOOP('',(#38720,#38721,#38722,#38723)) ;
#15591=EDGE_LOOP('',(#38724,#38725,#38726,#38727)) ;
#15592=EDGE_LOOP('',(#38728,#38729,#38730,#38731)) ;
#15593=EDGE_LOOP('',(#38732,#38733,#38734,#38735)) ;
#15594=EDGE_LOOP('',(#38736,#38737,#38738,#38739,#38740)) ;
#15595=EDGE_LOOP('',(#38741,#38742,#38743,#38744)) ;
#15596=EDGE_LOOP('',(#38745,#38746,#38747,#38748,#38749)) ;
#15597=EDGE_LOOP('',(#38750,#38751,#38752,#38753)) ;
#15598=EDGE_LOOP('',(#38754,#38755,#38756)) ;
#15599=EDGE_LOOP('',(#38757,#38758,#38759,#38760,#38761,#38762,#38763,#38764,
#38765,#38766,#38767,#38768,#38769,#38770,#38771,#38772,#38773)) ;
#15600=EDGE_LOOP('',(#38774,#38775,#38776,#38777,#38778)) ;
#15601=EDGE_LOOP('',(#38779,#38780,#38781,#38782)) ;
#15602=EDGE_LOOP('',(#38783,#38784,#38785,#38786)) ;
#15603=EDGE_LOOP('',(#38787,#38788,#38789)) ;
#15604=EDGE_LOOP('',(#38790,#38791,#38792,#38793,#38794)) ;
#15605=EDGE_LOOP('',(#38795,#38796,#38797,#38798,#38799)) ;
#15606=EDGE_LOOP('',(#38800,#38801,#38802,#38803,#38804)) ;
#15607=EDGE_LOOP('',(#38805,#38806,#38807,#38808,#38809)) ;
#15608=EDGE_LOOP('',(#38810,#38811,#38812,#38813)) ;
#15609=EDGE_LOOP('',(#38814,#38815,#38816,#38817)) ;
#15610=EDGE_LOOP('',(#38818,#38819,#38820,#38821,#38822)) ;
#15611=EDGE_LOOP('',(#38823,#38824,#38825,#38826,#38827,#38828,#38829,#38830,
#38831,#38832,#38833,#38834,#38835,#38836,#38837,#38838)) ;
#15612=EDGE_LOOP('',(#38839,#38840,#38841,#38842,#38843)) ;
#15613=EDGE_LOOP('',(#38844,#38845,#38846,#38847,#38848)) ;
#15614=EDGE_LOOP('',(#38849,#38850,#38851)) ;
#15615=EDGE_LOOP('',(#38852,#38853,#38854,#38855)) ;
#15616=EDGE_LOOP('',(#38856,#38857,#38858,#38859,#38860,#38861)) ;
#15617=EDGE_LOOP('',(#38862,#38863,#38864,#38865,#38866,#38867,#38868,#38869,
#38870)) ;
#15618=EDGE_LOOP('',(#38871,#38872,#38873,#38874)) ;
#15619=EDGE_LOOP('',(#38875,#38876,#38877,#38878,#38879)) ;
#15620=EDGE_LOOP('',(#38880,#38881,#38882,#38883)) ;
#15621=EDGE_LOOP('',(#38884,#38885,#38886,#38887)) ;
#15622=EDGE_LOOP('',(#38888,#38889,#38890,#38891,#38892,#38893)) ;
#15623=EDGE_LOOP('',(#38894,#38895,#38896,#38897)) ;
#15624=EDGE_LOOP('',(#38898,#38899,#38900,#38901)) ;
#15625=EDGE_LOOP('',(#38902,#38903,#38904,#38905,#38906)) ;
#15626=EDGE_LOOP('',(#38907,#38908,#38909,#38910)) ;
#15627=EDGE_LOOP('',(#38911,#38912,#38913,#38914,#38915,#38916,#38917,#38918,
#38919)) ;
#15628=EDGE_LOOP('',(#38920,#38921,#38922,#38923)) ;
#15629=EDGE_LOOP('',(#38924,#38925,#38926,#38927)) ;
#15630=EDGE_LOOP('',(#38928,#38929,#38930,#38931)) ;
#15631=EDGE_LOOP('',(#38932,#38933,#38934,#38935,#38936,#38937,#38938)) ;
#15632=EDGE_LOOP('',(#38939,#38940,#38941,#38942)) ;
#15633=EDGE_LOOP('',(#38943,#38944,#38945,#38946,#38947)) ;
#15634=EDGE_LOOP('',(#38948,#38949,#38950,#38951)) ;
#15635=EDGE_LOOP('',(#38952,#38953,#38954,#38955)) ;
#15636=EDGE_LOOP('',(#38956,#38957,#38958,#38959)) ;
#15637=EDGE_LOOP('',(#38960,#38961,#38962,#38963)) ;
#15638=EDGE_LOOP('',(#38964,#38965,#38966,#38967)) ;
#15639=EDGE_LOOP('',(#38968,#38969,#38970,#38971)) ;
#15640=EDGE_LOOP('',(#38972,#38973,#38974,#38975)) ;
#15641=EDGE_LOOP('',(#38976,#38977,#38978,#38979,#38980,#38981)) ;
#15642=EDGE_LOOP('',(#38982,#38983,#38984,#38985,#38986,#38987,#38988,#38989,
#38990)) ;
#15643=EDGE_LOOP('',(#38991,#38992,#38993,#38994)) ;
#15644=EDGE_LOOP('',(#38995,#38996,#38997,#38998,#38999,#39000,#39001,#39002)) ;
#15645=EDGE_LOOP('',(#39003,#39004,#39005,#39006,#39007)) ;
#15646=EDGE_LOOP('',(#39008,#39009,#39010)) ;
#15647=EDGE_LOOP('',(#39011,#39012,#39013,#39014)) ;
#15648=EDGE_LOOP('',(#39015,#39016,#39017,#39018)) ;
#15649=EDGE_LOOP('',(#39019,#39020,#39021,#39022)) ;
#15650=EDGE_LOOP('',(#39023,#39024,#39025,#39026)) ;
#15651=EDGE_LOOP('',(#39027,#39028,#39029,#39030)) ;
#15652=EDGE_LOOP('',(#39031,#39032,#39033,#39034)) ;
#15653=EDGE_LOOP('',(#39035,#39036,#39037,#39038)) ;
#15654=EDGE_LOOP('',(#39039,#39040,#39041,#39042)) ;
#15655=EDGE_LOOP('',(#39043,#39044,#39045,#39046)) ;
#15656=EDGE_LOOP('',(#39047,#39048,#39049,#39050)) ;
#15657=EDGE_LOOP('',(#39051,#39052,#39053,#39054,#39055,#39056,#39057,#39058,
#39059,#39060,#39061,#39062,#39063,#39064,#39065,#39066,#39067,#39068)) ;
#15658=EDGE_LOOP('',(#39069,#39070,#39071,#39072)) ;
#15659=EDGE_LOOP('',(#39073,#39074,#39075,#39076,#39077)) ;
#15660=EDGE_LOOP('',(#39078,#39079,#39080,#39081,#39082)) ;
#15661=EDGE_LOOP('',(#39083,#39084,#39085,#39086)) ;
#15662=EDGE_LOOP('',(#39087,#39088,#39089,#39090,#39091)) ;
#15663=EDGE_LOOP('',(#39092,#39093,#39094,#39095)) ;
#15664=EDGE_LOOP('',(#39096,#39097,#39098,#39099)) ;
#15665=EDGE_LOOP('',(#39100,#39101,#39102,#39103,#39104,#39105,#39106)) ;
#15666=EDGE_LOOP('',(#39107,#39108,#39109,#39110)) ;
#15667=EDGE_LOOP('',(#39111,#39112,#39113,#39114)) ;
#15668=EDGE_LOOP('',(#39115,#39116,#39117,#39118)) ;
#15669=EDGE_LOOP('',(#39119,#39120,#39121,#39122)) ;
#15670=EDGE_LOOP('',(#39123,#39124,#39125,#39126)) ;
#15671=EDGE_LOOP('',(#39127,#39128,#39129,#39130)) ;
#15672=EDGE_LOOP('',(#39131,#39132,#39133,#39134)) ;
#15673=EDGE_LOOP('',(#39135,#39136,#39137,#39138,#39139)) ;
#15674=EDGE_LOOP('',(#39140,#39141,#39142,#39143)) ;
#15675=EDGE_LOOP('',(#39144,#39145,#39146,#39147)) ;
#15676=EDGE_LOOP('',(#39148,#39149,#39150,#39151)) ;
#15677=EDGE_LOOP('',(#39152,#39153,#39154,#39155)) ;
#15678=EDGE_LOOP('',(#39156,#39157,#39158,#39159)) ;
#15679=EDGE_LOOP('',(#39160,#39161,#39162,#39163)) ;
#15680=EDGE_LOOP('',(#39164,#39165,#39166,#39167)) ;
#15681=EDGE_LOOP('',(#39168,#39169,#39170,#39171)) ;
#15682=EDGE_LOOP('',(#39172,#39173,#39174,#39175,#39176,#39177,#39178,#39179,
#39180)) ;
#15683=EDGE_LOOP('',(#39181,#39182,#39183,#39184)) ;
#15684=EDGE_LOOP('',(#39185,#39186,#39187,#39188,#39189,#39190)) ;
#15685=EDGE_LOOP('',(#39191,#39192,#39193,#39194)) ;
#15686=EDGE_LOOP('',(#39195,#39196,#39197,#39198)) ;
#15687=EDGE_LOOP('',(#39199,#39200,#39201,#39202,#39203)) ;
#15688=EDGE_LOOP('',(#39204,#39205,#39206,#39207)) ;
#15689=EDGE_LOOP('',(#39208,#39209,#39210,#39211)) ;
#15690=EDGE_LOOP('',(#39212,#39213,#39214,#39215)) ;
#15691=EDGE_LOOP('',(#39216,#39217,#39218,#39219)) ;
#15692=EDGE_LOOP('',(#39220,#39221,#39222,#39223)) ;
#15693=EDGE_LOOP('',(#39224,#39225,#39226,#39227,#39228,#39229,#39230)) ;
#15694=EDGE_LOOP('',(#39231,#39232,#39233,#39234,#39235,#39236,#39237,#39238,
#39239)) ;
#15695=EDGE_LOOP('',(#39240,#39241,#39242)) ;
#15696=EDGE_LOOP('',(#39243,#39244,#39245,#39246,#39247,#39248)) ;
#15697=EDGE_LOOP('',(#39249,#39250,#39251,#39252)) ;
#15698=EDGE_LOOP('',(#39253,#39254,#39255,#39256)) ;
#15699=EDGE_LOOP('',(#39257,#39258,#39259,#39260)) ;
#15700=EDGE_LOOP('',(#39261,#39262,#39263,#39264)) ;
#15701=EDGE_LOOP('',(#39265,#39266,#39267,#39268)) ;
#15702=EDGE_LOOP('',(#39269,#39270,#39271,#39272)) ;
#15703=EDGE_LOOP('',(#39273,#39274,#39275,#39276,#39277,#39278,#39279,#39280)) ;
#15704=EDGE_LOOP('',(#39281,#39282,#39283)) ;
#15705=EDGE_LOOP('',(#39284,#39285,#39286,#39287)) ;
#15706=EDGE_LOOP('',(#39288,#39289,#39290,#39291)) ;
#15707=EDGE_LOOP('',(#39292,#39293,#39294,#39295,#39296,#39297)) ;
#15708=EDGE_LOOP('',(#39298,#39299,#39300,#39301,#39302)) ;
#15709=EDGE_LOOP('',(#39303,#39304,#39305,#39306)) ;
#15710=EDGE_LOOP('',(#39307,#39308,#39309)) ;
#15711=EDGE_LOOP('',(#39310,#39311,#39312,#39313)) ;
#15712=EDGE_LOOP('',(#39314,#39315,#39316,#39317)) ;
#15713=EDGE_LOOP('',(#39318,#39319,#39320,#39321)) ;
#15714=EDGE_LOOP('',(#39322,#39323,#39324,#39325)) ;
#15715=EDGE_LOOP('',(#39326,#39327,#39328,#39329)) ;
#15716=EDGE_LOOP('',(#39330,#39331,#39332,#39333)) ;
#15717=EDGE_LOOP('',(#39334,#39335,#39336,#39337,#39338,#39339,#39340,#39341,
#39342,#39343,#39344,#39345,#39346,#39347,#39348,#39349,#39350,#39351,#39352,
#39353,#39354,#39355,#39356,#39357,#39358,#39359,#39360,#39361,#39362,#39363,
#39364,#39365,#39366,#39367,#39368,#39369,#39370,#39371,#39372,#39373,#39374,
#39375,#39376,#39377,#39378,#39379,#39380,#39381,#39382,#39383,#39384,#39385,
#39386,#39387,#39388,#39389,#39390,#39391,#39392,#39393,#39394,#39395,#39396,
#39397,#39398,#39399,#39400,#39401,#39402,#39403,#39404,#39405,#39406,#39407,
#39408,#39409,#39410,#39411,#39412,#39413,#39414,#39415,#39416,#39417,#39418,
#39419,#39420,#39421,#39422,#39423,#39424,#39425,#39426,#39427,#39428,#39429,
#39430,#39431,#39432,#39433,#39434,#39435,#39436,#39437,#39438,#39439,#39440,
#39441,#39442,#39443,#39444)) ;
#15718=EDGE_LOOP('',(#39445,#39446,#39447,#39448,#39449,#39450,#39451,#39452)) ;
#15719=EDGE_LOOP('',(#39453)) ;
#15720=EDGE_LOOP('',(#39454,#39455,#39456,#39457,#39458,#39459,#39460,#39461,
#39462,#39463,#39464,#39465,#39466,#39467)) ;
#15721=EDGE_LOOP('',(#39468)) ;
#15722=EDGE_LOOP('',(#39469,#39470,#39471,#39472,#39473,#39474,#39475,#39476,
#39477,#39478,#39479,#39480)) ;
#15723=EDGE_LOOP('',(#39481,#39482,#39483,#39484,#39485,#39486,#39487,#39488,
#39489,#39490,#39491,#39492,#39493,#39494,#39495)) ;
#15724=EDGE_LOOP('',(#39496,#39497,#39498,#39499,#39500,#39501,#39502,#39503,
#39504,#39505,#39506,#39507,#39508,#39509)) ;
#15725=EDGE_LOOP('',(#39510,#39511,#39512,#39513)) ;
#15726=EDGE_LOOP('',(#39514,#39515,#39516,#39517)) ;
#15727=EDGE_LOOP('',(#39518,#39519,#39520,#39521,#39522)) ;
#15728=EDGE_LOOP('',(#39523,#39524,#39525,#39526)) ;
#15729=EDGE_LOOP('',(#39527,#39528,#39529,#39530)) ;
#15730=EDGE_LOOP('',(#39531,#39532,#39533,#39534)) ;
#15731=EDGE_LOOP('',(#39535,#39536,#39537,#39538)) ;
#15732=EDGE_LOOP('',(#39539,#39540,#39541,#39542,#39543,#39544,#39545)) ;
#15733=EDGE_LOOP('',(#39546,#39547,#39548,#39549,#39550,#39551,#39552,#39553)) ;
#15734=EDGE_LOOP('',(#39554,#39555,#39556,#39557,#39558,#39559)) ;
#15735=EDGE_LOOP('',(#39560,#39561,#39562)) ;
#15736=EDGE_LOOP('',(#39563,#39564,#39565,#39566)) ;
#15737=EDGE_LOOP('',(#39567,#39568,#39569,#39570)) ;
#15738=EDGE_LOOP('',(#39571,#39572,#39573,#39574)) ;
#15739=EDGE_LOOP('',(#39575,#39576,#39577,#39578)) ;
#15740=EDGE_LOOP('',(#39579,#39580,#39581,#39582)) ;
#15741=EDGE_LOOP('',(#39583,#39584,#39585,#39586)) ;
#15742=EDGE_LOOP('',(#39587,#39588,#39589,#39590)) ;
#15743=EDGE_LOOP('',(#39591,#39592,#39593,#39594)) ;
#15744=EDGE_LOOP('',(#39595,#39596,#39597,#39598)) ;
#15745=EDGE_LOOP('',(#39599,#39600,#39601,#39602,#39603)) ;
#15746=EDGE_LOOP('',(#39604,#39605,#39606,#39607)) ;
#15747=EDGE_LOOP('',(#39608,#39609,#39610,#39611)) ;
#15748=EDGE_LOOP('',(#39612,#39613,#39614,#39615)) ;
#15749=EDGE_LOOP('',(#39616,#39617,#39618,#39619)) ;
#15750=EDGE_LOOP('',(#39620,#39621,#39622,#39623)) ;
#15751=EDGE_LOOP('',(#39624,#39625,#39626,#39627)) ;
#15752=EDGE_LOOP('',(#39628,#39629,#39630,#39631)) ;
#15753=EDGE_LOOP('',(#39632,#39633,#39634,#39635)) ;
#15754=EDGE_LOOP('',(#39636,#39637,#39638,#39639)) ;
#15755=EDGE_LOOP('',(#39640,#39641,#39642,#39643,#39644,#39645,#39646,#39647,
#39648,#39649,#39650,#39651,#39652,#39653,#39654,#39655,#39656,#39657)) ;
#15756=EDGE_LOOP('',(#39658,#39659,#39660,#39661,#39662,#39663)) ;
#15757=EDGE_LOOP('',(#39664,#39665,#39666,#39667)) ;
#15758=EDGE_LOOP('',(#39668,#39669,#39670,#39671)) ;
#15759=EDGE_LOOP('',(#39672,#39673,#39674,#39675)) ;
#15760=EDGE_LOOP('',(#39676,#39677,#39678,#39679,#39680,#39681,#39682,#39683,
#39684,#39685,#39686,#39687,#39688)) ;
#15761=EDGE_LOOP('',(#39689,#39690,#39691,#39692)) ;
#15762=EDGE_LOOP('',(#39693,#39694,#39695,#39696)) ;
#15763=EDGE_LOOP('',(#39697,#39698,#39699,#39700)) ;
#15764=EDGE_LOOP('',(#39701,#39702,#39703,#39704,#39705,#39706)) ;
#15765=EDGE_LOOP('',(#39707,#39708,#39709,#39710)) ;
#15766=EDGE_LOOP('',(#39711,#39712,#39713,#39714)) ;
#15767=EDGE_LOOP('',(#39715,#39716,#39717,#39718)) ;
#15768=EDGE_LOOP('',(#39719,#39720,#39721,#39722)) ;
#15769=EDGE_LOOP('',(#39723,#39724,#39725,#39726)) ;
#15770=EDGE_LOOP('',(#39727,#39728,#39729,#39730)) ;
#15771=EDGE_LOOP('',(#39731,#39732,#39733,#39734)) ;
#15772=EDGE_LOOP('',(#39735,#39736,#39737,#39738)) ;
#15773=EDGE_LOOP('',(#39739,#39740,#39741,#39742)) ;
#15774=EDGE_LOOP('',(#39743,#39744,#39745,#39746)) ;
#15775=EDGE_LOOP('',(#39747,#39748,#39749,#39750)) ;
#15776=EDGE_LOOP('',(#39751,#39752,#39753,#39754)) ;
#15777=EDGE_LOOP('',(#39755,#39756,#39757,#39758)) ;
#15778=EDGE_LOOP('',(#39759,#39760,#39761,#39762)) ;
#15779=EDGE_LOOP('',(#39763,#39764,#39765,#39766)) ;
#15780=EDGE_LOOP('',(#39767,#39768,#39769,#39770)) ;
#15781=EDGE_LOOP('',(#39771,#39772,#39773,#39774)) ;
#15782=EDGE_LOOP('',(#39775,#39776,#39777,#39778)) ;
#15783=EDGE_LOOP('',(#39779,#39780,#39781,#39782)) ;
#15784=EDGE_LOOP('',(#39783,#39784,#39785,#39786)) ;
#15785=EDGE_LOOP('',(#39787,#39788,#39789,#39790)) ;
#15786=EDGE_LOOP('',(#39791,#39792,#39793,#39794)) ;
#15787=EDGE_LOOP('',(#39795,#39796,#39797,#39798)) ;
#15788=EDGE_LOOP('',(#39799,#39800,#39801,#39802)) ;
#15789=EDGE_LOOP('',(#39803,#39804,#39805,#39806)) ;
#15790=EDGE_LOOP('',(#39807,#39808,#39809,#39810)) ;
#15791=EDGE_LOOP('',(#39811,#39812,#39813,#39814)) ;
#15792=EDGE_LOOP('',(#39815,#39816,#39817,#39818)) ;
#15793=EDGE_LOOP('',(#39819,#39820,#39821,#39822)) ;
#15794=EDGE_LOOP('',(#39823,#39824,#39825,#39826)) ;
#15795=EDGE_LOOP('',(#39827,#39828,#39829,#39830)) ;
#15796=EDGE_LOOP('',(#39831,#39832,#39833,#39834)) ;
#15797=EDGE_LOOP('',(#39835,#39836,#39837,#39838,#39839,#39840,#39841)) ;
#15798=EDGE_LOOP('',(#39842,#39843,#39844,#39845,#39846,#39847,#39848)) ;
#15799=EDGE_LOOP('',(#39849,#39850,#39851,#39852,#39853)) ;
#15800=EDGE_LOOP('',(#39854,#39855,#39856,#39857)) ;
#15801=EDGE_LOOP('',(#39858,#39859,#39860,#39861)) ;
#15802=EDGE_LOOP('',(#39862,#39863,#39864,#39865)) ;
#15803=EDGE_LOOP('',(#39866,#39867,#39868,#39869,#39870)) ;
#15804=EDGE_LOOP('',(#39871,#39872,#39873,#39874,#39875,#39876,#39877,#39878,
#39879,#39880)) ;
#15805=EDGE_LOOP('',(#39881,#39882,#39883,#39884)) ;
#15806=EDGE_LOOP('',(#39885,#39886,#39887,#39888,#39889,#39890,#39891,#39892,
#39893,#39894)) ;
#15807=EDGE_LOOP('',(#39895,#39896,#39897,#39898,#39899)) ;
#15808=EDGE_LOOP('',(#39900,#39901,#39902,#39903,#39904,#39905,#39906,#39907)) ;
#15809=EDGE_LOOP('',(#39908,#39909,#39910,#39911)) ;
#15810=EDGE_LOOP('',(#39912,#39913,#39914,#39915)) ;
#15811=EDGE_LOOP('',(#39916,#39917,#39918,#39919)) ;
#15812=EDGE_LOOP('',(#39920,#39921,#39922,#39923)) ;
#15813=EDGE_LOOP('',(#39924,#39925,#39926,#39927)) ;
#15814=EDGE_LOOP('',(#39928,#39929,#39930,#39931)) ;
#15815=EDGE_LOOP('',(#39932,#39933,#39934,#39935)) ;
#15816=EDGE_LOOP('',(#39936,#39937,#39938,#39939)) ;
#15817=EDGE_LOOP('',(#39940,#39941,#39942,#39943)) ;
#15818=EDGE_LOOP('',(#39944,#39945,#39946,#39947)) ;
#15819=EDGE_LOOP('',(#39948,#39949,#39950,#39951)) ;
#15820=EDGE_LOOP('',(#39952,#39953,#39954,#39955)) ;
#15821=EDGE_LOOP('',(#39956,#39957,#39958,#39959)) ;
#15822=EDGE_LOOP('',(#39960,#39961,#39962,#39963)) ;
#15823=EDGE_LOOP('',(#39964,#39965,#39966,#39967)) ;
#15824=EDGE_LOOP('',(#39968,#39969,#39970,#39971,#39972,#39973,#39974,#39975,
#39976,#39977,#39978,#39979,#39980,#39981,#39982,#39983,#39984)) ;
#15825=EDGE_LOOP('',(#39985,#39986,#39987,#39988)) ;
#15826=EDGE_LOOP('',(#39989,#39990,#39991,#39992,#39993,#39994,#39995,#39996,
#39997,#39998,#39999,#40000,#40001)) ;
#15827=EDGE_LOOP('',(#40002,#40003,#40004,#40005)) ;
#15828=EDGE_LOOP('',(#40006,#40007,#40008,#40009,#40010)) ;
#15829=EDGE_LOOP('',(#40011,#40012,#40013,#40014)) ;
#15830=EDGE_LOOP('',(#40015,#40016,#40017,#40018)) ;
#15831=EDGE_LOOP('',(#40019,#40020,#40021,#40022)) ;
#15832=EDGE_LOOP('',(#40023,#40024,#40025,#40026)) ;
#15833=EDGE_LOOP('',(#40027,#40028,#40029,#40030)) ;
#15834=EDGE_LOOP('',(#40031,#40032,#40033,#40034)) ;
#15835=EDGE_LOOP('',(#40035,#40036,#40037,#40038)) ;
#15836=EDGE_LOOP('',(#40039,#40040,#40041,#40042)) ;
#15837=EDGE_LOOP('',(#40043,#40044,#40045,#40046)) ;
#15838=EDGE_LOOP('',(#40047,#40048,#40049,#40050)) ;
#15839=EDGE_LOOP('',(#40051,#40052,#40053,#40054)) ;
#15840=EDGE_LOOP('',(#40055,#40056,#40057,#40058)) ;
#15841=EDGE_LOOP('',(#40059,#40060,#40061,#40062)) ;
#15842=EDGE_LOOP('',(#40063,#40064,#40065,#40066)) ;
#15843=EDGE_LOOP('',(#40067,#40068,#40069,#40070)) ;
#15844=EDGE_LOOP('',(#40071,#40072,#40073,#40074)) ;
#15845=EDGE_LOOP('',(#40075,#40076,#40077,#40078)) ;
#15846=EDGE_LOOP('',(#40079,#40080,#40081,#40082)) ;
#15847=EDGE_LOOP('',(#40083,#40084,#40085,#40086)) ;
#15848=EDGE_LOOP('',(#40087,#40088,#40089,#40090)) ;
#15849=EDGE_LOOP('',(#40091,#40092,#40093,#40094)) ;
#15850=EDGE_LOOP('',(#40095,#40096,#40097,#40098)) ;
#15851=EDGE_LOOP('',(#40099,#40100,#40101,#40102)) ;
#15852=EDGE_LOOP('',(#40103,#40104,#40105,#40106)) ;
#15853=EDGE_LOOP('',(#40107,#40108,#40109,#40110)) ;
#15854=EDGE_LOOP('',(#40111,#40112,#40113,#40114)) ;
#15855=EDGE_LOOP('',(#40115,#40116,#40117,#40118)) ;
#15856=EDGE_LOOP('',(#40119,#40120,#40121,#40122)) ;
#15857=EDGE_LOOP('',(#40123,#40124,#40125,#40126)) ;
#15858=EDGE_LOOP('',(#40127,#40128,#40129,#40130)) ;
#15859=EDGE_LOOP('',(#40131,#40132,#40133,#40134)) ;
#15860=EDGE_LOOP('',(#40135,#40136,#40137,#40138)) ;
#15861=EDGE_LOOP('',(#40139,#40140,#40141,#40142)) ;
#15862=EDGE_LOOP('',(#40143,#40144,#40145,#40146)) ;
#15863=EDGE_LOOP('',(#40147,#40148,#40149,#40150,#40151)) ;
#15864=EDGE_LOOP('',(#40152,#40153,#40154,#40155)) ;
#15865=EDGE_LOOP('',(#40156,#40157,#40158,#40159)) ;
#15866=EDGE_LOOP('',(#40160,#40161,#40162,#40163)) ;
#15867=EDGE_LOOP('',(#40164,#40165,#40166,#40167)) ;
#15868=EDGE_LOOP('',(#40168,#40169,#40170,#40171)) ;
#15869=EDGE_LOOP('',(#40172,#40173,#40174,#40175)) ;
#15870=EDGE_LOOP('',(#40176,#40177,#40178,#40179)) ;
#15871=EDGE_LOOP('',(#40180,#40181,#40182,#40183)) ;
#15872=EDGE_LOOP('',(#40184,#40185,#40186,#40187)) ;
#15873=EDGE_LOOP('',(#40188,#40189,#40190,#40191)) ;
#15874=EDGE_LOOP('',(#40192,#40193,#40194,#40195)) ;
#15875=EDGE_LOOP('',(#40196,#40197,#40198,#40199)) ;
#15876=EDGE_LOOP('',(#40200,#40201,#40202,#40203)) ;
#15877=EDGE_LOOP('',(#40204,#40205,#40206,#40207)) ;
#15878=EDGE_LOOP('',(#40208,#40209,#40210,#40211)) ;
#15879=EDGE_LOOP('',(#40212,#40213,#40214,#40215)) ;
#15880=EDGE_LOOP('',(#40216,#40217,#40218,#40219)) ;
#15881=EDGE_LOOP('',(#40220,#40221,#40222,#40223)) ;
#15882=EDGE_LOOP('',(#40224,#40225,#40226,#40227,#40228)) ;
#15883=EDGE_LOOP('',(#40229,#40230,#40231,#40232,#40233)) ;
#15884=EDGE_LOOP('',(#40234,#40235,#40236,#40237)) ;
#15885=EDGE_LOOP('',(#40238,#40239,#40240,#40241,#40242,#40243,#40244,#40245,
#40246,#40247,#40248,#40249,#40250,#40251,#40252,#40253,#40254,#40255,#40256,
#40257,#40258,#40259)) ;
#15886=EDGE_LOOP('',(#40260,#40261,#40262,#40263,#40264,#40265,#40266)) ;
#15887=EDGE_LOOP('',(#40267,#40268,#40269,#40270,#40271,#40272,#40273)) ;
#15888=EDGE_LOOP('',(#40274,#40275,#40276,#40277)) ;
#15889=EDGE_LOOP('',(#40278,#40279,#40280,#40281,#40282)) ;
#15890=EDGE_LOOP('',(#40283,#40284,#40285,#40286,#40287,#40288,#40289)) ;
#15891=EDGE_LOOP('',(#40290)) ;
#15892=EDGE_LOOP('',(#40291,#40292,#40293,#40294)) ;
#15893=EDGE_LOOP('',(#40295,#40296,#40297,#40298,#40299,#40300,#40301,#40302,
#40303,#40304)) ;
#15894=EDGE_LOOP('',(#40305,#40306,#40307,#40308,#40309)) ;
#15895=EDGE_LOOP('',(#40310,#40311,#40312,#40313)) ;
#15896=EDGE_LOOP('',(#40314,#40315,#40316,#40317)) ;
#15897=EDGE_LOOP('',(#40318,#40319,#40320,#40321)) ;
#15898=EDGE_LOOP('',(#40322,#40323,#40324,#40325)) ;
#15899=EDGE_LOOP('',(#40326,#40327,#40328,#40329)) ;
#15900=EDGE_LOOP('',(#40330,#40331,#40332,#40333)) ;
#15901=EDGE_LOOP('',(#40334,#40335,#40336,#40337)) ;
#15902=EDGE_LOOP('',(#40338,#40339,#40340,#40341)) ;
#15903=EDGE_LOOP('',(#40342,#40343,#40344,#40345)) ;
#15904=EDGE_LOOP('',(#40346,#40347,#40348,#40349)) ;
#15905=EDGE_LOOP('',(#40350,#40351,#40352,#40353)) ;
#15906=EDGE_LOOP('',(#40354,#40355,#40356,#40357)) ;
#15907=EDGE_LOOP('',(#40358,#40359,#40360,#40361,#40362,#40363)) ;
#15908=EDGE_LOOP('',(#40364,#40365,#40366)) ;
#15909=EDGE_LOOP('',(#40367,#40368,#40369,#40370,#40371,#40372,#40373,#40374)) ;
#15910=EDGE_LOOP('',(#40375,#40376,#40377,#40378,#40379,#40380,#40381,#40382,
#40383,#40384,#40385)) ;
#15911=EDGE_LOOP('',(#40386,#40387,#40388,#40389,#40390,#40391,#40392)) ;
#15912=EDGE_LOOP('',(#40393,#40394,#40395,#40396)) ;
#15913=EDGE_LOOP('',(#40397,#40398,#40399,#40400,#40401,#40402,#40403)) ;
#15914=EDGE_LOOP('',(#40404,#40405,#40406,#40407,#40408,#40409,#40410,#40411,
#40412,#40413)) ;
#15915=EDGE_LOOP('',(#40414,#40415,#40416,#40417)) ;
#15916=EDGE_LOOP('',(#40418,#40419,#40420,#40421,#40422,#40423,#40424,#40425)) ;
#15917=EDGE_LOOP('',(#40426,#40427,#40428,#40429,#40430)) ;
#15918=EDGE_LOOP('',(#40431,#40432,#40433,#40434)) ;
#15919=EDGE_LOOP('',(#40435,#40436,#40437,#40438)) ;
#15920=EDGE_LOOP('',(#40439,#40440,#40441,#40442)) ;
#15921=EDGE_LOOP('',(#40443,#40444,#40445,#40446)) ;
#15922=EDGE_LOOP('',(#40447,#40448,#40449,#40450)) ;
#15923=EDGE_LOOP('',(#40451,#40452,#40453,#40454,#40455,#40456)) ;
#15924=EDGE_LOOP('',(#40457,#40458,#40459,#40460,#40461,#40462,#40463,#40464,
#40465)) ;
#15925=EDGE_LOOP('',(#40466,#40467,#40468,#40469,#40470,#40471,#40472,#40473)) ;
#15926=EDGE_LOOP('',(#40474,#40475,#40476,#40477)) ;
#15927=EDGE_LOOP('',(#40478,#40479,#40480,#40481)) ;
#15928=EDGE_LOOP('',(#40482,#40483,#40484,#40485)) ;
#15929=EDGE_LOOP('',(#40486,#40487,#40488,#40489,#40490,#40491,#40492,#40493,
#40494,#40495)) ;
#15930=EDGE_LOOP('',(#40496,#40497,#40498,#40499,#40500,#40501,#40502,#40503,
#40504,#40505,#40506)) ;
#15931=EDGE_LOOP('',(#40507,#40508,#40509,#40510,#40511,#40512,#40513,#40514,
#40515,#40516,#40517)) ;
#15932=EDGE_LOOP('',(#40518,#40519,#40520,#40521)) ;
#15933=EDGE_LOOP('',(#40522,#40523,#40524,#40525,#40526,#40527)) ;
#15934=EDGE_LOOP('',(#40528,#40529,#40530,#40531,#40532,#40533)) ;
#15935=EDGE_LOOP('',(#40534,#40535,#40536,#40537,#40538)) ;
#15936=EDGE_LOOP('',(#40539,#40540,#40541,#40542,#40543,#40544)) ;
#15937=EDGE_LOOP('',(#40545,#40546,#40547,#40548,#40549)) ;
#15938=EDGE_LOOP('',(#40550,#40551,#40552,#40553,#40554)) ;
#15939=EDGE_LOOP('',(#40555,#40556,#40557,#40558)) ;
#15940=EDGE_LOOP('',(#40559,#40560,#40561,#40562,#40563)) ;
#15941=EDGE_LOOP('',(#40564,#40565,#40566,#40567,#40568)) ;
#15942=EDGE_LOOP('',(#40569,#40570,#40571,#40572)) ;
#15943=EDGE_LOOP('',(#40573,#40574,#40575,#40576)) ;
#15944=EDGE_LOOP('',(#40577,#40578,#40579,#40580,#40581,#40582,#40583,#40584,
#40585,#40586)) ;
#15945=EDGE_LOOP('',(#40587,#40588,#40589,#40590,#40591,#40592,#40593,#40594)) ;
#15946=EDGE_LOOP('',(#40595,#40596,#40597,#40598)) ;
#15947=EDGE_LOOP('',(#40599,#40600,#40601,#40602)) ;
#15948=EDGE_LOOP('',(#40603,#40604,#40605,#40606,#40607,#40608,#40609,#40610,
#40611,#40612,#40613,#40614)) ;
#15949=EDGE_LOOP('',(#40615,#40616,#40617,#40618,#40619,#40620,#40621,#40622)) ;
#15950=EDGE_LOOP('',(#40623,#40624,#40625,#40626)) ;
#15951=EDGE_LOOP('',(#40627,#40628,#40629,#40630,#40631)) ;
#15952=EDGE_LOOP('',(#40632,#40633,#40634,#40635)) ;
#15953=EDGE_LOOP('',(#40636,#40637,#40638,#40639,#40640,#40641)) ;
#15954=EDGE_LOOP('',(#40642,#40643,#40644,#40645)) ;
#15955=EDGE_LOOP('',(#40646,#40647,#40648,#40649)) ;
#15956=EDGE_LOOP('',(#40650,#40651,#40652,#40653,#40654)) ;
#15957=EDGE_LOOP('',(#40655,#40656,#40657,#40658)) ;
#15958=EDGE_LOOP('',(#40659,#40660,#40661,#40662)) ;
#15959=EDGE_LOOP('',(#40663,#40664,#40665,#40666)) ;
#15960=EDGE_LOOP('',(#40667,#40668,#40669,#40670)) ;
#15961=EDGE_LOOP('',(#40671,#40672,#40673,#40674)) ;
#15962=EDGE_LOOP('',(#40675,#40676,#40677,#40678,#40679,#40680,#40681,#40682,
#40683,#40684,#40685,#40686,#40687,#40688,#40689,#40690)) ;
#15963=EDGE_LOOP('',(#40691,#40692,#40693,#40694)) ;
#15964=EDGE_LOOP('',(#40695,#40696,#40697,#40698)) ;
#15965=EDGE_LOOP('',(#40699,#40700,#40701,#40702)) ;
#15966=EDGE_LOOP('',(#40703,#40704,#40705,#40706)) ;
#15967=EDGE_LOOP('',(#40707,#40708,#40709,#40710)) ;
#15968=EDGE_LOOP('',(#40711,#40712,#40713,#40714,#40715)) ;
#15969=EDGE_LOOP('',(#40716,#40717,#40718,#40719)) ;
#15970=EDGE_LOOP('',(#40720,#40721,#40722,#40723)) ;
#15971=EDGE_LOOP('',(#40724,#40725,#40726,#40727)) ;
#15972=EDGE_LOOP('',(#40728,#40729,#40730,#40731,#40732)) ;
#15973=EDGE_LOOP('',(#40733,#40734,#40735,#40736,#40737,#40738)) ;
#15974=EDGE_LOOP('',(#40739,#40740,#40741,#40742)) ;
#15975=EDGE_LOOP('',(#40743,#40744,#40745,#40746,#40747)) ;
#15976=EDGE_LOOP('',(#40748,#40749,#40750,#40751,#40752,#40753)) ;
#15977=EDGE_LOOP('',(#40754,#40755,#40756,#40757,#40758,#40759,#40760,#40761)) ;
#15978=EDGE_LOOP('',(#40762,#40763,#40764,#40765)) ;
#15979=EDGE_LOOP('',(#40766,#40767,#40768,#40769)) ;
#15980=EDGE_LOOP('',(#40770,#40771,#40772,#40773)) ;
#15981=EDGE_LOOP('',(#40774,#40775,#40776,#40777)) ;
#15982=EDGE_LOOP('',(#40778,#40779,#40780,#40781)) ;
#15983=EDGE_LOOP('',(#40782,#40783,#40784,#40785)) ;
#15984=EDGE_LOOP('',(#40786,#40787,#40788,#40789)) ;
#15985=EDGE_LOOP('',(#40790,#40791,#40792,#40793)) ;
#15986=EDGE_LOOP('',(#40794,#40795,#40796,#40797)) ;
#15987=EDGE_LOOP('',(#40798,#40799,#40800,#40801)) ;
#15988=EDGE_LOOP('',(#40802,#40803,#40804,#40805)) ;
#15989=EDGE_LOOP('',(#40806,#40807,#40808,#40809,#40810,#40811,#40812)) ;
#15990=EDGE_LOOP('',(#40813,#40814,#40815,#40816)) ;
#15991=EDGE_LOOP('',(#40817,#40818,#40819,#40820)) ;
#15992=EDGE_LOOP('',(#40821,#40822,#40823,#40824)) ;
#15993=EDGE_LOOP('',(#40825,#40826,#40827,#40828)) ;
#15994=EDGE_LOOP('',(#40829,#40830,#40831,#40832)) ;
#15995=EDGE_LOOP('',(#40833,#40834,#40835,#40836)) ;
#15996=EDGE_LOOP('',(#40837,#40838,#40839,#40840)) ;
#15997=EDGE_LOOP('',(#40841,#40842,#40843,#40844)) ;
#15998=EDGE_LOOP('',(#40845,#40846,#40847,#40848)) ;
#15999=EDGE_LOOP('',(#40849,#40850,#40851,#40852)) ;
#16000=EDGE_LOOP('',(#40853,#40854,#40855,#40856)) ;
#16001=EDGE_LOOP('',(#40857,#40858,#40859,#40860,#40861,#40862,#40863)) ;
#16002=EDGE_LOOP('',(#40864,#40865,#40866,#40867)) ;
#16003=EDGE_LOOP('',(#40868,#40869,#40870,#40871)) ;
#16004=EDGE_LOOP('',(#40872,#40873,#40874,#40875)) ;
#16005=EDGE_LOOP('',(#40876,#40877,#40878,#40879)) ;
#16006=EDGE_LOOP('',(#40880,#40881,#40882,#40883)) ;
#16007=EDGE_LOOP('',(#40884,#40885,#40886,#40887)) ;
#16008=EDGE_LOOP('',(#40888,#40889,#40890,#40891)) ;
#16009=EDGE_LOOP('',(#40892,#40893,#40894,#40895)) ;
#16010=EDGE_LOOP('',(#40896,#40897,#40898,#40899)) ;
#16011=EDGE_LOOP('',(#40900,#40901,#40902,#40903)) ;
#16012=EDGE_LOOP('',(#40904,#40905,#40906,#40907)) ;
#16013=EDGE_LOOP('',(#40908,#40909,#40910,#40911,#40912,#40913,#40914)) ;
#16014=EDGE_LOOP('',(#40915,#40916,#40917,#40918)) ;
#16015=EDGE_LOOP('',(#40919,#40920,#40921,#40922)) ;
#16016=EDGE_LOOP('',(#40923,#40924,#40925,#40926)) ;
#16017=EDGE_LOOP('',(#40927,#40928,#40929,#40930)) ;
#16018=EDGE_LOOP('',(#40931,#40932,#40933,#40934)) ;
#16019=EDGE_LOOP('',(#40935,#40936,#40937,#40938)) ;
#16020=EDGE_LOOP('',(#40939,#40940,#40941,#40942)) ;
#16021=EDGE_LOOP('',(#40943,#40944,#40945,#40946)) ;
#16022=EDGE_LOOP('',(#40947,#40948,#40949,#40950)) ;
#16023=EDGE_LOOP('',(#40951,#40952,#40953,#40954)) ;
#16024=EDGE_LOOP('',(#40955,#40956,#40957,#40958)) ;
#16025=EDGE_LOOP('',(#40959,#40960,#40961,#40962)) ;
#16026=EDGE_LOOP('',(#40963,#40964,#40965,#40966)) ;
#16027=EDGE_LOOP('',(#40967,#40968,#40969,#40970)) ;
#16028=EDGE_LOOP('',(#40971,#40972,#40973,#40974)) ;
#16029=EDGE_LOOP('',(#40975,#40976,#40977,#40978)) ;
#16030=EDGE_LOOP('',(#40979,#40980,#40981,#40982)) ;
#16031=EDGE_LOOP('',(#40983,#40984,#40985,#40986)) ;
#16032=EDGE_LOOP('',(#40987,#40988,#40989,#40990,#40991,#40992,#40993)) ;
#16033=EDGE_LOOP('',(#40994,#40995,#40996,#40997)) ;
#16034=EDGE_LOOP('',(#40998,#40999,#41000,#41001)) ;
#16035=EDGE_LOOP('',(#41002,#41003,#41004,#41005)) ;
#16036=EDGE_LOOP('',(#41006,#41007,#41008,#41009)) ;
#16037=EDGE_LOOP('',(#41010,#41011,#41012,#41013)) ;
#16038=EDGE_LOOP('',(#41014,#41015,#41016,#41017)) ;
#16039=EDGE_LOOP('',(#41018,#41019,#41020,#41021)) ;
#16040=EDGE_LOOP('',(#41022,#41023,#41024,#41025)) ;
#16041=EDGE_LOOP('',(#41026,#41027,#41028,#41029)) ;
#16042=EDGE_LOOP('',(#41030,#41031,#41032,#41033)) ;
#16043=EDGE_LOOP('',(#41034,#41035,#41036,#41037)) ;
#16044=EDGE_LOOP('',(#41038,#41039,#41040,#41041)) ;
#16045=EDGE_LOOP('',(#41042,#41043,#41044,#41045)) ;
#16046=EDGE_LOOP('',(#41046,#41047,#41048,#41049)) ;
#16047=EDGE_LOOP('',(#41050,#41051,#41052,#41053)) ;
#16048=EDGE_LOOP('',(#41054,#41055,#41056,#41057)) ;
#16049=EDGE_LOOP('',(#41058,#41059,#41060,#41061)) ;
#16050=EDGE_LOOP('',(#41062,#41063,#41064,#41065)) ;
#16051=EDGE_LOOP('',(#41066,#41067,#41068,#41069)) ;
#16052=EDGE_LOOP('',(#41070,#41071,#41072,#41073)) ;
#16053=EDGE_LOOP('',(#41074,#41075,#41076,#41077)) ;
#16054=EDGE_LOOP('',(#41078,#41079,#41080,#41081)) ;
#16055=EDGE_LOOP('',(#41082,#41083,#41084,#41085)) ;
#16056=EDGE_LOOP('',(#41086,#41087,#41088,#41089)) ;
#16057=EDGE_LOOP('',(#41090,#41091,#41092,#41093,#41094,#41095,#41096,#41097,
#41098,#41099,#41100)) ;
#16058=EDGE_LOOP('',(#41101,#41102,#41103,#41104)) ;
#16059=EDGE_LOOP('',(#41105,#41106,#41107,#41108)) ;
#16060=EDGE_LOOP('',(#41109,#41110,#41111,#41112)) ;
#16061=EDGE_LOOP('',(#41113,#41114,#41115,#41116)) ;
#16062=EDGE_LOOP('',(#41117,#41118,#41119,#41120)) ;
#16063=EDGE_LOOP('',(#41121,#41122,#41123,#41124)) ;
#16064=EDGE_LOOP('',(#41125,#41126,#41127,#41128)) ;
#16065=EDGE_LOOP('',(#41129,#41130,#41131,#41132)) ;
#16066=EDGE_LOOP('',(#41133,#41134,#41135,#41136)) ;
#16067=EDGE_LOOP('',(#41137,#41138,#41139,#41140)) ;
#16068=EDGE_LOOP('',(#41141,#41142,#41143,#41144)) ;
#16069=EDGE_LOOP('',(#41145,#41146,#41147,#41148)) ;
#16070=EDGE_LOOP('',(#41149,#41150,#41151,#41152)) ;
#16071=EDGE_LOOP('',(#41153,#41154,#41155,#41156)) ;
#16072=EDGE_LOOP('',(#41157,#41158,#41159,#41160)) ;
#16073=EDGE_LOOP('',(#41161,#41162,#41163,#41164)) ;
#16074=EDGE_LOOP('',(#41165,#41166,#41167,#41168)) ;
#16075=EDGE_LOOP('',(#41169,#41170,#41171,#41172,#41173,#41174,#41175,#41176,
#41177,#41178,#41179)) ;
#16076=EDGE_LOOP('',(#41180,#41181,#41182,#41183)) ;
#16077=EDGE_LOOP('',(#41184,#41185,#41186,#41187)) ;
#16078=EDGE_LOOP('',(#41188,#41189,#41190,#41191)) ;
#16079=EDGE_LOOP('',(#41192,#41193,#41194,#41195)) ;
#16080=EDGE_LOOP('',(#41196,#41197,#41198,#41199)) ;
#16081=EDGE_LOOP('',(#41200,#41201,#41202,#41203)) ;
#16082=EDGE_LOOP('',(#41204,#41205,#41206,#41207)) ;
#16083=EDGE_LOOP('',(#41208,#41209,#41210,#41211)) ;
#16084=EDGE_LOOP('',(#41212,#41213,#41214,#41215)) ;
#16085=EDGE_LOOP('',(#41216,#41217,#41218,#41219)) ;
#16086=EDGE_LOOP('',(#41220,#41221,#41222,#41223)) ;
#16087=EDGE_LOOP('',(#41224,#41225,#41226,#41227)) ;
#16088=EDGE_LOOP('',(#41228,#41229,#41230,#41231)) ;
#16089=EDGE_LOOP('',(#41232,#41233,#41234,#41235)) ;
#16090=EDGE_LOOP('',(#41236,#41237,#41238,#41239)) ;
#16091=EDGE_LOOP('',(#41240,#41241,#41242,#41243)) ;
#16092=EDGE_LOOP('',(#41244,#41245,#41246,#41247)) ;
#16093=EDGE_LOOP('',(#41248,#41249,#41250,#41251)) ;
#16094=EDGE_LOOP('',(#41252,#41253,#41254,#41255)) ;
#16095=EDGE_LOOP('',(#41256,#41257,#41258,#41259)) ;
#16096=EDGE_LOOP('',(#41260,#41261,#41262,#41263)) ;
#16097=EDGE_LOOP('',(#41264,#41265,#41266,#41267)) ;
#16098=EDGE_LOOP('',(#41268,#41269,#41270,#41271)) ;
#16099=EDGE_LOOP('',(#41272,#41273,#41274,#41275)) ;
#16100=EDGE_LOOP('',(#41276,#41277,#41278,#41279)) ;
#16101=EDGE_LOOP('',(#41280,#41281,#41282,#41283)) ;
#16102=EDGE_LOOP('',(#41284,#41285,#41286,#41287)) ;
#16103=EDGE_LOOP('',(#41288,#41289,#41290,#41291)) ;
#16104=EDGE_LOOP('',(#41292,#41293,#41294,#41295)) ;
#16105=EDGE_LOOP('',(#41296,#41297,#41298,#41299,#41300,#41301,#41302,#41303,
#41304,#41305,#41306,#41307,#41308)) ;
#16106=EDGE_LOOP('',(#41309,#41310,#41311,#41312)) ;
#16107=EDGE_LOOP('',(#41313,#41314,#41315,#41316,#41317,#41318,#41319)) ;
#16108=EDGE_LOOP('',(#41320,#41321,#41322,#41323,#41324,#41325,#41326)) ;
#16109=EDGE_LOOP('',(#41327,#41328,#41329,#41330)) ;
#16110=EDGE_LOOP('',(#41331,#41332,#41333,#41334)) ;
#16111=EDGE_LOOP('',(#41335,#41336,#41337,#41338)) ;
#16112=EDGE_LOOP('',(#41339,#41340,#41341,#41342)) ;
#16113=EDGE_LOOP('',(#41343,#41344,#41345,#41346)) ;
#16114=EDGE_LOOP('',(#41347,#41348,#41349,#41350)) ;
#16115=EDGE_LOOP('',(#41351,#41352,#41353,#41354)) ;
#16116=EDGE_LOOP('',(#41355,#41356,#41357,#41358)) ;
#16117=EDGE_LOOP('',(#41359,#41360,#41361,#41362)) ;
#16118=EDGE_LOOP('',(#41363,#41364,#41365,#41366)) ;
#16119=EDGE_LOOP('',(#41367,#41368,#41369,#41370)) ;
#16120=EDGE_LOOP('',(#41371,#41372,#41373,#41374)) ;
#16121=EDGE_LOOP('',(#41375,#41376,#41377,#41378)) ;
#16122=EDGE_LOOP('',(#41379,#41380,#41381,#41382)) ;
#16123=EDGE_LOOP('',(#41383,#41384,#41385,#41386)) ;
#16124=EDGE_LOOP('',(#41387,#41388,#41389,#41390)) ;
#16125=EDGE_LOOP('',(#41391,#41392,#41393,#41394)) ;
#16126=EDGE_LOOP('',(#41395,#41396,#41397,#41398)) ;
#16127=EDGE_LOOP('',(#41399,#41400,#41401,#41402)) ;
#16128=EDGE_LOOP('',(#41403,#41404,#41405,#41406)) ;
#16129=EDGE_LOOP('',(#41407,#41408,#41409,#41410)) ;
#16130=EDGE_LOOP('',(#41411,#41412,#41413,#41414)) ;
#16131=EDGE_LOOP('',(#41415,#41416,#41417,#41418)) ;
#16132=EDGE_LOOP('',(#41419,#41420,#41421,#41422)) ;
#16133=EDGE_LOOP('',(#41423,#41424,#41425,#41426)) ;
#16134=EDGE_LOOP('',(#41427,#41428,#41429,#41430)) ;
#16135=EDGE_LOOP('',(#41431,#41432,#41433,#41434)) ;
#16136=EDGE_LOOP('',(#41435,#41436,#41437,#41438)) ;
#16137=EDGE_LOOP('',(#41439,#41440,#41441,#41442)) ;
#16138=EDGE_LOOP('',(#41443,#41444,#41445,#41446)) ;
#16139=EDGE_LOOP('',(#41447,#41448,#41449,#41450)) ;
#16140=EDGE_LOOP('',(#41451,#41452,#41453,#41454)) ;
#16141=EDGE_LOOP('',(#41455,#41456,#41457,#41458)) ;
#16142=EDGE_LOOP('',(#41459,#41460,#41461,#41462)) ;
#16143=EDGE_LOOP('',(#41463,#41464,#41465,#41466)) ;
#16144=EDGE_LOOP('',(#41467,#41468,#41469,#41470)) ;
#16145=EDGE_LOOP('',(#41471,#41472,#41473,#41474)) ;
#16146=EDGE_LOOP('',(#41475,#41476,#41477,#41478)) ;
#16147=EDGE_LOOP('',(#41479,#41480,#41481,#41482)) ;
#16148=EDGE_LOOP('',(#41483,#41484,#41485,#41486)) ;
#16149=EDGE_LOOP('',(#41487,#41488,#41489,#41490)) ;
#16150=EDGE_LOOP('',(#41491,#41492,#41493,#41494)) ;
#16151=EDGE_LOOP('',(#41495,#41496,#41497,#41498)) ;
#16152=EDGE_LOOP('',(#41499,#41500,#41501,#41502)) ;
#16153=EDGE_LOOP('',(#41503,#41504,#41505,#41506)) ;
#16154=EDGE_LOOP('',(#41507,#41508,#41509,#41510)) ;
#16155=EDGE_LOOP('',(#41511,#41512,#41513,#41514)) ;
#16156=EDGE_LOOP('',(#41515,#41516,#41517,#41518)) ;
#16157=EDGE_LOOP('',(#41519,#41520,#41521,#41522,#41523,#41524)) ;
#16158=EDGE_LOOP('',(#41525,#41526,#41527,#41528)) ;
#16159=EDGE_LOOP('',(#41529,#41530,#41531,#41532)) ;
#16160=EDGE_LOOP('',(#41533,#41534,#41535,#41536)) ;
#16161=EDGE_LOOP('',(#41537,#41538,#41539,#41540)) ;
#16162=EDGE_LOOP('',(#41541,#41542,#41543,#41544)) ;
#16163=EDGE_LOOP('',(#41545,#41546,#41547,#41548,#41549)) ;
#16164=EDGE_LOOP('',(#41550,#41551,#41552,#41553,#41554,#41555,#41556,#41557,
#41558,#41559,#41560)) ;
#16165=EDGE_LOOP('',(#41561,#41562,#41563,#41564,#41565)) ;
#16166=EDGE_LOOP('',(#41566,#41567,#41568,#41569)) ;
#16167=EDGE_LOOP('',(#41570,#41571,#41572,#41573)) ;
#16168=EDGE_LOOP('',(#41574,#41575,#41576,#41577)) ;
#16169=EDGE_LOOP('',(#41578,#41579,#41580,#41581)) ;
#16170=EDGE_LOOP('',(#41582,#41583,#41584,#41585)) ;
#16171=EDGE_LOOP('',(#41586,#41587,#41588,#41589)) ;
#16172=EDGE_LOOP('',(#41590,#41591,#41592,#41593,#41594,#41595,#41596,#41597,
#41598,#41599,#41600,#41601,#41602,#41603,#41604,#41605,#41606)) ;
#16173=EDGE_LOOP('',(#41607,#41608,#41609,#41610)) ;
#16174=EDGE_LOOP('',(#41611,#41612,#41613,#41614,#41615)) ;
#16175=EDGE_LOOP('',(#41616,#41617,#41618,#41619)) ;
#16176=EDGE_LOOP('',(#41620,#41621,#41622,#41623)) ;
#16177=EDGE_LOOP('',(#41624,#41625,#41626,#41627,#41628)) ;
#16178=EDGE_LOOP('',(#41629,#41630,#41631,#41632)) ;
#16179=EDGE_LOOP('',(#41633,#41634,#41635,#41636)) ;
#16180=EDGE_LOOP('',(#41637,#41638,#41639,#41640)) ;
#16181=EDGE_LOOP('',(#41641,#41642,#41643,#41644)) ;
#16182=EDGE_LOOP('',(#41645,#41646,#41647,#41648)) ;
#16183=EDGE_LOOP('',(#41649,#41650,#41651,#41652)) ;
#16184=EDGE_LOOP('',(#41653,#41654,#41655,#41656,#41657)) ;
#16185=EDGE_LOOP('',(#41658,#41659,#41660,#41661,#41662)) ;
#16186=EDGE_LOOP('',(#41663,#41664,#41665,#41666)) ;
#16187=EDGE_LOOP('',(#41667,#41668,#41669,#41670,#41671)) ;
#16188=EDGE_LOOP('',(#41672,#41673,#41674,#41675,#41676,#41677,#41678,#41679)) ;
#16189=EDGE_LOOP('',(#41680,#41681,#41682,#41683,#41684)) ;
#16190=EDGE_LOOP('',(#41685,#41686,#41687,#41688,#41689)) ;
#16191=EDGE_LOOP('',(#41690,#41691,#41692,#41693,#41694,#41695,#41696,#41697,
#41698,#41699,#41700,#41701,#41702,#41703,#41704)) ;
#16192=EDGE_LOOP('',(#41705,#41706,#41707,#41708,#41709)) ;
#16193=EDGE_LOOP('',(#41710,#41711,#41712,#41713)) ;
#16194=EDGE_LOOP('',(#41714,#41715,#41716,#41717)) ;
#16195=EDGE_LOOP('',(#41718,#41719,#41720,#41721)) ;
#16196=EDGE_LOOP('',(#41722,#41723,#41724,#41725)) ;
#16197=EDGE_LOOP('',(#41726,#41727,#41728,#41729)) ;
#16198=EDGE_LOOP('',(#41730,#41731,#41732,#41733)) ;
#16199=EDGE_LOOP('',(#41734,#41735,#41736,#41737)) ;
#16200=EDGE_LOOP('',(#41738,#41739,#41740)) ;
#16201=EDGE_LOOP('',(#41741,#41742,#41743,#41744)) ;
#16202=EDGE_LOOP('',(#41745,#41746,#41747)) ;
#16203=EDGE_LOOP('',(#41748,#41749,#41750,#41751)) ;
#16204=EDGE_LOOP('',(#41752,#41753,#41754,#41755)) ;
#16205=EDGE_LOOP('',(#41756,#41757,#41758,#41759,#41760)) ;
#16206=EDGE_LOOP('',(#41761,#41762,#41763,#41764)) ;
#16207=EDGE_LOOP('',(#41765,#41766,#41767,#41768)) ;
#16208=EDGE_LOOP('',(#41769,#41770,#41771,#41772)) ;
#16209=EDGE_LOOP('',(#41773,#41774,#41775,#41776)) ;
#16210=EDGE_LOOP('',(#41777,#41778,#41779)) ;
#16211=EDGE_LOOP('',(#41780,#41781,#41782,#41783)) ;
#16212=EDGE_LOOP('',(#41784,#41785,#41786,#41787)) ;
#16213=EDGE_LOOP('',(#41788,#41789,#41790,#41791)) ;
#16214=EDGE_LOOP('',(#41792,#41793,#41794,#41795)) ;
#16215=EDGE_LOOP('',(#41796,#41797,#41798,#41799)) ;
#16216=EDGE_LOOP('',(#41800,#41801,#41802,#41803)) ;
#16217=EDGE_LOOP('',(#41804,#41805,#41806,#41807)) ;
#16218=EDGE_LOOP('',(#41808,#41809,#41810,#41811)) ;
#16219=EDGE_LOOP('',(#41812,#41813,#41814,#41815)) ;
#16220=EDGE_LOOP('',(#41816,#41817,#41818,#41819)) ;
#16221=EDGE_LOOP('',(#41820,#41821,#41822,#41823)) ;
#16222=EDGE_LOOP('',(#41824,#41825,#41826,#41827)) ;
#16223=EDGE_LOOP('',(#41828,#41829,#41830,#41831)) ;
#16224=EDGE_LOOP('',(#41832,#41833,#41834,#41835)) ;
#16225=EDGE_LOOP('',(#41836,#41837,#41838,#41839)) ;
#16226=EDGE_LOOP('',(#41840,#41841,#41842,#41843)) ;
#16227=EDGE_LOOP('',(#41844,#41845,#41846,#41847)) ;
#16228=EDGE_LOOP('',(#41848,#41849,#41850,#41851,#41852)) ;
#16229=EDGE_LOOP('',(#41853,#41854,#41855,#41856)) ;
#16230=EDGE_LOOP('',(#41857,#41858,#41859,#41860)) ;
#16231=EDGE_LOOP('',(#41861,#41862,#41863,#41864)) ;
#16232=EDGE_LOOP('',(#41865,#41866,#41867,#41868,#41869)) ;
#16233=EDGE_LOOP('',(#41870,#41871,#41872,#41873)) ;
#16234=EDGE_LOOP('',(#41874,#41875,#41876,#41877)) ;
#16235=EDGE_LOOP('',(#41878,#41879,#41880,#41881)) ;
#16236=EDGE_LOOP('',(#41882,#41883,#41884,#41885)) ;
#16237=EDGE_LOOP('',(#41886,#41887,#41888,#41889)) ;
#16238=EDGE_LOOP('',(#41890,#41891,#41892,#41893)) ;
#16239=EDGE_LOOP('',(#41894,#41895,#41896,#41897)) ;
#16240=EDGE_LOOP('',(#41898,#41899,#41900,#41901)) ;
#16241=EDGE_LOOP('',(#41902,#41903,#41904,#41905)) ;
#16242=EDGE_LOOP('',(#41906,#41907,#41908,#41909,#41910)) ;
#16243=EDGE_LOOP('',(#41911,#41912,#41913,#41914)) ;
#16244=EDGE_LOOP('',(#41915,#41916,#41917,#41918,#41919)) ;
#16245=EDGE_LOOP('',(#41920,#41921,#41922,#41923)) ;
#16246=EDGE_LOOP('',(#41924,#41925,#41926,#41927)) ;
#16247=EDGE_LOOP('',(#41928,#41929,#41930,#41931)) ;
#16248=EDGE_LOOP('',(#41932,#41933,#41934,#41935)) ;
#16249=EDGE_LOOP('',(#41936,#41937,#41938,#41939)) ;
#16250=EDGE_LOOP('',(#41940,#41941,#41942,#41943)) ;
#16251=EDGE_LOOP('',(#41944,#41945,#41946,#41947)) ;
#16252=EDGE_LOOP('',(#41948,#41949,#41950,#41951)) ;
#16253=EDGE_LOOP('',(#41952,#41953,#41954,#41955)) ;
#16254=EDGE_LOOP('',(#41956,#41957,#41958,#41959)) ;
#16255=EDGE_LOOP('',(#41960,#41961,#41962,#41963)) ;
#16256=EDGE_LOOP('',(#41964,#41965,#41966,#41967)) ;
#16257=EDGE_LOOP('',(#41968,#41969,#41970,#41971)) ;
#16258=EDGE_LOOP('',(#41972,#41973,#41974,#41975)) ;
#16259=EDGE_LOOP('',(#41976,#41977,#41978,#41979)) ;
#16260=EDGE_LOOP('',(#41980,#41981,#41982,#41983)) ;
#16261=EDGE_LOOP('',(#41984,#41985,#41986,#41987)) ;
#16262=EDGE_LOOP('',(#41988)) ;
#16263=EDGE_LOOP('',(#41989,#41990,#41991,#41992)) ;
#16264=EDGE_LOOP('',(#41993,#41994,#41995,#41996)) ;
#16265=EDGE_LOOP('',(#41997,#41998,#41999,#42000)) ;
#16266=EDGE_LOOP('',(#42001,#42002,#42003,#42004)) ;
#16267=EDGE_LOOP('',(#42005,#42006,#42007,#42008)) ;
#16268=EDGE_LOOP('',(#42009,#42010,#42011,#42012)) ;
#16269=EDGE_LOOP('',(#42013,#42014,#42015,#42016)) ;
#16270=EDGE_LOOP('',(#42017,#42018,#42019,#42020)) ;
#16271=EDGE_LOOP('',(#42021,#42022,#42023,#42024)) ;
#16272=EDGE_LOOP('',(#42025,#42026,#42027,#42028)) ;
#16273=EDGE_LOOP('',(#42029,#42030,#42031,#42032)) ;
#16274=EDGE_LOOP('',(#42033,#42034,#42035,#42036)) ;
#16275=EDGE_LOOP('',(#42037,#42038,#42039,#42040)) ;
#16276=EDGE_LOOP('',(#42041,#42042,#42043,#42044)) ;
#16277=EDGE_LOOP('',(#42045,#42046,#42047,#42048)) ;
#16278=EDGE_LOOP('',(#42049,#42050,#42051,#42052)) ;
#16279=EDGE_LOOP('',(#42053,#42054,#42055,#42056)) ;
#16280=EDGE_LOOP('',(#42057,#42058,#42059,#42060)) ;
#16281=EDGE_LOOP('',(#42061,#42062,#42063,#42064)) ;
#16282=EDGE_LOOP('',(#42065,#42066,#42067,#42068)) ;
#16283=EDGE_LOOP('',(#42069,#42070,#42071,#42072)) ;
#16284=EDGE_LOOP('',(#42073,#42074,#42075,#42076)) ;
#16285=EDGE_LOOP('',(#42077,#42078,#42079,#42080)) ;
#16286=EDGE_LOOP('',(#42081,#42082,#42083,#42084)) ;
#16287=EDGE_LOOP('',(#42085,#42086,#42087,#42088)) ;
#16288=EDGE_LOOP('',(#42089,#42090,#42091,#42092)) ;
#16289=EDGE_LOOP('',(#42093,#42094,#42095,#42096)) ;
#16290=EDGE_LOOP('',(#42097,#42098,#42099,#42100)) ;
#16291=EDGE_LOOP('',(#42101,#42102,#42103,#42104,#42105,#42106)) ;
#16292=EDGE_LOOP('',(#42107,#42108,#42109,#42110)) ;
#16293=EDGE_LOOP('',(#42111,#42112,#42113,#42114)) ;
#16294=EDGE_LOOP('',(#42115,#42116,#42117,#42118)) ;
#16295=EDGE_LOOP('',(#42119,#42120,#42121,#42122)) ;
#16296=EDGE_LOOP('',(#42123,#42124,#42125,#42126)) ;
#16297=EDGE_LOOP('',(#42127,#42128,#42129,#42130)) ;
#16298=EDGE_LOOP('',(#42131,#42132,#42133,#42134)) ;
#16299=EDGE_LOOP('',(#42135,#42136,#42137,#42138)) ;
#16300=EDGE_LOOP('',(#42139,#42140,#42141,#42142)) ;
#16301=EDGE_LOOP('',(#42143,#42144,#42145,#42146)) ;
#16302=EDGE_LOOP('',(#42147,#42148,#42149,#42150)) ;
#16303=EDGE_LOOP('',(#42151,#42152,#42153,#42154)) ;
#16304=EDGE_LOOP('',(#42155,#42156,#42157,#42158)) ;
#16305=EDGE_LOOP('',(#42159,#42160,#42161,#42162)) ;
#16306=EDGE_LOOP('',(#42163,#42164,#42165,#42166)) ;
#16307=EDGE_LOOP('',(#42167,#42168,#42169,#42170)) ;
#16308=EDGE_LOOP('',(#42171,#42172,#42173,#42174)) ;
#16309=EDGE_LOOP('',(#42175,#42176,#42177,#42178,#42179,#42180,#42181,#42182,
#42183,#42184,#42185,#42186,#42187,#42188)) ;
#16310=EDGE_LOOP('',(#42189,#42190,#42191,#42192)) ;
#16311=EDGE_LOOP('',(#42193,#42194,#42195,#42196)) ;
#16312=EDGE_LOOP('',(#42197,#42198,#42199,#42200)) ;
#16313=EDGE_LOOP('',(#42201,#42202,#42203,#42204)) ;
#16314=EDGE_LOOP('',(#42205,#42206,#42207,#42208)) ;
#16315=EDGE_LOOP('',(#42209,#42210,#42211,#42212)) ;
#16316=EDGE_LOOP('',(#42213,#42214,#42215,#42216,#42217,#42218,#42219,#42220,
#42221,#42222,#42223,#42224)) ;
#16317=EDGE_LOOP('',(#42225,#42226,#42227,#42228)) ;
#16318=EDGE_LOOP('',(#42229,#42230,#42231,#42232)) ;
#16319=EDGE_LOOP('',(#42233,#42234,#42235,#42236)) ;
#16320=EDGE_LOOP('',(#42237,#42238,#42239,#42240)) ;
#16321=EDGE_LOOP('',(#42241,#42242,#42243,#42244)) ;
#16322=EDGE_LOOP('',(#42245,#42246,#42247,#42248)) ;
#16323=EDGE_LOOP('',(#42249,#42250,#42251,#42252)) ;
#16324=EDGE_LOOP('',(#42253,#42254,#42255,#42256,#42257,#42258,#42259,#42260,
#42261,#42262,#42263,#42264,#42265,#42266,#42267)) ;
#16325=EDGE_LOOP('',(#42268,#42269,#42270,#42271)) ;
#16326=EDGE_LOOP('',(#42272,#42273,#42274,#42275)) ;
#16327=EDGE_LOOP('',(#42276,#42277,#42278,#42279)) ;
#16328=EDGE_LOOP('',(#42280,#42281,#42282,#42283)) ;
#16329=EDGE_LOOP('',(#42284,#42285,#42286,#42287)) ;
#16330=EDGE_LOOP('',(#42288,#42289,#42290,#42291)) ;
#16331=EDGE_LOOP('',(#42292,#42293,#42294,#42295)) ;
#16332=EDGE_LOOP('',(#42296,#42297,#42298,#42299,#42300,#42301,#42302,#42303,
#42304,#42305,#42306,#42307,#42308,#42309)) ;
#16333=EDGE_LOOP('',(#42310,#42311,#42312,#42313)) ;
#16334=EDGE_LOOP('',(#42314,#42315,#42316,#42317)) ;
#16335=EDGE_LOOP('',(#42318,#42319,#42320,#42321)) ;
#16336=EDGE_LOOP('',(#42322,#42323,#42324,#42325)) ;
#16337=EDGE_LOOP('',(#42326,#42327,#42328,#42329)) ;
#16338=EDGE_LOOP('',(#42330,#42331,#42332,#42333)) ;
#16339=EDGE_LOOP('',(#42334,#42335,#42336,#42337)) ;
#16340=EDGE_LOOP('',(#42338,#42339,#42340,#42341,#42342,#42343,#42344,#42345,
#42346,#42347,#42348,#42349,#42350,#42351)) ;
#16341=EDGE_LOOP('',(#42352,#42353,#42354,#42355)) ;
#16342=EDGE_LOOP('',(#42356,#42357,#42358,#42359)) ;
#16343=EDGE_LOOP('',(#42360,#42361,#42362,#42363)) ;
#16344=EDGE_LOOP('',(#42364,#42365,#42366,#42367)) ;
#16345=EDGE_LOOP('',(#42368,#42369,#42370,#42371)) ;
#16346=EDGE_LOOP('',(#42372,#42373,#42374,#42375)) ;
#16347=EDGE_LOOP('',(#42376,#42377,#42378,#42379,#42380,#42381,#42382,#42383,
#42384,#42385,#42386,#42387)) ;
#16348=EDGE_LOOP('',(#42388)) ;
#16349=EDGE_LOOP('',(#42389,#42390,#42391,#42392)) ;
#16350=EDGE_LOOP('',(#42393,#42394,#42395,#42396)) ;
#16351=EDGE_LOOP('',(#42397)) ;
#16352=EDGE_LOOP('',(#42398,#42399,#42400,#42401)) ;
#16353=EDGE_LOOP('',(#42402,#42403,#42404,#42405,#42406,#42407)) ;
#16354=EDGE_LOOP('',(#42408,#42409,#42410,#42411)) ;
#16355=EDGE_LOOP('',(#42412,#42413,#42414,#42415,#42416)) ;
#16356=EDGE_LOOP('',(#42417,#42418,#42419,#42420)) ;
#16357=EDGE_LOOP('',(#42421,#42422,#42423,#42424)) ;
#16358=EDGE_LOOP('',(#42425,#42426,#42427,#42428)) ;
#16359=EDGE_LOOP('',(#42429,#42430,#42431,#42432)) ;
#16360=EDGE_LOOP('',(#42433,#42434,#42435,#42436)) ;
#16361=EDGE_LOOP('',(#42437,#42438,#42439,#42440,#42441,#42442,#42443)) ;
#16362=EDGE_LOOP('',(#42444,#42445,#42446,#42447)) ;
#16363=EDGE_LOOP('',(#42448,#42449,#42450,#42451,#42452,#42453,#42454,#42455,
#42456,#42457,#42458,#42459,#42460)) ;
#16364=EDGE_LOOP('',(#42461,#42462,#42463,#42464)) ;
#16365=EDGE_LOOP('',(#42465,#42466,#42467,#42468)) ;
#16366=EDGE_LOOP('',(#42469,#42470,#42471,#42472,#42473,#42474,#42475,#42476,
#42477)) ;
#16367=EDGE_LOOP('',(#42478,#42479,#42480,#42481)) ;
#16368=EDGE_LOOP('',(#42482,#42483,#42484,#42485)) ;
#16369=EDGE_LOOP('',(#42486,#42487,#42488,#42489,#42490)) ;
#16370=EDGE_LOOP('',(#42491,#42492,#42493,#42494)) ;
#16371=EDGE_LOOP('',(#42495,#42496,#42497,#42498)) ;
#16372=EDGE_LOOP('',(#42499,#42500,#42501,#42502,#42503)) ;
#16373=EDGE_LOOP('',(#42504,#42505,#42506,#42507,#42508,#42509)) ;
#16374=EDGE_LOOP('',(#42510,#42511,#42512,#42513)) ;
#16375=EDGE_LOOP('',(#42514,#42515,#42516,#42517,#42518,#42519,#42520,#42521)) ;
#16376=EDGE_LOOP('',(#42522,#42523,#42524,#42525,#42526,#42527)) ;
#16377=EDGE_LOOP('',(#42528,#42529,#42530,#42531,#42532)) ;
#16378=EDGE_LOOP('',(#42533,#42534,#42535,#42536)) ;
#16379=EDGE_LOOP('',(#42537,#42538,#42539,#42540)) ;
#16380=EDGE_LOOP('',(#42541,#42542,#42543,#42544)) ;
#16381=EDGE_LOOP('',(#42545,#42546,#42547,#42548)) ;
#16382=EDGE_LOOP('',(#42549,#42550,#42551,#42552,#42553,#42554,#42555,#42556,
#42557,#42558,#42559,#42560)) ;
#16383=EDGE_LOOP('',(#42561,#42562,#42563,#42564)) ;
#16384=EDGE_LOOP('',(#42565,#42566,#42567,#42568)) ;
#16385=EDGE_LOOP('',(#42569,#42570,#42571,#42572,#42573,#42574,#42575,#42576)) ;
#16386=EDGE_LOOP('',(#42577,#42578,#42579,#42580,#42581,#42582,#42583,#42584)) ;
#16387=EDGE_LOOP('',(#42585,#42586,#42587,#42588,#42589)) ;
#16388=EDGE_LOOP('',(#42590,#42591,#42592,#42593)) ;
#16389=EDGE_LOOP('',(#42594,#42595,#42596,#42597,#42598,#42599,#42600,#42601,
#42602,#42603)) ;
#16390=EDGE_LOOP('',(#42604,#42605,#42606,#42607)) ;
#18545=CIRCLE('',#52527,0.499999999999998) ;
#18546=CIRCLE('',#52528,0.500000000000009) ;
#18547=CIRCLE('',#52529,0.500000000000009) ;
#18548=CIRCLE('',#52530,0.499999999999998) ;
#18549=CIRCLE('',#52531,0.499999999999998) ;
#18550=CIRCLE('',#52545,6.15) ;
#18551=CIRCLE('',#52546,1.1) ;
#18552=CIRCLE('',#52547,0.500000000000129) ;
#18553=CIRCLE('',#52548,0.700000000000129) ;
#18554=CIRCLE('',#52549,0.9) ;
#18555=CIRCLE('',#52550,4.09999999999997) ;
#18556=CIRCLE('',#52551,1.40000000000004) ;
#18557=CIRCLE('',#52552,3.79999999999997) ;
#18558=CIRCLE('',#52553,3.79999999999982) ;
#18559=CIRCLE('',#52554,1.9) ;
#18560=CIRCLE('',#52558,0.240000000000009) ;
#18561=CIRCLE('',#52559,0.24) ;
#18562=CIRCLE('',#52560,0.48) ;
#18563=CIRCLE('',#52562,0.240000000000009) ;
#18564=CIRCLE('',#52563,0.239999999999991) ;
#18565=CIRCLE('',#52564,0.16) ;
#18566=CIRCLE('',#52565,0.4) ;
#18567=CIRCLE('',#52567,0.239999999999991) ;
#18568=CIRCLE('',#52568,1.53630687649659) ;
#18569=CIRCLE('',#52571,0.4) ;
#18570=CIRCLE('',#52574,0.24) ;
#18571=CIRCLE('',#52577,0.239999999999991) ;
#18572=CIRCLE('',#52578,0.239999999999974) ;
#18573=CIRCLE('',#52579,0.16) ;
#18574=CIRCLE('',#52580,0.4) ;
#18575=CIRCLE('',#52582,0.240000000000009) ;
#18576=CIRCLE('',#52584,0.24) ;
#18577=CIRCLE('',#52585,0.48) ;
#18578=CIRCLE('',#52588,0.4) ;
#18579=CIRCLE('',#52597,0.24) ;
#18580=CIRCLE('',#52603,0.24) ;
#18581=CIRCLE('',#52604,0.239999999999998) ;
#18582=CIRCLE('',#52608,0.299999999999998) ;
#18583=CIRCLE('',#52610,0.45) ;
#18584=CIRCLE('',#52612,0.0999999999999979) ;
#18585=CIRCLE('',#52613,0.240000000000002) ;
#18586=CIRCLE('',#52619,0.24) ;
#18587=CIRCLE('',#52620,0.24) ;
#18588=CIRCLE('',#52624,0.300000000000031) ;
#18589=CIRCLE('',#52625,0.299999999999996) ;
#18590=CIRCLE('',#52626,1.4) ;
#18591=CIRCLE('',#52630,0.0999999999999446) ;
#18592=CIRCLE('',#52633,0.100000000000002) ;
#18593=CIRCLE('',#52635,0.24) ;
#18594=CIRCLE('',#52637,0.24) ;
#18595=CIRCLE('',#52643,0.1) ;
#18596=CIRCLE('',#52645,0.0999999999999979) ;
#18597=CIRCLE('',#52649,0.199999999999984) ;
#18598=CIRCLE('',#52651,0.200000000000005) ;
#18599=CIRCLE('',#52657,0.199999999999996) ;
#18600=CIRCLE('',#52660,0.0999999999999934) ;
#18601=CIRCLE('',#52661,0.24) ;
#18602=CIRCLE('',#52662,0.0999999999999894) ;
#18603=CIRCLE('',#52663,0.14) ;
#18604=CIRCLE('',#52666,0.0999999999999979) ;
#18605=CIRCLE('',#52670,0.1) ;
#18606=CIRCLE('',#52671,0.14) ;
#18607=CIRCLE('',#52672,0.0999999999999979) ;
#18608=CIRCLE('',#52673,0.24) ;
#18609=CIRCLE('',#52676,0.1) ;
#18610=CIRCLE('',#52678,0.2) ;
#18611=CIRCLE('',#52679,0.099999999999838) ;
#18612=CIRCLE('',#52680,0.3) ;
#18613=CIRCLE('',#52682,0.299999999999998) ;
#18614=CIRCLE('',#52683,0.75) ;
#18615=CIRCLE('',#52686,0.3) ;
#18616=CIRCLE('',#52687,0.1) ;
#18617=CIRCLE('',#52688,0.2) ;
#18618=CIRCLE('',#52690,0.300000000000002) ;
#18619=CIRCLE('',#52692,0.300000000000011) ;
#18620=CIRCLE('',#52693,0.75) ;
#18621=CIRCLE('',#52694,0.45) ;
#18622=CIRCLE('',#52698,0.0999999999999801) ;
#18623=CIRCLE('',#52701,0.800000000000003) ;
#18624=CIRCLE('',#52704,0.100000000000016) ;
#18625=CIRCLE('',#52705,0.0999999999999979) ;
#18626=CIRCLE('',#52706,0.0999999999999979) ;
#18627=CIRCLE('',#52710,3.99999999999997) ;
#18628=CIRCLE('',#52711,0.0999999999999801) ;
#18629=CIRCLE('',#52712,4.09999999999997) ;
#18630=CIRCLE('',#52714,0.100000000000016) ;
#18631=CIRCLE('',#52716,0.0999999999999977) ;
#18632=CIRCLE('',#52717,0.9) ;
#18633=CIRCLE('',#52718,1.) ;
#18634=CIRCLE('',#52720,0.0999999999999973) ;
#18635=CIRCLE('',#52721,0.700000000000129) ;
#18636=CIRCLE('',#52722,0.600000000000129) ;
#18637=CIRCLE('',#52724,0.0999999999999847) ;
#18638=CIRCLE('',#52726,0.0999999999999979) ;
#18639=CIRCLE('',#52727,0.500000000000129) ;
#18640=CIRCLE('',#52728,0.600000000000129) ;
#18641=CIRCLE('',#52731,0.0999999999999979) ;
#18642=CIRCLE('',#52733,0.2) ;
#18643=CIRCLE('',#52734,0.1) ;
#18644=CIRCLE('',#52736,0.100000000000051) ;
#18645=CIRCLE('',#52737,0.0999999999999979) ;
#18646=CIRCLE('',#52738,4.49999999999997) ;
#18647=CIRCLE('',#52739,2.9) ;
#18648=CIRCLE('',#52740,0.1) ;
#18649=CIRCLE('',#52742,0.1) ;
#18650=CIRCLE('',#52745,0.1) ;
#18651=CIRCLE('',#52746,0.100000000000013) ;
#18652=CIRCLE('',#52749,1.50000000000013) ;
#18653=CIRCLE('',#52750,1.50000000000013) ;
#18654=CIRCLE('',#52752,0.0999999999999979) ;
#18655=CIRCLE('',#52755,0.200000000000002) ;
#18656=CIRCLE('',#52756,0.100000000000002) ;
#18657=CIRCLE('',#52757,0.1) ;
#18658=CIRCLE('',#52758,0.100000000000096) ;
#18659=CIRCLE('',#52760,0.0999999999999801) ;
#18660=CIRCLE('',#52762,0.700000000000003) ;
#18661=CIRCLE('',#52764,0.1) ;
#18662=CIRCLE('',#52765,0.0999999999999957) ;
#18663=CIRCLE('',#52766,0.100000000000004) ;
#18664=CIRCLE('',#52770,0.0999999999999941) ;
#18665=CIRCLE('',#52775,3.89999999999997) ;
#18666=CIRCLE('',#52776,0.100000000000022) ;
#18667=CIRCLE('',#52778,0.0999999999999856) ;
#18668=CIRCLE('',#52780,0.099999999999989) ;
#18669=CIRCLE('',#52781,3.89999999999982) ;
#18670=CIRCLE('',#52783,0.0999999999999979) ;
#18671=CIRCLE('',#52785,0.10000000000006) ;
#18672=CIRCLE('',#52786,0.75) ;
#18673=CIRCLE('',#52787,0.65) ;
#18674=CIRCLE('',#52789,0.0999999999999979) ;
#18675=CIRCLE('',#52791,0.75) ;
#18676=CIRCLE('',#52792,0.65) ;
#18677=CIRCLE('',#52794,0.700000000000003) ;
#18678=CIRCLE('',#52797,3.89999999999982) ;
#18679=CIRCLE('',#52800,3.89999999999997) ;
#18680=CIRCLE('',#52802,0.100000000000027) ;
#18681=CIRCLE('',#52803,0.0999999999999976) ;
#18682=CIRCLE('',#52804,0.0999999999999801) ;
#18683=CIRCLE('',#52808,0.100000000000016) ;
#18684=CIRCLE('',#52809,0.100000000000014) ;
#18685=CIRCLE('',#52812,0.100000000000001) ;
#18686=CIRCLE('',#52823,0.100000000000016) ;
#18687=CIRCLE('',#52827,2.) ;
#18688=CIRCLE('',#52832,2.) ;
#18689=CIRCLE('',#52835,0.0999999999999801) ;
#18690=CIRCLE('',#52839,0.0999999999999973) ;
#18691=CIRCLE('',#52840,0.2) ;
#18692=CIRCLE('',#52841,0.1) ;
#18693=CIRCLE('',#52845,0.1) ;
#18694=CIRCLE('',#52847,0.0999999999999979) ;
#18695=CIRCLE('',#52849,0.0999999999999847) ;
#18696=CIRCLE('',#52850,0.0999999999999979) ;
#18697=CIRCLE('',#52851,0.0999999999999979) ;
#18698=CIRCLE('',#52855,0.0999999999999979) ;
#18699=CIRCLE('',#52856,0.0999999999999979) ;
#18700=CIRCLE('',#52857,0.199999999999978) ;
#18701=CIRCLE('',#52858,0.0999999999999847) ;
#18702=CIRCLE('',#52863,1.) ;
#18703=CIRCLE('',#52864,4.06491106406736) ;
#18704=CIRCLE('',#52865,4.05) ;
#18705=CIRCLE('',#52866,0.200000000000031) ;
#18706=CIRCLE('',#52867,0.199999999999996) ;
#18707=CIRCLE('',#52868,0.199999999999996) ;
#18708=CIRCLE('',#52869,0.200000000000001) ;
#18709=CIRCLE('',#52870,4.05) ;
#18710=CIRCLE('',#52871,4.06491106406736) ;
#18711=CIRCLE('',#52872,1.) ;
#18712=CIRCLE('',#52873,1.) ;
#18713=CIRCLE('',#52874,4.06491106406736) ;
#18714=CIRCLE('',#52875,4.05) ;
#18715=CIRCLE('',#52876,4.06491106406736) ;
#18716=CIRCLE('',#52877,1.) ;
#18717=CIRCLE('',#52878,1.60000000000004) ;
#18718=CIRCLE('',#52879,2.99999999999998) ;
#18719=CIRCLE('',#52880,3.6) ;
#18720=CIRCLE('',#52881,3.6) ;
#18721=CIRCLE('',#52882,4.09999999999997) ;
#18722=CIRCLE('',#52883,3.) ;
#18723=CIRCLE('',#52884,4.49999999999997) ;
#18724=CIRCLE('',#52885,0.199999999999996) ;
#18725=CIRCLE('',#52886,0.199999999999996) ;
#18726=CIRCLE('',#52887,0.199999999999996) ;
#18727=CIRCLE('',#52888,0.199999999999996) ;
#18728=CIRCLE('',#52889,0.200000000000031) ;
#18729=CIRCLE('',#52890,4.49999999999997) ;
#18730=CIRCLE('',#52891,0.100000000000016) ;
#18731=CIRCLE('',#52892,0.100000000000004) ;
#18732=CIRCLE('',#52893,0.0999999999999979) ;
#18733=CIRCLE('',#52894,0.0999999999999973) ;
#18734=CIRCLE('',#52895,1.1) ;
#18735=CIRCLE('',#52896,0.100000000000106) ;
#18736=CIRCLE('',#52897,0.3999999999999) ;
#18737=CIRCLE('',#52898,0.400000000000114) ;
#18738=CIRCLE('',#52899,0.100000000000016) ;
#18739=CIRCLE('',#52900,0.500000000000025) ;
#18740=CIRCLE('',#52901,0.199999999999996) ;
#18741=CIRCLE('',#52902,0.200000000000031) ;
#18742=CIRCLE('',#52903,0.2) ;
#18743=CIRCLE('',#52904,0.200000000000031) ;
#18744=CIRCLE('',#52905,2.6) ;
#18745=CIRCLE('',#52906,0.199999999999996) ;
#18746=CIRCLE('',#52907,0.199999999999996) ;
#18747=CIRCLE('',#52908,0.199999999999996) ;
#18748=CIRCLE('',#52909,0.199999999999996) ;
#18749=CIRCLE('',#52910,0.199999999999996) ;
#18750=CIRCLE('',#52911,0.199999999999996) ;
#18751=CIRCLE('',#52912,2.49999999999999) ;
#18752=CIRCLE('',#52913,0.199999999999996) ;
#18753=CIRCLE('',#52914,0.199999999999995) ;
#18754=CIRCLE('',#52915,0.199999999999996) ;
#18755=CIRCLE('',#52916,0.199999999999995) ;
#18756=CIRCLE('',#52917,0.199999999999996) ;
#18757=CIRCLE('',#52918,0.199999999999996) ;
#18758=CIRCLE('',#52919,0.200000000000031) ;
#18759=CIRCLE('',#52920,0.199999999999996) ;
#18760=CIRCLE('',#52921,0.199999999999996) ;
#18761=CIRCLE('',#52922,0.199999999999996) ;
#18762=CIRCLE('',#52923,0.199999999999996) ;
#18763=CIRCLE('',#52924,0.199999999999996) ;
#18764=CIRCLE('',#52925,0.199999999999996) ;
#18765=CIRCLE('',#52926,0.199999999999996) ;
#18766=CIRCLE('',#52928,0.10000000000001) ;
#18767=CIRCLE('',#52929,0.0999999999999845) ;
#18768=CIRCLE('',#52932,2.9) ;
#18769=CIRCLE('',#52934,0.0999999999999979) ;
#18770=CIRCLE('',#52935,3.99999999999997) ;
#18771=CIRCLE('',#52937,0.1) ;
#18772=CIRCLE('',#52940,3.99999999999997) ;
#18773=CIRCLE('',#52944,0.0999999999999801) ;
#18774=CIRCLE('',#52945,0.0999999999999979) ;
#18775=CIRCLE('',#52946,0.0999999999999848) ;
#18776=CIRCLE('',#52948,0.0999999999999979) ;
#18777=CIRCLE('',#52950,0.0999999999999979) ;
#18778=CIRCLE('',#52951,0.599999999999915) ;
#18779=CIRCLE('',#52952,0.699999999999915) ;
#18780=CIRCLE('',#52954,0.0999999999999979) ;
#18781=CIRCLE('',#52956,0.0999999999999979) ;
#18782=CIRCLE('',#52957,1.) ;
#18783=CIRCLE('',#52958,0.9) ;
#18784=CIRCLE('',#52961,0.100000000000016) ;
#18785=CIRCLE('',#52963,0.0999999999999984) ;
#18786=CIRCLE('',#52964,0.600000000000114) ;
#18787=CIRCLE('',#52965,0.500000000000114) ;
#18788=CIRCLE('',#52968,0.0999999999999979) ;
#18789=CIRCLE('',#52970,0.0999999999999984) ;
#18790=CIRCLE('',#52972,0.999999999999996) ;
#18791=CIRCLE('',#52973,0.100000000000022) ;
#18792=CIRCLE('',#52974,0.100000000000008) ;
#18793=CIRCLE('',#52975,0.200000000000106) ;
#18794=CIRCLE('',#52977,0.0999999999999848) ;
#18795=CIRCLE('',#52979,0.0999999999999979) ;
#18796=CIRCLE('',#52980,0.499999999999901) ;
#18797=CIRCLE('',#52984,0.100000000000162) ;
#18798=CIRCLE('',#52986,0.0999999999999801) ;
#18799=CIRCLE('',#52987,0.500000000000114) ;
#18800=CIRCLE('',#52989,0.0999999999999801) ;
#18801=CIRCLE('',#52991,0.500000000000025) ;
#18802=CIRCLE('',#52995,0.599999999999915) ;
#18803=CIRCLE('',#52998,1.) ;
#18804=CIRCLE('',#53000,0.85) ;
#18805=CIRCLE('',#53001,0.65) ;
#18806=CIRCLE('',#53002,0.6) ;
#18807=CIRCLE('',#53009,0.999999999999996) ;
#18808=CIRCLE('',#53011,0.0999999999999979) ;
#18809=CIRCLE('',#53012,0.0999999999999915) ;
#18810=CIRCLE('',#53014,0.1) ;
#18811=CIRCLE('',#53016,0.0999999999999979) ;
#18812=CIRCLE('',#53017,0.0999999999999979) ;
#18813=CIRCLE('',#53018,0.199999999999996) ;
#18814=CIRCLE('',#53019,0.100000000000016) ;
#18815=CIRCLE('',#53021,0.0999999999999979) ;
#18816=CIRCLE('',#53023,0.6) ;
#18817=CIRCLE('',#53024,0.5) ;
#18818=CIRCLE('',#53026,0.200000000000031) ;
#18819=CIRCLE('',#53027,0.0999999999999979) ;
#18820=CIRCLE('',#53028,0.100000000000016) ;
#18821=CIRCLE('',#53029,0.0999999999999979) ;
#18822=CIRCLE('',#53030,0.100000000000005) ;
#18823=CIRCLE('',#53031,0.100000000000016) ;
#18824=CIRCLE('',#53033,0.0999999999999979) ;
#18825=CIRCLE('',#53034,0.5) ;
#18826=CIRCLE('',#53035,0.6) ;
#18827=CIRCLE('',#53038,0.0999999999999915) ;
#18828=CIRCLE('',#53039,0.0999999999999926) ;
#18829=CIRCLE('',#53040,0.0999999999999879) ;
#18830=CIRCLE('',#53044,0.1) ;
#18831=CIRCLE('',#53046,0.1) ;
#18832=CIRCLE('',#53047,0.199999999999996) ;
#18833=CIRCLE('',#53049,0.1) ;
#18834=CIRCLE('',#53051,0.1) ;
#18835=CIRCLE('',#53052,0.200000000000031) ;
#18836=CIRCLE('',#53055,0.1) ;
#18837=CIRCLE('',#53057,0.100000000000016) ;
#18838=CIRCLE('',#53059,0.100000000000007) ;
#18839=CIRCLE('',#53060,0.3) ;
#18840=CIRCLE('',#53061,0.4) ;
#18841=CIRCLE('',#53063,0.0999999999999623) ;
#18842=CIRCLE('',#53065,0.100000000000016) ;
#18843=CIRCLE('',#53066,0.300000000000031) ;
#18844=CIRCLE('',#53067,0.200000000000031) ;
#18845=CIRCLE('',#53069,0.100000000000016) ;
#18846=CIRCLE('',#53071,0.100000000000002) ;
#18847=CIRCLE('',#53072,0.3) ;
#18848=CIRCLE('',#53073,0.2) ;
#18849=CIRCLE('',#53075,0.0999999999999979) ;
#18850=CIRCLE('',#53077,0.0999999999999801) ;
#18851=CIRCLE('',#53078,0.3) ;
#18852=CIRCLE('',#53079,0.4) ;
#18853=CIRCLE('',#53082,0.100000000000016) ;
#18854=CIRCLE('',#53083,0.100000000000009) ;
#18855=CIRCLE('',#53086,0.1) ;
#18856=CIRCLE('',#53088,0.5) ;
#18857=CIRCLE('',#53091,0.4) ;
#18858=CIRCLE('',#53096,0.4) ;
#18859=CIRCLE('',#53102,0.4) ;
#18860=CIRCLE('',#53104,0.1) ;
#18861=CIRCLE('',#53105,0.1) ;
#18862=CIRCLE('',#53108,0.1) ;
#18863=CIRCLE('',#53109,0.1) ;
#18864=CIRCLE('',#53111,0.199999999999996) ;
#18865=CIRCLE('',#53112,0.100000000000016) ;
#18866=CIRCLE('',#53113,0.0999999999999979) ;
#18867=CIRCLE('',#53114,0.0999999999999979) ;
#18868=CIRCLE('',#53116,0.100000000000051) ;
#18869=CIRCLE('',#53117,0.0999999999999979) ;
#18870=CIRCLE('',#53118,0.200000000000067) ;
#18871=CIRCLE('',#53119,0.0999999999999979) ;
#18872=CIRCLE('',#53122,0.0999999999999979) ;
#18873=CIRCLE('',#53123,0.1) ;
#18874=CIRCLE('',#53125,0.0999999999999979) ;
#18875=CIRCLE('',#53126,0.500000000000007) ;
#18876=CIRCLE('',#53127,0.400000000000007) ;
#18877=CIRCLE('',#53130,0.1) ;
#18878=CIRCLE('',#53132,0.1) ;
#18879=CIRCLE('',#53134,0.0999999999999979) ;
#18880=CIRCLE('',#53136,0.0999999999999979) ;
#18881=CIRCLE('',#53137,0.500000000000007) ;
#18882=CIRCLE('',#53138,0.400000000000007) ;
#18883=CIRCLE('',#53140,0.1) ;
#18884=CIRCLE('',#53142,0.500000000000007) ;
#18885=CIRCLE('',#53144,0.3) ;
#18886=CIRCLE('',#53145,0.4) ;
#18887=CIRCLE('',#53146,0.6) ;
#18888=CIRCLE('',#53147,0.65) ;
#18889=CIRCLE('',#53149,0.500000000000007) ;
#18890=CIRCLE('',#53152,0.0999999999999979) ;
#18891=CIRCLE('',#53154,0.0999999999999979) ;
#18892=CIRCLE('',#53158,0.10000000000001) ;
#18893=CIRCLE('',#53159,0.699999999999915) ;
#18894=CIRCLE('',#53161,0.0999999999999847) ;
#18895=CIRCLE('',#53163,0.0999999999999979) ;
#18896=CIRCLE('',#53164,0.9) ;
#18897=CIRCLE('',#53166,0.0999999999999979) ;
#18898=CIRCLE('',#53168,0.0999999999999801) ;
#18899=CIRCLE('',#53169,0.5) ;
#18900=CIRCLE('',#53171,0.0999999999999979) ;
#18901=CIRCLE('',#53173,0.0999999999999446) ;
#18902=CIRCLE('',#53174,0.75) ;
#18903=CIRCLE('',#53176,0.0999999999999979) ;
#18904=CIRCLE('',#53178,0.0999999999999091) ;
#18905=CIRCLE('',#53179,0.75) ;
#18906=CIRCLE('',#53181,0.0999999999999979) ;
#18907=CIRCLE('',#53182,0.0999999999999984) ;
#18908=CIRCLE('',#53185,0.0999999999999984) ;
#18909=CIRCLE('',#53186,0.100000000000022) ;
#18910=CIRCLE('',#53188,0.0999999999999918) ;
#18911=CIRCLE('',#53190,0.100000000000001) ;
#18912=CIRCLE('',#53192,0.0999999999999979) ;
#18913=CIRCLE('',#53194,0.0999999999999801) ;
#18914=CIRCLE('',#53196,0.0999999999999973) ;
#18915=CIRCLE('',#53197,0.600000000000129) ;
#18916=CIRCLE('',#53199,0.0999999999999973) ;
#18917=CIRCLE('',#53201,0.10000000000002) ;
#18918=CIRCLE('',#53202,0.600000000000129) ;
#18919=CIRCLE('',#53204,0.0999999999999801) ;
#18920=CIRCLE('',#53205,1.) ;
#18921=CIRCLE('',#53207,0.100000000000016) ;
#18922=CIRCLE('',#53209,0.0999999999999979) ;
#18923=CIRCLE('',#53211,0.0999999999999979) ;
#18924=CIRCLE('',#53213,1.50000000000004) ;
#18925=CIRCLE('',#53216,1.50000000000004) ;
#18926=CIRCLE('',#53223,0.100000000000264) ;
#18927=CIRCLE('',#53227,0.0999999999999979) ;
#18928=CIRCLE('',#53229,0.0999999999999934) ;
#18929=CIRCLE('',#53230,1.5) ;
#18930=CIRCLE('',#53233,0.0999999999999979) ;
#18931=CIRCLE('',#53234,0.400000000000007) ;
#18932=CIRCLE('',#53236,0.0999999999999979) ;
#18933=CIRCLE('',#53238,0.100000000000002) ;
#18934=CIRCLE('',#53239,0.75) ;
#18935=CIRCLE('',#53241,0.0999999999999979) ;
#18936=CIRCLE('',#53243,0.100000000000007) ;
#18937=CIRCLE('',#53245,0.0999999999999934) ;
#18938=CIRCLE('',#53247,0.100000000000016) ;
#18939=CIRCLE('',#53248,0.5) ;
#18940=CIRCLE('',#53252,0.1) ;
#18941=CIRCLE('',#53253,0.0999999999999979) ;
#18942=CIRCLE('',#53255,0.0999999999999979) ;
#18943=CIRCLE('',#53256,0.500000000000043) ;
#18944=CIRCLE('',#53257,0.400000000000043) ;
#18945=CIRCLE('',#53259,0.0999999999999979) ;
#18946=CIRCLE('',#53261,0.0999999999999979) ;
#18947=CIRCLE('',#53262,0.400000000000007) ;
#18948=CIRCLE('',#53264,0.0999999999999979) ;
#18949=CIRCLE('',#53266,0.0999999999999801) ;
#18950=CIRCLE('',#53267,0.4) ;
#18951=CIRCLE('',#53273,0.5) ;
#18952=CIRCLE('',#53274,4.56491106406736) ;
#18953=CIRCLE('',#53275,4.55) ;
#18954=CIRCLE('',#53277,0.500000000000009) ;
#18955=CIRCLE('',#53282,2.) ;
#18956=CIRCLE('',#53284,0.4) ;
#18957=CIRCLE('',#53288,0.100000000000016) ;
#18958=CIRCLE('',#53290,0.100000000000003) ;
#18959=CIRCLE('',#53292,0.0999999999999979) ;
#18960=CIRCLE('',#53294,0.100000000000007) ;
#18961=CIRCLE('',#53296,0.0999999999999981) ;
#18962=CIRCLE('',#53297,0.0999999999999979) ;
#18963=CIRCLE('',#53299,0.099999999999989) ;
#18964=CIRCLE('',#53300,0.75) ;
#18965=CIRCLE('',#53301,0.65) ;
#18966=CIRCLE('',#53304,0.1) ;
#18967=CIRCLE('',#53307,0.1) ;
#18968=CIRCLE('',#53309,0.0999999999999979) ;
#18969=CIRCLE('',#53310,0.100000000000003) ;
#18970=CIRCLE('',#53313,0.4) ;
#18971=CIRCLE('',#53319,0.515810020027939) ;
#18972=CIRCLE('',#53330,0.200000000000009) ;
#18973=CIRCLE('',#53332,0.200000000000046) ;
#18974=CIRCLE('',#53333,0.200000000000015) ;
#18975=CIRCLE('',#53335,0.199999999999996) ;
#18976=CIRCLE('',#53336,0.19999999999999) ;
#18977=CIRCLE('',#53342,0.199999999999979) ;
#18978=CIRCLE('',#53345,0.200000000000007) ;
#18979=CIRCLE('',#53346,0.199999999999997) ;
#18980=CIRCLE('',#53351,6.15) ;
#18981=CIRCLE('',#53352,6.15) ;
#18982=CIRCLE('',#53353,0.799999999999972) ;
#18983=CIRCLE('',#53354,0.199999999999963) ;
#18984=CIRCLE('',#53355,0.199999999999963) ;
#18985=CIRCLE('',#53356,0.799999999999972) ;
#18986=CIRCLE('',#53362,0.2) ;
#18987=CIRCLE('',#53364,0.199999999999978) ;
#18988=CIRCLE('',#53369,0.200000000000008) ;
#18989=CIRCLE('',#53370,0.2) ;
#18990=CIRCLE('',#53378,6.15) ;
#18991=CIRCLE('',#53386,3.6) ;
#18992=CIRCLE('',#53389,3.6) ;
#18993=CIRCLE('',#53390,3.6) ;
#18994=CIRCLE('',#53392,3.6) ;
#18995=CIRCLE('',#53397,3.79999999999997) ;
#18996=CIRCLE('',#53398,1.40000000000004) ;
#18997=CIRCLE('',#53400,0.0999999999999979) ;
#18998=CIRCLE('',#53403,0.0999999999999928) ;
#18999=CIRCLE('',#53505,0.1) ;
#19000=CIRCLE('',#53507,0.1) ;
#19001=CIRCLE('',#53508,0.699999999999972) ;
#19002=CIRCLE('',#53509,0.599999999999972) ;
#19003=CIRCLE('',#53515,0.1) ;
#19004=CIRCLE('',#53517,0.1) ;
#19005=CIRCLE('',#53518,0.299999999999963) ;
#19006=CIRCLE('',#53519,0.399999999999963) ;
#19007=CIRCLE('',#53527,0.299999999999963) ;
#19008=CIRCLE('',#53537,0.1) ;
#19009=CIRCLE('',#53539,0.1) ;
#19010=CIRCLE('',#53540,0.699999999999972) ;
#19011=CIRCLE('',#53541,0.599999999999972) ;
#19012=CIRCLE('',#53547,0.1) ;
#19013=CIRCLE('',#53549,0.1) ;
#19014=CIRCLE('',#53550,0.299999999999963) ;
#19015=CIRCLE('',#53551,0.399999999999963) ;
#19016=CIRCLE('',#53560,0.299999999999963) ;
#19017=CIRCLE('',#53604,4.56491106406736) ;
#19018=CIRCLE('',#53605,4.55) ;
#19019=CIRCLE('',#53606,4.55) ;
#19020=CIRCLE('',#53607,4.56491106406736) ;
#19021=CIRCLE('',#53608,0.5) ;
#19022=CIRCLE('',#53643,0.0999999999999801) ;
#19023=CIRCLE('',#53654,0.100000000000005) ;
#19024=CIRCLE('',#53655,0.1) ;
#19025=CIRCLE('',#53657,0.0999999999999979) ;
#19026=CIRCLE('',#53660,0.0999999999999745) ;
#19027=CIRCLE('',#53661,0.699999999999972) ;
#19028=CIRCLE('',#53663,0.1) ;
#19029=CIRCLE('',#53672,0.099999999999989) ;
#19030=CIRCLE('',#53683,0.0999999999999745) ;
#19031=CIRCLE('',#53684,0.699999999999972) ;
#19032=CIRCLE('',#53687,0.100000000000005) ;
#19033=CIRCLE('',#53689,0.100000000000007) ;
#19034=CIRCLE('',#53704,4.55) ;
#19035=CIRCLE('',#53705,4.56491106406736) ;
#19036=CIRCLE('',#53708,2.99999999999998) ;
#19037=CIRCLE('',#53711,1.60000000000004) ;
#19038=CIRCLE('',#53716,0.500000000000043) ;
#19039=CIRCLE('',#53718,0.500000000000043) ;
#19040=CIRCLE('',#53729,1.5) ;
#19041=CIRCLE('',#53734,0.399999999999992) ;
#19042=CIRCLE('',#53741,0.4) ;
#19043=CIRCLE('',#53752,0.499999999999998) ;
#19044=CIRCLE('',#53753,0.500000000000009) ;
#19045=CIRCLE('',#53754,0.499999999999997) ;
#19046=CIRCLE('',#53756,4.06491106406736) ;
#19047=CIRCLE('',#53757,0.499999999999998) ;
#19048=CIRCLE('',#53759,0.499999999999998) ;
#19049=CIRCLE('',#53760,0.499999999999998) ;
#19050=CIRCLE('',#53762,0.499999999999998) ;
#19051=CIRCLE('',#53763,4.05) ;
#19052=CIRCLE('',#53767,0.499999999999998) ;
#19053=CIRCLE('',#53768,0.499999999999992) ;
#19054=CIRCLE('',#53769,0.500000000000009) ;
#19055=CIRCLE('',#53773,4.06491106406736) ;
#19056=CIRCLE('',#53774,0.499999999999998) ;
#19057=CIRCLE('',#53775,0.500000000000018) ;
#19058=CIRCLE('',#53776,0.500000000000019) ;
#19059=CIRCLE('',#53778,0.499999999999998) ;
#19060=CIRCLE('',#53780,4.05) ;
#19061=CIRCLE('',#53782,0.499999999999998) ;
#19062=CIRCLE('',#53783,0.499999999999998) ;
#19063=CIRCLE('',#53785,0.499999999999998) ;
#19064=CIRCLE('',#53786,4.05) ;
#19065=CIRCLE('',#53788,0.50000000000001) ;
#19066=CIRCLE('',#53789,0.500000000000019) ;
#19067=CIRCLE('',#53791,0.499999999999998) ;
#19068=CIRCLE('',#53793,4.05) ;
#19069=CIRCLE('',#53796,0.499999999999998) ;
#19070=CIRCLE('',#53797,0.499999999999989) ;
#19071=CIRCLE('',#53799,4.06491106406736) ;
#19072=CIRCLE('',#53800,1.) ;
#19073=CIRCLE('',#53803,0.499999999999998) ;
#19074=CIRCLE('',#53804,0.499999999999998) ;
#19075=CIRCLE('',#53806,4.06491106406736) ;
#19076=CIRCLE('',#53809,0.500000000000012) ;
#19077=CIRCLE('',#53812,1.) ;
#19078=CIRCLE('',#53813,0.500000000000009) ;
#19079=CIRCLE('',#53819,0.500000000000009) ;
#19080=CIRCLE('',#53820,0.500000000000009) ;
#19081=CIRCLE('',#53831,0.500000000000043) ;
#19082=CIRCLE('',#53836,0.200000000000031) ;
#19083=CIRCLE('',#53840,0.199999999999996) ;
#19084=CIRCLE('',#53843,0.199999999999996) ;
#19085=CIRCLE('',#53849,2.) ;
#19086=CIRCLE('',#53852,2.6) ;
#19087=CIRCLE('',#53855,0.200000000000001) ;
#19088=CIRCLE('',#53858,0.199999999999996) ;
#19089=CIRCLE('',#53861,0.199999999999996) ;
#19090=CIRCLE('',#53864,0.199999999999996) ;
#19091=CIRCLE('',#53868,0.199999999999996) ;
#19092=CIRCLE('',#53871,2.49999999999999) ;
#19093=CIRCLE('',#53874,0.199999999999995) ;
#19094=CIRCLE('',#53877,0.199999999999996) ;
#19095=CIRCLE('',#53880,0.199999999999996) ;
#19096=CIRCLE('',#53883,0.199999999999996) ;
#19097=CIRCLE('',#53888,0.100000000000016) ;
#19098=CIRCLE('',#53891,0.0999999999999979) ;
#19099=CIRCLE('',#53894,0.100000000000051) ;
#19100=CIRCLE('',#53896,0.199999999999996) ;
#19101=CIRCLE('',#53899,0.199999999999996) ;
#19102=CIRCLE('',#53903,0.199999999999996) ;
#19103=CIRCLE('',#53906,0.199999999999996) ;
#19104=CIRCLE('',#53910,0.199999999999996) ;
#19105=CIRCLE('',#53913,0.199999999999996) ;
#19106=CIRCLE('',#53919,0.199999999999995) ;
#19107=CIRCLE('',#53922,0.199999999999996) ;
#19108=CIRCLE('',#53927,0.199999999999996) ;
#19109=CIRCLE('',#53930,0.200000000000031) ;
#19110=CIRCLE('',#53934,0.199999999999996) ;
#19111=CIRCLE('',#53941,0.200000000000031) ;
#19112=CIRCLE('',#53943,4.05) ;
#19113=CIRCLE('',#53945,0.199999999999996) ;
#19114=CIRCLE('',#53949,0.199999999999996) ;
#19115=CIRCLE('',#53952,0.199999999999996) ;
#19116=CIRCLE('',#53956,0.0999999999999973) ;
#19117=CIRCLE('',#53959,0.0999999999999979) ;
#19118=CIRCLE('',#53962,0.100000000000004) ;
#19119=CIRCLE('',#53967,0.199999999999996) ;
#19120=CIRCLE('',#53982,4.49999999999997) ;
#19121=CIRCLE('',#53983,0.199999999999996) ;
#21716=VERTEX_POINT('',#89078) ;
#21717=VERTEX_POINT('',#89079) ;
#21718=VERTEX_POINT('',#89093) ;
#21719=VERTEX_POINT('',#89100) ;
#21720=VERTEX_POINT('',#89244) ;
#21721=VERTEX_POINT('',#89258) ;
#21722=VERTEX_POINT('',#89405) ;
#21723=VERTEX_POINT('',#89412) ;
#21724=VERTEX_POINT('',#89456) ;
#21725=VERTEX_POINT('',#89624) ;
#21726=VERTEX_POINT('',#89636) ;
#21727=VERTEX_POINT('',#89804) ;
#21728=VERTEX_POINT('',#89811) ;
#21729=VERTEX_POINT('',#89875) ;
#21730=VERTEX_POINT('',#89876) ;
#21731=VERTEX_POINT('',#89878) ;
#21732=VERTEX_POINT('',#89880) ;
#21733=VERTEX_POINT('',#89893) ;
#21734=VERTEX_POINT('',#89899) ;
#21735=VERTEX_POINT('',#89916) ;
#21736=VERTEX_POINT('',#89922) ;
#21737=VERTEX_POINT('',#89939) ;
#21738=VERTEX_POINT('',#89945) ;
#21739=VERTEX_POINT('',#89962) ;
#21740=VERTEX_POINT('',#89968) ;
#21741=VERTEX_POINT('',#89985) ;
#21742=VERTEX_POINT('',#89991) ;
#21743=VERTEX_POINT('',#89999) ;
#21744=VERTEX_POINT('',#90001) ;
#21745=VERTEX_POINT('',#90008) ;
#21746=VERTEX_POINT('',#90009) ;
#21747=VERTEX_POINT('',#90011) ;
#21748=VERTEX_POINT('',#90013) ;
#21749=VERTEX_POINT('',#90017) ;
#21750=VERTEX_POINT('',#90019) ;
#21751=VERTEX_POINT('',#90032) ;
#21752=VERTEX_POINT('',#90038) ;
#21753=VERTEX_POINT('',#90055) ;
#21754=VERTEX_POINT('',#90061) ;
#21755=VERTEX_POINT('',#90078) ;
#21756=VERTEX_POINT('',#90084) ;
#21757=VERTEX_POINT('',#90101) ;
#21758=VERTEX_POINT('',#90107) ;
#21759=VERTEX_POINT('',#90115) ;
#21760=VERTEX_POINT('',#90117) ;
#21761=VERTEX_POINT('',#90121) ;
#21762=VERTEX_POINT('',#90123) ;
#21763=VERTEX_POINT('',#90127) ;
#21764=VERTEX_POINT('',#90129) ;
#21765=VERTEX_POINT('',#90142) ;
#21766=VERTEX_POINT('',#90148) ;
#21767=VERTEX_POINT('',#90165) ;
#21768=VERTEX_POINT('',#90171) ;
#21769=VERTEX_POINT('',#90188) ;
#21770=VERTEX_POINT('',#90194) ;
#21771=VERTEX_POINT('',#90211) ;
#21772=VERTEX_POINT('',#90217) ;
#21773=VERTEX_POINT('',#90234) ;
#21774=VERTEX_POINT('',#90240) ;
#21775=VERTEX_POINT('',#90257) ;
#21776=VERTEX_POINT('',#90263) ;
#21777=VERTEX_POINT('',#90280) ;
#21778=VERTEX_POINT('',#90286) ;
#21779=VERTEX_POINT('',#90294) ;
#21780=VERTEX_POINT('',#90296) ;
#21781=VERTEX_POINT('',#90300) ;
#21782=VERTEX_POINT('',#90302) ;
#21783=VERTEX_POINT('',#90310) ;
#21784=VERTEX_POINT('',#90311) ;
#21785=VERTEX_POINT('',#90313) ;
#21786=VERTEX_POINT('',#90315) ;
#21787=VERTEX_POINT('',#90317) ;
#21788=VERTEX_POINT('',#90319) ;
#21789=VERTEX_POINT('',#90321) ;
#21790=VERTEX_POINT('',#90323) ;
#21791=VERTEX_POINT('',#90325) ;
#21792=VERTEX_POINT('',#90327) ;
#21793=VERTEX_POINT('',#90329) ;
#21794=VERTEX_POINT('',#90331) ;
#21795=VERTEX_POINT('',#90333) ;
#21796=VERTEX_POINT('',#90335) ;
#21797=VERTEX_POINT('',#90337) ;
#21798=VERTEX_POINT('',#90339) ;
#21799=VERTEX_POINT('',#90341) ;
#21800=VERTEX_POINT('',#90343) ;
#21801=VERTEX_POINT('',#90346) ;
#21802=VERTEX_POINT('',#90347) ;
#21803=VERTEX_POINT('',#90349) ;
#21804=VERTEX_POINT('',#90351) ;
#21805=VERTEX_POINT('',#90362) ;
#21806=VERTEX_POINT('',#90363) ;
#21807=VERTEX_POINT('',#90365) ;
#21808=VERTEX_POINT('',#90367) ;
#21809=VERTEX_POINT('',#90382) ;
#21810=VERTEX_POINT('',#90389) ;
#21811=VERTEX_POINT('',#90398) ;
#21812=VERTEX_POINT('',#90399) ;
#21813=VERTEX_POINT('',#90401) ;
#21814=VERTEX_POINT('',#90403) ;
#21815=VERTEX_POINT('',#90414) ;
#21816=VERTEX_POINT('',#90415) ;
#21817=VERTEX_POINT('',#90428) ;
#21818=VERTEX_POINT('',#90429) ;
#21819=VERTEX_POINT('',#90434) ;
#21820=VERTEX_POINT('',#90435) ;
#21821=VERTEX_POINT('',#90437) ;
#21822=VERTEX_POINT('',#90464) ;
#21823=VERTEX_POINT('',#90465) ;
#21824=VERTEX_POINT('',#90494) ;
#21825=VERTEX_POINT('',#90508) ;
#21826=VERTEX_POINT('',#90510) ;
#21827=VERTEX_POINT('',#90512) ;
#21828=VERTEX_POINT('',#90514) ;
#21829=VERTEX_POINT('',#90518) ;
#21830=VERTEX_POINT('',#90522) ;
#21831=VERTEX_POINT('',#90550) ;
#21832=VERTEX_POINT('',#90551) ;
#21833=VERTEX_POINT('',#90558) ;
#21834=VERTEX_POINT('',#90560) ;
#21835=VERTEX_POINT('',#90562) ;
#21836=VERTEX_POINT('',#90564) ;
#21837=VERTEX_POINT('',#90578) ;
#21838=VERTEX_POINT('',#90592) ;
#21839=VERTEX_POINT('',#90593) ;
#21840=VERTEX_POINT('',#90606) ;
#21841=VERTEX_POINT('',#90607) ;
#21842=VERTEX_POINT('',#90612) ;
#21843=VERTEX_POINT('',#90613) ;
#21844=VERTEX_POINT('',#90618) ;
#21845=VERTEX_POINT('',#90619) ;
#21846=VERTEX_POINT('',#90629) ;
#21847=VERTEX_POINT('',#90631) ;
#21848=VERTEX_POINT('',#90635) ;
#21849=VERTEX_POINT('',#90639) ;
#21850=VERTEX_POINT('',#90708) ;
#21851=VERTEX_POINT('',#90710) ;
#21852=VERTEX_POINT('',#90723) ;
#21853=VERTEX_POINT('',#90756) ;
#21854=VERTEX_POINT('',#90763) ;
#21855=VERTEX_POINT('',#90772) ;
#21856=VERTEX_POINT('',#90774) ;
#21857=VERTEX_POINT('',#90776) ;
#21858=VERTEX_POINT('',#90782) ;
#21859=VERTEX_POINT('',#90784) ;
#21860=VERTEX_POINT('',#90786) ;
#21861=VERTEX_POINT('',#90788) ;
#21862=VERTEX_POINT('',#90790) ;
#21863=VERTEX_POINT('',#90792) ;
#21864=VERTEX_POINT('',#90794) ;
#21865=VERTEX_POINT('',#90796) ;
#21866=VERTEX_POINT('',#90824) ;
#21867=VERTEX_POINT('',#90825) ;
#21868=VERTEX_POINT('',#90827) ;
#21869=VERTEX_POINT('',#90829) ;
#21870=VERTEX_POINT('',#90831) ;
#21871=VERTEX_POINT('',#90835) ;
#21872=VERTEX_POINT('',#90836) ;
#21873=VERTEX_POINT('',#90860) ;
#21874=VERTEX_POINT('',#90861) ;
#21875=VERTEX_POINT('',#90889) ;
#21876=VERTEX_POINT('',#90903) ;
#21877=VERTEX_POINT('',#90905) ;
#21878=VERTEX_POINT('',#90909) ;
#21879=VERTEX_POINT('',#90911) ;
#21880=VERTEX_POINT('',#90915) ;
#21881=VERTEX_POINT('',#90943) ;
#21882=VERTEX_POINT('',#90944) ;
#21883=VERTEX_POINT('',#90946) ;
#21884=VERTEX_POINT('',#90948) ;
#21885=VERTEX_POINT('',#90950) ;
#21886=VERTEX_POINT('',#90954) ;
#21887=VERTEX_POINT('',#90955) ;
#21888=VERTEX_POINT('',#90979) ;
#21889=VERTEX_POINT('',#90980) ;
#21890=VERTEX_POINT('',#91008) ;
#21891=VERTEX_POINT('',#91019) ;
#21892=VERTEX_POINT('',#91031) ;
#21893=VERTEX_POINT('',#91033) ;
#21894=VERTEX_POINT('',#91035) ;
#21895=VERTEX_POINT('',#91037) ;
#21896=VERTEX_POINT('',#91039) ;
#21897=VERTEX_POINT('',#91041) ;
#21898=VERTEX_POINT('',#91044) ;
#21899=VERTEX_POINT('',#91046) ;
#21900=VERTEX_POINT('',#91048) ;
#21901=VERTEX_POINT('',#91050) ;
#21902=VERTEX_POINT('',#91054) ;
#21903=VERTEX_POINT('',#91058) ;
#21904=VERTEX_POINT('',#91060) ;
#21905=VERTEX_POINT('',#91083) ;
#21906=VERTEX_POINT('',#91084) ;
#21907=VERTEX_POINT('',#91086) ;
#21908=VERTEX_POINT('',#91090) ;
#21909=VERTEX_POINT('',#91092) ;
#21910=VERTEX_POINT('',#91096) ;
#21911=VERTEX_POINT('',#91098) ;
#21912=VERTEX_POINT('',#91109) ;
#21913=VERTEX_POINT('',#91111) ;
#21914=VERTEX_POINT('',#91115) ;
#21915=VERTEX_POINT('',#91117) ;
#21916=VERTEX_POINT('',#91119) ;
#21917=VERTEX_POINT('',#91121) ;
#21918=VERTEX_POINT('',#91123) ;
#21919=VERTEX_POINT('',#91125) ;
#21920=VERTEX_POINT('',#91127) ;
#21921=VERTEX_POINT('',#91133) ;
#21922=VERTEX_POINT('',#91137) ;
#21923=VERTEX_POINT('',#91141) ;
#21924=VERTEX_POINT('',#91143) ;
#21925=VERTEX_POINT('',#91147) ;
#21926=VERTEX_POINT('',#91180) ;
#21927=VERTEX_POINT('',#91181) ;
#21928=VERTEX_POINT('',#91183) ;
#21929=VERTEX_POINT('',#91185) ;
#21930=VERTEX_POINT('',#91192) ;
#21931=VERTEX_POINT('',#91194) ;
#21932=VERTEX_POINT('',#91196) ;
#21933=VERTEX_POINT('',#91200) ;
#21934=VERTEX_POINT('',#91204) ;
#21935=VERTEX_POINT('',#91206) ;
#21936=VERTEX_POINT('',#91208) ;
#21937=VERTEX_POINT('',#91210) ;
#21938=VERTEX_POINT('',#91214) ;
#21939=VERTEX_POINT('',#91216) ;
#21940=VERTEX_POINT('',#91218) ;
#21941=VERTEX_POINT('',#91224) ;
#21942=VERTEX_POINT('',#91226) ;
#21943=VERTEX_POINT('',#91230) ;
#21944=VERTEX_POINT('',#91232) ;
#21945=VERTEX_POINT('',#91234) ;
#21946=VERTEX_POINT('',#91238) ;
#21947=VERTEX_POINT('',#91240) ;
#21948=VERTEX_POINT('',#91246) ;
#21949=VERTEX_POINT('',#91250) ;
#21950=VERTEX_POINT('',#91252) ;
#21951=VERTEX_POINT('',#91256) ;
#21952=VERTEX_POINT('',#91262) ;
#21953=VERTEX_POINT('',#91264) ;
#21954=VERTEX_POINT('',#91268) ;
#21955=VERTEX_POINT('',#91269) ;
#21956=VERTEX_POINT('',#91274) ;
#21957=VERTEX_POINT('',#91281) ;
#21958=VERTEX_POINT('',#91283) ;
#21959=VERTEX_POINT('',#91285) ;
#21960=VERTEX_POINT('',#91287) ;
#21961=VERTEX_POINT('',#91289) ;
#21962=VERTEX_POINT('',#91293) ;
#21963=VERTEX_POINT('',#91297) ;
#21964=VERTEX_POINT('',#91299) ;
#21965=VERTEX_POINT('',#91301) ;
#21966=VERTEX_POINT('',#91303) ;
#21967=VERTEX_POINT('',#91305) ;
#21968=VERTEX_POINT('',#91309) ;
#21969=VERTEX_POINT('',#91320) ;
#21970=VERTEX_POINT('',#91321) ;
#21971=VERTEX_POINT('',#91323) ;
#21972=VERTEX_POINT('',#91327) ;
#21973=VERTEX_POINT('',#91328) ;
#21974=VERTEX_POINT('',#91333) ;
#21975=VERTEX_POINT('',#91334) ;
#21976=VERTEX_POINT('',#91351) ;
#21977=VERTEX_POINT('',#91353) ;
#21978=VERTEX_POINT('',#91357) ;
#21979=VERTEX_POINT('',#91358) ;
#21980=VERTEX_POINT('',#91363) ;
#21981=VERTEX_POINT('',#91364) ;
#21982=VERTEX_POINT('',#91369) ;
#21983=VERTEX_POINT('',#91370) ;
#21984=VERTEX_POINT('',#91375) ;
#21985=VERTEX_POINT('',#91376) ;
#21986=VERTEX_POINT('',#91381) ;
#21987=VERTEX_POINT('',#91382) ;
#21988=VERTEX_POINT('',#91390) ;
#21989=VERTEX_POINT('',#91391) ;
#21990=VERTEX_POINT('',#91396) ;
#21991=VERTEX_POINT('',#91397) ;
#21992=VERTEX_POINT('',#91407) ;
#21993=VERTEX_POINT('',#91409) ;
#21994=VERTEX_POINT('',#91411) ;
#21995=VERTEX_POINT('',#91413) ;
#21996=VERTEX_POINT('',#91415) ;
#21997=VERTEX_POINT('',#91417) ;
#21998=VERTEX_POINT('',#91419) ;
#21999=VERTEX_POINT('',#91421) ;
#22000=VERTEX_POINT('',#91423) ;
#22001=VERTEX_POINT('',#91427) ;
#22002=VERTEX_POINT('',#91431) ;
#22003=VERTEX_POINT('',#91435) ;
#22004=VERTEX_POINT('',#91436) ;
#22005=VERTEX_POINT('',#91438) ;
#22006=VERTEX_POINT('',#91440) ;
#22007=VERTEX_POINT('',#91442) ;
#22008=VERTEX_POINT('',#91487) ;
#22009=VERTEX_POINT('',#91488) ;
#22010=VERTEX_POINT('',#91513) ;
#22011=VERTEX_POINT('',#91515) ;
#22012=VERTEX_POINT('',#91519) ;
#22013=VERTEX_POINT('',#91521) ;
#22014=VERTEX_POINT('',#91554) ;
#22015=VERTEX_POINT('',#91561) ;
#22016=VERTEX_POINT('',#91573) ;
#22017=VERTEX_POINT('',#91575) ;
#22018=VERTEX_POINT('',#91579) ;
#22019=VERTEX_POINT('',#91580) ;
#22020=VERTEX_POINT('',#91583) ;
#22021=VERTEX_POINT('',#91587) ;
#22022=VERTEX_POINT('',#91593) ;
#22023=VERTEX_POINT('',#91616) ;
#22024=VERTEX_POINT('',#91621) ;
#22025=VERTEX_POINT('',#91647) ;
#22026=VERTEX_POINT('',#91648) ;
#22027=VERTEX_POINT('',#91653) ;
#22028=VERTEX_POINT('',#91654) ;
#22029=VERTEX_POINT('',#91683) ;
#22030=VERTEX_POINT('',#91684) ;
#22031=VERTEX_POINT('',#91696) ;
#22032=VERTEX_POINT('',#91705) ;
#22033=VERTEX_POINT('',#91707) ;
#22034=VERTEX_POINT('',#91711) ;
#22035=VERTEX_POINT('',#91715) ;
#22036=VERTEX_POINT('',#91719) ;
#22037=VERTEX_POINT('',#91723) ;
#22038=VERTEX_POINT('',#91724) ;
#22039=VERTEX_POINT('',#91729) ;
#22040=VERTEX_POINT('',#91730) ;
#22041=VERTEX_POINT('',#91738) ;
#22042=VERTEX_POINT('',#91742) ;
#22043=VERTEX_POINT('',#91746) ;
#22044=VERTEX_POINT('',#91750) ;
#22045=VERTEX_POINT('',#91752) ;
#22046=VERTEX_POINT('',#91754) ;
#22047=VERTEX_POINT('',#91758) ;
#22048=VERTEX_POINT('',#91762) ;
#22049=VERTEX_POINT('',#91789) ;
#22050=VERTEX_POINT('',#91790) ;
#22051=VERTEX_POINT('',#91792) ;
#22052=VERTEX_POINT('',#91812) ;
#22053=VERTEX_POINT('',#91820) ;
#22054=VERTEX_POINT('',#91851) ;
#22055=VERTEX_POINT('',#91852) ;
#22056=VERTEX_POINT('',#91857) ;
#22057=VERTEX_POINT('',#91858) ;
#22058=VERTEX_POINT('',#91882) ;
#22059=VERTEX_POINT('',#91883) ;
#22060=VERTEX_POINT('',#91907) ;
#22061=VERTEX_POINT('',#91908) ;
#22062=VERTEX_POINT('',#91928) ;
#22063=VERTEX_POINT('',#91930) ;
#22064=VERTEX_POINT('',#91943) ;
#22065=VERTEX_POINT('',#91945) ;
#22066=VERTEX_POINT('',#91950) ;
#22067=VERTEX_POINT('',#91954) ;
#22068=VERTEX_POINT('',#91956) ;
#22069=VERTEX_POINT('',#91958) ;
#22070=VERTEX_POINT('',#91960) ;
#22071=VERTEX_POINT('',#91969) ;
#22072=VERTEX_POINT('',#91975) ;
#22073=VERTEX_POINT('',#91979) ;
#22074=VERTEX_POINT('',#91981) ;
#22075=VERTEX_POINT('',#91998) ;
#22076=VERTEX_POINT('',#92015) ;
#22077=VERTEX_POINT('',#92021) ;
#22078=VERTEX_POINT('',#92023) ;
#22079=VERTEX_POINT('',#92027) ;
#22080=VERTEX_POINT('',#92051) ;
#22081=VERTEX_POINT('',#92052) ;
#22082=VERTEX_POINT('',#92054) ;
#22083=VERTEX_POINT('',#92058) ;
#22084=VERTEX_POINT('',#92059) ;
#22085=VERTEX_POINT('',#92064) ;
#22086=VERTEX_POINT('',#92065) ;
#22087=VERTEX_POINT('',#92091) ;
#22088=VERTEX_POINT('',#92093) ;
#22089=VERTEX_POINT('',#92095) ;
#22090=VERTEX_POINT('',#92097) ;
#22091=VERTEX_POINT('',#92101) ;
#22092=VERTEX_POINT('',#92105) ;
#22093=VERTEX_POINT('',#92107) ;
#22094=VERTEX_POINT('',#92111) ;
#22095=VERTEX_POINT('',#92112) ;
#22096=VERTEX_POINT('',#92114) ;
#22097=VERTEX_POINT('',#92124) ;
#22098=VERTEX_POINT('',#92125) ;
#22099=VERTEX_POINT('',#92127) ;
#22100=VERTEX_POINT('',#92129) ;
#22101=VERTEX_POINT('',#92142) ;
#22102=VERTEX_POINT('',#92144) ;
#22103=VERTEX_POINT('',#92146) ;
#22104=VERTEX_POINT('',#92148) ;
#22105=VERTEX_POINT('',#92150) ;
#22106=VERTEX_POINT('',#92152) ;
#22107=VERTEX_POINT('',#92154) ;
#22108=VERTEX_POINT('',#92156) ;
#22109=VERTEX_POINT('',#92158) ;
#22110=VERTEX_POINT('',#92160) ;
#22111=VERTEX_POINT('',#92162) ;
#22112=VERTEX_POINT('',#92164) ;
#22113=VERTEX_POINT('',#92166) ;
#22114=VERTEX_POINT('',#92168) ;
#22115=VERTEX_POINT('',#92170) ;
#22116=VERTEX_POINT('',#92172) ;
#22117=VERTEX_POINT('',#92174) ;
#22118=VERTEX_POINT('',#92176) ;
#22119=VERTEX_POINT('',#92178) ;
#22120=VERTEX_POINT('',#92180) ;
#22121=VERTEX_POINT('',#92182) ;
#22122=VERTEX_POINT('',#92184) ;
#22123=VERTEX_POINT('',#92186) ;
#22124=VERTEX_POINT('',#92188) ;
#22125=VERTEX_POINT('',#92190) ;
#22126=VERTEX_POINT('',#92192) ;
#22127=VERTEX_POINT('',#92194) ;
#22128=VERTEX_POINT('',#92196) ;
#22129=VERTEX_POINT('',#92198) ;
#22130=VERTEX_POINT('',#92200) ;
#22131=VERTEX_POINT('',#92202) ;
#22132=VERTEX_POINT('',#92204) ;
#22133=VERTEX_POINT('',#92206) ;
#22134=VERTEX_POINT('',#92208) ;
#22135=VERTEX_POINT('',#92210) ;
#22136=VERTEX_POINT('',#92212) ;
#22137=VERTEX_POINT('',#92214) ;
#22138=VERTEX_POINT('',#92216) ;
#22139=VERTEX_POINT('',#92218) ;
#22140=VERTEX_POINT('',#92220) ;
#22141=VERTEX_POINT('',#92222) ;
#22142=VERTEX_POINT('',#92224) ;
#22143=VERTEX_POINT('',#92226) ;
#22144=VERTEX_POINT('',#92233) ;
#22145=VERTEX_POINT('',#92235) ;
#22146=VERTEX_POINT('',#92242) ;
#22147=VERTEX_POINT('',#92244) ;
#22148=VERTEX_POINT('',#92246) ;
#22149=VERTEX_POINT('',#92248) ;
#22150=VERTEX_POINT('',#92250) ;
#22151=VERTEX_POINT('',#92252) ;
#22152=VERTEX_POINT('',#92254) ;
#22153=VERTEX_POINT('',#92256) ;
#22154=VERTEX_POINT('',#92258) ;
#22155=VERTEX_POINT('',#92260) ;
#22156=VERTEX_POINT('',#92262) ;
#22157=VERTEX_POINT('',#92264) ;
#22158=VERTEX_POINT('',#92266) ;
#22159=VERTEX_POINT('',#92275) ;
#22160=VERTEX_POINT('',#92277) ;
#22161=VERTEX_POINT('',#92279) ;
#22162=VERTEX_POINT('',#92281) ;
#22163=VERTEX_POINT('',#92283) ;
#22164=VERTEX_POINT('',#92285) ;
#22165=VERTEX_POINT('',#92287) ;
#22166=VERTEX_POINT('',#92289) ;
#22167=VERTEX_POINT('',#92291) ;
#22168=VERTEX_POINT('',#92293) ;
#22169=VERTEX_POINT('',#92295) ;
#22170=VERTEX_POINT('',#92297) ;
#22171=VERTEX_POINT('',#92299) ;
#22172=VERTEX_POINT('',#92301) ;
#22173=VERTEX_POINT('',#92303) ;
#22174=VERTEX_POINT('',#92305) ;
#22175=VERTEX_POINT('',#92307) ;
#22176=VERTEX_POINT('',#92309) ;
#22177=VERTEX_POINT('',#92311) ;
#22178=VERTEX_POINT('',#92313) ;
#22179=VERTEX_POINT('',#92315) ;
#22180=VERTEX_POINT('',#92317) ;
#22181=VERTEX_POINT('',#92319) ;
#22182=VERTEX_POINT('',#92321) ;
#22183=VERTEX_POINT('',#92323) ;
#22184=VERTEX_POINT('',#92325) ;
#22185=VERTEX_POINT('',#92327) ;
#22186=VERTEX_POINT('',#92329) ;
#22187=VERTEX_POINT('',#92331) ;
#22188=VERTEX_POINT('',#92333) ;
#22189=VERTEX_POINT('',#92336) ;
#22190=VERTEX_POINT('',#92338) ;
#22191=VERTEX_POINT('',#92340) ;
#22192=VERTEX_POINT('',#92342) ;
#22193=VERTEX_POINT('',#92344) ;
#22194=VERTEX_POINT('',#92346) ;
#22195=VERTEX_POINT('',#92348) ;
#22196=VERTEX_POINT('',#92350) ;
#22197=VERTEX_POINT('',#92352) ;
#22198=VERTEX_POINT('',#92354) ;
#22199=VERTEX_POINT('',#92356) ;
#22200=VERTEX_POINT('',#92359) ;
#22201=VERTEX_POINT('',#92360) ;
#22202=VERTEX_POINT('',#92362) ;
#22203=VERTEX_POINT('',#92364) ;
#22204=VERTEX_POINT('',#92366) ;
#22205=VERTEX_POINT('',#92368) ;
#22206=VERTEX_POINT('',#92370) ;
#22207=VERTEX_POINT('',#92372) ;
#22208=VERTEX_POINT('',#92375) ;
#22209=VERTEX_POINT('',#92377) ;
#22210=VERTEX_POINT('',#92378) ;
#22211=VERTEX_POINT('',#92380) ;
#22212=VERTEX_POINT('',#92382) ;
#22213=VERTEX_POINT('',#92384) ;
#22214=VERTEX_POINT('',#92386) ;
#22215=VERTEX_POINT('',#92388) ;
#22216=VERTEX_POINT('',#92390) ;
#22217=VERTEX_POINT('',#92392) ;
#22218=VERTEX_POINT('',#92394) ;
#22219=VERTEX_POINT('',#92396) ;
#22220=VERTEX_POINT('',#92398) ;
#22221=VERTEX_POINT('',#92400) ;
#22222=VERTEX_POINT('',#92402) ;
#22223=VERTEX_POINT('',#92405) ;
#22224=VERTEX_POINT('',#92407) ;
#22225=VERTEX_POINT('',#92408) ;
#22226=VERTEX_POINT('',#92410) ;
#22227=VERTEX_POINT('',#92417) ;
#22228=VERTEX_POINT('',#92419) ;
#22229=VERTEX_POINT('',#92421) ;
#22230=VERTEX_POINT('',#92423) ;
#22231=VERTEX_POINT('',#92425) ;
#22232=VERTEX_POINT('',#92427) ;
#22233=VERTEX_POINT('',#92429) ;
#22234=VERTEX_POINT('',#92431) ;
#22235=VERTEX_POINT('',#92433) ;
#22236=VERTEX_POINT('',#92441) ;
#22237=VERTEX_POINT('',#92442) ;
#22238=VERTEX_POINT('',#92450) ;
#22239=VERTEX_POINT('',#92452) ;
#22240=VERTEX_POINT('',#92454) ;
#22241=VERTEX_POINT('',#92456) ;
#22242=VERTEX_POINT('',#92458) ;
#22243=VERTEX_POINT('',#92460) ;
#22244=VERTEX_POINT('',#92462) ;
#22245=VERTEX_POINT('',#92464) ;
#22246=VERTEX_POINT('',#92466) ;
#22247=VERTEX_POINT('',#92468) ;
#22248=VERTEX_POINT('',#92471) ;
#22249=VERTEX_POINT('',#92472) ;
#22250=VERTEX_POINT('',#92474) ;
#22251=VERTEX_POINT('',#92476) ;
#22252=VERTEX_POINT('',#92478) ;
#22253=VERTEX_POINT('',#92480) ;
#22254=VERTEX_POINT('',#92482) ;
#22255=VERTEX_POINT('',#92484) ;
#22256=VERTEX_POINT('',#92486) ;
#22257=VERTEX_POINT('',#92488) ;
#22258=VERTEX_POINT('',#92490) ;
#22259=VERTEX_POINT('',#92492) ;
#22260=VERTEX_POINT('',#92494) ;
#22261=VERTEX_POINT('',#92496) ;
#22262=VERTEX_POINT('',#92556) ;
#22263=VERTEX_POINT('',#92557) ;
#22264=VERTEX_POINT('',#92566) ;
#22265=VERTEX_POINT('',#92581) ;
#22266=VERTEX_POINT('',#92603) ;
#22267=VERTEX_POINT('',#92607) ;
#22268=VERTEX_POINT('',#92613) ;
#22269=VERTEX_POINT('',#92615) ;
#22270=VERTEX_POINT('',#92619) ;
#22271=VERTEX_POINT('',#92622) ;
#22272=VERTEX_POINT('',#92627) ;
#22273=VERTEX_POINT('',#92629) ;
#22274=VERTEX_POINT('',#92633) ;
#22275=VERTEX_POINT('',#92634) ;
#22276=VERTEX_POINT('',#92636) ;
#22277=VERTEX_POINT('',#92640) ;
#22278=VERTEX_POINT('',#92642) ;
#22279=VERTEX_POINT('',#92646) ;
#22280=VERTEX_POINT('',#92647) ;
#22281=VERTEX_POINT('',#92652) ;
#22282=VERTEX_POINT('',#92653) ;
#22283=VERTEX_POINT('',#92658) ;
#22284=VERTEX_POINT('',#92659) ;
#22285=VERTEX_POINT('',#92667) ;
#22286=VERTEX_POINT('',#92668) ;
#22287=VERTEX_POINT('',#92683) ;
#22288=VERTEX_POINT('',#92685) ;
#22289=VERTEX_POINT('',#92689) ;
#22290=VERTEX_POINT('',#92690) ;
#22291=VERTEX_POINT('',#92746) ;
#22292=VERTEX_POINT('',#92748) ;
#22293=VERTEX_POINT('',#92750) ;
#22294=VERTEX_POINT('',#92754) ;
#22295=VERTEX_POINT('',#92766) ;
#22296=VERTEX_POINT('',#92770) ;
#22297=VERTEX_POINT('',#92774) ;
#22298=VERTEX_POINT('',#92783) ;
#22299=VERTEX_POINT('',#92787) ;
#22300=VERTEX_POINT('',#92791) ;
#22301=VERTEX_POINT('',#92809) ;
#22302=VERTEX_POINT('',#92840) ;
#22303=VERTEX_POINT('',#92842) ;
#22304=VERTEX_POINT('',#92846) ;
#22305=VERTEX_POINT('',#92848) ;
#22306=VERTEX_POINT('',#92850) ;
#22307=VERTEX_POINT('',#92854) ;
#22308=VERTEX_POINT('',#92858) ;
#22309=VERTEX_POINT('',#92862) ;
#22310=VERTEX_POINT('',#92866) ;
#22311=VERTEX_POINT('',#92868) ;
#22312=VERTEX_POINT('',#92870) ;
#22313=VERTEX_POINT('',#92872) ;
#22314=VERTEX_POINT('',#92874) ;
#22315=VERTEX_POINT('',#92876) ;
#22316=VERTEX_POINT('',#92878) ;
#22317=VERTEX_POINT('',#92882) ;
#22318=VERTEX_POINT('',#92886) ;
#22319=VERTEX_POINT('',#92890) ;
#22320=VERTEX_POINT('',#92894) ;
#22321=VERTEX_POINT('',#92896) ;
#22322=VERTEX_POINT('',#92932) ;
#22323=VERTEX_POINT('',#92933) ;
#22324=VERTEX_POINT('',#92935) ;
#22325=VERTEX_POINT('',#92961) ;
#22326=VERTEX_POINT('',#92970) ;
#22327=VERTEX_POINT('',#92971) ;
#22328=VERTEX_POINT('',#92976) ;
#22329=VERTEX_POINT('',#92977) ;
#22330=VERTEX_POINT('',#92979) ;
#22331=VERTEX_POINT('',#92981) ;
#22332=VERTEX_POINT('',#92985) ;
#22333=VERTEX_POINT('',#92986) ;
#22334=VERTEX_POINT('',#92994) ;
#22335=VERTEX_POINT('',#92995) ;
#22336=VERTEX_POINT('',#92997) ;
#22337=VERTEX_POINT('',#92999) ;
#22338=VERTEX_POINT('',#93032) ;
#22339=VERTEX_POINT('',#93033) ;
#22340=VERTEX_POINT('',#93059) ;
#22341=VERTEX_POINT('',#93061) ;
#22342=VERTEX_POINT('',#93070) ;
#22343=VERTEX_POINT('',#93071) ;
#22344=VERTEX_POINT('',#93079) ;
#22345=VERTEX_POINT('',#93080) ;
#22346=VERTEX_POINT('',#93109) ;
#22347=VERTEX_POINT('',#93141) ;
#22348=VERTEX_POINT('',#93147) ;
#22349=VERTEX_POINT('',#93148) ;
#22350=VERTEX_POINT('',#93153) ;
#22351=VERTEX_POINT('',#93157) ;
#22352=VERTEX_POINT('',#93161) ;
#22353=VERTEX_POINT('',#93167) ;
#22354=VERTEX_POINT('',#93168) ;
#22355=VERTEX_POINT('',#93173) ;
#22356=VERTEX_POINT('',#93174) ;
#22357=VERTEX_POINT('',#93179) ;
#22358=VERTEX_POINT('',#93180) ;
#22359=VERTEX_POINT('',#93185) ;
#22360=VERTEX_POINT('',#93186) ;
#22361=VERTEX_POINT('',#93191) ;
#22362=VERTEX_POINT('',#93192) ;
#22363=VERTEX_POINT('',#93197) ;
#22364=VERTEX_POINT('',#93198) ;
#22365=VERTEX_POINT('',#93203) ;
#22366=VERTEX_POINT('',#93204) ;
#22367=VERTEX_POINT('',#93209) ;
#22368=VERTEX_POINT('',#93210) ;
#22369=VERTEX_POINT('',#93215) ;
#22370=VERTEX_POINT('',#93216) ;
#22371=VERTEX_POINT('',#93224) ;
#22372=VERTEX_POINT('',#93225) ;
#22373=VERTEX_POINT('',#93254) ;
#22374=VERTEX_POINT('',#93288) ;
#22375=VERTEX_POINT('',#93289) ;
#22376=VERTEX_POINT('',#93294) ;
#22377=VERTEX_POINT('',#93298) ;
#22378=VERTEX_POINT('',#93305) ;
#22379=VERTEX_POINT('',#93307) ;
#22380=VERTEX_POINT('',#93318) ;
#22381=VERTEX_POINT('',#93320) ;
#22382=VERTEX_POINT('',#93325) ;
#22383=VERTEX_POINT('',#93331) ;
#22384=VERTEX_POINT('',#93338) ;
#22385=VERTEX_POINT('',#93342) ;
#22386=VERTEX_POINT('',#93343) ;
#22387=VERTEX_POINT('',#93345) ;
#22388=VERTEX_POINT('',#93347) ;
#22389=VERTEX_POINT('',#93351) ;
#22390=VERTEX_POINT('',#93353) ;
#22391=VERTEX_POINT('',#93357) ;
#22392=VERTEX_POINT('',#93359) ;
#22393=VERTEX_POINT('',#93363) ;
#22394=VERTEX_POINT('',#93364) ;
#22395=VERTEX_POINT('',#93366) ;
#22396=VERTEX_POINT('',#93368) ;
#22397=VERTEX_POINT('',#93372) ;
#22398=VERTEX_POINT('',#93373) ;
#22399=VERTEX_POINT('',#93375) ;
#22400=VERTEX_POINT('',#93377) ;
#22401=VERTEX_POINT('',#93384) ;
#22402=VERTEX_POINT('',#93385) ;
#22403=VERTEX_POINT('',#93387) ;
#22404=VERTEX_POINT('',#93389) ;
#22405=VERTEX_POINT('',#93393) ;
#22406=VERTEX_POINT('',#93394) ;
#22407=VERTEX_POINT('',#93402) ;
#22408=VERTEX_POINT('',#93403) ;
#22409=VERTEX_POINT('',#93408) ;
#22410=VERTEX_POINT('',#93409) ;
#22411=VERTEX_POINT('',#93414) ;
#22412=VERTEX_POINT('',#93415) ;
#22413=VERTEX_POINT('',#93420) ;
#22414=VERTEX_POINT('',#93421) ;
#22415=VERTEX_POINT('',#93426) ;
#22416=VERTEX_POINT('',#93427) ;
#22417=VERTEX_POINT('',#93432) ;
#22418=VERTEX_POINT('',#93434) ;
#22419=VERTEX_POINT('',#93438) ;
#22420=VERTEX_POINT('',#93440) ;
#22421=VERTEX_POINT('',#93442) ;
#22422=VERTEX_POINT('',#93444) ;
#22423=VERTEX_POINT('',#93446) ;
#22424=VERTEX_POINT('',#93448) ;
#22425=VERTEX_POINT('',#93450) ;
#22426=VERTEX_POINT('',#93452) ;
#22427=VERTEX_POINT('',#93454) ;
#22428=VERTEX_POINT('',#93456) ;
#22429=VERTEX_POINT('',#93460) ;
#22430=VERTEX_POINT('',#93464) ;
#22431=VERTEX_POINT('',#93466) ;
#22432=VERTEX_POINT('',#93468) ;
#22433=VERTEX_POINT('',#93470) ;
#22434=VERTEX_POINT('',#93476) ;
#22435=VERTEX_POINT('',#93478) ;
#22436=VERTEX_POINT('',#93516) ;
#22437=VERTEX_POINT('',#93522) ;
#22438=VERTEX_POINT('',#93526) ;
#22439=VERTEX_POINT('',#93530) ;
#22440=VERTEX_POINT('',#93534) ;
#22441=VERTEX_POINT('',#93538) ;
#22442=VERTEX_POINT('',#93542) ;
#22443=VERTEX_POINT('',#93546) ;
#22444=VERTEX_POINT('',#93550) ;
#22445=VERTEX_POINT('',#93554) ;
#22446=VERTEX_POINT('',#93558) ;
#22447=VERTEX_POINT('',#93585) ;
#22448=VERTEX_POINT('',#93589) ;
#22449=VERTEX_POINT('',#93620) ;
#22450=VERTEX_POINT('',#93651) ;
#22451=VERTEX_POINT('',#93688) ;
#22452=VERTEX_POINT('',#93692) ;
#22453=VERTEX_POINT('',#93696) ;
#22454=VERTEX_POINT('',#93700) ;
#22455=VERTEX_POINT('',#93713) ;
#22456=VERTEX_POINT('',#93728) ;
#22457=VERTEX_POINT('',#93734) ;
#22458=VERTEX_POINT('',#93738) ;
#22459=VERTEX_POINT('',#93744) ;
#22460=VERTEX_POINT('',#93748) ;
#22461=VERTEX_POINT('',#93759) ;
#22462=VERTEX_POINT('',#93763) ;
#22463=VERTEX_POINT('',#93767) ;
#22464=VERTEX_POINT('',#93771) ;
#22465=VERTEX_POINT('',#93772) ;
#22466=VERTEX_POINT('',#93774) ;
#22467=VERTEX_POINT('',#93776) ;
#22468=VERTEX_POINT('',#93780) ;
#22469=VERTEX_POINT('',#93785) ;
#22470=VERTEX_POINT('',#93789) ;
#22471=VERTEX_POINT('',#93793) ;
#22472=VERTEX_POINT('',#93797) ;
#22473=VERTEX_POINT('',#93807) ;
#22474=VERTEX_POINT('',#93809) ;
#22475=VERTEX_POINT('',#93811) ;
#22476=VERTEX_POINT('',#93813) ;
#22477=VERTEX_POINT('',#93815) ;
#22478=VERTEX_POINT('',#93818) ;
#22479=VERTEX_POINT('',#93819) ;
#22480=VERTEX_POINT('',#93843) ;
#22481=VERTEX_POINT('',#93845) ;
#22482=VERTEX_POINT('',#93857) ;
#22483=VERTEX_POINT('',#93859) ;
#22484=VERTEX_POINT('',#93861) ;
#22485=VERTEX_POINT('',#93864) ;
#22486=VERTEX_POINT('',#93865) ;
#22487=VERTEX_POINT('',#93867) ;
#22488=VERTEX_POINT('',#93869) ;
#22489=VERTEX_POINT('',#93871) ;
#22490=VERTEX_POINT('',#93888) ;
#22491=VERTEX_POINT('',#93890) ;
#22492=VERTEX_POINT('',#93904) ;
#22493=VERTEX_POINT('',#93908) ;
#22494=VERTEX_POINT('',#93910) ;
#22495=VERTEX_POINT('',#93914) ;
#22496=VERTEX_POINT('',#93917) ;
#22497=VERTEX_POINT('',#93920) ;
#22498=VERTEX_POINT('',#93923) ;
#22499=VERTEX_POINT('',#93927) ;
#22500=VERTEX_POINT('',#93929) ;
#22501=VERTEX_POINT('',#93931) ;
#22502=VERTEX_POINT('',#93967) ;
#22503=VERTEX_POINT('',#93968) ;
#22504=VERTEX_POINT('',#93970) ;
#22505=VERTEX_POINT('',#93972) ;
#22506=VERTEX_POINT('',#94005) ;
#22507=VERTEX_POINT('',#94006) ;
#22508=VERTEX_POINT('',#94008) ;
#22509=VERTEX_POINT('',#94010) ;
#22510=VERTEX_POINT('',#94014) ;
#22511=VERTEX_POINT('',#94016) ;
#22512=VERTEX_POINT('',#94044) ;
#22513=VERTEX_POINT('',#94045) ;
#22514=VERTEX_POINT('',#94081) ;
#22515=VERTEX_POINT('',#94082) ;
#22516=VERTEX_POINT('',#94090) ;
#22517=VERTEX_POINT('',#94091) ;
#22518=VERTEX_POINT('',#94099) ;
#22519=VERTEX_POINT('',#94100) ;
#22520=VERTEX_POINT('',#94105) ;
#22521=VERTEX_POINT('',#94129) ;
#22522=VERTEX_POINT('',#94157) ;
#22523=VERTEX_POINT('',#94159) ;
#22524=VERTEX_POINT('',#94167) ;
#22525=VERTEX_POINT('',#94169) ;
#22526=VERTEX_POINT('',#94173) ;
#22527=VERTEX_POINT('',#94175) ;
#22528=VERTEX_POINT('',#94177) ;
#22529=VERTEX_POINT('',#94193) ;
#22530=VERTEX_POINT('',#94194) ;
#22531=VERTEX_POINT('',#94199) ;
#22532=VERTEX_POINT('',#94201) ;
#22533=VERTEX_POINT('',#94203) ;
#22534=VERTEX_POINT('',#94208) ;
#22535=VERTEX_POINT('',#94210) ;
#22536=VERTEX_POINT('',#94212) ;
#22537=VERTEX_POINT('',#94216) ;
#22538=VERTEX_POINT('',#94242) ;
#22539=VERTEX_POINT('',#94315) ;
#22540=VERTEX_POINT('',#94373) ;
#22541=VERTEX_POINT('',#94411) ;
#22542=VERTEX_POINT('',#94432) ;
#22543=VERTEX_POINT('',#94437) ;
#22544=VERTEX_POINT('',#94439) ;
#22545=VERTEX_POINT('',#94444) ;
#22546=VERTEX_POINT('',#94446) ;
#22547=VERTEX_POINT('',#94478) ;
#22548=VERTEX_POINT('',#94482) ;
#22549=VERTEX_POINT('',#94483) ;
#22550=VERTEX_POINT('',#94515) ;
#22551=VERTEX_POINT('',#94539) ;
#22552=VERTEX_POINT('',#94560) ;
#22553=VERTEX_POINT('',#94562) ;
#22554=VERTEX_POINT('',#94564) ;
#22555=VERTEX_POINT('',#94566) ;
#22556=VERTEX_POINT('',#94568) ;
#22557=VERTEX_POINT('',#94571) ;
#22558=VERTEX_POINT('',#94574) ;
#22559=VERTEX_POINT('',#94575) ;
#22560=VERTEX_POINT('',#94577) ;
#22561=VERTEX_POINT('',#94579) ;
#22562=VERTEX_POINT('',#94581) ;
#22563=VERTEX_POINT('',#94583) ;
#22564=VERTEX_POINT('',#94585) ;
#22565=VERTEX_POINT('',#94587) ;
#22566=VERTEX_POINT('',#94589) ;
#22567=VERTEX_POINT('',#94591) ;
#22568=VERTEX_POINT('',#94593) ;
#22569=VERTEX_POINT('',#94596) ;
#22570=VERTEX_POINT('',#94597) ;
#22571=VERTEX_POINT('',#94599) ;
#22572=VERTEX_POINT('',#94601) ;
#22573=VERTEX_POINT('',#94603) ;
#22574=VERTEX_POINT('',#94605) ;
#22575=VERTEX_POINT('',#94607) ;
#22576=VERTEX_POINT('',#94609) ;
#22577=VERTEX_POINT('',#94611) ;
#22578=VERTEX_POINT('',#94613) ;
#22579=VERTEX_POINT('',#94615) ;
#22580=VERTEX_POINT('',#94618) ;
#22581=VERTEX_POINT('',#94619) ;
#22582=VERTEX_POINT('',#94621) ;
#22583=VERTEX_POINT('',#94623) ;
#22584=VERTEX_POINT('',#94630) ;
#22585=VERTEX_POINT('',#94667) ;
#22586=VERTEX_POINT('',#94671) ;
#22587=VERTEX_POINT('',#94684) ;
#22588=VERTEX_POINT('',#94733) ;
#22589=VERTEX_POINT('',#94776) ;
#22590=VERTEX_POINT('',#94782) ;
#22591=VERTEX_POINT('',#94786) ;
#22592=VERTEX_POINT('',#94793) ;
#22593=VERTEX_POINT('',#94804) ;
#22594=VERTEX_POINT('',#94806) ;
#22595=VERTEX_POINT('',#94809) ;
#22596=VERTEX_POINT('',#94831) ;
#22597=VERTEX_POINT('',#94832) ;
#22598=VERTEX_POINT('',#94834) ;
#22599=VERTEX_POINT('',#94836) ;
#22600=VERTEX_POINT('',#94841) ;
#22601=VERTEX_POINT('',#94845) ;
#22602=VERTEX_POINT('',#94847) ;
#22603=VERTEX_POINT('',#94888) ;
#22604=VERTEX_POINT('',#94890) ;
#22605=VERTEX_POINT('',#94894) ;
#22606=VERTEX_POINT('',#94898) ;
#22607=VERTEX_POINT('',#94902) ;
#22608=VERTEX_POINT('',#94908) ;
#22609=VERTEX_POINT('',#94910) ;
#22610=VERTEX_POINT('',#94912) ;
#22611=VERTEX_POINT('',#94914) ;
#22612=VERTEX_POINT('',#94917) ;
#22613=VERTEX_POINT('',#94931) ;
#22614=VERTEX_POINT('',#94933) ;
#22615=VERTEX_POINT('',#94937) ;
#22616=VERTEX_POINT('',#94939) ;
#22617=VERTEX_POINT('',#94953) ;
#22618=VERTEX_POINT('',#94954) ;
#22619=VERTEX_POINT('',#94956) ;
#22620=VERTEX_POINT('',#94971) ;
#22621=VERTEX_POINT('',#95024) ;
#22622=VERTEX_POINT('',#95035) ;
#22623=VERTEX_POINT('',#95157) ;
#22624=VERTEX_POINT('',#95159) ;
#22625=VERTEX_POINT('',#95230) ;
#22626=VERTEX_POINT('',#95242) ;
#22627=VERTEX_POINT('',#95269) ;
#22628=VERTEX_POINT('',#95271) ;
#22629=VERTEX_POINT('',#95275) ;
#22630=VERTEX_POINT('',#95277) ;
#22631=VERTEX_POINT('',#95284) ;
#22632=VERTEX_POINT('',#95286) ;
#22633=VERTEX_POINT('',#95290) ;
#22634=VERTEX_POINT('',#95294) ;
#22635=VERTEX_POINT('',#95298) ;
#22636=VERTEX_POINT('',#95382) ;
#22637=VERTEX_POINT('',#95383) ;
#22638=VERTEX_POINT('',#95400) ;
#22639=VERTEX_POINT('',#95415) ;
#22640=VERTEX_POINT('',#95537) ;
#22641=VERTEX_POINT('',#95539) ;
#22642=VERTEX_POINT('',#95543) ;
#22643=VERTEX_POINT('',#95545) ;
#22644=VERTEX_POINT('',#95549) ;
#22645=VERTEX_POINT('',#95551) ;
#22646=VERTEX_POINT('',#95555) ;
#22647=VERTEX_POINT('',#95557) ;
#22648=VERTEX_POINT('',#95638) ;
#22649=VERTEX_POINT('',#95754) ;
#22650=VERTEX_POINT('',#95786) ;
#22651=VERTEX_POINT('',#95788) ;
#22652=VERTEX_POINT('',#95811) ;
#22653=VERTEX_POINT('',#95965) ;
#22654=VERTEX_POINT('',#95988) ;
#22655=VERTEX_POINT('',#96077) ;
#22656=VERTEX_POINT('',#96078) ;
#22657=VERTEX_POINT('',#96080) ;
#22658=VERTEX_POINT('',#96082) ;
#22659=VERTEX_POINT('',#96086) ;
#22660=VERTEX_POINT('',#96088) ;
#22661=VERTEX_POINT('',#96092) ;
#22662=VERTEX_POINT('',#96094) ;
#22663=VERTEX_POINT('',#96098) ;
#22664=VERTEX_POINT('',#96100) ;
#22665=VERTEX_POINT('',#96104) ;
#22666=VERTEX_POINT('',#96106) ;
#22667=VERTEX_POINT('',#96110) ;
#22668=VERTEX_POINT('',#96112) ;
#22669=VERTEX_POINT('',#96119) ;
#22670=VERTEX_POINT('',#96121) ;
#22671=VERTEX_POINT('',#96125) ;
#22672=VERTEX_POINT('',#96129) ;
#22673=VERTEX_POINT('',#96133) ;
#22674=VERTEX_POINT('',#96138) ;
#22675=VERTEX_POINT('',#96139) ;
#22676=VERTEX_POINT('',#96141) ;
#22677=VERTEX_POINT('',#96143) ;
#22678=VERTEX_POINT('',#96147) ;
#22679=VERTEX_POINT('',#96149) ;
#22680=VERTEX_POINT('',#96153) ;
#22681=VERTEX_POINT('',#96155) ;
#22682=VERTEX_POINT('',#96162) ;
#22683=VERTEX_POINT('',#96164) ;
#22684=VERTEX_POINT('',#96168) ;
#22685=VERTEX_POINT('',#96173) ;
#22686=VERTEX_POINT('',#96174) ;
#22687=VERTEX_POINT('',#96176) ;
#22688=VERTEX_POINT('',#96178) ;
#22689=VERTEX_POINT('',#96182) ;
#22690=VERTEX_POINT('',#96184) ;
#22691=VERTEX_POINT('',#96188) ;
#22692=VERTEX_POINT('',#96190) ;
#22693=VERTEX_POINT('',#96194) ;
#22694=VERTEX_POINT('',#96196) ;
#22695=VERTEX_POINT('',#96200) ;
#22696=VERTEX_POINT('',#96202) ;
#22697=VERTEX_POINT('',#96206) ;
#22698=VERTEX_POINT('',#96208) ;
#22699=VERTEX_POINT('',#96215) ;
#22700=VERTEX_POINT('',#96217) ;
#22701=VERTEX_POINT('',#96221) ;
#22702=VERTEX_POINT('',#96225) ;
#22703=VERTEX_POINT('',#96229) ;
#22704=VERTEX_POINT('',#96234) ;
#22705=VERTEX_POINT('',#96235) ;
#22706=VERTEX_POINT('',#96237) ;
#22707=VERTEX_POINT('',#96239) ;
#22708=VERTEX_POINT('',#96243) ;
#22709=VERTEX_POINT('',#96245) ;
#22710=VERTEX_POINT('',#96249) ;
#22711=VERTEX_POINT('',#96251) ;
#22712=VERTEX_POINT('',#96258) ;
#22713=VERTEX_POINT('',#96260) ;
#22714=VERTEX_POINT('',#96264) ;
#22715=VERTEX_POINT('',#96269) ;
#22716=VERTEX_POINT('',#96270) ;
#22717=VERTEX_POINT('',#96272) ;
#22718=VERTEX_POINT('',#96274) ;
#22719=VERTEX_POINT('',#96278) ;
#22720=VERTEX_POINT('',#96280) ;
#22721=VERTEX_POINT('',#96284) ;
#22722=VERTEX_POINT('',#96286) ;
#22723=VERTEX_POINT('',#96290) ;
#22724=VERTEX_POINT('',#96291) ;
#22725=VERTEX_POINT('',#96296) ;
#22726=VERTEX_POINT('',#96298) ;
#22727=VERTEX_POINT('',#96302) ;
#22728=VERTEX_POINT('',#96304) ;
#22729=VERTEX_POINT('',#96308) ;
#22730=VERTEX_POINT('',#96310) ;
#22731=VERTEX_POINT('',#96314) ;
#22732=VERTEX_POINT('',#96315) ;
#22733=VERTEX_POINT('',#96320) ;
#22734=VERTEX_POINT('',#96322) ;
#22735=VERTEX_POINT('',#96326) ;
#22736=VERTEX_POINT('',#96328) ;
#22737=VERTEX_POINT('',#96335) ;
#22738=VERTEX_POINT('',#96337) ;
#22739=VERTEX_POINT('',#96341) ;
#22740=VERTEX_POINT('',#96345) ;
#22741=VERTEX_POINT('',#96349) ;
#22742=VERTEX_POINT('',#96353) ;
#22743=VERTEX_POINT('',#96357) ;
#22744=VERTEX_POINT('',#96362) ;
#22745=VERTEX_POINT('',#96363) ;
#22746=VERTEX_POINT('',#96365) ;
#22747=VERTEX_POINT('',#96367) ;
#22748=VERTEX_POINT('',#96371) ;
#22749=VERTEX_POINT('',#96373) ;
#22750=VERTEX_POINT('',#96377) ;
#22751=VERTEX_POINT('',#96378) ;
#22752=VERTEX_POINT('',#96383) ;
#22753=VERTEX_POINT('',#96385) ;
#22754=VERTEX_POINT('',#96389) ;
#22755=VERTEX_POINT('',#96391) ;
#22756=VERTEX_POINT('',#96395) ;
#22757=VERTEX_POINT('',#96397) ;
#22758=VERTEX_POINT('',#96401) ;
#22759=VERTEX_POINT('',#96402) ;
#22760=VERTEX_POINT('',#96407) ;
#22761=VERTEX_POINT('',#96409) ;
#22762=VERTEX_POINT('',#96413) ;
#22763=VERTEX_POINT('',#96415) ;
#22764=VERTEX_POINT('',#96419) ;
#22765=VERTEX_POINT('',#96421) ;
#22766=VERTEX_POINT('',#96428) ;
#22767=VERTEX_POINT('',#96430) ;
#22768=VERTEX_POINT('',#96434) ;
#22769=VERTEX_POINT('',#96438) ;
#22770=VERTEX_POINT('',#96442) ;
#22771=VERTEX_POINT('',#96446) ;
#22772=VERTEX_POINT('',#96450) ;
#22773=VERTEX_POINT('',#96606) ;
#22774=VERTEX_POINT('',#96758) ;
#22775=VERTEX_POINT('',#97051) ;
#22776=VERTEX_POINT('',#97053) ;
#22777=VERTEX_POINT('',#97193) ;
#22778=VERTEX_POINT('',#97194) ;
#22779=VERTEX_POINT('',#97197) ;
#22780=VERTEX_POINT('',#97201) ;
#22781=VERTEX_POINT('',#97203) ;
#22782=VERTEX_POINT('',#97207) ;
#22783=VERTEX_POINT('',#97211) ;
#22784=VERTEX_POINT('',#97215) ;
#22785=VERTEX_POINT('',#97219) ;
#22786=VERTEX_POINT('',#97231) ;
#22787=VERTEX_POINT('',#97232) ;
#22788=VERTEX_POINT('',#97234) ;
#22789=VERTEX_POINT('',#97236) ;
#22790=VERTEX_POINT('',#97239) ;
#22791=VERTEX_POINT('',#97241) ;
#22792=VERTEX_POINT('',#97243) ;
#22793=VERTEX_POINT('',#97246) ;
#22794=VERTEX_POINT('',#97296) ;
#22795=VERTEX_POINT('',#97299) ;
#22796=VERTEX_POINT('',#97300) ;
#22797=VERTEX_POINT('',#97302) ;
#22798=VERTEX_POINT('',#97304) ;
#22799=VERTEX_POINT('',#97307) ;
#22800=VERTEX_POINT('',#97308) ;
#22801=VERTEX_POINT('',#97310) ;
#22802=VERTEX_POINT('',#97312) ;
#22803=VERTEX_POINT('',#97314) ;
#22804=VERTEX_POINT('',#97316) ;
#22805=VERTEX_POINT('',#97318) ;
#22806=VERTEX_POINT('',#97327) ;
#22807=VERTEX_POINT('',#97335) ;
#22808=VERTEX_POINT('',#97337) ;
#22809=VERTEX_POINT('',#97361) ;
#22810=VERTEX_POINT('',#97369) ;
#22811=VERTEX_POINT('',#97370) ;
#22812=VERTEX_POINT('',#97390) ;
#22813=VERTEX_POINT('',#97394) ;
#22814=VERTEX_POINT('',#97406) ;
#22815=VERTEX_POINT('',#97408) ;
#22816=VERTEX_POINT('',#97412) ;
#22817=VERTEX_POINT('',#97425) ;
#22818=VERTEX_POINT('',#97453) ;
#22819=VERTEX_POINT('',#97457) ;
#22820=VERTEX_POINT('',#97459) ;
#22821=VERTEX_POINT('',#97461) ;
#22822=VERTEX_POINT('',#97463) ;
#22823=VERTEX_POINT('',#97465) ;
#22824=VERTEX_POINT('',#97471) ;
#22825=VERTEX_POINT('',#97475) ;
#22826=VERTEX_POINT('',#97479) ;
#22827=VERTEX_POINT('',#97483) ;
#22828=VERTEX_POINT('',#97487) ;
#22829=VERTEX_POINT('',#97491) ;
#22830=VERTEX_POINT('',#97495) ;
#22831=VERTEX_POINT('',#97499) ;
#22832=VERTEX_POINT('',#97503) ;
#22833=VERTEX_POINT('',#97510) ;
#22834=VERTEX_POINT('',#97512) ;
#22835=VERTEX_POINT('',#97516) ;
#22836=VERTEX_POINT('',#97520) ;
#22837=VERTEX_POINT('',#97528) ;
#22838=VERTEX_POINT('',#97530) ;
#22839=VERTEX_POINT('',#97534) ;
#22840=VERTEX_POINT('',#97536) ;
#22841=VERTEX_POINT('',#97545) ;
#22842=VERTEX_POINT('',#97558) ;
#22843=VERTEX_POINT('',#97572) ;
#22844=VERTEX_POINT('',#97589) ;
#22845=VERTEX_POINT('',#97593) ;
#22846=VERTEX_POINT('',#97595) ;
#22847=VERTEX_POINT('',#97599) ;
#22848=VERTEX_POINT('',#97718) ;
#22849=VERTEX_POINT('',#97719) ;
#22850=VERTEX_POINT('',#97731) ;
#22851=VERTEX_POINT('',#97738) ;
#22852=VERTEX_POINT('',#97761) ;
#22853=VERTEX_POINT('',#97767) ;
#22854=VERTEX_POINT('',#97768) ;
#22855=VERTEX_POINT('',#97807) ;
#22856=VERTEX_POINT('',#97809) ;
#22857=VERTEX_POINT('',#97816) ;
#22858=VERTEX_POINT('',#97817) ;
#22859=VERTEX_POINT('',#97889) ;
#22860=VERTEX_POINT('',#97890) ;
#22861=VERTEX_POINT('',#97898) ;
#22862=VERTEX_POINT('',#97923) ;
#22863=VERTEX_POINT('',#97925) ;
#22864=VERTEX_POINT('',#97932) ;
#22865=VERTEX_POINT('',#97933) ;
#22866=VERTEX_POINT('',#97986) ;
#22867=VERTEX_POINT('',#97988) ;
#22868=VERTEX_POINT('',#98006) ;
#22869=VERTEX_POINT('',#98008) ;
#22870=VERTEX_POINT('',#98014) ;
#22871=VERTEX_POINT('',#98015) ;
#22872=VERTEX_POINT('',#98017) ;
#22873=VERTEX_POINT('',#98019) ;
#22874=VERTEX_POINT('',#98074) ;
#22875=VERTEX_POINT('',#98075) ;
#22876=VERTEX_POINT('',#98080) ;
#22877=VERTEX_POINT('',#98081) ;
#22878=VERTEX_POINT('',#98086) ;
#22879=VERTEX_POINT('',#98088) ;
#22880=VERTEX_POINT('',#98111) ;
#22881=VERTEX_POINT('',#98112) ;
#22882=VERTEX_POINT('',#98139) ;
#22883=VERTEX_POINT('',#98141) ;
#22884=VERTEX_POINT('',#98145) ;
#22885=VERTEX_POINT('',#98149) ;
#22886=VERTEX_POINT('',#98153) ;
#22887=VERTEX_POINT('',#98157) ;
#22888=VERTEX_POINT('',#98161) ;
#22889=VERTEX_POINT('',#98165) ;
#22890=VERTEX_POINT('',#98169) ;
#22891=VERTEX_POINT('',#98173) ;
#22892=VERTEX_POINT('',#98188) ;
#22893=VERTEX_POINT('',#98197) ;
#22894=VERTEX_POINT('',#98222) ;
#22895=VERTEX_POINT('',#98226) ;
#22896=VERTEX_POINT('',#98230) ;
#22897=VERTEX_POINT('',#98232) ;
#22898=VERTEX_POINT('',#98236) ;
#22899=VERTEX_POINT('',#98240) ;
#22900=VERTEX_POINT('',#98244) ;
#22901=VERTEX_POINT('',#98248) ;
#22902=VERTEX_POINT('',#98252) ;
#22903=VERTEX_POINT('',#98253) ;
#22904=VERTEX_POINT('',#98258) ;
#22905=VERTEX_POINT('',#98262) ;
#22906=VERTEX_POINT('',#98266) ;
#22907=VERTEX_POINT('',#98270) ;
#22908=VERTEX_POINT('',#98274) ;
#22909=VERTEX_POINT('',#98278) ;
#22910=VERTEX_POINT('',#98282) ;
#22911=VERTEX_POINT('',#98286) ;
#22912=VERTEX_POINT('',#98287) ;
#22913=VERTEX_POINT('',#98292) ;
#22914=VERTEX_POINT('',#98296) ;
#22915=VERTEX_POINT('',#98300) ;
#22916=VERTEX_POINT('',#98304) ;
#22917=VERTEX_POINT('',#98319) ;
#22918=VERTEX_POINT('',#98328) ;
#22919=VERTEX_POINT('',#98329) ;
#22920=VERTEX_POINT('',#98334) ;
#22921=VERTEX_POINT('',#98338) ;
#22922=VERTEX_POINT('',#98342) ;
#22923=VERTEX_POINT('',#98348) ;
#22924=VERTEX_POINT('',#98352) ;
#22925=VERTEX_POINT('',#98353) ;
#22926=VERTEX_POINT('',#98358) ;
#22927=VERTEX_POINT('',#98363) ;
#22928=VERTEX_POINT('',#98367) ;
#22929=VERTEX_POINT('',#98373) ;
#22930=VERTEX_POINT('',#98374) ;
#22931=VERTEX_POINT('',#98379) ;
#22932=VERTEX_POINT('',#98383) ;
#22933=VERTEX_POINT('',#98387) ;
#22934=VERTEX_POINT('',#98391) ;
#22935=VERTEX_POINT('',#98395) ;
#22936=VERTEX_POINT('',#98399) ;
#22937=VERTEX_POINT('',#98403) ;
#22938=VERTEX_POINT('',#98407) ;
#22939=VERTEX_POINT('',#98411) ;
#22940=VERTEX_POINT('',#98415) ;
#22941=VERTEX_POINT('',#98419) ;
#22942=VERTEX_POINT('',#98423) ;
#22943=VERTEX_POINT('',#98430) ;
#22944=VERTEX_POINT('',#98445) ;
#22945=VERTEX_POINT('',#98454) ;
#22946=VERTEX_POINT('',#98458) ;
#22947=VERTEX_POINT('',#98462) ;
#22948=VERTEX_POINT('',#98480) ;
#22949=VERTEX_POINT('',#98489) ;
#22950=VERTEX_POINT('',#98493) ;
#22951=VERTEX_POINT('',#98497) ;
#22952=VERTEX_POINT('',#98501) ;
#22953=VERTEX_POINT('',#98505) ;
#22954=VERTEX_POINT('',#98512) ;
#22955=VERTEX_POINT('',#98516) ;
#22956=VERTEX_POINT('',#98520) ;
#22957=VERTEX_POINT('',#98524) ;
#22958=VERTEX_POINT('',#98528) ;
#22959=VERTEX_POINT('',#98532) ;
#22960=VERTEX_POINT('',#98536) ;
#22961=VERTEX_POINT('',#98540) ;
#22962=VERTEX_POINT('',#98544) ;
#22963=VERTEX_POINT('',#98548) ;
#22964=VERTEX_POINT('',#98552) ;
#22965=VERTEX_POINT('',#98556) ;
#22966=VERTEX_POINT('',#98560) ;
#22967=VERTEX_POINT('',#98564) ;
#22968=VERTEX_POINT('',#98571) ;
#22969=VERTEX_POINT('',#98575) ;
#22970=VERTEX_POINT('',#98579) ;
#22971=VERTEX_POINT('',#98583) ;
#22972=VERTEX_POINT('',#98587) ;
#22973=VERTEX_POINT('',#98595) ;
#22974=VERTEX_POINT('',#98599) ;
#22975=VERTEX_POINT('',#98627) ;
#27513=EDGE_CURVE('',#21716,#21717,#1149,.T.) ;
#27514=EDGE_CURVE('',#21716,#21718,#1150,.T.) ;
#27515=EDGE_CURVE('',#21718,#21719,#1151,.T.) ;
#27516=EDGE_CURVE('',#21717,#21719,#18545,.T.) ;
#27517=EDGE_CURVE('',#21716,#21720,#1152,.T.) ;
#27518=EDGE_CURVE('',#21721,#21720,#18546,.T.) ;
#27519=EDGE_CURVE('',#21721,#21718,#1153,.T.) ;
#27520=EDGE_CURVE('',#21716,#21722,#1154,.T.) ;
#27521=EDGE_CURVE('',#21722,#21723,#1155,.T.) ;
#27522=EDGE_CURVE('',#21723,#21724,#1156,.T.) ;
#27523=EDGE_CURVE('',#21720,#21724,#18547,.T.) ;
#27524=EDGE_CURVE('',#21716,#21725,#1157,.T.) ;
#27525=EDGE_CURVE('',#21726,#21725,#18548,.T.) ;
#27526=EDGE_CURVE('',#21726,#21722,#1158,.T.) ;
#27527=EDGE_CURVE('',#21716,#21727,#1159,.T.) ;
#27528=EDGE_CURVE('',#21727,#21728,#1160,.T.) ;
#27529=EDGE_CURVE('',#21725,#21728,#18549,.T.) ;
#27530=EDGE_CURVE('',#21729,#21730,#4592,.T.) ;
#27531=EDGE_CURVE('',#21729,#21731,#4593,.T.) ;
#27532=EDGE_CURVE('',#21731,#21732,#4594,.T.) ;
#27533=EDGE_CURVE('',#21730,#21732,#4595,.T.) ;
#27534=EDGE_CURVE('',#21733,#21729,#1161,.T.) ;
#27535=EDGE_CURVE('',#21733,#21734,#4596,.T.) ;
#27536=EDGE_CURVE('',#21734,#21731,#1162,.T.) ;
#27537=EDGE_CURVE('',#21735,#21733,#1163,.T.) ;
#27538=EDGE_CURVE('',#21735,#21736,#4597,.T.) ;
#27539=EDGE_CURVE('',#21736,#21734,#1164,.T.) ;
#27540=EDGE_CURVE('',#21737,#21735,#1165,.T.) ;
#27541=EDGE_CURVE('',#21737,#21738,#4598,.T.) ;
#27542=EDGE_CURVE('',#21738,#21736,#1166,.T.) ;
#27543=EDGE_CURVE('',#21739,#21737,#1167,.T.) ;
#27544=EDGE_CURVE('',#21739,#21740,#4599,.T.) ;
#27545=EDGE_CURVE('',#21740,#21738,#1168,.T.) ;
#27546=EDGE_CURVE('',#21741,#21739,#1169,.T.) ;
#27547=EDGE_CURVE('',#21741,#21742,#4600,.T.) ;
#27548=EDGE_CURVE('',#21742,#21740,#1170,.T.) ;
#27549=EDGE_CURVE('',#21743,#21741,#4601,.T.) ;
#27550=EDGE_CURVE('',#21743,#21744,#4602,.T.) ;
#27551=EDGE_CURVE('',#21744,#21742,#4603,.T.) ;
#27552=EDGE_CURVE('',#21730,#21743,#4604,.T.) ;
#27553=EDGE_CURVE('',#21732,#21744,#4605,.T.) ;
#27554=EDGE_CURVE('',#21745,#21746,#4606,.T.) ;
#27555=EDGE_CURVE('',#21745,#21747,#4607,.T.) ;
#27556=EDGE_CURVE('',#21747,#21748,#4608,.T.) ;
#27557=EDGE_CURVE('',#21746,#21748,#4609,.T.) ;
#27558=EDGE_CURVE('',#21749,#21745,#4610,.T.) ;
#27559=EDGE_CURVE('',#21749,#21750,#4611,.T.) ;
#27560=EDGE_CURVE('',#21750,#21747,#4612,.T.) ;
#27561=EDGE_CURVE('',#21751,#21749,#1171,.T.) ;
#27562=EDGE_CURVE('',#21751,#21752,#4613,.T.) ;
#27563=EDGE_CURVE('',#21752,#21750,#1172,.T.) ;
#27564=EDGE_CURVE('',#21753,#21751,#1173,.T.) ;
#27565=EDGE_CURVE('',#21753,#21754,#4614,.T.) ;
#27566=EDGE_CURVE('',#21754,#21752,#1174,.T.) ;
#27567=EDGE_CURVE('',#21755,#21753,#1175,.T.) ;
#27568=EDGE_CURVE('',#21755,#21756,#4615,.T.) ;
#27569=EDGE_CURVE('',#21756,#21754,#1176,.T.) ;
#27570=EDGE_CURVE('',#21757,#21755,#1177,.T.) ;
#27571=EDGE_CURVE('',#21757,#21758,#4616,.T.) ;
#27572=EDGE_CURVE('',#21758,#21756,#1178,.T.) ;
#27573=EDGE_CURVE('',#21759,#21757,#4617,.T.) ;
#27574=EDGE_CURVE('',#21759,#21760,#4618,.T.) ;
#27575=EDGE_CURVE('',#21760,#21758,#4619,.T.) ;
#27576=EDGE_CURVE('',#21761,#21759,#4620,.T.) ;
#27577=EDGE_CURVE('',#21761,#21762,#4621,.T.) ;
#27578=EDGE_CURVE('',#21762,#21760,#4622,.T.) ;
#27579=EDGE_CURVE('',#21763,#21761,#4623,.T.) ;
#27580=EDGE_CURVE('',#21763,#21764,#4624,.T.) ;
#27581=EDGE_CURVE('',#21764,#21762,#4625,.T.) ;
#27582=EDGE_CURVE('',#21765,#21763,#1179,.T.) ;
#27583=EDGE_CURVE('',#21765,#21766,#4626,.T.) ;
#27584=EDGE_CURVE('',#21766,#21764,#1180,.T.) ;
#27585=EDGE_CURVE('',#21767,#21765,#1181,.T.) ;
#27586=EDGE_CURVE('',#21767,#21768,#4627,.T.) ;
#27587=EDGE_CURVE('',#21768,#21766,#1182,.T.) ;
#27588=EDGE_CURVE('',#21769,#21767,#1183,.T.) ;
#27589=EDGE_CURVE('',#21769,#21770,#4628,.T.) ;
#27590=EDGE_CURVE('',#21770,#21768,#1184,.T.) ;
#27591=EDGE_CURVE('',#21771,#21769,#1185,.T.) ;
#27592=EDGE_CURVE('',#21771,#21772,#4629,.T.) ;
#27593=EDGE_CURVE('',#21772,#21770,#1186,.T.) ;
#27594=EDGE_CURVE('',#21773,#21771,#1187,.T.) ;
#27595=EDGE_CURVE('',#21773,#21774,#4630,.T.) ;
#27596=EDGE_CURVE('',#21774,#21772,#1188,.T.) ;
#27597=EDGE_CURVE('',#21775,#21773,#1189,.T.) ;
#27598=EDGE_CURVE('',#21775,#21776,#4631,.T.) ;
#27599=EDGE_CURVE('',#21776,#21774,#1190,.T.) ;
#27600=EDGE_CURVE('',#21777,#21775,#1191,.T.) ;
#27601=EDGE_CURVE('',#21777,#21778,#4632,.T.) ;
#27602=EDGE_CURVE('',#21778,#21776,#1192,.T.) ;
#27603=EDGE_CURVE('',#21779,#21777,#4633,.T.) ;
#27604=EDGE_CURVE('',#21779,#21780,#4634,.T.) ;
#27605=EDGE_CURVE('',#21780,#21778,#4635,.T.) ;
#27606=EDGE_CURVE('',#21781,#21779,#4636,.T.) ;
#27607=EDGE_CURVE('',#21781,#21782,#4637,.T.) ;
#27608=EDGE_CURVE('',#21782,#21780,#4638,.T.) ;
#27609=EDGE_CURVE('',#21746,#21781,#4639,.T.) ;
#27610=EDGE_CURVE('',#21748,#21782,#4640,.T.) ;
#27611=EDGE_CURVE('',#21783,#21784,#4641,.T.) ;
#27612=EDGE_CURVE('',#21785,#21783,#4642,.T.) ;
#27613=EDGE_CURVE('',#21785,#21786,#18550,.T.) ;
#27614=EDGE_CURVE('',#21787,#21786,#4643,.T.) ;
#27615=EDGE_CURVE('',#21788,#21787,#18551,.T.) ;
#27616=EDGE_CURVE('',#21789,#21788,#4644,.T.) ;
#27617=EDGE_CURVE('',#21790,#21789,#18552,.T.) ;
#27618=EDGE_CURVE('',#21791,#21790,#4645,.T.) ;
#27619=EDGE_CURVE('',#21792,#21791,#18553,.T.) ;
#27620=EDGE_CURVE('',#21793,#21792,#18554,.T.) ;
#27621=EDGE_CURVE('',#21794,#21793,#4646,.T.) ;
#27622=EDGE_CURVE('',#21795,#21794,#18555,.T.) ;
#27623=EDGE_CURVE('',#21796,#21795,#4647,.T.) ;
#27624=EDGE_CURVE('',#21797,#21796,#18556,.T.) ;
#27625=EDGE_CURVE('',#21798,#21797,#4648,.T.) ;
#27626=EDGE_CURVE('',#21799,#21798,#18557,.T.) ;
#27627=EDGE_CURVE('',#21800,#21799,#4649,.T.) ;
#27628=EDGE_CURVE('',#21784,#21800,#18558,.T.) ;
#27629=EDGE_CURVE('',#21801,#21802,#4650,.T.) ;
#27630=EDGE_CURVE('',#21803,#21801,#18559,.T.) ;
#27631=EDGE_CURVE('',#21804,#21803,#4651,.T.) ;
#27632=EDGE_CURVE('',#21802,#21804,#4652,.T.) ;
#27633=EDGE_CURVE('',#21805,#21806,#395,.T.) ;
#27634=EDGE_CURVE('',#21805,#21807,#4653,.T.) ;
#27635=EDGE_CURVE('',#21807,#21808,#396,.T.) ;
#27636=EDGE_CURVE('',#21808,#21806,#4654,.T.) ;
#27637=EDGE_CURVE('',#21808,#21809,#1193,.T.) ;
#27638=EDGE_CURVE('',#21809,#21810,#4655,.T.) ;
#27639=EDGE_CURVE('',#21810,#21806,#1194,.T.) ;
#27640=EDGE_CURVE('',#21811,#21812,#18560,.T.) ;
#27641=EDGE_CURVE('',#21812,#21813,#18561,.T.) ;
#27642=EDGE_CURVE('',#21813,#21814,#1195,.F.) ;
#27643=EDGE_CURVE('',#21814,#21811,#18562,.T.) ;
#27644=EDGE_CURVE('',#21815,#21816,#18563,.T.) ;
#27645=EDGE_CURVE('',#21816,#21812,#4656,.T.) ;
#27646=EDGE_CURVE('',#21811,#21815,#4657,.T.) ;
#27647=EDGE_CURVE('',#21817,#21818,#18564,.T.) ;
#27648=EDGE_CURVE('',#21818,#21816,#18565,.T.) ;
#27649=EDGE_CURVE('',#21815,#21817,#18566,.T.) ;
#27650=EDGE_CURVE('',#21819,#21820,#18567,.T.) ;
#27651=EDGE_CURVE('',#21820,#21821,#1196,.T.) ;
#27652=EDGE_CURVE('',#21821,#21818,#4658,.T.) ;
#27653=EDGE_CURVE('',#21817,#21819,#4659,.T.) ;
#27654=EDGE_CURVE('',#21822,#21823,#1197,.T.) ;
#27655=EDGE_CURVE('',#21824,#21822,#1198,.F.) ;
#27656=EDGE_CURVE('',#21820,#21824,#1199,.F.) ;
#27657=EDGE_CURVE('',#21819,#21823,#18568,.T.) ;
#27658=EDGE_CURVE('',#21825,#21817,#4660,.T.) ;
#27659=EDGE_CURVE('',#21826,#21825,#4661,.T.) ;
#27660=EDGE_CURVE('',#21827,#21826,#4662,.T.) ;
#27661=EDGE_CURVE('',#21828,#21827,#4663,.T.) ;
#27662=EDGE_CURVE('',#21828,#21823,#4664,.T.) ;
#27663=EDGE_CURVE('',#21815,#21829,#4665,.T.) ;
#27664=EDGE_CURVE('',#21829,#21825,#18569,.T.) ;
#27665=EDGE_CURVE('',#21830,#21814,#4666,.F.) ;
#27666=EDGE_CURVE('',#21829,#21830,#4667,.F.) ;
#27667=EDGE_CURVE('',#21831,#21832,#1200,.T.) ;
#27668=EDGE_CURVE('',#21831,#21833,#397,.T.) ;
#27669=EDGE_CURVE('',#21833,#21834,#18570,.T.) ;
#27670=EDGE_CURVE('',#21834,#21835,#398,.T.) ;
#27671=EDGE_CURVE('',#21835,#21836,#1201,.T.) ;
#27672=EDGE_CURVE('',#21836,#21837,#1202,.T.) ;
#27673=EDGE_CURVE('',#21837,#21832,#1203,.T.) ;
#27674=EDGE_CURVE('',#21838,#21839,#18571,.T.) ;
#27675=EDGE_CURVE('',#21839,#21834,#4668,.T.) ;
#27676=EDGE_CURVE('',#21833,#21838,#4669,.T.) ;
#27677=EDGE_CURVE('',#21840,#21841,#18572,.T.) ;
#27678=EDGE_CURVE('',#21841,#21839,#18573,.T.) ;
#27679=EDGE_CURVE('',#21838,#21840,#18574,.T.) ;
#27680=EDGE_CURVE('',#21842,#21843,#18575,.T.) ;
#27681=EDGE_CURVE('',#21843,#21841,#4670,.T.) ;
#27682=EDGE_CURVE('',#21840,#21842,#4671,.T.) ;
#27683=EDGE_CURVE('',#21844,#21845,#1204,.F.) ;
#27684=EDGE_CURVE('',#21845,#21843,#18576,.T.) ;
#27685=EDGE_CURVE('',#21842,#21844,#18577,.T.) ;
#27686=EDGE_CURVE('',#21846,#21840,#4672,.T.) ;
#27687=EDGE_CURVE('',#21847,#21846,#4673,.F.) ;
#27688=EDGE_CURVE('',#21844,#21847,#4674,.F.) ;
#27689=EDGE_CURVE('',#21838,#21848,#4675,.T.) ;
#27690=EDGE_CURVE('',#21848,#21846,#18578,.T.) ;
#27691=EDGE_CURVE('',#21849,#21831,#4676,.T.) ;
#27692=EDGE_CURVE('',#21848,#21849,#4677,.T.) ;
#27693=EDGE_CURVE('',#21832,#21850,#4678,.T.) ;
#27694=EDGE_CURVE('',#21851,#21850,#1205,.T.) ;
#27695=EDGE_CURVE('',#21851,#21852,#1206,.T.) ;
#27696=EDGE_CURVE('',#21852,#21832,#399,.F.) ;
#27697=EDGE_CURVE('',#21837,#21850,#4679,.T.) ;
#27698=EDGE_CURVE('',#21853,#21836,#1207,.T.) ;
#27699=EDGE_CURVE('',#21853,#21854,#1208,.T.) ;
#27700=EDGE_CURVE('',#21855,#21854,#400,.T.) ;
#27701=EDGE_CURVE('',#21856,#21855,#4680,.T.) ;
#27702=EDGE_CURVE('',#21857,#21856,#1209,.T.) ;
#27703=EDGE_CURVE('',#21858,#21857,#401,.T.) ;
#27704=EDGE_CURVE('',#21859,#21858,#4681,.T.) ;
#27705=EDGE_CURVE('',#21860,#21859,#4682,.T.) ;
#27706=EDGE_CURVE('',#21861,#21860,#4683,.T.) ;
#27707=EDGE_CURVE('',#21862,#21861,#4684,.T.) ;
#27708=EDGE_CURVE('',#21863,#21862,#402,.T.) ;
#27709=EDGE_CURVE('',#21864,#21863,#4685,.T.) ;
#27710=EDGE_CURVE('',#21865,#21864,#403,.T.) ;
#27711=EDGE_CURVE('',#21851,#21865,#4686,.T.) ;
#27712=EDGE_CURVE('',#21866,#21867,#18579,.T.) ;
#27713=EDGE_CURVE('',#21867,#21868,#404,.T.) ;
#27714=EDGE_CURVE('',#21868,#21869,#405,.T.) ;
#27715=EDGE_CURVE('',#21869,#21870,#406,.T.) ;
#27716=EDGE_CURVE('',#21870,#21866,#407,.T.) ;
#27717=EDGE_CURVE('',#21871,#21872,#18580,.T.) ;
#27718=EDGE_CURVE('',#21872,#21867,#4687,.T.) ;
#27719=EDGE_CURVE('',#21866,#21871,#4688,.T.) ;
#27720=EDGE_CURVE('',#21873,#21874,#18581,.T.) ;
#27721=EDGE_CURVE('',#21874,#21872,#408,.T.) ;
#27722=EDGE_CURVE('',#21871,#21873,#409,.T.) ;
#27723=EDGE_CURVE('',#21873,#21875,#1210,.T.) ;
#27724=EDGE_CURVE('',#21875,#21874,#1211,.T.) ;
#27725=EDGE_CURVE('',#21871,#21876,#4689,.T.) ;
#27726=EDGE_CURVE('',#21876,#21877,#18582,.T.) ;
#27727=EDGE_CURVE('',#21877,#21875,#4690,.T.) ;
#27728=EDGE_CURVE('',#21878,#21866,#4691,.T.) ;
#27729=EDGE_CURVE('',#21879,#21878,#4692,.T.) ;
#27730=EDGE_CURVE('',#21876,#21879,#18583,.T.) ;
#27731=EDGE_CURVE('',#21869,#21880,#4693,.T.) ;
#27732=EDGE_CURVE('',#21878,#21880,#18584,.T.) ;
#27733=EDGE_CURVE('',#21881,#21882,#18585,.T.) ;
#27734=EDGE_CURVE('',#21882,#21883,#410,.T.) ;
#27735=EDGE_CURVE('',#21883,#21884,#411,.T.) ;
#27736=EDGE_CURVE('',#21884,#21885,#412,.T.) ;
#27737=EDGE_CURVE('',#21885,#21881,#413,.T.) ;
#27738=EDGE_CURVE('',#21886,#21887,#18586,.T.) ;
#27739=EDGE_CURVE('',#21887,#21882,#4694,.T.) ;
#27740=EDGE_CURVE('',#21881,#21886,#4695,.T.) ;
#27741=EDGE_CURVE('',#21888,#21889,#18587,.T.) ;
#27742=EDGE_CURVE('',#21889,#21887,#414,.T.) ;
#27743=EDGE_CURVE('',#21886,#21888,#415,.T.) ;
#27744=EDGE_CURVE('',#21888,#21890,#1212,.T.) ;
#27745=EDGE_CURVE('',#21890,#21860,#1213,.T.) ;
#27746=EDGE_CURVE('',#21860,#21891,#1214,.T.) ;
#27747=EDGE_CURVE('',#21891,#21889,#1215,.T.) ;
#27748=EDGE_CURVE('',#21892,#21874,#4696,.T.) ;
#27749=EDGE_CURVE('',#21893,#21892,#4697,.T.) ;
#27750=EDGE_CURVE('',#21894,#21893,#18588,.T.) ;
#27751=EDGE_CURVE('',#21895,#21894,#4698,.T.) ;
#27752=EDGE_CURVE('',#21896,#21895,#18589,.T.) ;
#27753=EDGE_CURVE('',#21897,#21896,#4699,.T.) ;
#27754=EDGE_CURVE('',#21888,#21897,#4700,.T.) ;
#27755=EDGE_CURVE('',#21898,#21881,#4701,.T.) ;
#27756=EDGE_CURVE('',#21899,#21898,#4702,.T.) ;
#27757=EDGE_CURVE('',#21900,#21899,#18590,.T.) ;
#27758=EDGE_CURVE('',#21901,#21900,#4703,.T.) ;
#27759=EDGE_CURVE('',#21867,#21901,#4704,.T.) ;
#27760=EDGE_CURVE('',#21884,#21902,#4705,.T.) ;
#27761=EDGE_CURVE('',#21902,#21898,#416,.T.) ;
#27762=EDGE_CURVE('',#21882,#21903,#4706,.T.) ;
#27763=EDGE_CURVE('',#21904,#21903,#18591,.T.) ;
#27764=EDGE_CURVE('',#21904,#21884,#4707,.T.) ;
#27765=EDGE_CURVE('',#21905,#21906,#417,.T.) ;
#27766=EDGE_CURVE('',#21906,#21907,#418,.T.) ;
#27767=EDGE_CURVE('',#21907,#21905,#18592,.T.) ;
#27768=EDGE_CURVE('',#21906,#21908,#4708,.T.) ;
#27769=EDGE_CURVE('',#21908,#21909,#18593,.T.) ;
#27770=EDGE_CURVE('',#21909,#21907,#4709,.T.) ;
#27771=EDGE_CURVE('',#21905,#21910,#4710,.T.) ;
#27772=EDGE_CURVE('',#21910,#21911,#1216,.T.) ;
#27773=EDGE_CURVE('',#21911,#21912,#4711,.T.) ;
#27774=EDGE_CURVE('',#21912,#21913,#18594,.T.) ;
#27775=EDGE_CURVE('',#21913,#21906,#4712,.T.) ;
#27776=EDGE_CURVE('',#21908,#21914,#4713,.T.) ;
#27777=EDGE_CURVE('',#21915,#21914,#4714,.T.) ;
#27778=EDGE_CURVE('',#21916,#21915,#4715,.T.) ;
#27779=EDGE_CURVE('',#21917,#21916,#4716,.T.) ;
#27780=EDGE_CURVE('',#21918,#21917,#419,.T.) ;
#27781=EDGE_CURVE('',#21919,#21918,#4717,.T.) ;
#27782=EDGE_CURVE('',#21920,#21919,#420,.T.) ;
#27783=EDGE_CURVE('',#21909,#21920,#4718,.T.) ;
#27784=EDGE_CURVE('',#21914,#21913,#4719,.T.) ;
#27785=EDGE_CURVE('',#21912,#21921,#18595,.T.) ;
#27786=EDGE_CURVE('',#21915,#21921,#4720,.T.) ;
#27787=EDGE_CURVE('',#21911,#21922,#18596,.T.) ;
#27788=EDGE_CURVE('',#21922,#21921,#4721,.T.) ;
#27789=EDGE_CURVE('',#21812,#21923,#4722,.T.) ;
#27790=EDGE_CURVE('',#21924,#21923,#421,.T.) ;
#27791=EDGE_CURVE('',#21924,#21813,#4723,.T.) ;
#27792=EDGE_CURVE('',#21925,#21821,#1217,.F.) ;
#27793=EDGE_CURVE('',#21923,#21925,#4724,.T.) ;
#27794=EDGE_CURVE('',#21926,#21927,#18597,.T.) ;
#27795=EDGE_CURVE('',#21927,#21928,#422,.T.) ;
#27796=EDGE_CURVE('',#21928,#21929,#18598,.T.) ;
#27797=EDGE_CURVE('',#21929,#21926,#423,.T.) ;
#27798=EDGE_CURVE('',#21845,#21928,#4725,.T.) ;
#27799=EDGE_CURVE('',#21927,#21843,#4726,.T.) ;
#27800=EDGE_CURVE('',#21930,#21929,#4727,.T.) ;
#27801=EDGE_CURVE('',#21931,#21930,#424,.T.) ;
#27802=EDGE_CURVE('',#21932,#21931,#4728,.T.) ;
#27803=EDGE_CURVE('',#21926,#21932,#4729,.T.) ;
#27804=EDGE_CURVE('',#21928,#21933,#4730,.T.) ;
#27805=EDGE_CURVE('',#21933,#21930,#18599,.T.) ;
#27806=EDGE_CURVE('',#21847,#21934,#4731,.T.) ;
#27807=EDGE_CURVE('',#21934,#21935,#4732,.T.) ;
#27808=EDGE_CURVE('',#21935,#21936,#4733,.T.) ;
#27809=EDGE_CURVE('',#21937,#21936,#4734,.T.) ;
#27810=EDGE_CURVE('',#21933,#21937,#4735,.T.) ;
#27811=EDGE_CURVE('',#21938,#21892,#18600,.T.) ;
#27812=EDGE_CURVE('',#21892,#21939,#18601,.T.) ;
#27813=EDGE_CURVE('',#21939,#21940,#18602,.T.) ;
#27814=EDGE_CURVE('',#21940,#21938,#18603,.T.) ;
#27815=EDGE_CURVE('',#21875,#21939,#4736,.T.) ;
#27816=EDGE_CURVE('',#21939,#21941,#4737,.T.) ;
#27817=EDGE_CURVE('',#21942,#21941,#18604,.T.) ;
#27818=EDGE_CURVE('',#21942,#21940,#4738,.T.) ;
#27819=EDGE_CURVE('',#21943,#21877,#4739,.T.) ;
#27820=EDGE_CURVE('',#21944,#21943,#4740,.T.) ;
#27821=EDGE_CURVE('',#21945,#21944,#4741,.T.) ;
#27822=EDGE_CURVE('',#21941,#21945,#425,.T.) ;
#27823=EDGE_CURVE('',#21897,#21946,#18605,.T.) ;
#27824=EDGE_CURVE('',#21946,#21947,#18606,.T.) ;
#27825=EDGE_CURVE('',#21947,#21861,#18607,.T.) ;
#27826=EDGE_CURVE('',#21861,#21897,#18608,.T.) ;
#27827=EDGE_CURVE('',#21896,#21948,#18609,.T.) ;
#27828=EDGE_CURVE('',#21948,#21946,#4742,.T.) ;
#27829=EDGE_CURVE('',#21880,#21949,#18610,.T.) ;
#27830=EDGE_CURVE('',#21949,#21950,#18611,.T.) ;
#27831=EDGE_CURVE('',#21950,#21878,#18612,.T.) ;
#27832=EDGE_CURVE('',#21879,#21951,#18613,.T.) ;
#27833=EDGE_CURVE('',#21951,#21877,#18614,.T.) ;
#27834=EDGE_CURVE('',#21950,#21951,#4743,.T.) ;
#27835=EDGE_CURVE('',#21903,#21952,#18615,.T.) ;
#27836=EDGE_CURVE('',#21952,#21953,#18616,.T.) ;
#27837=EDGE_CURVE('',#21953,#21904,#18617,.T.) ;
#27838=EDGE_CURVE('',#21954,#21955,#18618,.T.) ;
#27839=EDGE_CURVE('',#21955,#21952,#4744,.T.) ;
#27840=EDGE_CURVE('',#21903,#21954,#4745,.T.) ;
#27841=EDGE_CURVE('',#21956,#21859,#18619,.T.) ;
#27842=EDGE_CURVE('',#21859,#21955,#18620,.T.) ;
#27843=EDGE_CURVE('',#21954,#21956,#18621,.T.) ;
#27844=EDGE_CURVE('',#21956,#21887,#4746,.T.) ;
#27845=EDGE_CURVE('',#21957,#21953,#4747,.T.) ;
#27846=EDGE_CURVE('',#21958,#21957,#4748,.T.) ;
#27847=EDGE_CURVE('',#21958,#21959,#4749,.T.) ;
#27848=EDGE_CURVE('',#21959,#21960,#4750,.T.) ;
#27849=EDGE_CURVE('',#21961,#21960,#4751,.T.) ;
#27850=EDGE_CURVE('',#21961,#21902,#4752,.T.) ;
#27851=EDGE_CURVE('',#21952,#21962,#4753,.T.) ;
#27852=EDGE_CURVE('',#21957,#21962,#18622,.T.) ;
#27853=EDGE_CURVE('',#21963,#21955,#4754,.T.) ;
#27854=EDGE_CURVE('',#21964,#21963,#426,.T.) ;
#27855=EDGE_CURVE('',#21965,#21964,#4755,.T.) ;
#27856=EDGE_CURVE('',#21966,#21965,#4756,.T.) ;
#27857=EDGE_CURVE('',#21967,#21966,#4757,.T.) ;
#27858=EDGE_CURVE('',#21962,#21967,#18623,.T.) ;
#27859=EDGE_CURVE('',#21968,#21858,#1218,.T.) ;
#27860=EDGE_CURVE('',#21963,#21968,#1219,.T.) ;
#27861=EDGE_CURVE('',#21969,#21970,#18624,.F.) ;
#27862=EDGE_CURVE('',#21971,#21969,#18625,.F.) ;
#27863=EDGE_CURVE('',#21970,#21971,#18626,.F.) ;
#27864=EDGE_CURVE('',#21972,#21973,#427,.T.) ;
#27865=EDGE_CURVE('',#21973,#21971,#4758,.T.) ;
#27866=EDGE_CURVE('',#21969,#21972,#4759,.T.) ;
#27867=EDGE_CURVE('',#21974,#21975,#1220,.T.) ;
#27868=EDGE_CURVE('',#21975,#21976,#18627,.T.) ;
#27869=EDGE_CURVE('',#21976,#21977,#18628,.T.) ;
#27870=EDGE_CURVE('',#21977,#21974,#18629,.T.) ;
#27871=EDGE_CURVE('',#21978,#21979,#18630,.T.) ;
#27872=EDGE_CURVE('',#21979,#21977,#4760,.T.) ;
#27873=EDGE_CURVE('',#21976,#21978,#4761,.T.) ;
#27874=EDGE_CURVE('',#21980,#21981,#18631,.T.) ;
#27875=EDGE_CURVE('',#21981,#21979,#18632,.T.) ;
#27876=EDGE_CURVE('',#21978,#21980,#18633,.T.) ;
#27877=EDGE_CURVE('',#21982,#21983,#18634,.T.) ;
#27878=EDGE_CURVE('',#21983,#21981,#18635,.T.) ;
#27879=EDGE_CURVE('',#21980,#21982,#18636,.T.) ;
#27880=EDGE_CURVE('',#21984,#21985,#18637,.T.) ;
#27881=EDGE_CURVE('',#21985,#21983,#4762,.T.) ;
#27882=EDGE_CURVE('',#21982,#21984,#4763,.T.) ;
#27883=EDGE_CURVE('',#21986,#21987,#18638,.T.) ;
#27884=EDGE_CURVE('',#21987,#21985,#18639,.T.) ;
#27885=EDGE_CURVE('',#21984,#21986,#18640,.T.) ;
#27886=EDGE_CURVE('',#21971,#21987,#4764,.T.) ;
#27887=EDGE_CURVE('',#21986,#21970,#4765,.T.) ;
#27888=EDGE_CURVE('',#21988,#21989,#18641,.T.) ;
#27889=EDGE_CURVE('',#21989,#21969,#4766,.T.) ;
#27890=EDGE_CURVE('',#21970,#21988,#4767,.T.) ;
#27891=EDGE_CURVE('',#21990,#21991,#1221,.F.) ;
#27892=EDGE_CURVE('',#21991,#21989,#18642,.T.) ;
#27893=EDGE_CURVE('',#21988,#21990,#18643,.T.) ;
#27894=EDGE_CURVE('',#21992,#21973,#4768,.T.) ;
#27895=EDGE_CURVE('',#21992,#21993,#18644,.T.) ;
#27896=EDGE_CURVE('',#21994,#21993,#4769,.T.) ;
#27897=EDGE_CURVE('',#21994,#21995,#18645,.T.) ;
#27898=EDGE_CURVE('',#21996,#21995,#4770,.T.) ;
#27899=EDGE_CURVE('',#21997,#21996,#4771,.T.) ;
#27900=EDGE_CURVE('',#21997,#21998,#4772,.T.) ;
#27901=EDGE_CURVE('',#21999,#21998,#18646,.T.) ;
#27902=EDGE_CURVE('',#21999,#22000,#18647,.F.) ;
#27903=EDGE_CURVE('',#21974,#22000,#18648,.T.) ;
#27904=EDGE_CURVE('',#21972,#22001,#4773,.T.) ;
#27905=EDGE_CURVE('',#22001,#21992,#18649,.T.) ;
#27906=EDGE_CURVE('',#22002,#21991,#4774,.T.) ;
#27907=EDGE_CURVE('',#21972,#22002,#4775,.T.) ;
#27908=EDGE_CURVE('',#22003,#22004,#18650,.T.) ;
#27909=EDGE_CURVE('',#22003,#22005,#4776,.T.) ;
#27910=EDGE_CURVE('',#22005,#22006,#18651,.T.) ;
#27911=EDGE_CURVE('',#22006,#22007,#4777,.T.) ;
#27912=EDGE_CURVE('',#22004,#22007,#428,.T.) ;
#27913=EDGE_CURVE('',#22008,#22009,#1222,.T.) ;
#27914=EDGE_CURVE('',#22009,#22006,#1223,.T.) ;
#27915=EDGE_CURVE('',#22005,#22008,#1224,.T.) ;
#27916=EDGE_CURVE('',#22010,#22003,#18652,.T.) ;
#27917=EDGE_CURVE('',#22011,#22010,#4778,.T.) ;
#27918=EDGE_CURVE('',#22011,#22008,#18653,.T.) ;
#27919=EDGE_CURVE('',#21988,#22012,#4779,.T.) ;
#27920=EDGE_CURVE('',#22012,#22013,#18654,.T.) ;
#27921=EDGE_CURVE('',#22013,#21990,#4780,.T.) ;
#27922=EDGE_CURVE('',#22012,#22014,#1225,.T.) ;
#27923=EDGE_CURVE('',#22014,#22015,#1226,.T.) ;
#27924=EDGE_CURVE('',#22015,#22013,#1227,.T.) ;
#27925=EDGE_CURVE('',#21986,#22016,#4781,.T.) ;
#27926=EDGE_CURVE('',#22017,#22016,#4782,.T.) ;
#27927=EDGE_CURVE('',#22014,#22017,#4783,.T.) ;
#27928=EDGE_CURVE('',#22018,#22019,#18655,.T.) ;
#27929=EDGE_CURVE('',#21966,#22019,#18656,.T.) ;
#27930=EDGE_CURVE('',#22020,#21966,#18657,.F.) ;
#27931=EDGE_CURVE('',#22018,#22020,#18658,.T.) ;
#27932=EDGE_CURVE('',#22021,#21967,#18659,.T.) ;
#27933=EDGE_CURVE('',#22019,#22021,#4784,.T.) ;
#27934=EDGE_CURVE('',#22021,#21957,#18660,.T.) ;
#27935=EDGE_CURVE('',#21965,#22022,#18661,.T.) ;
#27936=EDGE_CURVE('',#22022,#22020,#4785,.T.) ;
#27937=EDGE_CURVE('',#21965,#22023,#1228,.T.) ;
#27938=EDGE_CURVE('',#22023,#22024,#18662,.T.) ;
#27939=EDGE_CURVE('',#22024,#22022,#1229,.T.) ;
#27940=EDGE_CURVE('',#22025,#22026,#18663,.T.) ;
#27941=EDGE_CURVE('',#22026,#22024,#429,.T.) ;
#27942=EDGE_CURVE('',#22023,#22025,#430,.T.) ;
#27943=EDGE_CURVE('',#22027,#22028,#18664,.T.) ;
#27944=EDGE_CURVE('',#22028,#22026,#4786,.T.) ;
#27945=EDGE_CURVE('',#22025,#22027,#4787,.T.) ;
#27946=EDGE_CURVE('',#22029,#22030,#1230,.T.) ;
#27947=EDGE_CURVE('',#22030,#22028,#431,.T.) ;
#27948=EDGE_CURVE('',#22027,#22031,#432,.T.) ;
#27949=EDGE_CURVE('',#22031,#22029,#1231,.T.) ;
#27950=EDGE_CURVE('',#21798,#22032,#433,.T.) ;
#27951=EDGE_CURVE('',#22032,#22033,#18665,.T.) ;
#27952=EDGE_CURVE('',#22033,#21799,#18666,.T.) ;
#27953=EDGE_CURVE('',#22034,#21800,#18667,.T.) ;
#27954=EDGE_CURVE('',#22033,#22034,#4788,.T.) ;
#27955=EDGE_CURVE('',#22035,#21784,#18668,.T.) ;
#27956=EDGE_CURVE('',#22034,#22035,#18669,.T.) ;
#27957=EDGE_CURVE('',#22036,#21783,#18670,.T.) ;
#27958=EDGE_CURVE('',#22035,#22036,#4789,.T.) ;
#27959=EDGE_CURVE('',#22037,#22038,#18671,.T.) ;
#27960=EDGE_CURVE('',#22038,#21783,#18672,.T.) ;
#27961=EDGE_CURVE('',#22036,#22037,#18673,.T.) ;
#27962=EDGE_CURVE('',#22039,#22040,#18674,.T.) ;
#27963=EDGE_CURVE('',#22040,#22038,#4790,.T.) ;
#27964=EDGE_CURVE('',#22037,#22039,#4791,.T.) ;
#27965=EDGE_CURVE('',#22020,#22040,#18675,.T.) ;
#27966=EDGE_CURVE('',#22039,#22018,#18676,.T.) ;
#27967=EDGE_CURVE('',#22041,#22021,#4792,.T.) ;
#27968=EDGE_CURVE('',#21958,#22041,#18677,.T.) ;
#27969=EDGE_CURVE('',#22042,#22035,#4793,.T.) ;
#27970=EDGE_CURVE('',#22042,#22041,#4794,.T.) ;
#27971=EDGE_CURVE('',#22043,#22034,#4795,.T.) ;
#27972=EDGE_CURVE('',#22043,#22042,#18678,.T.) ;
#27973=EDGE_CURVE('',#22044,#22033,#4796,.T.) ;
#27974=EDGE_CURVE('',#22045,#22044,#4797,.T.) ;
#27975=EDGE_CURVE('',#22046,#22045,#4798,.T.) ;
#27976=EDGE_CURVE('',#22046,#22043,#4799,.T.) ;
#27977=EDGE_CURVE('',#22047,#22032,#4800,.T.) ;
#27978=EDGE_CURVE('',#22044,#22047,#18679,.T.) ;
#27979=EDGE_CURVE('',#22048,#21797,#18680,.T.) ;
#27980=EDGE_CURVE('',#22048,#22032,#4801,.T.) ;
#27981=EDGE_CURVE('',#22049,#22050,#18681,.T.) ;
#27982=EDGE_CURVE('',#22050,#22051,#1232,.T.) ;
#27983=EDGE_CURVE('',#22051,#22052,#1233,.T.) ;
#27984=EDGE_CURVE('',#22052,#22053,#1234,.T.) ;
#27985=EDGE_CURVE('',#22053,#22049,#1235,.T.) ;
#27986=EDGE_CURVE('',#22054,#22055,#18682,.T.) ;
#27987=EDGE_CURVE('',#22055,#22050,#434,.T.) ;
#27988=EDGE_CURVE('',#22049,#22054,#435,.T.) ;
#27989=EDGE_CURVE('',#22056,#22057,#18683,.T.) ;
#27990=EDGE_CURVE('',#22057,#22055,#4802,.T.) ;
#27991=EDGE_CURVE('',#22054,#22056,#4803,.T.) ;
#27992=EDGE_CURVE('',#22058,#22059,#18684,.T.) ;
#27993=EDGE_CURVE('',#22059,#22057,#436,.T.) ;
#27994=EDGE_CURVE('',#22056,#22058,#437,.T.) ;
#27995=EDGE_CURVE('',#22060,#22061,#18685,.T.) ;
#27996=EDGE_CURVE('',#22061,#22059,#438,.T.) ;
#27997=EDGE_CURVE('',#22058,#22060,#439,.T.) ;
#27998=EDGE_CURVE('',#22060,#22062,#440,.T.) ;
#27999=EDGE_CURVE('',#22062,#22063,#1236,.T.) ;
#28000=EDGE_CURVE('',#22063,#22061,#441,.T.) ;
#28001=EDGE_CURVE('',#22056,#22064,#4804,.T.) ;
#28002=EDGE_CURVE('',#22065,#22064,#1237,.T.) ;
#28003=EDGE_CURVE('',#22066,#22065,#442,.T.) ;
#28004=EDGE_CURVE('',#22066,#22062,#4805,.T.) ;
#28005=EDGE_CURVE('',#22067,#22059,#4806,.T.) ;
#28006=EDGE_CURVE('',#22068,#22067,#4807,.T.) ;
#28007=EDGE_CURVE('',#22068,#22069,#4808,.T.) ;
#28008=EDGE_CURVE('',#22070,#22069,#1238,.F.) ;
#28009=EDGE_CURVE('',#22071,#22070,#4809,.T.) ;
#28010=EDGE_CURVE('',#22050,#22071,#443,.T.) ;
#28011=EDGE_CURVE('',#22064,#22054,#4810,.T.) ;
#28012=EDGE_CURVE('',#22052,#22072,#4811,.T.) ;
#28013=EDGE_CURVE('',#22064,#22072,#18686,.T.) ;
#28014=EDGE_CURVE('',#21802,#22073,#444,.T.) ;
#28015=EDGE_CURVE('',#22073,#22074,#4812,.T.) ;
#28016=EDGE_CURVE('',#22074,#21801,#1239,.T.) ;
#28017=EDGE_CURVE('',#22074,#22075,#18687,.T.) ;
#28018=EDGE_CURVE('',#22075,#21803,#1240,.T.) ;
#28019=EDGE_CURVE('',#22075,#22076,#4813,.T.) ;
#28020=EDGE_CURVE('',#22076,#21804,#445,.T.) ;
#28021=EDGE_CURVE('',#22076,#22073,#4814,.T.) ;
#28022=EDGE_CURVE('',#22077,#22074,#4815,.T.) ;
#28023=EDGE_CURVE('',#22078,#22077,#18688,.T.) ;
#28024=EDGE_CURVE('',#22078,#22075,#4816,.T.) ;
#28025=EDGE_CURVE('',#22073,#22079,#4817,.T.) ;
#28026=EDGE_CURVE('',#22077,#22079,#4818,.T.) ;
#28027=EDGE_CURVE('',#22080,#22081,#18689,.T.) ;
#28028=EDGE_CURVE('',#22081,#22082,#446,.T.) ;
#28029=EDGE_CURVE('',#22082,#22080,#447,.T.) ;
#28030=EDGE_CURVE('',#22083,#22084,#18690,.T.) ;
#28031=EDGE_CURVE('',#22084,#22081,#18691,.T.) ;
#28032=EDGE_CURVE('',#22080,#22083,#18692,.T.) ;
#28033=EDGE_CURVE('',#22085,#22086,#1241,.T.) ;
#28034=EDGE_CURVE('',#22086,#22084,#4819,.T.) ;
#28035=EDGE_CURVE('',#22083,#22085,#4820,.T.) ;
#28036=EDGE_CURVE('',#22087,#22083,#4821,.T.) ;
#28037=EDGE_CURVE('',#22087,#22088,#4822,.T.) ;
#28038=EDGE_CURVE('',#22088,#22089,#4823,.T.) ;
#28039=EDGE_CURVE('',#22089,#22090,#4824,.T.) ;
#28040=EDGE_CURVE('',#22090,#22085,#4825,.T.) ;
#28041=EDGE_CURVE('',#22082,#22091,#4826,.T.) ;
#28042=EDGE_CURVE('',#22091,#22087,#18693,.T.) ;
#28043=EDGE_CURVE('',#22081,#22092,#4827,.T.) ;
#28044=EDGE_CURVE('',#22093,#22092,#18694,.T.) ;
#28045=EDGE_CURVE('',#22093,#22082,#4828,.T.) ;
#28046=EDGE_CURVE('',#22094,#22095,#18695,.F.) ;
#28047=EDGE_CURVE('',#22096,#22094,#18696,.F.) ;
#28048=EDGE_CURVE('',#22095,#22096,#18697,.F.) ;
#28049=EDGE_CURVE('',#21917,#22096,#4829,.T.) ;
#28050=EDGE_CURVE('',#22094,#21918,#4830,.T.) ;
#28051=EDGE_CURVE('',#22007,#22095,#4831,.T.) ;
#28052=EDGE_CURVE('',#22096,#22004,#4832,.T.) ;
#28053=EDGE_CURVE('',#22097,#22098,#18698,.F.) ;
#28054=EDGE_CURVE('',#22099,#22097,#18699,.T.) ;
#28055=EDGE_CURVE('',#22099,#22100,#18700,.T.) ;
#28056=EDGE_CURVE('',#22098,#22100,#18701,.T.) ;
#28057=EDGE_CURVE('',#22009,#22099,#4833,.T.) ;
#28058=EDGE_CURVE('',#22097,#22006,#4834,.T.) ;
#28059=EDGE_CURVE('',#21919,#22098,#4835,.T.) ;
#28060=EDGE_CURVE('',#22100,#21920,#4836,.T.) ;
#28061=EDGE_CURVE('',#22095,#22097,#4837,.T.) ;
#28062=EDGE_CURVE('',#22098,#22094,#4838,.T.) ;
#28063=EDGE_CURVE('',#22101,#21916,#4839,.T.) ;
#28064=EDGE_CURVE('',#22102,#22101,#18702,.T.) ;
#28065=EDGE_CURVE('',#22103,#22102,#4840,.T.) ;
#28066=EDGE_CURVE('',#22103,#22104,#18703,.T.) ;
#28067=EDGE_CURVE('',#22104,#22105,#4841,.T.) ;
#28068=EDGE_CURVE('',#22105,#22106,#18704,.T.) ;
#28069=EDGE_CURVE('',#22107,#22106,#4842,.T.) ;
#28070=EDGE_CURVE('',#22108,#22107,#18705,.T.) ;
#28071=EDGE_CURVE('',#22109,#22108,#4843,.T.) ;
#28072=EDGE_CURVE('',#22110,#22109,#4844,.T.) ;
#28073=EDGE_CURVE('',#22111,#22110,#4845,.T.) ;
#28074=EDGE_CURVE('',#22112,#22111,#4846,.T.) ;
#28075=EDGE_CURVE('',#22113,#22112,#4847,.T.) ;
#28076=EDGE_CURVE('',#22114,#22113,#18706,.T.) ;
#28077=EDGE_CURVE('',#22115,#22114,#4848,.T.) ;
#28078=EDGE_CURVE('',#22116,#22115,#18707,.T.) ;
#28079=EDGE_CURVE('',#22117,#22116,#4849,.T.) ;
#28080=EDGE_CURVE('',#22118,#22117,#18708,.T.) ;
#28081=EDGE_CURVE('',#22119,#22118,#4850,.T.) ;
#28082=EDGE_CURVE('',#22119,#22120,#18709,.T.) ;
#28083=EDGE_CURVE('',#22120,#22121,#4851,.T.) ;
#28084=EDGE_CURVE('',#22121,#22122,#18710,.T.) ;
#28085=EDGE_CURVE('',#22122,#22123,#4852,.T.) ;
#28086=EDGE_CURVE('',#22124,#22123,#18711,.T.) ;
#28087=EDGE_CURVE('',#22125,#22124,#4853,.T.) ;
#28088=EDGE_CURVE('',#22126,#22125,#4854,.T.) ;
#28089=EDGE_CURVE('',#22127,#22126,#4855,.T.) ;
#28090=EDGE_CURVE('',#22128,#22127,#18712,.T.) ;
#28091=EDGE_CURVE('',#22129,#22128,#4856,.T.) ;
#28092=EDGE_CURVE('',#22129,#22130,#18713,.T.) ;
#28093=EDGE_CURVE('',#22130,#22131,#4857,.T.) ;
#28094=EDGE_CURVE('',#22131,#22132,#18714,.T.) ;
#28095=EDGE_CURVE('',#22132,#22133,#4858,.T.) ;
#28096=EDGE_CURVE('',#22133,#22134,#18715,.T.) ;
#28097=EDGE_CURVE('',#22134,#22135,#4859,.T.) ;
#28098=EDGE_CURVE('',#22136,#22135,#18716,.T.) ;
#28099=EDGE_CURVE('',#22137,#22136,#4860,.T.) ;
#28100=EDGE_CURVE('',#22137,#22138,#4861,.T.) ;
#28101=EDGE_CURVE('',#22138,#22139,#4862,.T.) ;
#28102=EDGE_CURVE('',#22139,#22140,#4863,.T.) ;
#28103=EDGE_CURVE('',#22140,#22141,#4864,.T.) ;
#28104=EDGE_CURVE('',#22141,#22142,#4865,.T.) ;
#28105=EDGE_CURVE('',#22142,#22143,#1242,.T.) ;
#28106=EDGE_CURVE('',#22144,#22143,#4866,.T.) ;
#28107=EDGE_CURVE('',#22144,#22145,#1243,.T.) ;
#28108=EDGE_CURVE('',#22145,#22146,#4867,.T.) ;
#28109=EDGE_CURVE('',#22146,#22147,#4868,.T.) ;
#28110=EDGE_CURVE('',#22147,#22148,#4869,.T.) ;
#28111=EDGE_CURVE('',#22148,#22149,#18717,.T.) ;
#28112=EDGE_CURVE('',#22149,#22150,#4870,.T.) ;
#28113=EDGE_CURVE('',#22150,#22151,#18718,.T.) ;
#28114=EDGE_CURVE('',#22151,#22152,#4871,.T.) ;
#28115=EDGE_CURVE('',#22152,#22153,#4872,.T.) ;
#28116=EDGE_CURVE('',#22153,#22154,#18719,.T.) ;
#28117=EDGE_CURVE('',#22154,#22155,#4873,.T.) ;
#28118=EDGE_CURVE('',#22156,#22155,#4874,.T.) ;
#28119=EDGE_CURVE('',#22156,#22157,#18720,.T.) ;
#28120=EDGE_CURVE('',#22157,#22158,#4875,.T.) ;
#28121=EDGE_CURVE('',#22158,#22090,#1244,.T.) ;
#28122=EDGE_CURVE('',#22089,#22159,#4876,.T.) ;
#28123=EDGE_CURVE('',#22160,#22159,#4877,.F.) ;
#28124=EDGE_CURVE('',#22161,#22160,#4878,.T.) ;
#28125=EDGE_CURVE('',#22162,#22161,#18721,.T.) ;
#28126=EDGE_CURVE('',#22163,#22162,#18722,.T.) ;
#28127=EDGE_CURVE('',#22164,#22163,#18723,.T.) ;
#28128=EDGE_CURVE('',#22164,#22165,#18724,.T.) ;
#28129=EDGE_CURVE('',#22166,#22165,#4879,.T.) ;
#28130=EDGE_CURVE('',#22166,#22167,#18725,.T.) ;
#28131=EDGE_CURVE('',#22168,#22167,#4880,.T.) ;
#28132=EDGE_CURVE('',#22169,#22168,#4881,.T.) ;
#28133=EDGE_CURVE('',#22169,#22170,#18726,.T.) ;
#28134=EDGE_CURVE('',#22171,#22170,#4882,.T.) ;
#28135=EDGE_CURVE('',#22171,#22172,#18727,.T.) ;
#28136=EDGE_CURVE('',#22173,#22172,#4883,.T.) ;
#28137=EDGE_CURVE('',#22174,#22173,#4884,.T.) ;
#28138=EDGE_CURVE('',#22174,#22175,#18728,.T.) ;
#28139=EDGE_CURVE('',#22176,#22175,#4885,.T.) ;
#28140=EDGE_CURVE('',#22176,#22177,#18729,.T.) ;
#28141=EDGE_CURVE('',#22177,#22178,#4886,.T.) ;
#28142=EDGE_CURVE('',#22178,#22179,#4887,.T.) ;
#28143=EDGE_CURVE('',#22180,#22179,#4888,.T.) ;
#28144=EDGE_CURVE('',#22181,#22180,#18730,.T.) ;
#28145=EDGE_CURVE('',#22182,#22181,#4889,.T.) ;
#28146=EDGE_CURVE('',#22183,#22182,#18731,.T.) ;
#28147=EDGE_CURVE('',#22184,#22183,#4890,.T.) ;
#28148=EDGE_CURVE('',#22185,#22184,#18732,.T.) ;
#28149=EDGE_CURVE('',#22186,#22185,#4891,.T.) ;
#28150=EDGE_CURVE('',#22187,#22186,#18733,.T.) ;
#28151=EDGE_CURVE('',#22188,#22187,#4892,.T.) ;
#28152=EDGE_CURVE('',#22188,#22002,#4893,.T.) ;
#28153=EDGE_CURVE('',#22189,#22013,#18734,.T.) ;
#28154=EDGE_CURVE('',#22190,#22189,#18735,.T.) ;
#28155=EDGE_CURVE('',#22191,#22190,#4894,.T.) ;
#28156=EDGE_CURVE('',#22192,#22191,#18736,.T.) ;
#28157=EDGE_CURVE('',#22193,#22192,#4895,.T.) ;
#28158=EDGE_CURVE('',#22194,#22193,#4896,.T.) ;
#28159=EDGE_CURVE('',#22195,#22194,#18737,.T.) ;
#28160=EDGE_CURVE('',#22196,#22195,#4897,.T.) ;
#28161=EDGE_CURVE('',#22197,#22196,#18738,.T.) ;
#28162=EDGE_CURVE('',#22197,#22198,#18739,.T.) ;
#28163=EDGE_CURVE('',#22198,#22199,#4898,.T.) ;
#28164=EDGE_CURVE('',#22199,#22010,#4899,.T.) ;
#28165=EDGE_CURVE('',#22200,#22201,#18740,.T.) ;
#28166=EDGE_CURVE('',#22202,#22200,#4900,.T.) ;
#28167=EDGE_CURVE('',#22203,#22202,#18741,.T.) ;
#28168=EDGE_CURVE('',#22204,#22203,#4901,.T.) ;
#28169=EDGE_CURVE('',#22205,#22204,#18742,.T.) ;
#28170=EDGE_CURVE('',#22206,#22205,#4902,.T.) ;
#28171=EDGE_CURVE('',#22207,#22206,#18743,.T.) ;
#28172=EDGE_CURVE('',#22201,#22207,#4903,.T.) ;
#28173=EDGE_CURVE('',#22208,#22208,#18744,.T.) ;
#28174=EDGE_CURVE('',#22209,#22210,#18745,.T.) ;
#28175=EDGE_CURVE('',#22211,#22209,#4904,.T.) ;
#28176=EDGE_CURVE('',#22212,#22211,#18746,.T.) ;
#28177=EDGE_CURVE('',#22213,#22212,#4905,.T.) ;
#28178=EDGE_CURVE('',#22214,#22213,#4906,.T.) ;
#28179=EDGE_CURVE('',#22215,#22214,#18747,.T.) ;
#28180=EDGE_CURVE('',#22216,#22215,#4907,.T.) ;
#28181=EDGE_CURVE('',#22217,#22216,#18748,.T.) ;
#28182=EDGE_CURVE('',#22218,#22217,#4908,.T.) ;
#28183=EDGE_CURVE('',#22219,#22218,#18749,.T.) ;
#28184=EDGE_CURVE('',#22220,#22219,#4909,.T.) ;
#28185=EDGE_CURVE('',#22221,#22220,#18750,.T.) ;
#28186=EDGE_CURVE('',#22222,#22221,#4910,.T.) ;
#28187=EDGE_CURVE('',#22210,#22222,#4911,.T.) ;
#28188=EDGE_CURVE('',#22223,#22223,#18751,.T.) ;
#28189=EDGE_CURVE('',#22224,#22225,#4912,.T.) ;
#28190=EDGE_CURVE('',#22226,#22224,#1245,.T.) ;
#28191=EDGE_CURVE('',#22227,#22226,#4913,.T.) ;
#28192=EDGE_CURVE('',#22228,#22227,#18752,.T.) ;
#28193=EDGE_CURVE('',#22229,#22228,#4914,.T.) ;
#28194=EDGE_CURVE('',#22230,#22229,#18753,.T.) ;
#28195=EDGE_CURVE('',#22231,#22230,#4915,.T.) ;
#28196=EDGE_CURVE('',#22232,#22231,#18754,.T.) ;
#28197=EDGE_CURVE('',#22233,#22232,#4916,.T.) ;
#28198=EDGE_CURVE('',#22234,#22233,#18755,.T.) ;
#28199=EDGE_CURVE('',#22235,#22234,#4917,.T.) ;
#28200=EDGE_CURVE('',#22225,#22235,#1246,.T.) ;
#28201=EDGE_CURVE('',#22236,#22237,#1247,.T.) ;
#28202=EDGE_CURVE('',#21809,#22236,#4918,.T.) ;
#28203=EDGE_CURVE('',#22238,#21807,#4919,.T.) ;
#28204=EDGE_CURVE('',#22239,#22238,#4920,.T.) ;
#28205=EDGE_CURVE('',#22240,#22239,#18756,.T.) ;
#28206=EDGE_CURVE('',#22241,#22240,#4921,.T.) ;
#28207=EDGE_CURVE('',#22242,#22241,#18757,.T.) ;
#28208=EDGE_CURVE('',#22243,#22242,#4922,.T.) ;
#28209=EDGE_CURVE('',#22244,#22243,#18758,.T.) ;
#28210=EDGE_CURVE('',#22245,#22244,#4923,.T.) ;
#28211=EDGE_CURVE('',#22246,#22245,#18759,.T.) ;
#28212=EDGE_CURVE('',#22247,#22246,#4924,.T.) ;
#28213=EDGE_CURVE('',#22237,#22247,#4925,.T.) ;
#28214=EDGE_CURVE('',#22248,#22249,#18760,.T.) ;
#28215=EDGE_CURVE('',#22250,#22248,#4926,.T.) ;
#28216=EDGE_CURVE('',#22251,#22250,#18761,.T.) ;
#28217=EDGE_CURVE('',#22252,#22251,#4927,.T.) ;
#28218=EDGE_CURVE('',#22253,#22252,#4928,.T.) ;
#28219=EDGE_CURVE('',#22254,#22253,#18762,.T.) ;
#28220=EDGE_CURVE('',#22255,#22254,#4929,.T.) ;
#28221=EDGE_CURVE('',#22256,#22255,#18763,.T.) ;
#28222=EDGE_CURVE('',#22257,#22256,#4930,.T.) ;
#28223=EDGE_CURVE('',#22258,#22257,#18764,.T.) ;
#28224=EDGE_CURVE('',#22259,#22258,#4931,.T.) ;
#28225=EDGE_CURVE('',#22260,#22259,#18765,.T.) ;
#28226=EDGE_CURVE('',#22261,#22260,#4932,.T.) ;
#28227=EDGE_CURVE('',#22249,#22261,#4933,.T.) ;
#28228=EDGE_CURVE('',#22262,#22263,#1248,.T.) ;
#28229=EDGE_CURVE('',#22264,#22263,#18766,.T.) ;
#28230=EDGE_CURVE('',#22162,#22264,#1249,.F.) ;
#28231=EDGE_CURVE('',#22262,#22162,#18767,.T.) ;
#28232=EDGE_CURVE('',#22000,#22264,#4934,.T.) ;
#28233=EDGE_CURVE('',#22263,#21975,#4935,.T.) ;
#28234=EDGE_CURVE('',#22265,#22163,#1250,.T.) ;
#28235=EDGE_CURVE('',#22264,#22265,#18768,.T.) ;
#28236=EDGE_CURVE('',#22161,#22266,#18769,.T.) ;
#28237=EDGE_CURVE('',#22266,#22262,#18770,.T.) ;
#28238=EDGE_CURVE('',#22160,#22267,#18771,.F.) ;
#28239=EDGE_CURVE('',#22267,#22266,#4936,.T.) ;
#28240=EDGE_CURVE('',#22265,#21999,#4937,.T.) ;
#28241=EDGE_CURVE('',#22266,#22268,#4938,.T.) ;
#28242=EDGE_CURVE('',#22269,#22268,#18772,.T.) ;
#28243=EDGE_CURVE('',#21976,#22269,#4939,.T.) ;
#28244=EDGE_CURVE('',#22270,#22267,#4940,.T.) ;
#28245=EDGE_CURVE('',#22270,#22091,#4941,.T.) ;
#28246=EDGE_CURVE('',#22093,#22271,#4942,.T.) ;
#28247=EDGE_CURVE('',#22268,#22271,#4943,.T.) ;
#28248=EDGE_CURVE('',#22001,#22188,#4944,.T.) ;
#28249=EDGE_CURVE('',#22187,#22272,#4945,.T.) ;
#28250=EDGE_CURVE('',#22272,#22273,#4946,.T.) ;
#28251=EDGE_CURVE('',#21992,#22273,#4947,.T.) ;
#28252=EDGE_CURVE('',#22274,#22275,#18773,.F.) ;
#28253=EDGE_CURVE('',#22276,#22274,#18774,.F.) ;
#28254=EDGE_CURVE('',#22275,#22276,#18775,.F.) ;
#28255=EDGE_CURVE('',#21907,#22277,#4948,.T.) ;
#28256=EDGE_CURVE('',#22277,#22278,#18776,.T.) ;
#28257=EDGE_CURVE('',#22278,#21905,#4949,.T.) ;
#28258=EDGE_CURVE('',#22279,#22280,#18777,.T.) ;
#28259=EDGE_CURVE('',#22280,#22278,#18778,.T.) ;
#28260=EDGE_CURVE('',#22277,#22279,#18779,.T.) ;
#28261=EDGE_CURVE('',#22281,#22282,#18780,.T.) ;
#28262=EDGE_CURVE('',#22282,#22280,#4950,.T.) ;
#28263=EDGE_CURVE('',#22279,#22281,#4951,.T.) ;
#28264=EDGE_CURVE('',#22283,#22284,#18781,.T.) ;
#28265=EDGE_CURVE('',#22284,#22282,#18782,.T.) ;
#28266=EDGE_CURVE('',#22281,#22283,#18783,.T.) ;
#28267=EDGE_CURVE('',#22274,#22284,#4952,.T.) ;
#28268=EDGE_CURVE('',#22283,#22276,#4953,.T.) ;
#28269=EDGE_CURVE('',#22285,#22286,#1251,.T.) ;
#28270=EDGE_CURVE('',#22286,#22287,#4954,.T.) ;
#28271=EDGE_CURVE('',#22287,#22288,#18784,.T.) ;
#28272=EDGE_CURVE('',#22288,#22285,#4955,.T.) ;
#28273=EDGE_CURVE('',#22289,#22290,#18785,.T.) ;
#28274=EDGE_CURVE('',#22290,#22288,#18786,.T.) ;
#28275=EDGE_CURVE('',#22287,#22289,#18787,.T.) ;
#28276=EDGE_CURVE('',#22276,#22290,#4956,.T.) ;
#28277=EDGE_CURVE('',#22289,#22275,#4957,.T.) ;
#28278=EDGE_CURVE('',#22193,#22291,#448,.F.) ;
#28279=EDGE_CURVE('',#22292,#22193,#18788,.T.) ;
#28280=EDGE_CURVE('',#22292,#22293,#449,.T.) ;
#28281=EDGE_CURVE('',#22291,#22293,#18789,.T.) ;
#28282=EDGE_CURVE('',#22014,#22294,#18790,.T.) ;
#28283=EDGE_CURVE('',#22294,#22189,#18791,.T.) ;
#28284=EDGE_CURVE('',#22295,#22190,#18792,.T.) ;
#28285=EDGE_CURVE('',#22294,#22295,#18793,.T.) ;
#28286=EDGE_CURVE('',#22296,#22191,#18794,.T.) ;
#28287=EDGE_CURVE('',#22295,#22296,#4958,.T.) ;
#28288=EDGE_CURVE('',#22297,#22192,#18795,.T.) ;
#28289=EDGE_CURVE('',#22296,#22297,#18796,.T.) ;
#28290=EDGE_CURVE('',#22297,#22292,#4959,.T.) ;
#28291=EDGE_CURVE('',#22293,#22274,#4960,.T.) ;
#28292=EDGE_CURVE('',#22275,#22291,#4961,.T.) ;
#28293=EDGE_CURVE('',#22298,#22194,#18797,.T.) ;
#28294=EDGE_CURVE('',#22291,#22298,#4962,.T.) ;
#28295=EDGE_CURVE('',#22299,#22195,#18798,.T.) ;
#28296=EDGE_CURVE('',#22298,#22299,#18799,.T.) ;
#28297=EDGE_CURVE('',#22300,#22196,#18800,.T.) ;
#28298=EDGE_CURVE('',#22299,#22300,#4963,.T.) ;
#28299=EDGE_CURVE('',#22197,#22301,#1252,.F.) ;
#28300=EDGE_CURVE('',#22301,#22300,#1253,.F.) ;
#28301=EDGE_CURVE('',#22011,#22302,#4964,.T.) ;
#28302=EDGE_CURVE('',#22302,#22303,#4965,.T.) ;
#28303=EDGE_CURVE('',#22303,#22285,#18801,.T.) ;
#28304=EDGE_CURVE('',#22278,#22304,#4966,.T.) ;
#28305=EDGE_CURVE('',#22305,#22304,#4967,.T.) ;
#28306=EDGE_CURVE('',#22306,#22305,#4968,.T.) ;
#28307=EDGE_CURVE('',#21910,#22306,#450,.T.) ;
#28308=EDGE_CURVE('',#22280,#22307,#4969,.T.) ;
#28309=EDGE_CURVE('',#22304,#22307,#18802,.T.) ;
#28310=EDGE_CURVE('',#22308,#22282,#4970,.T.) ;
#28311=EDGE_CURVE('',#22307,#22308,#4971,.T.) ;
#28312=EDGE_CURVE('',#22284,#22309,#4972,.T.) ;
#28313=EDGE_CURVE('',#22308,#22309,#18803,.T.) ;
#28314=EDGE_CURVE('',#22297,#22310,#4973,.T.) ;
#28315=EDGE_CURVE('',#22311,#22310,#4974,.T.) ;
#28316=EDGE_CURVE('',#22312,#22311,#18804,.T.) ;
#28317=EDGE_CURVE('',#22313,#22312,#4975,.T.) ;
#28318=EDGE_CURVE('',#22314,#22313,#18805,.T.) ;
#28319=EDGE_CURVE('',#22315,#22314,#4976,.T.) ;
#28320=EDGE_CURVE('',#22316,#22315,#18806,.T.) ;
#28321=EDGE_CURVE('',#22309,#22316,#4977,.T.) ;
#28322=EDGE_CURVE('',#22296,#22317,#4978,.T.) ;
#28323=EDGE_CURVE('',#22310,#22317,#451,.T.) ;
#28324=EDGE_CURVE('',#22295,#22318,#4979,.T.) ;
#28325=EDGE_CURVE('',#22317,#22318,#4980,.T.) ;
#28326=EDGE_CURVE('',#22319,#22294,#4981,.T.) ;
#28327=EDGE_CURVE('',#22318,#22319,#452,.T.) ;
#28328=EDGE_CURVE('',#22320,#22017,#18807,.T.) ;
#28329=EDGE_CURVE('',#22321,#22320,#1254,.T.) ;
#28330=EDGE_CURVE('',#22319,#22321,#453,.T.) ;
#28331=EDGE_CURVE('',#22322,#22323,#18808,.T.) ;
#28332=EDGE_CURVE('',#22324,#22322,#1255,.F.) ;
#28333=EDGE_CURVE('',#22325,#22324,#18809,.T.) ;
#28334=EDGE_CURVE('',#22325,#22323,#1256,.T.) ;
#28335=EDGE_CURVE('',#22326,#22327,#18810,.T.) ;
#28336=EDGE_CURVE('',#22326,#22324,#4982,.T.) ;
#28337=EDGE_CURVE('',#22322,#22327,#4983,.T.) ;
#28338=EDGE_CURVE('',#22328,#22329,#18811,.F.) ;
#28339=EDGE_CURVE('',#22330,#22328,#18812,.T.) ;
#28340=EDGE_CURVE('',#22330,#22331,#18813,.T.) ;
#28341=EDGE_CURVE('',#22329,#22331,#18814,.T.) ;
#28342=EDGE_CURVE('',#22332,#22333,#18815,.T.) ;
#28343=EDGE_CURVE('',#22333,#22330,#4984,.T.) ;
#28344=EDGE_CURVE('',#22328,#22332,#4985,.T.) ;
#28345=EDGE_CURVE('',#22332,#22322,#18816,.T.) ;
#28346=EDGE_CURVE('',#22323,#22333,#18817,.T.) ;
#28347=EDGE_CURVE('',#22334,#22335,#18818,.T.) ;
#28348=EDGE_CURVE('',#22336,#22335,#18819,.T.) ;
#28349=EDGE_CURVE('',#22337,#22336,#18820,.F.) ;
#28350=EDGE_CURVE('',#22334,#22337,#18821,.T.) ;
#28351=EDGE_CURVE('',#22338,#22339,#1257,.F.) ;
#28352=EDGE_CURVE('',#22340,#22338,#18822,.T.) ;
#28353=EDGE_CURVE('',#22340,#22341,#1258,.T.) ;
#28354=EDGE_CURVE('',#22339,#22341,#18823,.T.) ;
#28355=EDGE_CURVE('',#22342,#22343,#18824,.T.) ;
#28356=EDGE_CURVE('',#22343,#22340,#18825,.T.) ;
#28357=EDGE_CURVE('',#22338,#22342,#18826,.T.) ;
#28358=EDGE_CURVE('',#22335,#22343,#4986,.T.) ;
#28359=EDGE_CURVE('',#22342,#22336,#4987,.T.) ;
#28360=EDGE_CURVE('',#22344,#22345,#18827,.T.) ;
#28361=EDGE_CURVE('',#22345,#22339,#4988,.T.) ;
#28362=EDGE_CURVE('',#22341,#22344,#4989,.T.) ;
#28363=EDGE_CURVE('',#21863,#22346,#18828,.T.) ;
#28364=EDGE_CURVE('',#22346,#22345,#1259,.T.) ;
#28365=EDGE_CURVE('',#22344,#21863,#1260,.T.) ;
#28366=EDGE_CURVE('',#21862,#22347,#18829,.T.) ;
#28367=EDGE_CURVE('',#22347,#22346,#454,.T.) ;
#28368=EDGE_CURVE('',#21947,#22347,#4990,.T.) ;
#28369=EDGE_CURVE('',#22348,#22349,#18830,.T.) ;
#28370=EDGE_CURVE('',#22348,#22338,#4991,.T.) ;
#28371=EDGE_CURVE('',#22339,#22349,#4992,.T.) ;
#28372=EDGE_CURVE('',#21895,#22350,#18831,.T.) ;
#28373=EDGE_CURVE('',#22350,#21948,#18832,.T.) ;
#28374=EDGE_CURVE('',#21894,#22351,#18833,.T.) ;
#28375=EDGE_CURVE('',#22351,#22350,#4993,.T.) ;
#28376=EDGE_CURVE('',#21893,#22352,#18834,.T.) ;
#28377=EDGE_CURVE('',#22352,#22351,#18835,.T.) ;
#28378=EDGE_CURVE('',#21938,#22352,#4994,.T.) ;
#28379=EDGE_CURVE('',#22353,#22354,#18836,.T.) ;
#28380=EDGE_CURVE('',#22353,#22337,#4995,.T.) ;
#28381=EDGE_CURVE('',#22336,#22354,#4996,.T.) ;
#28382=EDGE_CURVE('',#22355,#22356,#18837,.T.) ;
#28383=EDGE_CURVE('',#22356,#22334,#4997,.T.) ;
#28384=EDGE_CURVE('',#22337,#22355,#4998,.T.) ;
#28385=EDGE_CURVE('',#22357,#22358,#18838,.T.) ;
#28386=EDGE_CURVE('',#22358,#22356,#18839,.T.) ;
#28387=EDGE_CURVE('',#22355,#22357,#18840,.T.) ;
#28388=EDGE_CURVE('',#22359,#22360,#18841,.T.) ;
#28389=EDGE_CURVE('',#22360,#22358,#4999,.T.) ;
#28390=EDGE_CURVE('',#22357,#22359,#5000,.T.) ;
#28391=EDGE_CURVE('',#22361,#22362,#18842,.T.) ;
#28392=EDGE_CURVE('',#22362,#22360,#18843,.T.) ;
#28393=EDGE_CURVE('',#22359,#22361,#18844,.T.) ;
#28394=EDGE_CURVE('',#22363,#22364,#18845,.T.) ;
#28395=EDGE_CURVE('',#22364,#22362,#5001,.T.) ;
#28396=EDGE_CURVE('',#22361,#22363,#5002,.T.) ;
#28397=EDGE_CURVE('',#22365,#22366,#18846,.T.) ;
#28398=EDGE_CURVE('',#22366,#22364,#18847,.T.) ;
#28399=EDGE_CURVE('',#22363,#22365,#18848,.T.) ;
#28400=EDGE_CURVE('',#22367,#22368,#18849,.T.) ;
#28401=EDGE_CURVE('',#22368,#22366,#5003,.T.) ;
#28402=EDGE_CURVE('',#22365,#22367,#5004,.T.) ;
#28403=EDGE_CURVE('',#22369,#22370,#18850,.T.) ;
#28404=EDGE_CURVE('',#22370,#22368,#18851,.T.) ;
#28405=EDGE_CURVE('',#22367,#22369,#18852,.T.) ;
#28406=EDGE_CURVE('',#22331,#22370,#5005,.T.) ;
#28407=EDGE_CURVE('',#22369,#22329,#5006,.T.) ;
#28408=EDGE_CURVE('',#22371,#22372,#18853,.T.) ;
#28409=EDGE_CURVE('',#22372,#22325,#5007,.T.) ;
#28410=EDGE_CURVE('',#22324,#22371,#5008,.T.) ;
#28411=EDGE_CURVE('',#22371,#22373,#1261,.T.) ;
#28412=EDGE_CURVE('',#22373,#21945,#18854,.T.) ;
#28413=EDGE_CURVE('',#21945,#22372,#1262,.T.) ;
#28414=EDGE_CURVE('',#22373,#21942,#455,.T.) ;
#28415=EDGE_CURVE('',#22374,#22375,#18855,.T.) ;
#28416=EDGE_CURVE('',#22374,#22328,#5009,.T.) ;
#28417=EDGE_CURVE('',#22329,#22375,#5010,.T.) ;
#28418=EDGE_CURVE('',#22376,#21944,#18856,.T.) ;
#28419=EDGE_CURVE('',#22376,#22333,#5011,.T.) ;
#28420=EDGE_CURVE('',#22343,#22377,#5012,.T.) ;
#28421=EDGE_CURVE('',#22377,#21864,#1263,.F.) ;
#28422=EDGE_CURVE('',#22347,#22378,#5013,.T.) ;
#28423=EDGE_CURVE('',#22378,#22379,#18857,.F.) ;
#28424=EDGE_CURVE('',#22379,#22345,#5014,.T.) ;
#28425=EDGE_CURVE('',#22200,#22350,#5015,.T.) ;
#28426=EDGE_CURVE('',#22201,#21948,#5016,.T.) ;
#28427=EDGE_CURVE('',#22202,#22351,#5017,.T.) ;
#28428=EDGE_CURVE('',#22203,#22352,#5018,.T.) ;
#28429=EDGE_CURVE('',#22371,#22380,#5019,.T.) ;
#28430=EDGE_CURVE('',#22380,#22381,#18858,.F.) ;
#28431=EDGE_CURVE('',#22381,#21942,#5020,.T.) ;
#28432=EDGE_CURVE('',#22207,#22359,#5021,.T.) ;
#28433=EDGE_CURVE('',#22382,#22357,#5022,.T.) ;
#28434=EDGE_CURVE('',#22382,#22378,#5023,.T.) ;
#28435=EDGE_CURVE('',#22326,#22380,#5024,.T.) ;
#28436=EDGE_CURVE('',#22381,#22383,#5025,.T.) ;
#28437=EDGE_CURVE('',#22367,#22383,#5026,.T.) ;
#28438=EDGE_CURVE('',#22204,#22365,#5027,.T.) ;
#28439=EDGE_CURVE('',#22374,#22327,#5028,.T.) ;
#28440=EDGE_CURVE('',#22384,#22375,#5029,.T.) ;
#28441=EDGE_CURVE('',#22383,#22384,#18859,.F.) ;
#28442=EDGE_CURVE('',#22385,#22386,#18860,.F.) ;
#28443=EDGE_CURVE('',#22386,#22387,#5030,.T.) ;
#28444=EDGE_CURVE('',#22387,#22388,#18861,.F.) ;
#28445=EDGE_CURVE('',#22388,#22385,#5031,.T.) ;
#28446=EDGE_CURVE('',#22389,#22386,#5032,.T.) ;
#28447=EDGE_CURVE('',#22390,#22389,#5033,.T.) ;
#28448=EDGE_CURVE('',#22387,#22390,#5034,.T.) ;
#28449=EDGE_CURVE('',#22391,#22390,#18862,.F.) ;
#28450=EDGE_CURVE('',#22389,#22392,#18863,.F.) ;
#28451=EDGE_CURVE('',#22392,#22391,#5035,.T.) ;
#28452=EDGE_CURVE('',#22393,#22394,#18864,.T.) ;
#28453=EDGE_CURVE('',#22395,#22394,#18865,.T.) ;
#28454=EDGE_CURVE('',#22396,#22395,#18866,.F.) ;
#28455=EDGE_CURVE('',#22393,#22396,#18867,.T.) ;
#28456=EDGE_CURVE('',#22397,#22398,#18868,.F.) ;
#28457=EDGE_CURVE('',#22399,#22397,#18869,.T.) ;
#28458=EDGE_CURVE('',#22399,#22400,#18870,.T.) ;
#28459=EDGE_CURVE('',#22398,#22400,#18871,.T.) ;
#28460=EDGE_CURVE('',#22394,#22399,#5036,.T.) ;
#28461=EDGE_CURVE('',#22397,#22395,#5037,.T.) ;
#28462=EDGE_CURVE('',#22401,#22402,#18872,.T.) ;
#28463=EDGE_CURVE('',#22402,#22403,#5038,.T.) ;
#28464=EDGE_CURVE('',#22403,#22404,#18873,.F.) ;
#28465=EDGE_CURVE('',#22404,#22401,#5039,.T.) ;
#28466=EDGE_CURVE('',#22405,#22406,#18874,.T.) ;
#28467=EDGE_CURVE('',#22406,#22402,#18875,.T.) ;
#28468=EDGE_CURVE('',#22401,#22405,#18876,.T.) ;
#28469=EDGE_CURVE('',#22400,#22406,#5040,.T.) ;
#28470=EDGE_CURVE('',#22405,#22398,#5041,.T.) ;
#28471=EDGE_CURVE('',#22407,#22408,#18877,.T.) ;
#28472=EDGE_CURVE('',#22407,#22397,#5042,.T.) ;
#28473=EDGE_CURVE('',#22398,#22408,#5043,.T.) ;
#28474=EDGE_CURVE('',#22409,#22410,#18878,.T.) ;
#28475=EDGE_CURVE('',#22409,#22396,#5044,.T.) ;
#28476=EDGE_CURVE('',#22395,#22410,#5045,.T.) ;
#28477=EDGE_CURVE('',#22411,#22412,#18879,.T.) ;
#28478=EDGE_CURVE('',#22412,#22393,#5046,.T.) ;
#28479=EDGE_CURVE('',#22396,#22411,#5047,.T.) ;
#28480=EDGE_CURVE('',#22413,#22414,#18880,.T.) ;
#28481=EDGE_CURVE('',#22414,#22412,#18881,.T.) ;
#28482=EDGE_CURVE('',#22411,#22413,#18882,.T.) ;
#28483=EDGE_CURVE('',#22415,#22416,#18883,.F.) ;
#28484=EDGE_CURVE('',#22416,#22414,#5048,.T.) ;
#28485=EDGE_CURVE('',#22413,#22415,#5049,.T.) ;
#28486=EDGE_CURVE('',#22406,#22417,#5050,.T.) ;
#28487=EDGE_CURVE('',#22418,#22417,#18884,.T.) ;
#28488=EDGE_CURVE('',#22402,#22418,#5051,.T.) ;
#28489=EDGE_CURVE('',#22419,#22412,#5052,.T.) ;
#28490=EDGE_CURVE('',#22420,#22419,#5053,.T.) ;
#28491=EDGE_CURVE('',#22421,#22420,#18885,.T.) ;
#28492=EDGE_CURVE('',#22422,#22421,#5054,.T.) ;
#28493=EDGE_CURVE('',#22423,#22422,#5055,.T.) ;
#28494=EDGE_CURVE('',#22424,#22423,#18886,.T.) ;
#28495=EDGE_CURVE('',#22425,#22424,#5056,.T.) ;
#28496=EDGE_CURVE('',#22426,#22425,#18887,.T.) ;
#28497=EDGE_CURVE('',#22427,#22426,#5057,.T.) ;
#28498=EDGE_CURVE('',#22428,#22427,#18888,.T.) ;
#28499=EDGE_CURVE('',#22417,#22428,#5058,.T.) ;
#28500=EDGE_CURVE('',#22429,#22414,#5059,.T.) ;
#28501=EDGE_CURVE('',#22419,#22429,#18889,.T.) ;
#28502=EDGE_CURVE('',#22430,#21869,#5060,.T.) ;
#28503=EDGE_CURVE('',#22430,#22431,#5061,.T.) ;
#28504=EDGE_CURVE('',#22432,#22431,#5062,.T.) ;
#28505=EDGE_CURVE('',#22433,#22432,#5063,.T.) ;
#28506=EDGE_CURVE('',#22429,#22433,#5064,.T.) ;
#28507=EDGE_CURVE('',#22416,#22403,#5065,.T.) ;
#28508=EDGE_CURVE('',#21949,#22418,#5066,.T.) ;
#28509=EDGE_CURVE('',#22304,#22434,#18890,.T.) ;
#28510=EDGE_CURVE('',#22434,#22435,#5067,.T.) ;
#28511=EDGE_CURVE('',#22435,#22305,#456,.T.) ;
#28512=EDGE_CURVE('',#22306,#22436,#18891,.T.) ;
#28513=EDGE_CURVE('',#22436,#21922,#457,.T.) ;
#28514=EDGE_CURVE('',#22435,#22436,#5068,.T.) ;
#28515=EDGE_CURVE('',#22307,#22437,#18892,.T.) ;
#28516=EDGE_CURVE('',#22437,#22434,#18893,.T.) ;
#28517=EDGE_CURVE('',#22308,#22438,#18894,.T.) ;
#28518=EDGE_CURVE('',#22438,#22437,#5069,.T.) ;
#28519=EDGE_CURVE('',#22309,#22439,#18895,.T.) ;
#28520=EDGE_CURVE('',#22439,#22438,#18896,.T.) ;
#28521=EDGE_CURVE('',#22316,#22440,#18897,.T.) ;
#28522=EDGE_CURVE('',#22440,#22439,#5070,.T.) ;
#28523=EDGE_CURVE('',#22315,#22441,#18898,.T.) ;
#28524=EDGE_CURVE('',#22441,#22440,#18899,.T.) ;
#28525=EDGE_CURVE('',#22314,#22442,#18900,.T.) ;
#28526=EDGE_CURVE('',#22442,#22441,#5071,.T.) ;
#28527=EDGE_CURVE('',#22313,#22443,#18901,.T.) ;
#28528=EDGE_CURVE('',#22443,#22442,#18902,.T.) ;
#28529=EDGE_CURVE('',#22312,#22444,#18903,.T.) ;
#28530=EDGE_CURVE('',#22444,#22443,#5072,.T.) ;
#28531=EDGE_CURVE('',#22311,#22445,#18904,.T.) ;
#28532=EDGE_CURVE('',#22445,#22444,#18905,.T.) ;
#28533=EDGE_CURVE('',#22310,#22446,#18906,.T.) ;
#28534=EDGE_CURVE('',#22446,#22445,#5073,.T.) ;
#28535=EDGE_CURVE('',#22317,#22447,#18907,.T.) ;
#28536=EDGE_CURVE('',#22447,#22446,#458,.T.) ;
#28537=EDGE_CURVE('',#22318,#22448,#18908,.T.) ;
#28538=EDGE_CURVE('',#22448,#22447,#5074,.T.) ;
#28539=EDGE_CURVE('',#22319,#22449,#18909,.T.) ;
#28540=EDGE_CURVE('',#22449,#22448,#459,.T.) ;
#28541=EDGE_CURVE('',#22321,#22450,#18910,.T.) ;
#28542=EDGE_CURVE('',#22450,#22449,#460,.T.) ;
#28543=EDGE_CURVE('',#22320,#21787,#18911,.T.) ;
#28544=EDGE_CURVE('',#21787,#22450,#1264,.T.) ;
#28545=EDGE_CURVE('',#22017,#21788,#18912,.T.) ;
#28546=EDGE_CURVE('',#22016,#21789,#18913,.T.) ;
#28547=EDGE_CURVE('',#22451,#21790,#18914,.T.) ;
#28548=EDGE_CURVE('',#22016,#22451,#18915,.T.) ;
#28549=EDGE_CURVE('',#22452,#21791,#18916,.T.) ;
#28550=EDGE_CURVE('',#22451,#22452,#5075,.T.) ;
#28551=EDGE_CURVE('',#22453,#21792,#18917,.T.) ;
#28552=EDGE_CURVE('',#22452,#22453,#18918,.T.) ;
#28553=EDGE_CURVE('',#22454,#21793,#18919,.T.) ;
#28554=EDGE_CURVE('',#22453,#22454,#18920,.T.) ;
#28555=EDGE_CURVE('',#22269,#21794,#18921,.T.) ;
#28556=EDGE_CURVE('',#22454,#22269,#5076,.T.) ;
#28557=EDGE_CURVE('',#22268,#21795,#18922,.T.) ;
#28558=EDGE_CURVE('',#22271,#21796,#18923,.T.) ;
#28559=EDGE_CURVE('',#22271,#22048,#18924,.T.) ;
#28560=EDGE_CURVE('',#22455,#22048,#5077,.T.) ;
#28561=EDGE_CURVE('',#22047,#22455,#5078,.T.) ;
#28562=EDGE_CURVE('',#22455,#22093,#18925,.T.) ;
#28563=EDGE_CURVE('',#21978,#22454,#5079,.T.) ;
#28564=EDGE_CURVE('',#22453,#21980,#5080,.T.) ;
#28565=EDGE_CURVE('',#21982,#22452,#5081,.T.) ;
#28566=EDGE_CURVE('',#21984,#22451,#5082,.T.) ;
#28567=EDGE_CURVE('',#22418,#22456,#18926,.T.) ;
#28568=EDGE_CURVE('',#22456,#21950,#5083,.T.) ;
#28569=EDGE_CURVE('',#21901,#22430,#461,.T.) ;
#28570=EDGE_CURVE('',#21902,#22457,#5084,.T.) ;
#28571=EDGE_CURVE('',#22457,#21899,#18927,.T.) ;
#28572=EDGE_CURVE('',#22458,#21900,#18928,.T.) ;
#28573=EDGE_CURVE('',#22457,#22458,#18929,.T.) ;
#28574=EDGE_CURVE('',#22458,#22430,#5085,.T.) ;
#28575=EDGE_CURVE('',#22417,#22459,#18930,.T.) ;
#28576=EDGE_CURVE('',#22459,#22456,#18931,.T.) ;
#28577=EDGE_CURVE('',#22428,#22460,#18932,.T.) ;
#28578=EDGE_CURVE('',#22460,#22459,#5086,.T.) ;
#28579=EDGE_CURVE('',#22427,#21943,#18933,.T.) ;
#28580=EDGE_CURVE('',#21943,#22460,#18934,.T.) ;
#28581=EDGE_CURVE('',#22426,#21944,#18935,.T.) ;
#28582=EDGE_CURVE('',#22425,#22376,#18936,.T.) ;
#28583=EDGE_CURVE('',#22424,#22461,#18937,.T.) ;
#28584=EDGE_CURVE('',#22461,#22376,#5087,.T.) ;
#28585=EDGE_CURVE('',#22423,#22462,#18938,.T.) ;
#28586=EDGE_CURVE('',#22462,#22461,#18939,.T.) ;
#28587=EDGE_CURVE('',#22463,#22462,#5088,.T.) ;
#28588=EDGE_CURVE('',#22422,#22463,#462,.T.) ;
#28589=EDGE_CURVE('',#22464,#22465,#18940,.T.) ;
#28590=EDGE_CURVE('',#22465,#22466,#5089,.T.) ;
#28591=EDGE_CURVE('',#22466,#22467,#18941,.T.) ;
#28592=EDGE_CURVE('',#22467,#22464,#5090,.T.) ;
#28593=EDGE_CURVE('',#22468,#22433,#18942,.T.) ;
#28594=EDGE_CURVE('',#22433,#22467,#18943,.T.) ;
#28595=EDGE_CURVE('',#22466,#22468,#18944,.T.) ;
#28596=EDGE_CURVE('',#22469,#22429,#18945,.T.) ;
#28597=EDGE_CURVE('',#22468,#22469,#5091,.T.) ;
#28598=EDGE_CURVE('',#22470,#22419,#18946,.T.) ;
#28599=EDGE_CURVE('',#22469,#22470,#18947,.T.) ;
#28600=EDGE_CURVE('',#22471,#22420,#18948,.T.) ;
#28601=EDGE_CURVE('',#22470,#22471,#5092,.T.) ;
#28602=EDGE_CURVE('',#22472,#22421,#18949,.T.) ;
#28603=EDGE_CURVE('',#22471,#22472,#18950,.T.) ;
#28604=EDGE_CURVE('',#22472,#22463,#5093,.T.) ;
#28605=EDGE_CURVE('',#21951,#22460,#5094,.T.) ;
#28606=EDGE_CURVE('',#22473,#22461,#5095,.T.) ;
#28607=EDGE_CURVE('',#22474,#22473,#18951,.T.) ;
#28608=EDGE_CURVE('',#22475,#22474,#5096,.T.) ;
#28609=EDGE_CURVE('',#22476,#22475,#18952,.T.) ;
#28610=EDGE_CURVE('',#22477,#22476,#5097,.T.) ;
#28611=EDGE_CURVE('',#22377,#22477,#18953,.T.) ;
#28612=EDGE_CURVE('',#22478,#22479,#1265,.T.) ;
#28613=EDGE_CURVE('',#22480,#22478,#5098,.T.) ;
#28614=EDGE_CURVE('',#22481,#22480,#1266,.T.) ;
#28615=EDGE_CURVE('',#22482,#22481,#5099,.T.) ;
#28616=EDGE_CURVE('',#22483,#22482,#5100,.T.) ;
#28617=EDGE_CURVE('',#22484,#22483,#5101,.T.) ;
#28618=EDGE_CURVE('',#22479,#22484,#5102,.T.) ;
#28619=EDGE_CURVE('',#22485,#22486,#5103,.T.) ;
#28620=EDGE_CURVE('',#22487,#22485,#5104,.T.) ;
#28621=EDGE_CURVE('',#22488,#22487,#5105,.T.) ;
#28622=EDGE_CURVE('',#22489,#22488,#1267,.T.) ;
#28623=EDGE_CURVE('',#22490,#22489,#5106,.T.) ;
#28624=EDGE_CURVE('',#22491,#22490,#1268,.T.) ;
#28625=EDGE_CURVE('',#22486,#22491,#5107,.T.) ;
#28626=EDGE_CURVE('',#22462,#22492,#5108,.T.) ;
#28627=EDGE_CURVE('',#22492,#22473,#18954,.F.) ;
#28628=EDGE_CURVE('',#22463,#22493,#5109,.T.) ;
#28629=EDGE_CURVE('',#22494,#22493,#5110,.T.) ;
#28630=EDGE_CURVE('',#22492,#22494,#463,.T.) ;
#28631=EDGE_CURVE('',#22495,#22472,#5111,.T.) ;
#28632=EDGE_CURVE('',#22495,#22138,#5112,.T.) ;
#28633=EDGE_CURVE('',#22496,#22137,#5113,.T.) ;
#28634=EDGE_CURVE('',#22493,#22496,#464,.T.) ;
#28635=EDGE_CURVE('',#22497,#22497,#18955,.T.) ;
#28636=EDGE_CURVE('',#22471,#22498,#5114,.T.) ;
#28637=EDGE_CURVE('',#22498,#22495,#18956,.T.) ;
#28638=EDGE_CURVE('',#22465,#22499,#5115,.T.) ;
#28639=EDGE_CURVE('',#22499,#22500,#5116,.T.) ;
#28640=EDGE_CURVE('',#22501,#22500,#5117,.T.) ;
#28641=EDGE_CURVE('',#22498,#22501,#5118,.T.) ;
#28642=EDGE_CURVE('',#22464,#22142,#5119,.T.) ;
#28643=EDGE_CURVE('',#22499,#22141,#5120,.T.) ;
#28644=EDGE_CURVE('',#22502,#22503,#465,.T.) ;
#28645=EDGE_CURVE('',#22504,#22503,#18957,.T.) ;
#28646=EDGE_CURVE('',#22505,#22504,#466,.F.) ;
#28647=EDGE_CURVE('',#22502,#22505,#18958,.T.) ;
#28648=EDGE_CURVE('',#22506,#22507,#467,.T.) ;
#28649=EDGE_CURVE('',#22508,#22507,#18959,.T.) ;
#28650=EDGE_CURVE('',#22509,#22508,#468,.F.) ;
#28651=EDGE_CURVE('',#22506,#22509,#18960,.T.) ;
#28652=EDGE_CURVE('',#22030,#22510,#5121,.T.) ;
#28653=EDGE_CURVE('',#22510,#22511,#18961,.T.) ;
#28654=EDGE_CURVE('',#22511,#22028,#5122,.T.) ;
#28655=EDGE_CURVE('',#22512,#22513,#18962,.T.) ;
#28656=EDGE_CURVE('',#22513,#22511,#1269,.T.) ;
#28657=EDGE_CURVE('',#22510,#22512,#1270,.T.) ;
#28658=EDGE_CURVE('',#22514,#22515,#18963,.T.) ;
#28659=EDGE_CURVE('',#22515,#22513,#18964,.T.) ;
#28660=EDGE_CURVE('',#22512,#22514,#18965,.T.) ;
#28661=EDGE_CURVE('',#22507,#22515,#5123,.T.) ;
#28662=EDGE_CURVE('',#22514,#22508,#5124,.T.) ;
#28663=EDGE_CURVE('',#22516,#22517,#18966,.T.) ;
#28664=EDGE_CURVE('',#22516,#22509,#5125,.T.) ;
#28665=EDGE_CURVE('',#22508,#22517,#5126,.T.) ;
#28666=EDGE_CURVE('',#22503,#22506,#5127,.T.) ;
#28667=EDGE_CURVE('',#22509,#22504,#5128,.T.) ;
#28668=EDGE_CURVE('',#22518,#22519,#18967,.T.) ;
#28669=EDGE_CURVE('',#22518,#22505,#5129,.T.) ;
#28670=EDGE_CURVE('',#22504,#22519,#5130,.T.) ;
#28671=EDGE_CURVE('',#22066,#22520,#18968,.T.) ;
#28672=EDGE_CURVE('',#22520,#22502,#5131,.T.) ;
#28673=EDGE_CURVE('',#22505,#22066,#5132,.T.) ;
#28674=EDGE_CURVE('',#22065,#22521,#18969,.T.) ;
#28675=EDGE_CURVE('',#22521,#22520,#469,.T.) ;
#28676=EDGE_CURVE('',#22072,#22521,#1271,.T.) ;
#28677=EDGE_CURVE('',#22029,#22522,#5133,.F.) ;
#28678=EDGE_CURVE('',#22522,#22523,#18970,.F.) ;
#28679=EDGE_CURVE('',#22523,#22512,#5134,.T.) ;
#28680=EDGE_CURVE('',#22026,#22511,#5135,.T.) ;
#28681=EDGE_CURVE('',#22515,#22040,#5136,.T.) ;
#28682=EDGE_CURVE('',#22524,#22521,#5137,.T.) ;
#28683=EDGE_CURVE('',#22524,#22525,#470,.T.) ;
#28684=EDGE_CURVE('',#22038,#22525,#5138,.T.) ;
#28685=EDGE_CURVE('',#22052,#22526,#18971,.T.) ;
#28686=EDGE_CURVE('',#22527,#22526,#471,.T.) ;
#28687=EDGE_CURVE('',#22527,#22528,#5139,.T.) ;
#28688=EDGE_CURVE('',#22528,#22524,#1272,.T.) ;
#28689=EDGE_CURVE('',#22529,#22530,#5140,.T.) ;
#28690=EDGE_CURVE('',#22530,#22068,#472,.F.) ;
#28691=EDGE_CURVE('',#22067,#22529,#473,.T.) ;
#28692=EDGE_CURVE('',#22061,#22531,#5141,.T.) ;
#28693=EDGE_CURVE('',#22531,#22532,#474,.T.) ;
#28694=EDGE_CURVE('',#22532,#22533,#5142,.T.) ;
#28695=EDGE_CURVE('',#22533,#22529,#475,.T.) ;
#28696=EDGE_CURVE('',#22530,#21924,#5143,.F.) ;
#28697=EDGE_CURVE('',#22534,#22533,#5144,.T.) ;
#28698=EDGE_CURVE('',#22534,#22535,#5145,.T.) ;
#28699=EDGE_CURVE('',#22536,#22535,#5146,.F.) ;
#28700=EDGE_CURVE('',#22536,#21830,#5147,.T.) ;
#28701=EDGE_CURVE('',#22532,#22537,#5148,.T.) ;
#28702=EDGE_CURVE('',#22534,#22537,#5149,.T.) ;
#28703=EDGE_CURVE('',#22537,#22518,#5150,.T.) ;
#28704=EDGE_CURVE('',#22063,#22531,#5151,.T.) ;
#28705=EDGE_CURVE('',#21835,#22538,#1273,.T.) ;
#28706=EDGE_CURVE('',#21854,#22538,#18972,.T.) ;
#28707=EDGE_CURVE('',#21931,#21856,#18973,.T.) ;
#28708=EDGE_CURVE('',#21855,#21932,#18974,.T.) ;
#28709=EDGE_CURVE('',#22538,#21932,#476,.T.) ;
#28710=EDGE_CURVE('',#22539,#21857,#18975,.T.) ;
#28711=EDGE_CURVE('',#21931,#22539,#1274,.T.) ;
#28712=EDGE_CURVE('',#22540,#21858,#18976,.T.) ;
#28713=EDGE_CURVE('',#22539,#22540,#477,.T.) ;
#28714=EDGE_CURVE('',#22541,#21968,#1275,.T.) ;
#28715=EDGE_CURVE('',#22540,#22541,#1276,.T.) ;
#28716=EDGE_CURVE('',#21834,#21927,#5152,.T.) ;
#28717=EDGE_CURVE('',#21865,#22542,#1277,.F.) ;
#28718=EDGE_CURVE('',#22542,#22543,#5153,.T.) ;
#28719=EDGE_CURVE('',#22543,#22544,#1278,.F.) ;
#28720=EDGE_CURVE('',#22544,#22545,#5154,.T.) ;
#28721=EDGE_CURVE('',#22546,#22545,#478,.T.) ;
#28722=EDGE_CURVE('',#21832,#22546,#5155,.T.) ;
#28723=EDGE_CURVE('',#22546,#21822,#479,.T.) ;
#28724=EDGE_CURVE('',#22545,#22547,#18977,.T.) ;
#28725=EDGE_CURVE('',#22547,#21925,#480,.T.) ;
#28726=EDGE_CURVE('',#22548,#22549,#18978,.T.) ;
#28727=EDGE_CURVE('',#22549,#22547,#5156,.T.) ;
#28728=EDGE_CURVE('',#22545,#22548,#5157,.T.) ;
#28729=EDGE_CURVE('',#22550,#22069,#18979,.T.) ;
#28730=EDGE_CURVE('',#22069,#22549,#481,.T.) ;
#28731=EDGE_CURVE('',#22548,#22550,#482,.T.) ;
#28732=EDGE_CURVE('',#22550,#22551,#483,.T.) ;
#28733=EDGE_CURVE('',#22551,#22070,#1279,.F.) ;
#28734=EDGE_CURVE('',#22552,#22444,#5158,.T.) ;
#28735=EDGE_CURVE('',#22552,#22553,#18980,.T.) ;
#28736=EDGE_CURVE('',#22553,#22554,#5159,.T.) ;
#28737=EDGE_CURVE('',#22554,#22555,#5160,.T.) ;
#28738=EDGE_CURVE('',#22555,#22556,#5161,.T.) ;
#28739=EDGE_CURVE('',#22556,#22528,#18981,.T.) ;
#28740=EDGE_CURVE('',#22557,#22527,#5162,.T.) ;
#28741=EDGE_CURVE('',#22443,#22557,#5163,.T.) ;
#28742=EDGE_CURVE('',#22558,#22559,#5164,.T.) ;
#28743=EDGE_CURVE('',#22560,#22558,#18982,.T.) ;
#28744=EDGE_CURVE('',#22561,#22560,#5165,.T.) ;
#28745=EDGE_CURVE('',#22562,#22561,#5166,.T.) ;
#28746=EDGE_CURVE('',#22563,#22562,#5167,.T.) ;
#28747=EDGE_CURVE('',#22564,#22563,#18983,.T.) ;
#28748=EDGE_CURVE('',#22565,#22564,#5168,.T.) ;
#28749=EDGE_CURVE('',#22566,#22565,#5169,.T.) ;
#28750=EDGE_CURVE('',#22567,#22566,#5170,.T.) ;
#28751=EDGE_CURVE('',#22568,#22567,#5171,.T.) ;
#28752=EDGE_CURVE('',#22559,#22568,#5172,.T.) ;
#28753=EDGE_CURVE('',#22569,#22570,#5173,.T.) ;
#28754=EDGE_CURVE('',#22571,#22570,#5174,.T.) ;
#28755=EDGE_CURVE('',#22572,#22571,#18984,.T.) ;
#28756=EDGE_CURVE('',#22573,#22572,#5175,.T.) ;
#28757=EDGE_CURVE('',#22574,#22573,#5176,.T.) ;
#28758=EDGE_CURVE('',#22575,#22574,#5177,.T.) ;
#28759=EDGE_CURVE('',#22576,#22575,#5178,.T.) ;
#28760=EDGE_CURVE('',#22577,#22576,#5179,.T.) ;
#28761=EDGE_CURVE('',#22578,#22577,#5180,.T.) ;
#28762=EDGE_CURVE('',#22579,#22578,#18985,.T.) ;
#28763=EDGE_CURVE('',#22569,#22579,#5181,.T.) ;
#28764=EDGE_CURVE('',#22580,#22581,#5182,.T.) ;
#28765=EDGE_CURVE('',#22582,#22580,#5183,.T.) ;
#28766=EDGE_CURVE('',#22583,#22582,#5184,.T.) ;
#28767=EDGE_CURVE('',#22581,#22583,#5185,.T.) ;
#28768=EDGE_CURVE('',#22551,#22557,#484,.T.) ;
#28769=EDGE_CURVE('',#22548,#22442,#5186,.T.) ;
#28770=EDGE_CURVE('',#22584,#22544,#485,.T.) ;
#28771=EDGE_CURVE('',#22441,#22584,#5187,.T.) ;
#28772=EDGE_CURVE('',#22527,#22071,#18986,.T.) ;
#28773=EDGE_CURVE('',#22585,#21933,#486,.F.) ;
#28774=EDGE_CURVE('',#22539,#22585,#18987,.T.) ;
#28775=EDGE_CURVE('',#22585,#22586,#5188,.T.) ;
#28776=EDGE_CURVE('',#22586,#22541,#1280,.T.) ;
#28777=EDGE_CURVE('',#21937,#22587,#487,.F.) ;
#28778=EDGE_CURVE('',#22587,#22585,#5189,.T.) ;
#28779=EDGE_CURVE('',#22588,#22586,#5190,.T.) ;
#28780=EDGE_CURVE('',#22588,#21963,#18988,.T.) ;
#28781=EDGE_CURVE('',#21964,#22589,#18989,.F.) ;
#28782=EDGE_CURVE('',#22589,#22588,#5191,.F.) ;
#28783=EDGE_CURVE('',#22589,#22023,#5192,.T.) ;
#28784=EDGE_CURVE('',#22590,#22587,#5193,.T.) ;
#28785=EDGE_CURVE('',#22031,#22590,#488,.T.) ;
#28786=EDGE_CURVE('',#22591,#21828,#5194,.F.) ;
#28787=EDGE_CURVE('',#22591,#21849,#5195,.F.) ;
#28788=EDGE_CURVE('',#21826,#22536,#5196,.T.) ;
#28789=EDGE_CURVE('',#21827,#22535,#5197,.T.) ;
#28790=EDGE_CURVE('',#21786,#22592,#1281,.T.) ;
#28791=EDGE_CURVE('',#22592,#22450,#5198,.T.) ;
#28792=EDGE_CURVE('',#22525,#21785,#1282,.T.) ;
#28793=EDGE_CURVE('',#22556,#22593,#5199,.T.) ;
#28794=EDGE_CURVE('',#22593,#22594,#18990,.T.) ;
#28795=EDGE_CURVE('',#22553,#22594,#5200,.T.) ;
#28796=EDGE_CURVE('',#22595,#22552,#1283,.T.) ;
#28797=EDGE_CURVE('',#22592,#22595,#489,.T.) ;
#28798=EDGE_CURVE('',#22445,#22595,#5201,.T.) ;
#28799=EDGE_CURVE('',#22517,#22523,#5202,.T.) ;
#28800=EDGE_CURVE('',#22596,#22597,#5203,.T.) ;
#28801=EDGE_CURVE('',#22598,#22596,#5204,.T.) ;
#28802=EDGE_CURVE('',#22599,#22598,#5205,.T.) ;
#28803=EDGE_CURVE('',#22599,#22153,#5206,.T.) ;
#28804=EDGE_CURVE('',#22597,#22152,#5207,.T.) ;
#28805=EDGE_CURVE('',#22600,#22599,#18991,.T.) ;
#28806=EDGE_CURVE('',#22154,#22600,#5208,.T.) ;
#28807=EDGE_CURVE('',#22601,#22157,#5209,.T.) ;
#28808=EDGE_CURVE('',#22601,#22602,#5210,.T.) ;
#28809=EDGE_CURVE('',#22602,#22158,#5211,.T.) ;
#28810=EDGE_CURVE('',#22602,#22086,#1284,.T.) ;
#28811=EDGE_CURVE('',#22603,#22596,#18992,.T.) ;
#28812=EDGE_CURVE('',#22604,#22603,#5212,.T.) ;
#28813=EDGE_CURVE('',#22598,#22604,#18993,.T.) ;
#28814=EDGE_CURVE('',#22605,#22156,#5213,.T.) ;
#28815=EDGE_CURVE('',#22601,#22605,#18994,.T.) ;
#28816=EDGE_CURVE('',#22606,#22151,#5214,.T.) ;
#28817=EDGE_CURVE('',#22606,#22597,#5215,.T.) ;
#28818=EDGE_CURVE('',#22155,#22607,#5216,.T.) ;
#28819=EDGE_CURVE('',#22607,#22605,#5217,.F.) ;
#28820=EDGE_CURVE('',#22600,#22607,#5218,.F.) ;
#28821=EDGE_CURVE('',#22608,#22604,#5219,.F.) ;
#28822=EDGE_CURVE('',#22609,#22608,#5220,.T.) ;
#28823=EDGE_CURVE('',#22610,#22609,#18995,.T.) ;
#28824=EDGE_CURVE('',#22611,#22610,#5221,.T.) ;
#28825=EDGE_CURVE('',#22092,#22611,#18996,.T.) ;
#28826=EDGE_CURVE('',#22079,#22612,#5222,.T.) ;
#28827=EDGE_CURVE('',#22612,#22078,#5223,.T.) ;
#28828=EDGE_CURVE('',#22609,#22044,#18997,.T.) ;
#28829=EDGE_CURVE('',#22047,#22610,#490,.T.) ;
#28830=EDGE_CURVE('',#22455,#22611,#18998,.T.) ;
#28831=EDGE_CURVE('',#22608,#22045,#491,.F.) ;
#28832=EDGE_CURVE('',#22046,#22603,#5224,.T.) ;
#28833=EDGE_CURVE('',#22613,#22388,#5225,.T.) ;
#28834=EDGE_CURVE('',#22614,#22613,#5226,.T.) ;
#28835=EDGE_CURVE('',#22385,#22614,#5227,.T.) ;
#28836=EDGE_CURVE('',#22615,#22392,#5228,.T.) ;
#28837=EDGE_CURVE('',#22616,#22615,#5229,.T.) ;
#28838=EDGE_CURVE('',#22391,#22616,#5230,.T.) ;
#28839=EDGE_CURVE('',#22616,#22613,#5231,.T.) ;
#28840=EDGE_CURVE('',#22614,#22615,#5232,.T.) ;
#28841=EDGE_CURVE('',#22409,#22415,#5233,.T.) ;
#28842=EDGE_CURVE('',#22407,#22410,#5234,.T.) ;
#28843=EDGE_CURVE('',#22404,#22408,#5235,.T.) ;
#28844=EDGE_CURVE('',#22617,#22618,#5236,.T.) ;
#28845=EDGE_CURVE('',#22618,#22619,#1285,.T.) ;
#28846=EDGE_CURVE('',#22619,#22620,#5237,.T.) ;
#28847=EDGE_CURVE('',#22617,#22620,#492,.T.) ;
#28848=EDGE_CURVE('',#22618,#22621,#1286,.T.) ;
#28849=EDGE_CURVE('',#22621,#22622,#1287,.T.) ;
#28850=EDGE_CURVE('',#22622,#22619,#1288,.T.) ;
#28851=EDGE_CURVE('',#22621,#22623,#5238,.T.) ;
#28852=EDGE_CURVE('',#22623,#22624,#1289,.T.) ;
#28853=EDGE_CURVE('',#22624,#22622,#5239,.T.) ;
#28854=EDGE_CURVE('',#22625,#22624,#1290,.T.) ;
#28855=EDGE_CURVE('',#22623,#22626,#1291,.T.) ;
#28856=EDGE_CURVE('',#22626,#22625,#1292,.T.) ;
#28857=EDGE_CURVE('',#22627,#22625,#5240,.T.) ;
#28858=EDGE_CURVE('',#22626,#22628,#5241,.T.) ;
#28859=EDGE_CURVE('',#22628,#22627,#493,.T.) ;
#28860=EDGE_CURVE('',#22629,#22627,#5242,.T.) ;
#28861=EDGE_CURVE('',#22628,#22630,#5243,.T.) ;
#28862=EDGE_CURVE('',#22630,#22629,#494,.T.) ;
#28863=EDGE_CURVE('',#22620,#22629,#5244,.T.) ;
#28864=EDGE_CURVE('',#22630,#22617,#5245,.T.) ;
#28865=EDGE_CURVE('',#22631,#22627,#5246,.T.) ;
#28866=EDGE_CURVE('',#22632,#22631,#5247,.T.) ;
#28867=EDGE_CURVE('',#22632,#22625,#5248,.T.) ;
#28868=EDGE_CURVE('',#22633,#22629,#5249,.T.) ;
#28869=EDGE_CURVE('',#22631,#22633,#5250,.T.) ;
#28870=EDGE_CURVE('',#22634,#22620,#5251,.T.) ;
#28871=EDGE_CURVE('',#22633,#22634,#5252,.T.) ;
#28872=EDGE_CURVE('',#22635,#22619,#5253,.T.) ;
#28873=EDGE_CURVE('',#22634,#22635,#5254,.T.) ;
#28874=EDGE_CURVE('',#22636,#22637,#1293,.T.) ;
#28875=EDGE_CURVE('',#22637,#22638,#1294,.T.) ;
#28876=EDGE_CURVE('',#22638,#22639,#1295,.T.) ;
#28877=EDGE_CURVE('',#22636,#22639,#1296,.T.) ;
#28878=EDGE_CURVE('',#22637,#22640,#5255,.T.) ;
#28879=EDGE_CURVE('',#22640,#22641,#495,.T.) ;
#28880=EDGE_CURVE('',#22641,#22638,#5256,.T.) ;
#28881=EDGE_CURVE('',#22640,#22642,#5257,.T.) ;
#28882=EDGE_CURVE('',#22642,#22643,#496,.T.) ;
#28883=EDGE_CURVE('',#22643,#22641,#5258,.T.) ;
#28884=EDGE_CURVE('',#22644,#22643,#5259,.T.) ;
#28885=EDGE_CURVE('',#22642,#22645,#5260,.T.) ;
#28886=EDGE_CURVE('',#22645,#22644,#497,.T.) ;
#28887=EDGE_CURVE('',#22646,#22644,#5261,.T.) ;
#28888=EDGE_CURVE('',#22645,#22647,#5262,.T.) ;
#28889=EDGE_CURVE('',#22647,#22646,#1297,.T.) ;
#28890=EDGE_CURVE('',#22648,#22646,#1298,.T.) ;
#28891=EDGE_CURVE('',#22647,#22649,#1299,.T.) ;
#28892=EDGE_CURVE('',#22649,#22648,#1300,.T.) ;
#28893=EDGE_CURVE('',#22639,#22648,#5263,.T.) ;
#28894=EDGE_CURVE('',#22649,#22636,#5264,.T.) ;
#28895=EDGE_CURVE('',#22650,#22646,#5265,.T.) ;
#28896=EDGE_CURVE('',#22651,#22650,#5266,.T.) ;
#28897=EDGE_CURVE('',#22651,#22644,#5267,.T.) ;
#28898=EDGE_CURVE('',#22652,#22648,#5268,.T.) ;
#28899=EDGE_CURVE('',#22650,#22652,#1301,.T.) ;
#28900=EDGE_CURVE('',#22653,#22639,#5269,.T.) ;
#28901=EDGE_CURVE('',#22652,#22653,#5270,.T.) ;
#28902=EDGE_CURVE('',#22654,#22638,#5271,.T.) ;
#28903=EDGE_CURVE('',#22653,#22654,#1302,.T.) ;
#28904=EDGE_CURVE('',#22655,#22656,#5272,.T.) ;
#28905=EDGE_CURVE('',#22656,#22657,#498,.T.) ;
#28906=EDGE_CURVE('',#22657,#22658,#5273,.T.) ;
#28907=EDGE_CURVE('',#22655,#22658,#499,.T.) ;
#28908=EDGE_CURVE('',#22656,#22659,#5274,.T.) ;
#28909=EDGE_CURVE('',#22659,#22660,#500,.T.) ;
#28910=EDGE_CURVE('',#22660,#22657,#5275,.T.) ;
#28911=EDGE_CURVE('',#22659,#22661,#5276,.T.) ;
#28912=EDGE_CURVE('',#22661,#22662,#501,.T.) ;
#28913=EDGE_CURVE('',#22662,#22660,#5277,.T.) ;
#28914=EDGE_CURVE('',#22663,#22662,#5278,.T.) ;
#28915=EDGE_CURVE('',#22661,#22664,#5279,.T.) ;
#28916=EDGE_CURVE('',#22664,#22663,#502,.T.) ;
#28917=EDGE_CURVE('',#22665,#22663,#5280,.T.) ;
#28918=EDGE_CURVE('',#22664,#22666,#5281,.T.) ;
#28919=EDGE_CURVE('',#22666,#22665,#503,.T.) ;
#28920=EDGE_CURVE('',#22667,#22665,#5282,.T.) ;
#28921=EDGE_CURVE('',#22666,#22668,#5283,.T.) ;
#28922=EDGE_CURVE('',#22668,#22667,#504,.T.) ;
#28923=EDGE_CURVE('',#22658,#22667,#5284,.T.) ;
#28924=EDGE_CURVE('',#22668,#22655,#5285,.T.) ;
#28925=EDGE_CURVE('',#22669,#22665,#5286,.T.) ;
#28926=EDGE_CURVE('',#22670,#22669,#5287,.T.) ;
#28927=EDGE_CURVE('',#22670,#22663,#5288,.T.) ;
#28928=EDGE_CURVE('',#22671,#22667,#5289,.T.) ;
#28929=EDGE_CURVE('',#22669,#22671,#5290,.T.) ;
#28930=EDGE_CURVE('',#22672,#22658,#5291,.T.) ;
#28931=EDGE_CURVE('',#22671,#22672,#5292,.T.) ;
#28932=EDGE_CURVE('',#22673,#22657,#5293,.T.) ;
#28933=EDGE_CURVE('',#22672,#22673,#5294,.T.) ;
#28934=EDGE_CURVE('',#22674,#22675,#5295,.T.) ;
#28935=EDGE_CURVE('',#22675,#22676,#505,.T.) ;
#28936=EDGE_CURVE('',#22676,#22677,#5296,.T.) ;
#28937=EDGE_CURVE('',#22674,#22677,#506,.T.) ;
#28938=EDGE_CURVE('',#22678,#22676,#5297,.T.) ;
#28939=EDGE_CURVE('',#22675,#22679,#5298,.T.) ;
#28940=EDGE_CURVE('',#22679,#22678,#507,.T.) ;
#28941=EDGE_CURVE('',#22680,#22678,#5299,.T.) ;
#28942=EDGE_CURVE('',#22679,#22681,#5300,.T.) ;
#28943=EDGE_CURVE('',#22681,#22680,#508,.T.) ;
#28944=EDGE_CURVE('',#22677,#22680,#5301,.T.) ;
#28945=EDGE_CURVE('',#22681,#22674,#5302,.T.) ;
#28946=EDGE_CURVE('',#22682,#22677,#5303,.T.) ;
#28947=EDGE_CURVE('',#22683,#22682,#5304,.T.) ;
#28948=EDGE_CURVE('',#22683,#22680,#5305,.T.) ;
#28949=EDGE_CURVE('',#22684,#22676,#5306,.T.) ;
#28950=EDGE_CURVE('',#22682,#22684,#5307,.T.) ;
#28951=EDGE_CURVE('',#22685,#22686,#5308,.T.) ;
#28952=EDGE_CURVE('',#22686,#22687,#509,.T.) ;
#28953=EDGE_CURVE('',#22687,#22688,#5309,.T.) ;
#28954=EDGE_CURVE('',#22685,#22688,#510,.T.) ;
#28955=EDGE_CURVE('',#22686,#22689,#5310,.T.) ;
#28956=EDGE_CURVE('',#22689,#22690,#511,.T.) ;
#28957=EDGE_CURVE('',#22690,#22687,#5311,.T.) ;
#28958=EDGE_CURVE('',#22689,#22691,#5312,.T.) ;
#28959=EDGE_CURVE('',#22691,#22692,#512,.T.) ;
#28960=EDGE_CURVE('',#22692,#22690,#5313,.T.) ;
#28961=EDGE_CURVE('',#22693,#22692,#5314,.T.) ;
#28962=EDGE_CURVE('',#22691,#22694,#5315,.T.) ;
#28963=EDGE_CURVE('',#22694,#22693,#513,.T.) ;
#28964=EDGE_CURVE('',#22695,#22693,#5316,.T.) ;
#28965=EDGE_CURVE('',#22694,#22696,#5317,.T.) ;
#28966=EDGE_CURVE('',#22696,#22695,#514,.T.) ;
#28967=EDGE_CURVE('',#22697,#22695,#5318,.T.) ;
#28968=EDGE_CURVE('',#22696,#22698,#5319,.T.) ;
#28969=EDGE_CURVE('',#22698,#22697,#515,.T.) ;
#28970=EDGE_CURVE('',#22688,#22697,#5320,.T.) ;
#28971=EDGE_CURVE('',#22698,#22685,#5321,.T.) ;
#28972=EDGE_CURVE('',#22699,#22695,#5322,.T.) ;
#28973=EDGE_CURVE('',#22700,#22699,#5323,.T.) ;
#28974=EDGE_CURVE('',#22700,#22693,#5324,.T.) ;
#28975=EDGE_CURVE('',#22701,#22697,#5325,.T.) ;
#28976=EDGE_CURVE('',#22699,#22701,#5326,.T.) ;
#28977=EDGE_CURVE('',#22702,#22688,#5327,.T.) ;
#28978=EDGE_CURVE('',#22701,#22702,#5328,.T.) ;
#28979=EDGE_CURVE('',#22703,#22687,#5329,.T.) ;
#28980=EDGE_CURVE('',#22702,#22703,#5330,.T.) ;
#28981=EDGE_CURVE('',#22704,#22705,#5331,.T.) ;
#28982=EDGE_CURVE('',#22705,#22706,#516,.T.) ;
#28983=EDGE_CURVE('',#22706,#22707,#5332,.T.) ;
#28984=EDGE_CURVE('',#22704,#22707,#517,.T.) ;
#28985=EDGE_CURVE('',#22708,#22706,#5333,.T.) ;
#28986=EDGE_CURVE('',#22705,#22709,#5334,.T.) ;
#28987=EDGE_CURVE('',#22709,#22708,#518,.T.) ;
#28988=EDGE_CURVE('',#22710,#22708,#5335,.T.) ;
#28989=EDGE_CURVE('',#22709,#22711,#5336,.T.) ;
#28990=EDGE_CURVE('',#22711,#22710,#519,.T.) ;
#28991=EDGE_CURVE('',#22707,#22710,#5337,.T.) ;
#28992=EDGE_CURVE('',#22711,#22704,#5338,.T.) ;
#28993=EDGE_CURVE('',#22712,#22707,#5339,.T.) ;
#28994=EDGE_CURVE('',#22713,#22712,#5340,.T.) ;
#28995=EDGE_CURVE('',#22713,#22710,#5341,.T.) ;
#28996=EDGE_CURVE('',#22714,#22706,#5342,.T.) ;
#28997=EDGE_CURVE('',#22712,#22714,#5343,.T.) ;
#28998=EDGE_CURVE('',#22715,#22716,#5344,.T.) ;
#28999=EDGE_CURVE('',#22716,#22717,#520,.T.) ;
#29000=EDGE_CURVE('',#22717,#22718,#5345,.T.) ;
#29001=EDGE_CURVE('',#22715,#22718,#521,.T.) ;
#29002=EDGE_CURVE('',#22716,#22719,#5346,.T.) ;
#29003=EDGE_CURVE('',#22719,#22720,#522,.T.) ;
#29004=EDGE_CURVE('',#22720,#22717,#5347,.T.) ;
#29005=EDGE_CURVE('',#22719,#22721,#5348,.T.) ;
#29006=EDGE_CURVE('',#22721,#22722,#18999,.T.) ;
#29007=EDGE_CURVE('',#22722,#22720,#5349,.T.) ;
#29008=EDGE_CURVE('',#22723,#22724,#19000,.T.) ;
#29009=EDGE_CURVE('',#22724,#22722,#19001,.T.) ;
#29010=EDGE_CURVE('',#22721,#22723,#19002,.T.) ;
#29011=EDGE_CURVE('',#22725,#22724,#5350,.T.) ;
#29012=EDGE_CURVE('',#22723,#22726,#5351,.T.) ;
#29013=EDGE_CURVE('',#22726,#22725,#523,.T.) ;
#29014=EDGE_CURVE('',#22727,#22725,#5352,.T.) ;
#29015=EDGE_CURVE('',#22726,#22728,#5353,.T.) ;
#29016=EDGE_CURVE('',#22728,#22727,#524,.T.) ;
#29017=EDGE_CURVE('',#22728,#22729,#5354,.T.) ;
#29018=EDGE_CURVE('',#22729,#22730,#19003,.T.) ;
#29019=EDGE_CURVE('',#22730,#22727,#5355,.T.) ;
#29020=EDGE_CURVE('',#22731,#22732,#19004,.T.) ;
#29021=EDGE_CURVE('',#22732,#22730,#19005,.T.) ;
#29022=EDGE_CURVE('',#22729,#22731,#19006,.T.) ;
#29023=EDGE_CURVE('',#22733,#22732,#5356,.T.) ;
#29024=EDGE_CURVE('',#22731,#22734,#5357,.T.) ;
#29025=EDGE_CURVE('',#22734,#22733,#525,.T.) ;
#29026=EDGE_CURVE('',#22735,#22733,#5358,.T.) ;
#29027=EDGE_CURVE('',#22734,#22736,#5359,.T.) ;
#29028=EDGE_CURVE('',#22736,#22735,#526,.T.) ;
#29029=EDGE_CURVE('',#22718,#22735,#5360,.T.) ;
#29030=EDGE_CURVE('',#22736,#22715,#5361,.T.) ;
#29031=EDGE_CURVE('',#22737,#22730,#5362,.T.) ;
#29032=EDGE_CURVE('',#22738,#22737,#5363,.T.) ;
#29033=EDGE_CURVE('',#22738,#22727,#5364,.T.) ;
#29034=EDGE_CURVE('',#22739,#22732,#5365,.T.) ;
#29035=EDGE_CURVE('',#22737,#22739,#19007,.T.) ;
#29036=EDGE_CURVE('',#22740,#22733,#5366,.T.) ;
#29037=EDGE_CURVE('',#22739,#22740,#5367,.T.) ;
#29038=EDGE_CURVE('',#22741,#22735,#5368,.T.) ;
#29039=EDGE_CURVE('',#22740,#22741,#5369,.T.) ;
#29040=EDGE_CURVE('',#22742,#22718,#5370,.T.) ;
#29041=EDGE_CURVE('',#22741,#22742,#5371,.T.) ;
#29042=EDGE_CURVE('',#22743,#22717,#5372,.T.) ;
#29043=EDGE_CURVE('',#22742,#22743,#5373,.T.) ;
#29044=EDGE_CURVE('',#22744,#22745,#5374,.T.) ;
#29045=EDGE_CURVE('',#22745,#22746,#527,.T.) ;
#29046=EDGE_CURVE('',#22746,#22747,#5375,.T.) ;
#29047=EDGE_CURVE('',#22744,#22747,#528,.T.) ;
#29048=EDGE_CURVE('',#22745,#22748,#5376,.T.) ;
#29049=EDGE_CURVE('',#22748,#22749,#19008,.T.) ;
#29050=EDGE_CURVE('',#22749,#22746,#5377,.T.) ;
#29051=EDGE_CURVE('',#22750,#22751,#19009,.T.) ;
#29052=EDGE_CURVE('',#22751,#22749,#19010,.T.) ;
#29053=EDGE_CURVE('',#22748,#22750,#19011,.T.) ;
#29054=EDGE_CURVE('',#22752,#22751,#5378,.T.) ;
#29055=EDGE_CURVE('',#22750,#22753,#5379,.T.) ;
#29056=EDGE_CURVE('',#22753,#22752,#529,.T.) ;
#29057=EDGE_CURVE('',#22753,#22754,#5380,.T.) ;
#29058=EDGE_CURVE('',#22754,#22755,#530,.T.) ;
#29059=EDGE_CURVE('',#22755,#22752,#5381,.T.) ;
#29060=EDGE_CURVE('',#22754,#22756,#5382,.T.) ;
#29061=EDGE_CURVE('',#22756,#22757,#19012,.T.) ;
#29062=EDGE_CURVE('',#22757,#22755,#5383,.T.) ;
#29063=EDGE_CURVE('',#22758,#22759,#19013,.T.) ;
#29064=EDGE_CURVE('',#22759,#22757,#19014,.T.) ;
#29065=EDGE_CURVE('',#22756,#22758,#19015,.T.) ;
#29066=EDGE_CURVE('',#22760,#22759,#5384,.T.) ;
#29067=EDGE_CURVE('',#22758,#22761,#5385,.T.) ;
#29068=EDGE_CURVE('',#22761,#22760,#531,.T.) ;
#29069=EDGE_CURVE('',#22762,#22760,#5386,.T.) ;
#29070=EDGE_CURVE('',#22761,#22763,#5387,.T.) ;
#29071=EDGE_CURVE('',#22763,#22762,#532,.T.) ;
#29072=EDGE_CURVE('',#22764,#22762,#5388,.T.) ;
#29073=EDGE_CURVE('',#22763,#22765,#5389,.T.) ;
#29074=EDGE_CURVE('',#22765,#22764,#533,.T.) ;
#29075=EDGE_CURVE('',#22747,#22764,#5390,.T.) ;
#29076=EDGE_CURVE('',#22765,#22744,#5391,.T.) ;
#29077=EDGE_CURVE('',#22766,#22759,#5392,.T.) ;
#29078=EDGE_CURVE('',#22767,#22766,#19016,.T.) ;
#29079=EDGE_CURVE('',#22767,#22757,#5393,.T.) ;
#29080=EDGE_CURVE('',#22768,#22760,#5394,.T.) ;
#29081=EDGE_CURVE('',#22766,#22768,#5395,.T.) ;
#29082=EDGE_CURVE('',#22769,#22762,#5396,.T.) ;
#29083=EDGE_CURVE('',#22768,#22769,#5397,.T.) ;
#29084=EDGE_CURVE('',#22770,#22764,#5398,.T.) ;
#29085=EDGE_CURVE('',#22769,#22770,#5399,.T.) ;
#29086=EDGE_CURVE('',#22771,#22747,#5400,.T.) ;
#29087=EDGE_CURVE('',#22770,#22771,#5401,.T.) ;
#29088=EDGE_CURVE('',#22772,#22746,#5402,.T.) ;
#29089=EDGE_CURVE('',#22771,#22772,#5403,.T.) ;
#29090=EDGE_CURVE('',#22479,#22635,#1303,.T.) ;
#29091=EDGE_CURVE('',#22635,#22773,#1304,.T.) ;
#29092=EDGE_CURVE('',#22478,#22773,#1305,.T.) ;
#29093=EDGE_CURVE('',#22773,#22774,#5404,.T.) ;
#29094=EDGE_CURVE('',#22774,#22480,#1306,.T.) ;
#29095=EDGE_CURVE('',#22484,#22634,#534,.T.) ;
#29096=EDGE_CURVE('',#22483,#22633,#535,.T.) ;
#29097=EDGE_CURVE('',#22482,#22631,#536,.T.) ;
#29098=EDGE_CURVE('',#22481,#22632,#1307,.T.) ;
#29099=EDGE_CURVE('',#22774,#22632,#1308,.T.) ;
#29100=EDGE_CURVE('',#22774,#22624,#5405,.T.) ;
#29101=EDGE_CURVE('',#22773,#22622,#5406,.T.) ;
#29102=EDGE_CURVE('',#22488,#22650,#1309,.T.) ;
#29103=EDGE_CURVE('',#22489,#22652,#1310,.T.) ;
#29104=EDGE_CURVE('',#22487,#22651,#537,.T.) ;
#29105=EDGE_CURVE('',#22486,#22775,#538,.T.) ;
#29106=EDGE_CURVE('',#22775,#22776,#5407,.T.) ;
#29107=EDGE_CURVE('',#22776,#22485,#539,.T.) ;
#29108=EDGE_CURVE('',#22654,#22775,#5408,.T.) ;
#29109=EDGE_CURVE('',#22491,#22654,#1311,.T.) ;
#29110=EDGE_CURVE('',#22776,#22651,#5409,.T.) ;
#29111=EDGE_CURVE('',#22490,#22653,#1312,.T.) ;
#29112=EDGE_CURVE('',#22776,#22643,#5410,.T.) ;
#29113=EDGE_CURVE('',#22775,#22641,#5411,.T.) ;
#29114=EDGE_CURVE('',#22777,#22778,#5412,.T.) ;
#29115=EDGE_CURVE('',#22778,#22673,#540,.T.) ;
#29116=EDGE_CURVE('',#22673,#22779,#5413,.T.) ;
#29117=EDGE_CURVE('',#22777,#22779,#541,.T.) ;
#29118=EDGE_CURVE('',#22779,#22780,#5414,.T.) ;
#29119=EDGE_CURVE('',#22780,#22781,#542,.T.) ;
#29120=EDGE_CURVE('',#22781,#22777,#5415,.T.) ;
#29121=EDGE_CURVE('',#22778,#22782,#5416,.T.) ;
#29122=EDGE_CURVE('',#22782,#22672,#543,.T.) ;
#29123=EDGE_CURVE('',#22782,#22783,#5417,.T.) ;
#29124=EDGE_CURVE('',#22783,#22671,#544,.T.) ;
#29125=EDGE_CURVE('',#22783,#22784,#5418,.T.) ;
#29126=EDGE_CURVE('',#22784,#22669,#545,.T.) ;
#29127=EDGE_CURVE('',#22784,#22785,#5419,.T.) ;
#29128=EDGE_CURVE('',#22785,#22670,#546,.T.) ;
#29129=EDGE_CURVE('',#22780,#22670,#5420,.T.) ;
#29130=EDGE_CURVE('',#22785,#22781,#5421,.T.) ;
#29131=EDGE_CURVE('',#22780,#22662,#5422,.T.) ;
#29132=EDGE_CURVE('',#22779,#22660,#5423,.T.) ;
#29133=EDGE_CURVE('',#22786,#22787,#5424,.T.) ;
#29134=EDGE_CURVE('',#22788,#22786,#19017,.T.) ;
#29135=EDGE_CURVE('',#22789,#22788,#5425,.T.) ;
#29136=EDGE_CURVE('',#22543,#22789,#19018,.T.) ;
#29137=EDGE_CURVE('',#22790,#22542,#19019,.T.) ;
#29138=EDGE_CURVE('',#22791,#22790,#5426,.T.) ;
#29139=EDGE_CURVE('',#22792,#22791,#19020,.T.) ;
#29140=EDGE_CURVE('',#21728,#22792,#5427,.T.) ;
#29141=EDGE_CURVE('',#22793,#21727,#1313,.T.) ;
#29142=EDGE_CURVE('',#22794,#22793,#5428,.T.) ;
#29143=EDGE_CURVE('',#22787,#22794,#19021,.T.) ;
#29144=EDGE_CURVE('',#22795,#22796,#5429,.T.) ;
#29145=EDGE_CURVE('',#22797,#22795,#5430,.T.) ;
#29146=EDGE_CURVE('',#22798,#22797,#5431,.T.) ;
#29147=EDGE_CURVE('',#22796,#22798,#5432,.T.) ;
#29148=EDGE_CURVE('',#22799,#22800,#5433,.T.) ;
#29149=EDGE_CURVE('',#22801,#22799,#5434,.T.) ;
#29150=EDGE_CURVE('',#22802,#22801,#5435,.T.) ;
#29151=EDGE_CURVE('',#22803,#22802,#5436,.T.) ;
#29152=EDGE_CURVE('',#22804,#22803,#5437,.T.) ;
#29153=EDGE_CURVE('',#22805,#22804,#5438,.T.) ;
#29154=EDGE_CURVE('',#22800,#22805,#5439,.T.) ;
#29155=EDGE_CURVE('',#22796,#22682,#547,.T.) ;
#29156=EDGE_CURVE('',#22684,#22795,#548,.T.) ;
#29157=EDGE_CURVE('',#22798,#22683,#549,.T.) ;
#29158=EDGE_CURVE('',#22806,#22683,#5440,.T.) ;
#29159=EDGE_CURVE('',#22797,#22806,#550,.T.) ;
#29160=EDGE_CURVE('',#22684,#22806,#5441,.T.) ;
#29161=EDGE_CURVE('',#22806,#22678,#5442,.T.) ;
#29162=EDGE_CURVE('',#22800,#22807,#551,.T.) ;
#29163=EDGE_CURVE('',#22807,#22808,#5443,.T.) ;
#29164=EDGE_CURVE('',#22808,#22799,#552,.T.) ;
#29165=EDGE_CURVE('',#22805,#22703,#553,.T.) ;
#29166=EDGE_CURVE('',#22703,#22807,#5444,.T.) ;
#29167=EDGE_CURVE('',#22804,#22702,#554,.T.) ;
#29168=EDGE_CURVE('',#22803,#22701,#555,.T.) ;
#29169=EDGE_CURVE('',#22802,#22699,#556,.T.) ;
#29170=EDGE_CURVE('',#22801,#22700,#557,.T.) ;
#29171=EDGE_CURVE('',#22808,#22700,#5445,.T.) ;
#29172=EDGE_CURVE('',#22808,#22692,#5446,.T.) ;
#29173=EDGE_CURVE('',#22807,#22690,#5447,.T.) ;
#29174=EDGE_CURVE('',#22581,#22713,#558,.T.) ;
#29175=EDGE_CURVE('',#22580,#22712,#559,.T.) ;
#29176=EDGE_CURVE('',#22583,#22809,#560,.T.) ;
#29177=EDGE_CURVE('',#22809,#22713,#5448,.T.) ;
#29178=EDGE_CURVE('',#22714,#22582,#561,.T.) ;
#29179=EDGE_CURVE('',#22714,#22809,#5449,.T.) ;
#29180=EDGE_CURVE('',#22810,#22811,#5450,.T.) ;
#29181=EDGE_CURVE('',#22811,#22578,#19022,.T.) ;
#29182=EDGE_CURVE('',#22577,#22810,#562,.T.) ;
#29183=EDGE_CURVE('',#22576,#22743,#563,.T.) ;
#29184=EDGE_CURVE('',#22743,#22810,#5451,.T.) ;
#29185=EDGE_CURVE('',#22575,#22742,#564,.T.) ;
#29186=EDGE_CURVE('',#22574,#22741,#565,.T.) ;
#29187=EDGE_CURVE('',#22573,#22740,#566,.T.) ;
#29188=EDGE_CURVE('',#22737,#22571,#19023,.T.) ;
#29189=EDGE_CURVE('',#22570,#22738,#19024,.F.) ;
#29190=EDGE_CURVE('',#22739,#22572,#19025,.T.) ;
#29191=EDGE_CURVE('',#22812,#22579,#19026,.T.) ;
#29192=EDGE_CURVE('',#22811,#22812,#19027,.T.) ;
#29193=EDGE_CURVE('',#22813,#22569,#19028,.F.) ;
#29194=EDGE_CURVE('',#22812,#22813,#5452,.T.) ;
#29195=EDGE_CURVE('',#22813,#22725,#5453,.T.) ;
#29196=EDGE_CURVE('',#22812,#22724,#5454,.T.) ;
#29197=EDGE_CURVE('',#22811,#22722,#5455,.T.) ;
#29198=EDGE_CURVE('',#22810,#22720,#5456,.T.) ;
#29199=EDGE_CURVE('',#22561,#22814,#567,.T.) ;
#29200=EDGE_CURVE('',#22814,#22815,#5457,.T.) ;
#29201=EDGE_CURVE('',#22815,#22562,#568,.T.) ;
#29202=EDGE_CURVE('',#22772,#22816,#5458,.T.) ;
#29203=EDGE_CURVE('',#22816,#22558,#19029,.T.) ;
#29204=EDGE_CURVE('',#22559,#22772,#569,.T.) ;
#29205=EDGE_CURVE('',#22568,#22771,#570,.T.) ;
#29206=EDGE_CURVE('',#22567,#22770,#571,.T.) ;
#29207=EDGE_CURVE('',#22566,#22769,#572,.T.) ;
#29208=EDGE_CURVE('',#22565,#22768,#573,.T.) ;
#29209=EDGE_CURVE('',#22817,#22560,#19030,.T.) ;
#29210=EDGE_CURVE('',#22816,#22817,#19031,.T.) ;
#29211=EDGE_CURVE('',#22817,#22814,#5459,.T.) ;
#29212=EDGE_CURVE('',#22815,#22767,#5460,.T.) ;
#29213=EDGE_CURVE('',#22767,#22563,#19032,.T.) ;
#29214=EDGE_CURVE('',#22766,#22564,#19033,.T.) ;
#29215=EDGE_CURVE('',#22815,#22755,#5461,.T.) ;
#29216=EDGE_CURVE('',#22814,#22752,#5462,.T.) ;
#29217=EDGE_CURVE('',#22817,#22751,#5463,.T.) ;
#29218=EDGE_CURVE('',#22816,#22749,#5464,.T.) ;
#29219=EDGE_CURVE('',#22809,#22708,#5465,.T.) ;
#29220=EDGE_CURVE('',#22270,#22818,#5466,.F.) ;
#29221=EDGE_CURVE('',#22818,#22088,#5467,.T.) ;
#29222=EDGE_CURVE('',#22819,#22440,#5468,.T.) ;
#29223=EDGE_CURVE('',#22820,#22819,#19034,.T.) ;
#29224=EDGE_CURVE('',#22821,#22820,#5469,.T.) ;
#29225=EDGE_CURVE('',#22822,#22821,#19035,.T.) ;
#29226=EDGE_CURVE('',#22823,#22822,#5470,.T.) ;
#29227=EDGE_CURVE('',#22435,#22823,#5471,.T.) ;
#29228=EDGE_CURVE('',#22501,#22139,#5472,.T.) ;
#29229=EDGE_CURVE('',#22824,#22150,#5473,.T.) ;
#29230=EDGE_CURVE('',#22606,#22824,#19036,.T.) ;
#29231=EDGE_CURVE('',#22825,#22149,#5474,.T.) ;
#29232=EDGE_CURVE('',#22825,#22824,#5475,.T.) ;
#29233=EDGE_CURVE('',#22826,#22148,#5476,.T.) ;
#29234=EDGE_CURVE('',#22826,#22825,#19037,.T.) ;
#29235=EDGE_CURVE('',#22827,#22147,#5477,.T.) ;
#29236=EDGE_CURVE('',#22827,#22826,#5478,.T.) ;
#29237=EDGE_CURVE('',#22828,#22146,#5479,.T.) ;
#29238=EDGE_CURVE('',#22828,#22827,#5480,.T.) ;
#29239=EDGE_CURVE('',#22829,#22145,#5481,.T.) ;
#29240=EDGE_CURVE('',#22828,#22829,#5482,.T.) ;
#29241=EDGE_CURVE('',#22830,#22829,#5483,.T.) ;
#29242=EDGE_CURVE('',#21959,#22830,#19038,.T.) ;
#29243=EDGE_CURVE('',#22830,#22831,#5484,.T.) ;
#29244=EDGE_CURVE('',#21960,#22831,#19039,.T.) ;
#29245=EDGE_CURVE('',#22145,#22832,#5485,.T.) ;
#29246=EDGE_CURVE('',#22831,#22832,#5486,.T.) ;
#29247=EDGE_CURVE('',#22500,#22140,#5487,.T.) ;
#29248=EDGE_CURVE('',#22467,#22833,#5488,.T.) ;
#29249=EDGE_CURVE('',#22834,#22833,#5489,.T.) ;
#29250=EDGE_CURVE('',#22142,#22834,#5490,.T.) ;
#29251=EDGE_CURVE('',#22594,#22835,#5491,.T.) ;
#29252=EDGE_CURVE('',#22554,#22835,#5492,.T.) ;
#29253=EDGE_CURVE('',#22835,#22836,#5493,.T.) ;
#29254=EDGE_CURVE('',#22555,#22836,#5494,.T.) ;
#29255=EDGE_CURVE('',#22836,#22593,#5495,.T.) ;
#29256=EDGE_CURVE('',#22431,#21961,#5496,.T.) ;
#29257=EDGE_CURVE('',#22431,#22837,#5497,.T.) ;
#29258=EDGE_CURVE('',#22838,#22837,#5498,.T.) ;
#29259=EDGE_CURVE('',#21961,#22838,#5499,.T.) ;
#29260=EDGE_CURVE('',#22457,#22839,#5500,.T.) ;
#29261=EDGE_CURVE('',#22840,#22839,#19040,.T.) ;
#29262=EDGE_CURVE('',#22458,#22840,#5501,.T.) ;
#29263=EDGE_CURVE('',#22837,#22840,#5502,.T.) ;
#29264=EDGE_CURVE('',#22839,#22838,#5503,.T.) ;
#29265=EDGE_CURVE('',#22590,#22841,#5504,.T.) ;
#29266=EDGE_CURVE('',#22522,#22841,#19041,.T.) ;
#29267=EDGE_CURVE('',#21934,#21849,#5505,.T.) ;
#29268=EDGE_CURVE('',#22841,#21936,#5506,.T.) ;
#29269=EDGE_CURVE('',#22591,#21935,#5507,.F.) ;
#29270=EDGE_CURVE('',#22519,#22516,#5508,.T.) ;
#29271=EDGE_CURVE('',#22355,#22842,#5509,.T.) ;
#29272=EDGE_CURVE('',#22842,#22382,#19042,.F.) ;
#29273=EDGE_CURVE('',#22353,#22842,#5510,.T.) ;
#29274=EDGE_CURVE('',#22384,#22369,#5511,.T.) ;
#29275=EDGE_CURVE('',#22612,#22076,#5512,.T.) ;
#29276=EDGE_CURVE('',#22822,#22843,#1314,.T.) ;
#29277=EDGE_CURVE('',#22843,#22844,#5513,.T.) ;
#29278=EDGE_CURVE('',#22844,#22823,#574,.T.) ;
#29279=EDGE_CURVE('',#22794,#22845,#19043,.F.) ;
#29280=EDGE_CURVE('',#22846,#22794,#19044,.F.) ;
#29281=EDGE_CURVE('',#22845,#22846,#19045,.F.) ;
#29282=EDGE_CURVE('',#22821,#22847,#1315,.T.) ;
#29283=EDGE_CURVE('',#22847,#22843,#19046,.T.) ;
#29284=EDGE_CURVE('',#22793,#21717,#19047,.T.) ;
#29285=EDGE_CURVE('',#21719,#22846,#5514,.T.) ;
#29286=EDGE_CURVE('',#22848,#22849,#1316,.T.) ;
#29287=EDGE_CURVE('',#22819,#22849,#19048,.T.) ;
#29288=EDGE_CURVE('',#22584,#22819,#1317,.F.) ;
#29289=EDGE_CURVE('',#22848,#22584,#19049,.T.) ;
#29290=EDGE_CURVE('',#22850,#22820,#19050,.T.) ;
#29291=EDGE_CURVE('',#22849,#22850,#19051,.T.) ;
#29292=EDGE_CURVE('',#22850,#22847,#5515,.T.) ;
#29293=EDGE_CURVE('',#22473,#22851,#19052,.F.) ;
#29294=EDGE_CURVE('',#22851,#22492,#19053,.F.) ;
#29295=EDGE_CURVE('',#22494,#22852,#19054,.T.) ;
#29296=EDGE_CURVE('',#22852,#22851,#575,.T.) ;
#29297=EDGE_CURVE('',#22496,#22852,#5516,.T.) ;
#29298=EDGE_CURVE('',#22853,#22854,#19055,.T.) ;
#29299=EDGE_CURVE('',#22854,#22792,#19056,.T.) ;
#29300=EDGE_CURVE('',#22791,#22853,#1318,.T.) ;
#29301=EDGE_CURVE('',#22855,#22543,#19057,.T.) ;
#29302=EDGE_CURVE('',#22855,#22856,#1319,.T.) ;
#29303=EDGE_CURVE('',#22544,#22856,#19058,.T.) ;
#29304=EDGE_CURVE('',#22857,#22858,#5517,.T.) ;
#29305=EDGE_CURVE('',#22858,#22789,#19059,.T.) ;
#29306=EDGE_CURVE('',#22788,#22857,#1320,.T.) ;
#29307=EDGE_CURVE('',#22858,#22855,#19060,.T.) ;
#29308=EDGE_CURVE('',#22856,#22848,#576,.T.) ;
#29309=EDGE_CURVE('',#22859,#22860,#1321,.T.) ;
#29310=EDGE_CURVE('',#22542,#22860,#19061,.T.) ;
#29311=EDGE_CURVE('',#22859,#21865,#19062,.T.) ;
#29312=EDGE_CURVE('',#22861,#22790,#19063,.T.) ;
#29313=EDGE_CURVE('',#22860,#22861,#19064,.T.) ;
#29314=EDGE_CURVE('',#22861,#22853,#5518,.T.) ;
#29315=EDGE_CURVE('',#22862,#22377,#19065,.T.) ;
#29316=EDGE_CURVE('',#22862,#22863,#1322,.T.) ;
#29317=EDGE_CURVE('',#21864,#22863,#19066,.T.) ;
#29318=EDGE_CURVE('',#22864,#22865,#5519,.T.) ;
#29319=EDGE_CURVE('',#22865,#22477,#19067,.T.) ;
#29320=EDGE_CURVE('',#22476,#22864,#1323,.T.) ;
#29321=EDGE_CURVE('',#22865,#22862,#19068,.T.) ;
#29322=EDGE_CURVE('',#22863,#22859,#577,.T.) ;
#29323=EDGE_CURVE('',#22474,#22866,#19069,.T.) ;
#29324=EDGE_CURVE('',#22866,#22867,#5520,.T.) ;
#29325=EDGE_CURVE('',#22867,#22475,#19070,.T.) ;
#29326=EDGE_CURVE('',#22867,#22864,#19071,.T.) ;
#29327=EDGE_CURVE('',#22851,#22866,#19072,.T.) ;
#29328=EDGE_CURVE('',#22854,#21726,#5521,.T.) ;
#29329=EDGE_CURVE('',#22787,#22868,#19073,.T.) ;
#29330=EDGE_CURVE('',#22868,#22869,#5522,.T.) ;
#29331=EDGE_CURVE('',#22869,#22786,#19074,.T.) ;
#29332=EDGE_CURVE('',#22869,#22857,#19075,.T.) ;
#29333=EDGE_CURVE('',#22870,#22871,#578,.T.) ;
#29334=EDGE_CURVE('',#22871,#22872,#5523,.T.) ;
#29335=EDGE_CURVE('',#22872,#22873,#19076,.T.) ;
#29336=EDGE_CURVE('',#22873,#22870,#5524,.T.) ;
#29337=EDGE_CURVE('',#21724,#22873,#579,.T.) ;
#29338=EDGE_CURVE('',#22872,#21721,#580,.T.) ;
#29339=EDGE_CURVE('',#22845,#22868,#19077,.T.) ;
#29340=EDGE_CURVE('',#22874,#22875,#19078,.T.) ;
#29341=EDGE_CURVE('',#22875,#22845,#581,.T.) ;
#29342=EDGE_CURVE('',#22846,#22874,#582,.T.) ;
#29343=EDGE_CURVE('',#22876,#22877,#583,.T.) ;
#29344=EDGE_CURVE('',#22877,#22875,#5525,.T.) ;
#29345=EDGE_CURVE('',#22874,#22876,#5526,.T.) ;
#29346=EDGE_CURVE('',#22436,#22878,#5527,.T.) ;
#29347=EDGE_CURVE('',#22878,#22879,#19079,.T.) ;
#29348=EDGE_CURVE('',#22879,#21922,#5528,.T.) ;
#29349=EDGE_CURVE('',#22880,#22881,#19080,.T.) ;
#29350=EDGE_CURVE('',#22881,#22879,#584,.T.) ;
#29351=EDGE_CURVE('',#22878,#22880,#585,.T.) ;
#29352=EDGE_CURVE('',#22844,#22881,#5529,.T.) ;
#29353=EDGE_CURVE('',#22880,#22823,#5530,.T.) ;
#29354=EDGE_CURVE('',#22133,#22864,#5531,.T.) ;
#29355=EDGE_CURVE('',#22132,#22865,#5532,.T.) ;
#29356=EDGE_CURVE('',#22134,#22867,#5533,.T.) ;
#29357=EDGE_CURVE('',#22135,#22866,#5534,.T.) ;
#29358=EDGE_CURVE('',#22852,#22136,#5535,.T.) ;
#29359=EDGE_CURVE('',#22833,#22432,#19081,.T.) ;
#29360=EDGE_CURVE('',#22853,#22130,#5536,.T.) ;
#29361=EDGE_CURVE('',#22129,#22854,#5537,.T.) ;
#29362=EDGE_CURVE('',#22122,#22869,#5538,.T.) ;
#29363=EDGE_CURVE('',#22121,#22857,#5539,.T.) ;
#29364=EDGE_CURVE('',#22882,#22176,#5540,.T.) ;
#29365=EDGE_CURVE('',#22175,#22883,#5541,.T.) ;
#29366=EDGE_CURVE('',#22883,#22882,#5542,.T.) ;
#29367=EDGE_CURVE('',#22884,#22883,#19082,.T.) ;
#29368=EDGE_CURVE('',#22174,#22884,#5543,.T.) ;
#29369=EDGE_CURVE('',#22885,#22884,#5544,.T.) ;
#29370=EDGE_CURVE('',#22173,#22885,#5545,.T.) ;
#29371=EDGE_CURVE('',#22886,#22885,#5546,.T.) ;
#29372=EDGE_CURVE('',#22172,#22886,#5547,.T.) ;
#29373=EDGE_CURVE('',#22887,#22886,#19083,.T.) ;
#29374=EDGE_CURVE('',#22171,#22887,#5548,.T.) ;
#29375=EDGE_CURVE('',#22888,#22887,#5549,.T.) ;
#29376=EDGE_CURVE('',#22170,#22888,#5550,.T.) ;
#29377=EDGE_CURVE('',#22889,#22888,#19084,.T.) ;
#29378=EDGE_CURVE('',#22169,#22889,#5551,.T.) ;
#29379=EDGE_CURVE('',#22890,#22889,#5552,.T.) ;
#29380=EDGE_CURVE('',#22168,#22890,#5553,.T.) ;
#29381=EDGE_CURVE('',#22891,#22890,#5554,.T.) ;
#29382=EDGE_CURVE('',#22167,#22891,#5555,.T.) ;
#29383=EDGE_CURVE('',#22144,#22892,#5556,.T.) ;
#29384=EDGE_CURVE('',#22832,#22892,#1324,.T.) ;
#29385=EDGE_CURVE('',#22143,#22893,#5557,.T.) ;
#29386=EDGE_CURVE('',#22892,#22893,#5558,.T.) ;
#29387=EDGE_CURVE('',#22893,#22834,#1325,.T.) ;
#29388=EDGE_CURVE('',#22206,#22361,#5559,.T.) ;
#29389=EDGE_CURVE('',#22205,#22363,#5560,.T.) ;
#29390=EDGE_CURVE('',#22894,#22894,#19085,.T.) ;
#29391=EDGE_CURVE('',#22208,#22895,#5561,.T.) ;
#29392=EDGE_CURVE('',#22895,#22895,#19086,.T.) ;
#29393=EDGE_CURVE('',#22896,#22119,#5562,.T.) ;
#29394=EDGE_CURVE('',#22118,#22897,#5563,.T.) ;
#29395=EDGE_CURVE('',#22897,#22896,#5564,.T.) ;
#29396=EDGE_CURVE('',#22898,#22897,#19087,.T.) ;
#29397=EDGE_CURVE('',#22117,#22898,#5565,.T.) ;
#29398=EDGE_CURVE('',#22899,#22898,#5566,.T.) ;
#29399=EDGE_CURVE('',#22116,#22899,#5567,.T.) ;
#29400=EDGE_CURVE('',#22900,#22899,#19088,.T.) ;
#29401=EDGE_CURVE('',#22115,#22900,#5568,.T.) ;
#29402=EDGE_CURVE('',#22901,#22900,#5569,.T.) ;
#29403=EDGE_CURVE('',#22114,#22901,#5570,.T.) ;
#29404=EDGE_CURVE('',#22902,#22903,#19089,.T.) ;
#29405=EDGE_CURVE('',#22217,#22903,#5571,.T.) ;
#29406=EDGE_CURVE('',#22216,#22902,#5572,.T.) ;
#29407=EDGE_CURVE('',#22904,#22902,#5573,.T.) ;
#29408=EDGE_CURVE('',#22215,#22904,#5574,.T.) ;
#29409=EDGE_CURVE('',#22905,#22904,#19090,.T.) ;
#29410=EDGE_CURVE('',#22214,#22905,#5575,.T.) ;
#29411=EDGE_CURVE('',#22906,#22905,#5576,.T.) ;
#29412=EDGE_CURVE('',#22213,#22906,#5577,.T.) ;
#29413=EDGE_CURVE('',#22907,#22906,#5578,.T.) ;
#29414=EDGE_CURVE('',#22212,#22907,#5579,.T.) ;
#29415=EDGE_CURVE('',#22908,#22907,#19091,.T.) ;
#29416=EDGE_CURVE('',#22211,#22908,#5580,.T.) ;
#29417=EDGE_CURVE('',#22909,#22908,#5581,.T.) ;
#29418=EDGE_CURVE('',#22209,#22909,#5582,.T.) ;
#29419=EDGE_CURVE('',#22223,#22910,#5583,.T.) ;
#29420=EDGE_CURVE('',#22910,#22910,#19092,.T.) ;
#29421=EDGE_CURVE('',#22911,#22912,#5584,.T.) ;
#29422=EDGE_CURVE('',#22231,#22912,#5585,.T.) ;
#29423=EDGE_CURVE('',#22230,#22911,#5586,.T.) ;
#29424=EDGE_CURVE('',#22913,#22911,#19093,.T.) ;
#29425=EDGE_CURVE('',#22229,#22913,#5587,.T.) ;
#29426=EDGE_CURVE('',#22914,#22913,#5588,.T.) ;
#29427=EDGE_CURVE('',#22228,#22914,#5589,.T.) ;
#29428=EDGE_CURVE('',#22915,#22914,#19094,.T.) ;
#29429=EDGE_CURVE('',#22227,#22915,#5590,.T.) ;
#29430=EDGE_CURVE('',#22916,#22915,#5591,.T.) ;
#29431=EDGE_CURVE('',#22226,#22916,#5592,.T.) ;
#29432=EDGE_CURVE('',#22917,#22916,#1326,.T.) ;
#29433=EDGE_CURVE('',#22224,#22917,#5593,.T.) ;
#29434=EDGE_CURVE('',#22918,#22919,#19095,.T.) ;
#29435=EDGE_CURVE('',#22242,#22919,#5594,.T.) ;
#29436=EDGE_CURVE('',#22241,#22918,#5595,.T.) ;
#29437=EDGE_CURVE('',#22920,#22918,#5596,.T.) ;
#29438=EDGE_CURVE('',#22240,#22920,#5597,.T.) ;
#29439=EDGE_CURVE('',#22921,#22920,#19096,.T.) ;
#29440=EDGE_CURVE('',#22239,#22921,#5598,.T.) ;
#29441=EDGE_CURVE('',#22922,#22921,#5599,.T.) ;
#29442=EDGE_CURVE('',#22238,#22922,#5600,.T.) ;
#29443=EDGE_CURVE('',#21805,#22922,#5601,.T.) ;
#29444=EDGE_CURVE('',#22923,#21810,#5602,.T.) ;
#29445=EDGE_CURVE('',#22236,#22923,#5603,.T.) ;
#29446=EDGE_CURVE('',#22924,#22925,#19097,.T.) ;
#29447=EDGE_CURVE('',#22181,#22925,#5604,.T.) ;
#29448=EDGE_CURVE('',#22180,#22924,#5605,.T.) ;
#29449=EDGE_CURVE('',#22926,#22924,#5606,.T.) ;
#29450=EDGE_CURVE('',#21996,#22179,#5607,.T.) ;
#29451=EDGE_CURVE('',#21995,#22926,#5608,.T.) ;
#29452=EDGE_CURVE('',#22927,#22926,#19098,.T.) ;
#29453=EDGE_CURVE('',#21994,#22927,#5609,.T.) ;
#29454=EDGE_CURVE('',#22928,#22927,#5610,.T.) ;
#29455=EDGE_CURVE('',#21993,#22928,#5611,.T.) ;
#29456=EDGE_CURVE('',#22273,#22928,#19099,.T.) ;
#29457=EDGE_CURVE('',#22929,#22930,#19100,.T.) ;
#29458=EDGE_CURVE('',#22256,#22930,#5612,.T.) ;
#29459=EDGE_CURVE('',#22255,#22929,#5613,.T.) ;
#29460=EDGE_CURVE('',#22931,#22929,#5614,.T.) ;
#29461=EDGE_CURVE('',#22254,#22931,#5615,.T.) ;
#29462=EDGE_CURVE('',#22932,#22931,#19101,.T.) ;
#29463=EDGE_CURVE('',#22253,#22932,#5616,.T.) ;
#29464=EDGE_CURVE('',#22933,#22932,#5617,.T.) ;
#29465=EDGE_CURVE('',#22252,#22933,#5618,.T.) ;
#29466=EDGE_CURVE('',#22934,#22933,#5619,.T.) ;
#29467=EDGE_CURVE('',#22251,#22934,#5620,.T.) ;
#29468=EDGE_CURVE('',#22935,#22934,#19102,.T.) ;
#29469=EDGE_CURVE('',#22250,#22935,#5621,.T.) ;
#29470=EDGE_CURVE('',#22936,#22935,#5622,.T.) ;
#29471=EDGE_CURVE('',#22248,#22936,#5623,.T.) ;
#29472=EDGE_CURVE('',#22937,#22936,#19103,.T.) ;
#29473=EDGE_CURVE('',#22249,#22937,#5624,.T.) ;
#29474=EDGE_CURVE('',#22938,#22937,#5625,.T.) ;
#29475=EDGE_CURVE('',#22261,#22938,#5626,.T.) ;
#29476=EDGE_CURVE('',#22939,#22938,#5627,.T.) ;
#29477=EDGE_CURVE('',#22260,#22939,#5628,.T.) ;
#29478=EDGE_CURVE('',#22940,#22939,#19104,.T.) ;
#29479=EDGE_CURVE('',#22259,#22940,#5629,.T.) ;
#29480=EDGE_CURVE('',#22941,#22940,#5630,.T.) ;
#29481=EDGE_CURVE('',#22258,#22941,#5631,.T.) ;
#29482=EDGE_CURVE('',#22942,#22941,#19105,.T.) ;
#29483=EDGE_CURVE('',#22257,#22942,#5632,.T.) ;
#29484=EDGE_CURVE('',#22930,#22942,#5633,.T.) ;
#29485=EDGE_CURVE('',#22943,#22917,#5634,.T.) ;
#29486=EDGE_CURVE('',#22225,#22943,#5635,.T.) ;
#29487=EDGE_CURVE('',#22944,#22943,#1327,.T.) ;
#29488=EDGE_CURVE('',#22235,#22944,#5636,.T.) ;
#29489=EDGE_CURVE('',#22945,#22944,#5637,.T.) ;
#29490=EDGE_CURVE('',#22234,#22945,#5638,.T.) ;
#29491=EDGE_CURVE('',#22946,#22945,#19106,.T.) ;
#29492=EDGE_CURVE('',#22233,#22946,#5639,.T.) ;
#29493=EDGE_CURVE('',#22947,#22946,#5640,.T.) ;
#29494=EDGE_CURVE('',#22232,#22947,#5641,.T.) ;
#29495=EDGE_CURVE('',#22912,#22947,#19107,.T.) ;
#29496=EDGE_CURVE('',#22948,#22923,#1328,.T.) ;
#29497=EDGE_CURVE('',#22237,#22948,#5642,.T.) ;
#29498=EDGE_CURVE('',#22949,#22948,#5643,.T.) ;
#29499=EDGE_CURVE('',#22247,#22949,#5644,.T.) ;
#29500=EDGE_CURVE('',#22950,#22949,#5645,.T.) ;
#29501=EDGE_CURVE('',#22246,#22950,#5646,.T.) ;
#29502=EDGE_CURVE('',#22951,#22950,#19108,.T.) ;
#29503=EDGE_CURVE('',#22245,#22951,#5647,.T.) ;
#29504=EDGE_CURVE('',#22952,#22951,#5648,.T.) ;
#29505=EDGE_CURVE('',#22244,#22952,#5649,.T.) ;
#29506=EDGE_CURVE('',#22953,#22952,#19109,.T.) ;
#29507=EDGE_CURVE('',#22243,#22953,#5650,.T.) ;
#29508=EDGE_CURVE('',#22919,#22953,#5651,.T.) ;
#29509=EDGE_CURVE('',#22954,#22901,#19110,.T.) ;
#29510=EDGE_CURVE('',#22113,#22954,#5652,.T.) ;
#29511=EDGE_CURVE('',#22955,#22954,#5653,.T.) ;
#29512=EDGE_CURVE('',#22112,#22955,#5654,.T.) ;
#29513=EDGE_CURVE('',#22956,#22955,#5655,.T.) ;
#29514=EDGE_CURVE('',#22111,#22956,#5656,.T.) ;
#29515=EDGE_CURVE('',#22957,#22956,#5657,.T.) ;
#29516=EDGE_CURVE('',#22110,#22957,#5658,.T.) ;
#29517=EDGE_CURVE('',#22958,#22957,#5659,.T.) ;
#29518=EDGE_CURVE('',#22109,#22958,#5660,.T.) ;
#29519=EDGE_CURVE('',#22959,#22958,#5661,.T.) ;
#29520=EDGE_CURVE('',#22108,#22959,#5662,.T.) ;
#29521=EDGE_CURVE('',#22960,#22959,#19111,.T.) ;
#29522=EDGE_CURVE('',#22107,#22960,#5663,.T.) ;
#29523=EDGE_CURVE('',#22961,#22896,#19112,.T.) ;
#29524=EDGE_CURVE('',#22961,#22960,#5664,.T.) ;
#29525=EDGE_CURVE('',#22962,#22909,#19113,.T.) ;
#29526=EDGE_CURVE('',#22210,#22962,#5665,.T.) ;
#29527=EDGE_CURVE('',#22963,#22962,#5666,.T.) ;
#29528=EDGE_CURVE('',#22222,#22963,#5667,.T.) ;
#29529=EDGE_CURVE('',#22964,#22963,#5668,.T.) ;
#29530=EDGE_CURVE('',#22221,#22964,#5669,.T.) ;
#29531=EDGE_CURVE('',#22965,#22964,#19114,.T.) ;
#29532=EDGE_CURVE('',#22220,#22965,#5670,.T.) ;
#29533=EDGE_CURVE('',#22966,#22965,#5671,.T.) ;
#29534=EDGE_CURVE('',#22219,#22966,#5672,.T.) ;
#29535=EDGE_CURVE('',#22967,#22966,#19115,.T.) ;
#29536=EDGE_CURVE('',#22218,#22967,#5673,.T.) ;
#29537=EDGE_CURVE('',#22903,#22967,#5674,.T.) ;
#29538=EDGE_CURVE('',#22968,#22272,#19116,.T.) ;
#29539=EDGE_CURVE('',#22186,#22968,#5675,.T.) ;
#29540=EDGE_CURVE('',#22969,#22968,#5676,.T.) ;
#29541=EDGE_CURVE('',#22185,#22969,#5677,.T.) ;
#29542=EDGE_CURVE('',#22970,#22969,#19117,.T.) ;
#29543=EDGE_CURVE('',#22184,#22970,#5678,.T.) ;
#29544=EDGE_CURVE('',#22971,#22970,#5679,.T.) ;
#29545=EDGE_CURVE('',#22183,#22971,#5680,.T.) ;
#29546=EDGE_CURVE('',#22972,#22971,#19118,.T.) ;
#29547=EDGE_CURVE('',#22182,#22972,#5681,.T.) ;
#29548=EDGE_CURVE('',#22925,#22972,#5682,.T.) ;
#29549=EDGE_CURVE('',#22973,#22891,#19119,.T.) ;
#29550=EDGE_CURVE('',#22166,#22973,#5683,.T.) ;
#29551=EDGE_CURVE('',#22974,#22973,#5684,.T.) ;
#29552=EDGE_CURVE('',#22165,#22974,#5685,.T.) ;
#29553=EDGE_CURVE('',#22127,#22873,#5686,.T.) ;
#29554=EDGE_CURVE('',#22126,#22870,#5687,.T.) ;
#29555=EDGE_CURVE('',#22877,#22125,#5688,.T.) ;
#29556=EDGE_CURVE('',#22871,#22876,#5689,.T.) ;
#29557=EDGE_CURVE('',#22875,#22124,#5690,.T.) ;
#29558=EDGE_CURVE('',#22103,#22843,#5691,.T.) ;
#29559=EDGE_CURVE('',#22881,#22102,#5692,.T.) ;
#29560=EDGE_CURVE('',#22302,#22199,#5693,.T.) ;
#29561=EDGE_CURVE('',#22289,#22298,#5694,.T.) ;
#29562=EDGE_CURVE('',#22287,#22299,#5695,.T.) ;
#29563=EDGE_CURVE('',#22286,#22300,#5696,.T.) ;
#29564=EDGE_CURVE('',#22303,#22198,#5697,.T.) ;
#29565=EDGE_CURVE('',#22975,#22882,#19120,.T.) ;
#29566=EDGE_CURVE('',#22975,#22974,#19121,.T.) ;
#29567=EDGE_CURVE('',#22164,#22975,#5698,.T.) ;
#29568=EDGE_CURVE('',#21998,#22177,#5699,.T.) ;
#29569=EDGE_CURVE('',#21997,#22178,#5700,.T.) ;
#29570=EDGE_CURVE('',#22159,#22818,#5701,.T.) ;
#29571=EDGE_CURVE('',#22123,#22868,#5702,.T.) ;
#29572=EDGE_CURVE('',#22101,#22879,#5703,.T.) ;
#29573=EDGE_CURVE('',#21723,#22128,#5704,.T.) ;
#29574=EDGE_CURVE('',#22497,#22894,#5705,.T.) ;
#29575=EDGE_CURVE('',#22106,#22961,#5706,.T.) ;
#29576=EDGE_CURVE('',#22847,#22104,#5707,.T.) ;
#29577=EDGE_CURVE('',#22120,#22858,#5708,.T.) ;
#29578=EDGE_CURVE('',#22105,#22850,#5709,.T.) ;
#29579=EDGE_CURVE('',#22131,#22861,#5710,.T.) ;
#29580=EDGE_CURVE('',#22379,#22349,#5711,.T.) ;
#29581=EDGE_CURVE('',#22348,#22354,#5712,.T.) ;
#38470=ORIENTED_EDGE('',*,*,#27513,.F.) ;
#38471=ORIENTED_EDGE('',*,*,#27514,.T.) ;
#38472=ORIENTED_EDGE('',*,*,#27515,.T.) ;
#38473=ORIENTED_EDGE('',*,*,#27516,.F.) ;
#38474=ORIENTED_EDGE('',*,*,#27514,.F.) ;
#38475=ORIENTED_EDGE('',*,*,#27517,.T.) ;
#38476=ORIENTED_EDGE('',*,*,#27518,.F.) ;
#38477=ORIENTED_EDGE('',*,*,#27519,.T.) ;
#38478=ORIENTED_EDGE('',*,*,#27517,.F.) ;
#38479=ORIENTED_EDGE('',*,*,#27520,.T.) ;
#38480=ORIENTED_EDGE('',*,*,#27521,.T.) ;
#38481=ORIENTED_EDGE('',*,*,#27522,.T.) ;
#38482=ORIENTED_EDGE('',*,*,#27523,.F.) ;
#38483=ORIENTED_EDGE('',*,*,#27520,.F.) ;
#38484=ORIENTED_EDGE('',*,*,#27524,.T.) ;
#38485=ORIENTED_EDGE('',*,*,#27525,.F.) ;
#38486=ORIENTED_EDGE('',*,*,#27526,.T.) ;
#38487=ORIENTED_EDGE('',*,*,#27524,.F.) ;
#38488=ORIENTED_EDGE('',*,*,#27527,.T.) ;
#38489=ORIENTED_EDGE('',*,*,#27528,.T.) ;
#38490=ORIENTED_EDGE('',*,*,#27529,.F.) ;
#38491=ORIENTED_EDGE('',*,*,#27530,.F.) ;
#38492=ORIENTED_EDGE('',*,*,#27531,.T.) ;
#38493=ORIENTED_EDGE('',*,*,#27532,.T.) ;
#38494=ORIENTED_EDGE('',*,*,#27533,.F.) ;
#38495=ORIENTED_EDGE('',*,*,#27534,.F.) ;
#38496=ORIENTED_EDGE('',*,*,#27535,.T.) ;
#38497=ORIENTED_EDGE('',*,*,#27536,.T.) ;
#38498=ORIENTED_EDGE('',*,*,#27531,.F.) ;
#38499=ORIENTED_EDGE('',*,*,#27537,.F.) ;
#38500=ORIENTED_EDGE('',*,*,#27538,.T.) ;
#38501=ORIENTED_EDGE('',*,*,#27539,.T.) ;
#38502=ORIENTED_EDGE('',*,*,#27535,.F.) ;
#38503=ORIENTED_EDGE('',*,*,#27540,.F.) ;
#38504=ORIENTED_EDGE('',*,*,#27541,.T.) ;
#38505=ORIENTED_EDGE('',*,*,#27542,.T.) ;
#38506=ORIENTED_EDGE('',*,*,#27538,.F.) ;
#38507=ORIENTED_EDGE('',*,*,#27543,.F.) ;
#38508=ORIENTED_EDGE('',*,*,#27544,.T.) ;
#38509=ORIENTED_EDGE('',*,*,#27545,.T.) ;
#38510=ORIENTED_EDGE('',*,*,#27541,.F.) ;
#38511=ORIENTED_EDGE('',*,*,#27546,.F.) ;
#38512=ORIENTED_EDGE('',*,*,#27547,.T.) ;
#38513=ORIENTED_EDGE('',*,*,#27548,.T.) ;
#38514=ORIENTED_EDGE('',*,*,#27544,.F.) ;
#38515=ORIENTED_EDGE('',*,*,#27549,.F.) ;
#38516=ORIENTED_EDGE('',*,*,#27550,.T.) ;
#38517=ORIENTED_EDGE('',*,*,#27551,.T.) ;
#38518=ORIENTED_EDGE('',*,*,#27547,.F.) ;
#38519=ORIENTED_EDGE('',*,*,#27552,.F.) ;
#38520=ORIENTED_EDGE('',*,*,#27533,.T.) ;
#38521=ORIENTED_EDGE('',*,*,#27553,.T.) ;
#38522=ORIENTED_EDGE('',*,*,#27550,.F.) ;
#38523=ORIENTED_EDGE('',*,*,#27554,.F.) ;
#38524=ORIENTED_EDGE('',*,*,#27555,.T.) ;
#38525=ORIENTED_EDGE('',*,*,#27556,.T.) ;
#38526=ORIENTED_EDGE('',*,*,#27557,.F.) ;
#38527=ORIENTED_EDGE('',*,*,#27558,.F.) ;
#38528=ORIENTED_EDGE('',*,*,#27559,.T.) ;
#38529=ORIENTED_EDGE('',*,*,#27560,.T.) ;
#38530=ORIENTED_EDGE('',*,*,#27555,.F.) ;
#38531=ORIENTED_EDGE('',*,*,#27561,.F.) ;
#38532=ORIENTED_EDGE('',*,*,#27562,.T.) ;
#38533=ORIENTED_EDGE('',*,*,#27563,.T.) ;
#38534=ORIENTED_EDGE('',*,*,#27559,.F.) ;
#38535=ORIENTED_EDGE('',*,*,#27564,.F.) ;
#38536=ORIENTED_EDGE('',*,*,#27565,.T.) ;
#38537=ORIENTED_EDGE('',*,*,#27566,.T.) ;
#38538=ORIENTED_EDGE('',*,*,#27562,.F.) ;
#38539=ORIENTED_EDGE('',*,*,#27567,.F.) ;
#38540=ORIENTED_EDGE('',*,*,#27568,.T.) ;
#38541=ORIENTED_EDGE('',*,*,#27569,.T.) ;
#38542=ORIENTED_EDGE('',*,*,#27565,.F.) ;
#38543=ORIENTED_EDGE('',*,*,#27570,.F.) ;
#38544=ORIENTED_EDGE('',*,*,#27571,.T.) ;
#38545=ORIENTED_EDGE('',*,*,#27572,.T.) ;
#38546=ORIENTED_EDGE('',*,*,#27568,.F.) ;
#38547=ORIENTED_EDGE('',*,*,#27573,.F.) ;
#38548=ORIENTED_EDGE('',*,*,#27574,.T.) ;
#38549=ORIENTED_EDGE('',*,*,#27575,.T.) ;
#38550=ORIENTED_EDGE('',*,*,#27571,.F.) ;
#38551=ORIENTED_EDGE('',*,*,#27576,.F.) ;
#38552=ORIENTED_EDGE('',*,*,#27577,.T.) ;
#38553=ORIENTED_EDGE('',*,*,#27578,.T.) ;
#38554=ORIENTED_EDGE('',*,*,#27574,.F.) ;
#38555=ORIENTED_EDGE('',*,*,#27579,.F.) ;
#38556=ORIENTED_EDGE('',*,*,#27580,.T.) ;
#38557=ORIENTED_EDGE('',*,*,#27581,.T.) ;
#38558=ORIENTED_EDGE('',*,*,#27577,.F.) ;
#38559=ORIENTED_EDGE('',*,*,#27582,.F.) ;
#38560=ORIENTED_EDGE('',*,*,#27583,.T.) ;
#38561=ORIENTED_EDGE('',*,*,#27584,.T.) ;
#38562=ORIENTED_EDGE('',*,*,#27580,.F.) ;
#38563=ORIENTED_EDGE('',*,*,#27585,.F.) ;
#38564=ORIENTED_EDGE('',*,*,#27586,.T.) ;
#38565=ORIENTED_EDGE('',*,*,#27587,.T.) ;
#38566=ORIENTED_EDGE('',*,*,#27583,.F.) ;
#38567=ORIENTED_EDGE('',*,*,#27588,.F.) ;
#38568=ORIENTED_EDGE('',*,*,#27589,.T.) ;
#38569=ORIENTED_EDGE('',*,*,#27590,.T.) ;
#38570=ORIENTED_EDGE('',*,*,#27586,.F.) ;
#38571=ORIENTED_EDGE('',*,*,#27591,.F.) ;
#38572=ORIENTED_EDGE('',*,*,#27592,.T.) ;
#38573=ORIENTED_EDGE('',*,*,#27593,.T.) ;
#38574=ORIENTED_EDGE('',*,*,#27589,.F.) ;
#38575=ORIENTED_EDGE('',*,*,#27594,.F.) ;
#38576=ORIENTED_EDGE('',*,*,#27595,.T.) ;
#38577=ORIENTED_EDGE('',*,*,#27596,.T.) ;
#38578=ORIENTED_EDGE('',*,*,#27592,.F.) ;
#38579=ORIENTED_EDGE('',*,*,#27597,.F.) ;
#38580=ORIENTED_EDGE('',*,*,#27598,.T.) ;
#38581=ORIENTED_EDGE('',*,*,#27599,.T.) ;
#38582=ORIENTED_EDGE('',*,*,#27595,.F.) ;
#38583=ORIENTED_EDGE('',*,*,#27600,.F.) ;
#38584=ORIENTED_EDGE('',*,*,#27601,.T.) ;
#38585=ORIENTED_EDGE('',*,*,#27602,.T.) ;
#38586=ORIENTED_EDGE('',*,*,#27598,.F.) ;
#38587=ORIENTED_EDGE('',*,*,#27603,.F.) ;
#38588=ORIENTED_EDGE('',*,*,#27604,.T.) ;
#38589=ORIENTED_EDGE('',*,*,#27605,.T.) ;
#38590=ORIENTED_EDGE('',*,*,#27601,.F.) ;
#38591=ORIENTED_EDGE('',*,*,#27606,.F.) ;
#38592=ORIENTED_EDGE('',*,*,#27607,.T.) ;
#38593=ORIENTED_EDGE('',*,*,#27608,.T.) ;
#38594=ORIENTED_EDGE('',*,*,#27604,.F.) ;
#38595=ORIENTED_EDGE('',*,*,#27609,.F.) ;
#38596=ORIENTED_EDGE('',*,*,#27557,.T.) ;
#38597=ORIENTED_EDGE('',*,*,#27610,.T.) ;
#38598=ORIENTED_EDGE('',*,*,#27607,.F.) ;
#38599=ORIENTED_EDGE('',*,*,#27610,.F.) ;
#38600=ORIENTED_EDGE('',*,*,#27556,.F.) ;
#38601=ORIENTED_EDGE('',*,*,#27560,.F.) ;
#38602=ORIENTED_EDGE('',*,*,#27563,.F.) ;
#38603=ORIENTED_EDGE('',*,*,#27566,.F.) ;
#38604=ORIENTED_EDGE('',*,*,#27569,.F.) ;
#38605=ORIENTED_EDGE('',*,*,#27572,.F.) ;
#38606=ORIENTED_EDGE('',*,*,#27575,.F.) ;
#38607=ORIENTED_EDGE('',*,*,#27578,.F.) ;
#38608=ORIENTED_EDGE('',*,*,#27581,.F.) ;
#38609=ORIENTED_EDGE('',*,*,#27584,.F.) ;
#38610=ORIENTED_EDGE('',*,*,#27587,.F.) ;
#38611=ORIENTED_EDGE('',*,*,#27590,.F.) ;
#38612=ORIENTED_EDGE('',*,*,#27593,.F.) ;
#38613=ORIENTED_EDGE('',*,*,#27596,.F.) ;
#38614=ORIENTED_EDGE('',*,*,#27599,.F.) ;
#38615=ORIENTED_EDGE('',*,*,#27602,.F.) ;
#38616=ORIENTED_EDGE('',*,*,#27605,.F.) ;
#38617=ORIENTED_EDGE('',*,*,#27608,.F.) ;
#38618=ORIENTED_EDGE('',*,*,#27553,.F.) ;
#38619=ORIENTED_EDGE('',*,*,#27532,.F.) ;
#38620=ORIENTED_EDGE('',*,*,#27536,.F.) ;
#38621=ORIENTED_EDGE('',*,*,#27539,.F.) ;
#38622=ORIENTED_EDGE('',*,*,#27542,.F.) ;
#38623=ORIENTED_EDGE('',*,*,#27545,.F.) ;
#38624=ORIENTED_EDGE('',*,*,#27548,.F.) ;
#38625=ORIENTED_EDGE('',*,*,#27551,.F.) ;
#38626=ORIENTED_EDGE('',*,*,#27611,.F.) ;
#38627=ORIENTED_EDGE('',*,*,#27612,.F.) ;
#38628=ORIENTED_EDGE('',*,*,#27613,.T.) ;
#38629=ORIENTED_EDGE('',*,*,#27614,.F.) ;
#38630=ORIENTED_EDGE('',*,*,#27615,.F.) ;
#38631=ORIENTED_EDGE('',*,*,#27616,.F.) ;
#38632=ORIENTED_EDGE('',*,*,#27617,.F.) ;
#38633=ORIENTED_EDGE('',*,*,#27618,.F.) ;
#38634=ORIENTED_EDGE('',*,*,#27619,.F.) ;
#38635=ORIENTED_EDGE('',*,*,#27620,.F.) ;
#38636=ORIENTED_EDGE('',*,*,#27621,.F.) ;
#38637=ORIENTED_EDGE('',*,*,#27622,.F.) ;
#38638=ORIENTED_EDGE('',*,*,#27623,.F.) ;
#38639=ORIENTED_EDGE('',*,*,#27624,.F.) ;
#38640=ORIENTED_EDGE('',*,*,#27625,.F.) ;
#38641=ORIENTED_EDGE('',*,*,#27626,.F.) ;
#38642=ORIENTED_EDGE('',*,*,#27627,.F.) ;
#38643=ORIENTED_EDGE('',*,*,#27628,.F.) ;
#38644=ORIENTED_EDGE('',*,*,#27629,.F.) ;
#38645=ORIENTED_EDGE('',*,*,#27630,.F.) ;
#38646=ORIENTED_EDGE('',*,*,#27631,.F.) ;
#38647=ORIENTED_EDGE('',*,*,#27632,.F.) ;
#38648=ORIENTED_EDGE('',*,*,#27554,.T.) ;
#38649=ORIENTED_EDGE('',*,*,#27609,.T.) ;
#38650=ORIENTED_EDGE('',*,*,#27606,.T.) ;
#38651=ORIENTED_EDGE('',*,*,#27603,.T.) ;
#38652=ORIENTED_EDGE('',*,*,#27600,.T.) ;
#38653=ORIENTED_EDGE('',*,*,#27597,.T.) ;
#38654=ORIENTED_EDGE('',*,*,#27594,.T.) ;
#38655=ORIENTED_EDGE('',*,*,#27591,.T.) ;
#38656=ORIENTED_EDGE('',*,*,#27588,.T.) ;
#38657=ORIENTED_EDGE('',*,*,#27585,.T.) ;
#38658=ORIENTED_EDGE('',*,*,#27582,.T.) ;
#38659=ORIENTED_EDGE('',*,*,#27579,.T.) ;
#38660=ORIENTED_EDGE('',*,*,#27576,.T.) ;
#38661=ORIENTED_EDGE('',*,*,#27573,.T.) ;
#38662=ORIENTED_EDGE('',*,*,#27570,.T.) ;
#38663=ORIENTED_EDGE('',*,*,#27567,.T.) ;
#38664=ORIENTED_EDGE('',*,*,#27564,.T.) ;
#38665=ORIENTED_EDGE('',*,*,#27561,.T.) ;
#38666=ORIENTED_EDGE('',*,*,#27558,.T.) ;
#38667=ORIENTED_EDGE('',*,*,#27633,.F.) ;
#38668=ORIENTED_EDGE('',*,*,#27634,.T.) ;
#38669=ORIENTED_EDGE('',*,*,#27635,.T.) ;
#38670=ORIENTED_EDGE('',*,*,#27636,.T.) ;
#38671=ORIENTED_EDGE('',*,*,#27636,.F.) ;
#38672=ORIENTED_EDGE('',*,*,#27637,.T.) ;
#38673=ORIENTED_EDGE('',*,*,#27638,.T.) ;
#38674=ORIENTED_EDGE('',*,*,#27639,.T.) ;
#38675=ORIENTED_EDGE('',*,*,#27640,.T.) ;
#38676=ORIENTED_EDGE('',*,*,#27641,.T.) ;
#38677=ORIENTED_EDGE('',*,*,#27642,.T.) ;
#38678=ORIENTED_EDGE('',*,*,#27643,.T.) ;
#38679=ORIENTED_EDGE('',*,*,#27644,.T.) ;
#38680=ORIENTED_EDGE('',*,*,#27645,.T.) ;
#38681=ORIENTED_EDGE('',*,*,#27640,.F.) ;
#38682=ORIENTED_EDGE('',*,*,#27646,.T.) ;
#38683=ORIENTED_EDGE('',*,*,#27647,.T.) ;
#38684=ORIENTED_EDGE('',*,*,#27648,.T.) ;
#38685=ORIENTED_EDGE('',*,*,#27644,.F.) ;
#38686=ORIENTED_EDGE('',*,*,#27649,.T.) ;
#38687=ORIENTED_EDGE('',*,*,#27650,.T.) ;
#38688=ORIENTED_EDGE('',*,*,#27651,.T.) ;
#38689=ORIENTED_EDGE('',*,*,#27652,.T.) ;
#38690=ORIENTED_EDGE('',*,*,#27647,.F.) ;
#38691=ORIENTED_EDGE('',*,*,#27653,.T.) ;
#38692=ORIENTED_EDGE('',*,*,#27654,.F.) ;
#38693=ORIENTED_EDGE('',*,*,#27655,.F.) ;
#38694=ORIENTED_EDGE('',*,*,#27656,.F.) ;
#38695=ORIENTED_EDGE('',*,*,#27650,.F.) ;
#38696=ORIENTED_EDGE('',*,*,#27657,.T.) ;
#38697=ORIENTED_EDGE('',*,*,#27657,.F.) ;
#38698=ORIENTED_EDGE('',*,*,#27653,.F.) ;
#38699=ORIENTED_EDGE('',*,*,#27658,.F.) ;
#38700=ORIENTED_EDGE('',*,*,#27659,.F.) ;
#38701=ORIENTED_EDGE('',*,*,#27660,.F.) ;
#38702=ORIENTED_EDGE('',*,*,#27661,.F.) ;
#38703=ORIENTED_EDGE('',*,*,#27662,.T.) ;
#38704=ORIENTED_EDGE('',*,*,#27649,.F.) ;
#38705=ORIENTED_EDGE('',*,*,#27663,.T.) ;
#38706=ORIENTED_EDGE('',*,*,#27664,.T.) ;
#38707=ORIENTED_EDGE('',*,*,#27658,.T.) ;
#38708=ORIENTED_EDGE('',*,*,#27646,.F.) ;
#38709=ORIENTED_EDGE('',*,*,#27643,.F.) ;
#38710=ORIENTED_EDGE('',*,*,#27665,.F.) ;
#38711=ORIENTED_EDGE('',*,*,#27666,.F.) ;
#38712=ORIENTED_EDGE('',*,*,#27663,.F.) ;
#38713=ORIENTED_EDGE('',*,*,#27667,.F.) ;
#38714=ORIENTED_EDGE('',*,*,#27668,.T.) ;
#38715=ORIENTED_EDGE('',*,*,#27669,.T.) ;
#38716=ORIENTED_EDGE('',*,*,#27670,.T.) ;
#38717=ORIENTED_EDGE('',*,*,#27671,.T.) ;
#38718=ORIENTED_EDGE('',*,*,#27672,.T.) ;
#38719=ORIENTED_EDGE('',*,*,#27673,.T.) ;
#38720=ORIENTED_EDGE('',*,*,#27674,.T.) ;
#38721=ORIENTED_EDGE('',*,*,#27675,.T.) ;
#38722=ORIENTED_EDGE('',*,*,#27669,.F.) ;
#38723=ORIENTED_EDGE('',*,*,#27676,.T.) ;
#38724=ORIENTED_EDGE('',*,*,#27677,.T.) ;
#38725=ORIENTED_EDGE('',*,*,#27678,.T.) ;
#38726=ORIENTED_EDGE('',*,*,#27674,.F.) ;
#38727=ORIENTED_EDGE('',*,*,#27679,.T.) ;
#38728=ORIENTED_EDGE('',*,*,#27680,.T.) ;
#38729=ORIENTED_EDGE('',*,*,#27681,.T.) ;
#38730=ORIENTED_EDGE('',*,*,#27677,.F.) ;
#38731=ORIENTED_EDGE('',*,*,#27682,.T.) ;
#38732=ORIENTED_EDGE('',*,*,#27683,.T.) ;
#38733=ORIENTED_EDGE('',*,*,#27684,.T.) ;
#38734=ORIENTED_EDGE('',*,*,#27680,.F.) ;
#38735=ORIENTED_EDGE('',*,*,#27685,.T.) ;
#38736=ORIENTED_EDGE('',*,*,#27685,.F.) ;
#38737=ORIENTED_EDGE('',*,*,#27682,.F.) ;
#38738=ORIENTED_EDGE('',*,*,#27686,.F.) ;
#38739=ORIENTED_EDGE('',*,*,#27687,.F.) ;
#38740=ORIENTED_EDGE('',*,*,#27688,.F.) ;
#38741=ORIENTED_EDGE('',*,*,#27679,.F.) ;
#38742=ORIENTED_EDGE('',*,*,#27689,.T.) ;
#38743=ORIENTED_EDGE('',*,*,#27690,.T.) ;
#38744=ORIENTED_EDGE('',*,*,#27686,.T.) ;
#38745=ORIENTED_EDGE('',*,*,#27676,.F.) ;
#38746=ORIENTED_EDGE('',*,*,#27668,.F.) ;
#38747=ORIENTED_EDGE('',*,*,#27691,.F.) ;
#38748=ORIENTED_EDGE('',*,*,#27692,.F.) ;
#38749=ORIENTED_EDGE('',*,*,#27689,.F.) ;
#38750=ORIENTED_EDGE('',*,*,#27693,.T.) ;
#38751=ORIENTED_EDGE('',*,*,#27694,.F.) ;
#38752=ORIENTED_EDGE('',*,*,#27695,.T.) ;
#38753=ORIENTED_EDGE('',*,*,#27696,.T.) ;
#38754=ORIENTED_EDGE('',*,*,#27673,.F.) ;
#38755=ORIENTED_EDGE('',*,*,#27697,.T.) ;
#38756=ORIENTED_EDGE('',*,*,#27693,.F.) ;
#38757=ORIENTED_EDGE('',*,*,#27672,.F.) ;
#38758=ORIENTED_EDGE('',*,*,#27698,.F.) ;
#38759=ORIENTED_EDGE('',*,*,#27699,.T.) ;
#38760=ORIENTED_EDGE('',*,*,#27700,.F.) ;
#38761=ORIENTED_EDGE('',*,*,#27701,.F.) ;
#38762=ORIENTED_EDGE('',*,*,#27702,.F.) ;
#38763=ORIENTED_EDGE('',*,*,#27703,.F.) ;
#38764=ORIENTED_EDGE('',*,*,#27704,.F.) ;
#38765=ORIENTED_EDGE('',*,*,#27705,.F.) ;
#38766=ORIENTED_EDGE('',*,*,#27706,.F.) ;
#38767=ORIENTED_EDGE('',*,*,#27707,.F.) ;
#38768=ORIENTED_EDGE('',*,*,#27708,.F.) ;
#38769=ORIENTED_EDGE('',*,*,#27709,.F.) ;
#38770=ORIENTED_EDGE('',*,*,#27710,.F.) ;
#38771=ORIENTED_EDGE('',*,*,#27711,.F.) ;
#38772=ORIENTED_EDGE('',*,*,#27694,.T.) ;
#38773=ORIENTED_EDGE('',*,*,#27697,.F.) ;
#38774=ORIENTED_EDGE('',*,*,#27712,.T.) ;
#38775=ORIENTED_EDGE('',*,*,#27713,.T.) ;
#38776=ORIENTED_EDGE('',*,*,#27714,.T.) ;
#38777=ORIENTED_EDGE('',*,*,#27715,.T.) ;
#38778=ORIENTED_EDGE('',*,*,#27716,.T.) ;
#38779=ORIENTED_EDGE('',*,*,#27717,.T.) ;
#38780=ORIENTED_EDGE('',*,*,#27718,.T.) ;
#38781=ORIENTED_EDGE('',*,*,#27712,.F.) ;
#38782=ORIENTED_EDGE('',*,*,#27719,.T.) ;
#38783=ORIENTED_EDGE('',*,*,#27720,.T.) ;
#38784=ORIENTED_EDGE('',*,*,#27721,.T.) ;
#38785=ORIENTED_EDGE('',*,*,#27717,.F.) ;
#38786=ORIENTED_EDGE('',*,*,#27722,.T.) ;
#38787=ORIENTED_EDGE('',*,*,#27723,.T.) ;
#38788=ORIENTED_EDGE('',*,*,#27724,.T.) ;
#38789=ORIENTED_EDGE('',*,*,#27720,.F.) ;
#38790=ORIENTED_EDGE('',*,*,#27723,.F.) ;
#38791=ORIENTED_EDGE('',*,*,#27722,.F.) ;
#38792=ORIENTED_EDGE('',*,*,#27725,.T.) ;
#38793=ORIENTED_EDGE('',*,*,#27726,.T.) ;
#38794=ORIENTED_EDGE('',*,*,#27727,.T.) ;
#38795=ORIENTED_EDGE('',*,*,#27719,.F.) ;
#38796=ORIENTED_EDGE('',*,*,#27728,.F.) ;
#38797=ORIENTED_EDGE('',*,*,#27729,.F.) ;
#38798=ORIENTED_EDGE('',*,*,#27730,.F.) ;
#38799=ORIENTED_EDGE('',*,*,#27725,.F.) ;
#38800=ORIENTED_EDGE('',*,*,#27715,.F.) ;
#38801=ORIENTED_EDGE('',*,*,#27731,.T.) ;
#38802=ORIENTED_EDGE('',*,*,#27732,.F.) ;
#38803=ORIENTED_EDGE('',*,*,#27728,.T.) ;
#38804=ORIENTED_EDGE('',*,*,#27716,.F.) ;
#38805=ORIENTED_EDGE('',*,*,#27733,.T.) ;
#38806=ORIENTED_EDGE('',*,*,#27734,.T.) ;
#38807=ORIENTED_EDGE('',*,*,#27735,.T.) ;
#38808=ORIENTED_EDGE('',*,*,#27736,.T.) ;
#38809=ORIENTED_EDGE('',*,*,#27737,.T.) ;
#38810=ORIENTED_EDGE('',*,*,#27738,.T.) ;
#38811=ORIENTED_EDGE('',*,*,#27739,.T.) ;
#38812=ORIENTED_EDGE('',*,*,#27733,.F.) ;
#38813=ORIENTED_EDGE('',*,*,#27740,.T.) ;
#38814=ORIENTED_EDGE('',*,*,#27741,.T.) ;
#38815=ORIENTED_EDGE('',*,*,#27742,.T.) ;
#38816=ORIENTED_EDGE('',*,*,#27738,.F.) ;
#38817=ORIENTED_EDGE('',*,*,#27743,.T.) ;
#38818=ORIENTED_EDGE('',*,*,#27741,.F.) ;
#38819=ORIENTED_EDGE('',*,*,#27744,.T.) ;
#38820=ORIENTED_EDGE('',*,*,#27745,.T.) ;
#38821=ORIENTED_EDGE('',*,*,#27746,.T.) ;
#38822=ORIENTED_EDGE('',*,*,#27747,.T.) ;
#38823=ORIENTED_EDGE('',*,*,#27721,.F.) ;
#38824=ORIENTED_EDGE('',*,*,#27748,.F.) ;
#38825=ORIENTED_EDGE('',*,*,#27749,.F.) ;
#38826=ORIENTED_EDGE('',*,*,#27750,.F.) ;
#38827=ORIENTED_EDGE('',*,*,#27751,.F.) ;
#38828=ORIENTED_EDGE('',*,*,#27752,.F.) ;
#38829=ORIENTED_EDGE('',*,*,#27753,.F.) ;
#38830=ORIENTED_EDGE('',*,*,#27754,.F.) ;
#38831=ORIENTED_EDGE('',*,*,#27743,.F.) ;
#38832=ORIENTED_EDGE('',*,*,#27740,.F.) ;
#38833=ORIENTED_EDGE('',*,*,#27755,.F.) ;
#38834=ORIENTED_EDGE('',*,*,#27756,.F.) ;
#38835=ORIENTED_EDGE('',*,*,#27757,.F.) ;
#38836=ORIENTED_EDGE('',*,*,#27758,.F.) ;
#38837=ORIENTED_EDGE('',*,*,#27759,.F.) ;
#38838=ORIENTED_EDGE('',*,*,#27718,.F.) ;
#38839=ORIENTED_EDGE('',*,*,#27736,.F.) ;
#38840=ORIENTED_EDGE('',*,*,#27760,.T.) ;
#38841=ORIENTED_EDGE('',*,*,#27761,.T.) ;
#38842=ORIENTED_EDGE('',*,*,#27755,.T.) ;
#38843=ORIENTED_EDGE('',*,*,#27737,.F.) ;
#38844=ORIENTED_EDGE('',*,*,#27734,.F.) ;
#38845=ORIENTED_EDGE('',*,*,#27762,.T.) ;
#38846=ORIENTED_EDGE('',*,*,#27763,.F.) ;
#38847=ORIENTED_EDGE('',*,*,#27764,.T.) ;
#38848=ORIENTED_EDGE('',*,*,#27735,.F.) ;
#38849=ORIENTED_EDGE('',*,*,#27765,.T.) ;
#38850=ORIENTED_EDGE('',*,*,#27766,.T.) ;
#38851=ORIENTED_EDGE('',*,*,#27767,.T.) ;
#38852=ORIENTED_EDGE('',*,*,#27766,.F.) ;
#38853=ORIENTED_EDGE('',*,*,#27768,.T.) ;
#38854=ORIENTED_EDGE('',*,*,#27769,.T.) ;
#38855=ORIENTED_EDGE('',*,*,#27770,.T.) ;
#38856=ORIENTED_EDGE('',*,*,#27765,.F.) ;
#38857=ORIENTED_EDGE('',*,*,#27771,.T.) ;
#38858=ORIENTED_EDGE('',*,*,#27772,.T.) ;
#38859=ORIENTED_EDGE('',*,*,#27773,.T.) ;
#38860=ORIENTED_EDGE('',*,*,#27774,.T.) ;
#38861=ORIENTED_EDGE('',*,*,#27775,.T.) ;
#38862=ORIENTED_EDGE('',*,*,#27769,.F.) ;
#38863=ORIENTED_EDGE('',*,*,#27776,.T.) ;
#38864=ORIENTED_EDGE('',*,*,#27777,.F.) ;
#38865=ORIENTED_EDGE('',*,*,#27778,.F.) ;
#38866=ORIENTED_EDGE('',*,*,#27779,.F.) ;
#38867=ORIENTED_EDGE('',*,*,#27780,.F.) ;
#38868=ORIENTED_EDGE('',*,*,#27781,.F.) ;
#38869=ORIENTED_EDGE('',*,*,#27782,.F.) ;
#38870=ORIENTED_EDGE('',*,*,#27783,.F.) ;
#38871=ORIENTED_EDGE('',*,*,#27768,.F.) ;
#38872=ORIENTED_EDGE('',*,*,#27775,.F.) ;
#38873=ORIENTED_EDGE('',*,*,#27784,.F.) ;
#38874=ORIENTED_EDGE('',*,*,#27776,.F.) ;
#38875=ORIENTED_EDGE('',*,*,#27774,.F.) ;
#38876=ORIENTED_EDGE('',*,*,#27785,.T.) ;
#38877=ORIENTED_EDGE('',*,*,#27786,.F.) ;
#38878=ORIENTED_EDGE('',*,*,#27777,.T.) ;
#38879=ORIENTED_EDGE('',*,*,#27784,.T.) ;
#38880=ORIENTED_EDGE('',*,*,#27773,.F.) ;
#38881=ORIENTED_EDGE('',*,*,#27787,.T.) ;
#38882=ORIENTED_EDGE('',*,*,#27788,.T.) ;
#38883=ORIENTED_EDGE('',*,*,#27785,.F.) ;
#38884=ORIENTED_EDGE('',*,*,#27641,.F.) ;
#38885=ORIENTED_EDGE('',*,*,#27789,.T.) ;
#38886=ORIENTED_EDGE('',*,*,#27790,.F.) ;
#38887=ORIENTED_EDGE('',*,*,#27791,.T.) ;
#38888=ORIENTED_EDGE('',*,*,#27652,.F.) ;
#38889=ORIENTED_EDGE('',*,*,#27792,.F.) ;
#38890=ORIENTED_EDGE('',*,*,#27793,.F.) ;
#38891=ORIENTED_EDGE('',*,*,#27789,.F.) ;
#38892=ORIENTED_EDGE('',*,*,#27645,.F.) ;
#38893=ORIENTED_EDGE('',*,*,#27648,.F.) ;
#38894=ORIENTED_EDGE('',*,*,#27794,.T.) ;
#38895=ORIENTED_EDGE('',*,*,#27795,.T.) ;
#38896=ORIENTED_EDGE('',*,*,#27796,.T.) ;
#38897=ORIENTED_EDGE('',*,*,#27797,.T.) ;
#38898=ORIENTED_EDGE('',*,*,#27684,.F.) ;
#38899=ORIENTED_EDGE('',*,*,#27798,.T.) ;
#38900=ORIENTED_EDGE('',*,*,#27795,.F.) ;
#38901=ORIENTED_EDGE('',*,*,#27799,.T.) ;
#38902=ORIENTED_EDGE('',*,*,#27797,.F.) ;
#38903=ORIENTED_EDGE('',*,*,#27800,.F.) ;
#38904=ORIENTED_EDGE('',*,*,#27801,.F.) ;
#38905=ORIENTED_EDGE('',*,*,#27802,.F.) ;
#38906=ORIENTED_EDGE('',*,*,#27803,.F.) ;
#38907=ORIENTED_EDGE('',*,*,#27796,.F.) ;
#38908=ORIENTED_EDGE('',*,*,#27804,.T.) ;
#38909=ORIENTED_EDGE('',*,*,#27805,.T.) ;
#38910=ORIENTED_EDGE('',*,*,#27800,.T.) ;
#38911=ORIENTED_EDGE('',*,*,#27688,.T.) ;
#38912=ORIENTED_EDGE('',*,*,#27806,.T.) ;
#38913=ORIENTED_EDGE('',*,*,#27807,.T.) ;
#38914=ORIENTED_EDGE('',*,*,#27808,.T.) ;
#38915=ORIENTED_EDGE('',*,*,#27809,.F.) ;
#38916=ORIENTED_EDGE('',*,*,#27810,.F.) ;
#38917=ORIENTED_EDGE('',*,*,#27804,.F.) ;
#38918=ORIENTED_EDGE('',*,*,#27798,.F.) ;
#38919=ORIENTED_EDGE('',*,*,#27683,.F.) ;
#38920=ORIENTED_EDGE('',*,*,#27811,.T.) ;
#38921=ORIENTED_EDGE('',*,*,#27812,.T.) ;
#38922=ORIENTED_EDGE('',*,*,#27813,.T.) ;
#38923=ORIENTED_EDGE('',*,*,#27814,.T.) ;
#38924=ORIENTED_EDGE('',*,*,#27724,.F.) ;
#38925=ORIENTED_EDGE('',*,*,#27815,.T.) ;
#38926=ORIENTED_EDGE('',*,*,#27812,.F.) ;
#38927=ORIENTED_EDGE('',*,*,#27748,.T.) ;
#38928=ORIENTED_EDGE('',*,*,#27813,.F.) ;
#38929=ORIENTED_EDGE('',*,*,#27816,.T.) ;
#38930=ORIENTED_EDGE('',*,*,#27817,.F.) ;
#38931=ORIENTED_EDGE('',*,*,#27818,.T.) ;
#38932=ORIENTED_EDGE('',*,*,#27815,.F.) ;
#38933=ORIENTED_EDGE('',*,*,#27727,.F.) ;
#38934=ORIENTED_EDGE('',*,*,#27819,.F.) ;
#38935=ORIENTED_EDGE('',*,*,#27820,.F.) ;
#38936=ORIENTED_EDGE('',*,*,#27821,.F.) ;
#38937=ORIENTED_EDGE('',*,*,#27822,.F.) ;
#38938=ORIENTED_EDGE('',*,*,#27816,.F.) ;
#38939=ORIENTED_EDGE('',*,*,#27823,.T.) ;
#38940=ORIENTED_EDGE('',*,*,#27824,.T.) ;
#38941=ORIENTED_EDGE('',*,*,#27825,.T.) ;
#38942=ORIENTED_EDGE('',*,*,#27826,.T.) ;
#38943=ORIENTED_EDGE('',*,*,#27744,.F.) ;
#38944=ORIENTED_EDGE('',*,*,#27754,.T.) ;
#38945=ORIENTED_EDGE('',*,*,#27826,.F.) ;
#38946=ORIENTED_EDGE('',*,*,#27706,.T.) ;
#38947=ORIENTED_EDGE('',*,*,#27745,.F.) ;
#38948=ORIENTED_EDGE('',*,*,#27823,.F.) ;
#38949=ORIENTED_EDGE('',*,*,#27753,.T.) ;
#38950=ORIENTED_EDGE('',*,*,#27827,.T.) ;
#38951=ORIENTED_EDGE('',*,*,#27828,.T.) ;
#38952=ORIENTED_EDGE('',*,*,#27732,.T.) ;
#38953=ORIENTED_EDGE('',*,*,#27829,.T.) ;
#38954=ORIENTED_EDGE('',*,*,#27830,.T.) ;
#38955=ORIENTED_EDGE('',*,*,#27831,.T.) ;
#38956=ORIENTED_EDGE('',*,*,#27832,.T.) ;
#38957=ORIENTED_EDGE('',*,*,#27833,.T.) ;
#38958=ORIENTED_EDGE('',*,*,#27726,.F.) ;
#38959=ORIENTED_EDGE('',*,*,#27730,.T.) ;
#38960=ORIENTED_EDGE('',*,*,#27831,.F.) ;
#38961=ORIENTED_EDGE('',*,*,#27834,.T.) ;
#38962=ORIENTED_EDGE('',*,*,#27832,.F.) ;
#38963=ORIENTED_EDGE('',*,*,#27729,.T.) ;
#38964=ORIENTED_EDGE('',*,*,#27763,.T.) ;
#38965=ORIENTED_EDGE('',*,*,#27835,.T.) ;
#38966=ORIENTED_EDGE('',*,*,#27836,.T.) ;
#38967=ORIENTED_EDGE('',*,*,#27837,.T.) ;
#38968=ORIENTED_EDGE('',*,*,#27838,.T.) ;
#38969=ORIENTED_EDGE('',*,*,#27839,.T.) ;
#38970=ORIENTED_EDGE('',*,*,#27835,.F.) ;
#38971=ORIENTED_EDGE('',*,*,#27840,.T.) ;
#38972=ORIENTED_EDGE('',*,*,#27841,.T.) ;
#38973=ORIENTED_EDGE('',*,*,#27842,.T.) ;
#38974=ORIENTED_EDGE('',*,*,#27838,.F.) ;
#38975=ORIENTED_EDGE('',*,*,#27843,.T.) ;
#38976=ORIENTED_EDGE('',*,*,#27746,.F.) ;
#38977=ORIENTED_EDGE('',*,*,#27705,.T.) ;
#38978=ORIENTED_EDGE('',*,*,#27841,.F.) ;
#38979=ORIENTED_EDGE('',*,*,#27844,.T.) ;
#38980=ORIENTED_EDGE('',*,*,#27742,.F.) ;
#38981=ORIENTED_EDGE('',*,*,#27747,.F.) ;
#38982=ORIENTED_EDGE('',*,*,#27837,.F.) ;
#38983=ORIENTED_EDGE('',*,*,#27845,.F.) ;
#38984=ORIENTED_EDGE('',*,*,#27846,.F.) ;
#38985=ORIENTED_EDGE('',*,*,#27847,.T.) ;
#38986=ORIENTED_EDGE('',*,*,#27848,.T.) ;
#38987=ORIENTED_EDGE('',*,*,#27849,.F.) ;
#38988=ORIENTED_EDGE('',*,*,#27850,.T.) ;
#38989=ORIENTED_EDGE('',*,*,#27760,.F.) ;
#38990=ORIENTED_EDGE('',*,*,#27764,.F.) ;
#38991=ORIENTED_EDGE('',*,*,#27836,.F.) ;
#38992=ORIENTED_EDGE('',*,*,#27851,.T.) ;
#38993=ORIENTED_EDGE('',*,*,#27852,.F.) ;
#38994=ORIENTED_EDGE('',*,*,#27845,.T.) ;
#38995=ORIENTED_EDGE('',*,*,#27839,.F.) ;
#38996=ORIENTED_EDGE('',*,*,#27853,.F.) ;
#38997=ORIENTED_EDGE('',*,*,#27854,.F.) ;
#38998=ORIENTED_EDGE('',*,*,#27855,.F.) ;
#38999=ORIENTED_EDGE('',*,*,#27856,.F.) ;
#39000=ORIENTED_EDGE('',*,*,#27857,.F.) ;
#39001=ORIENTED_EDGE('',*,*,#27858,.F.) ;
#39002=ORIENTED_EDGE('',*,*,#27851,.F.) ;
#39003=ORIENTED_EDGE('',*,*,#27842,.F.) ;
#39004=ORIENTED_EDGE('',*,*,#27704,.T.) ;
#39005=ORIENTED_EDGE('',*,*,#27859,.F.) ;
#39006=ORIENTED_EDGE('',*,*,#27860,.F.) ;
#39007=ORIENTED_EDGE('',*,*,#27853,.T.) ;
#39008=ORIENTED_EDGE('',*,*,#27861,.F.) ;
#39009=ORIENTED_EDGE('',*,*,#27862,.F.) ;
#39010=ORIENTED_EDGE('',*,*,#27863,.F.) ;
#39011=ORIENTED_EDGE('',*,*,#27864,.T.) ;
#39012=ORIENTED_EDGE('',*,*,#27865,.T.) ;
#39013=ORIENTED_EDGE('',*,*,#27862,.T.) ;
#39014=ORIENTED_EDGE('',*,*,#27866,.T.) ;
#39015=ORIENTED_EDGE('',*,*,#27867,.T.) ;
#39016=ORIENTED_EDGE('',*,*,#27868,.T.) ;
#39017=ORIENTED_EDGE('',*,*,#27869,.T.) ;
#39018=ORIENTED_EDGE('',*,*,#27870,.T.) ;
#39019=ORIENTED_EDGE('',*,*,#27871,.T.) ;
#39020=ORIENTED_EDGE('',*,*,#27872,.T.) ;
#39021=ORIENTED_EDGE('',*,*,#27869,.F.) ;
#39022=ORIENTED_EDGE('',*,*,#27873,.T.) ;
#39023=ORIENTED_EDGE('',*,*,#27874,.T.) ;
#39024=ORIENTED_EDGE('',*,*,#27875,.T.) ;
#39025=ORIENTED_EDGE('',*,*,#27871,.F.) ;
#39026=ORIENTED_EDGE('',*,*,#27876,.T.) ;
#39027=ORIENTED_EDGE('',*,*,#27877,.T.) ;
#39028=ORIENTED_EDGE('',*,*,#27878,.T.) ;
#39029=ORIENTED_EDGE('',*,*,#27874,.F.) ;
#39030=ORIENTED_EDGE('',*,*,#27879,.T.) ;
#39031=ORIENTED_EDGE('',*,*,#27880,.T.) ;
#39032=ORIENTED_EDGE('',*,*,#27881,.T.) ;
#39033=ORIENTED_EDGE('',*,*,#27877,.F.) ;
#39034=ORIENTED_EDGE('',*,*,#27882,.T.) ;
#39035=ORIENTED_EDGE('',*,*,#27883,.T.) ;
#39036=ORIENTED_EDGE('',*,*,#27884,.T.) ;
#39037=ORIENTED_EDGE('',*,*,#27880,.F.) ;
#39038=ORIENTED_EDGE('',*,*,#27885,.T.) ;
#39039=ORIENTED_EDGE('',*,*,#27863,.T.) ;
#39040=ORIENTED_EDGE('',*,*,#27886,.T.) ;
#39041=ORIENTED_EDGE('',*,*,#27883,.F.) ;
#39042=ORIENTED_EDGE('',*,*,#27887,.T.) ;
#39043=ORIENTED_EDGE('',*,*,#27888,.T.) ;
#39044=ORIENTED_EDGE('',*,*,#27889,.T.) ;
#39045=ORIENTED_EDGE('',*,*,#27861,.T.) ;
#39046=ORIENTED_EDGE('',*,*,#27890,.T.) ;
#39047=ORIENTED_EDGE('',*,*,#27891,.T.) ;
#39048=ORIENTED_EDGE('',*,*,#27892,.T.) ;
#39049=ORIENTED_EDGE('',*,*,#27888,.F.) ;
#39050=ORIENTED_EDGE('',*,*,#27893,.T.) ;
#39051=ORIENTED_EDGE('',*,*,#27870,.F.) ;
#39052=ORIENTED_EDGE('',*,*,#27872,.F.) ;
#39053=ORIENTED_EDGE('',*,*,#27875,.F.) ;
#39054=ORIENTED_EDGE('',*,*,#27878,.F.) ;
#39055=ORIENTED_EDGE('',*,*,#27881,.F.) ;
#39056=ORIENTED_EDGE('',*,*,#27884,.F.) ;
#39057=ORIENTED_EDGE('',*,*,#27886,.F.) ;
#39058=ORIENTED_EDGE('',*,*,#27865,.F.) ;
#39059=ORIENTED_EDGE('',*,*,#27894,.F.) ;
#39060=ORIENTED_EDGE('',*,*,#27895,.T.) ;
#39061=ORIENTED_EDGE('',*,*,#27896,.F.) ;
#39062=ORIENTED_EDGE('',*,*,#27897,.T.) ;
#39063=ORIENTED_EDGE('',*,*,#27898,.F.) ;
#39064=ORIENTED_EDGE('',*,*,#27899,.F.) ;
#39065=ORIENTED_EDGE('',*,*,#27900,.T.) ;
#39066=ORIENTED_EDGE('',*,*,#27901,.F.) ;
#39067=ORIENTED_EDGE('',*,*,#27902,.T.) ;
#39068=ORIENTED_EDGE('',*,*,#27903,.F.) ;
#39069=ORIENTED_EDGE('',*,*,#27864,.F.) ;
#39070=ORIENTED_EDGE('',*,*,#27904,.T.) ;
#39071=ORIENTED_EDGE('',*,*,#27905,.T.) ;
#39072=ORIENTED_EDGE('',*,*,#27894,.T.) ;
#39073=ORIENTED_EDGE('',*,*,#27866,.F.) ;
#39074=ORIENTED_EDGE('',*,*,#27889,.F.) ;
#39075=ORIENTED_EDGE('',*,*,#27892,.F.) ;
#39076=ORIENTED_EDGE('',*,*,#27906,.F.) ;
#39077=ORIENTED_EDGE('',*,*,#27907,.F.) ;
#39078=ORIENTED_EDGE('',*,*,#27908,.F.) ;
#39079=ORIENTED_EDGE('',*,*,#27909,.T.) ;
#39080=ORIENTED_EDGE('',*,*,#27910,.T.) ;
#39081=ORIENTED_EDGE('',*,*,#27911,.T.) ;
#39082=ORIENTED_EDGE('',*,*,#27912,.F.) ;
#39083=ORIENTED_EDGE('',*,*,#27913,.T.) ;
#39084=ORIENTED_EDGE('',*,*,#27914,.T.) ;
#39085=ORIENTED_EDGE('',*,*,#27910,.F.) ;
#39086=ORIENTED_EDGE('',*,*,#27915,.T.) ;
#39087=ORIENTED_EDGE('',*,*,#27915,.F.) ;
#39088=ORIENTED_EDGE('',*,*,#27909,.F.) ;
#39089=ORIENTED_EDGE('',*,*,#27916,.F.) ;
#39090=ORIENTED_EDGE('',*,*,#27917,.F.) ;
#39091=ORIENTED_EDGE('',*,*,#27918,.T.) ;
#39092=ORIENTED_EDGE('',*,*,#27893,.F.) ;
#39093=ORIENTED_EDGE('',*,*,#27919,.T.) ;
#39094=ORIENTED_EDGE('',*,*,#27920,.T.) ;
#39095=ORIENTED_EDGE('',*,*,#27921,.T.) ;
#39096=ORIENTED_EDGE('',*,*,#27922,.T.) ;
#39097=ORIENTED_EDGE('',*,*,#27923,.T.) ;
#39098=ORIENTED_EDGE('',*,*,#27924,.T.) ;
#39099=ORIENTED_EDGE('',*,*,#27920,.F.) ;
#39100=ORIENTED_EDGE('',*,*,#27887,.F.) ;
#39101=ORIENTED_EDGE('',*,*,#27925,.T.) ;
#39102=ORIENTED_EDGE('',*,*,#27926,.F.) ;
#39103=ORIENTED_EDGE('',*,*,#27927,.F.) ;
#39104=ORIENTED_EDGE('',*,*,#27922,.F.) ;
#39105=ORIENTED_EDGE('',*,*,#27919,.F.) ;
#39106=ORIENTED_EDGE('',*,*,#27890,.F.) ;
#39107=ORIENTED_EDGE('',*,*,#27928,.T.) ;
#39108=ORIENTED_EDGE('',*,*,#27929,.F.) ;
#39109=ORIENTED_EDGE('',*,*,#27930,.F.) ;
#39110=ORIENTED_EDGE('',*,*,#27931,.F.) ;
#39111=ORIENTED_EDGE('',*,*,#27932,.T.) ;
#39112=ORIENTED_EDGE('',*,*,#27857,.T.) ;
#39113=ORIENTED_EDGE('',*,*,#27929,.T.) ;
#39114=ORIENTED_EDGE('',*,*,#27933,.T.) ;
#39115=ORIENTED_EDGE('',*,*,#27852,.T.) ;
#39116=ORIENTED_EDGE('',*,*,#27858,.T.) ;
#39117=ORIENTED_EDGE('',*,*,#27932,.F.) ;
#39118=ORIENTED_EDGE('',*,*,#27934,.T.) ;
#39119=ORIENTED_EDGE('',*,*,#27935,.T.) ;
#39120=ORIENTED_EDGE('',*,*,#27936,.T.) ;
#39121=ORIENTED_EDGE('',*,*,#27930,.T.) ;
#39122=ORIENTED_EDGE('',*,*,#27856,.T.) ;
#39123=ORIENTED_EDGE('',*,*,#27935,.F.) ;
#39124=ORIENTED_EDGE('',*,*,#27937,.T.) ;
#39125=ORIENTED_EDGE('',*,*,#27938,.T.) ;
#39126=ORIENTED_EDGE('',*,*,#27939,.T.) ;
#39127=ORIENTED_EDGE('',*,*,#27940,.T.) ;
#39128=ORIENTED_EDGE('',*,*,#27941,.T.) ;
#39129=ORIENTED_EDGE('',*,*,#27938,.F.) ;
#39130=ORIENTED_EDGE('',*,*,#27942,.T.) ;
#39131=ORIENTED_EDGE('',*,*,#27943,.T.) ;
#39132=ORIENTED_EDGE('',*,*,#27944,.T.) ;
#39133=ORIENTED_EDGE('',*,*,#27940,.F.) ;
#39134=ORIENTED_EDGE('',*,*,#27945,.T.) ;
#39135=ORIENTED_EDGE('',*,*,#27946,.T.) ;
#39136=ORIENTED_EDGE('',*,*,#27947,.T.) ;
#39137=ORIENTED_EDGE('',*,*,#27943,.F.) ;
#39138=ORIENTED_EDGE('',*,*,#27948,.T.) ;
#39139=ORIENTED_EDGE('',*,*,#27949,.T.) ;
#39140=ORIENTED_EDGE('',*,*,#27950,.T.) ;
#39141=ORIENTED_EDGE('',*,*,#27951,.T.) ;
#39142=ORIENTED_EDGE('',*,*,#27952,.T.) ;
#39143=ORIENTED_EDGE('',*,*,#27626,.T.) ;
#39144=ORIENTED_EDGE('',*,*,#27953,.T.) ;
#39145=ORIENTED_EDGE('',*,*,#27627,.T.) ;
#39146=ORIENTED_EDGE('',*,*,#27952,.F.) ;
#39147=ORIENTED_EDGE('',*,*,#27954,.T.) ;
#39148=ORIENTED_EDGE('',*,*,#27955,.T.) ;
#39149=ORIENTED_EDGE('',*,*,#27628,.T.) ;
#39150=ORIENTED_EDGE('',*,*,#27953,.F.) ;
#39151=ORIENTED_EDGE('',*,*,#27956,.T.) ;
#39152=ORIENTED_EDGE('',*,*,#27957,.T.) ;
#39153=ORIENTED_EDGE('',*,*,#27611,.T.) ;
#39154=ORIENTED_EDGE('',*,*,#27955,.F.) ;
#39155=ORIENTED_EDGE('',*,*,#27958,.T.) ;
#39156=ORIENTED_EDGE('',*,*,#27959,.T.) ;
#39157=ORIENTED_EDGE('',*,*,#27960,.T.) ;
#39158=ORIENTED_EDGE('',*,*,#27957,.F.) ;
#39159=ORIENTED_EDGE('',*,*,#27961,.T.) ;
#39160=ORIENTED_EDGE('',*,*,#27962,.T.) ;
#39161=ORIENTED_EDGE('',*,*,#27963,.T.) ;
#39162=ORIENTED_EDGE('',*,*,#27959,.F.) ;
#39163=ORIENTED_EDGE('',*,*,#27964,.T.) ;
#39164=ORIENTED_EDGE('',*,*,#27931,.T.) ;
#39165=ORIENTED_EDGE('',*,*,#27965,.T.) ;
#39166=ORIENTED_EDGE('',*,*,#27962,.F.) ;
#39167=ORIENTED_EDGE('',*,*,#27966,.T.) ;
#39168=ORIENTED_EDGE('',*,*,#27934,.F.) ;
#39169=ORIENTED_EDGE('',*,*,#27967,.F.) ;
#39170=ORIENTED_EDGE('',*,*,#27968,.F.) ;
#39171=ORIENTED_EDGE('',*,*,#27846,.T.) ;
#39172=ORIENTED_EDGE('',*,*,#27933,.F.) ;
#39173=ORIENTED_EDGE('',*,*,#27928,.F.) ;
#39174=ORIENTED_EDGE('',*,*,#27966,.F.) ;
#39175=ORIENTED_EDGE('',*,*,#27964,.F.) ;
#39176=ORIENTED_EDGE('',*,*,#27961,.F.) ;
#39177=ORIENTED_EDGE('',*,*,#27958,.F.) ;
#39178=ORIENTED_EDGE('',*,*,#27969,.F.) ;
#39179=ORIENTED_EDGE('',*,*,#27970,.T.) ;
#39180=ORIENTED_EDGE('',*,*,#27967,.T.) ;
#39181=ORIENTED_EDGE('',*,*,#27956,.F.) ;
#39182=ORIENTED_EDGE('',*,*,#27971,.F.) ;
#39183=ORIENTED_EDGE('',*,*,#27972,.T.) ;
#39184=ORIENTED_EDGE('',*,*,#27969,.T.) ;
#39185=ORIENTED_EDGE('',*,*,#27954,.F.) ;
#39186=ORIENTED_EDGE('',*,*,#27973,.F.) ;
#39187=ORIENTED_EDGE('',*,*,#27974,.F.) ;
#39188=ORIENTED_EDGE('',*,*,#27975,.F.) ;
#39189=ORIENTED_EDGE('',*,*,#27976,.T.) ;
#39190=ORIENTED_EDGE('',*,*,#27971,.T.) ;
#39191=ORIENTED_EDGE('',*,*,#27951,.F.) ;
#39192=ORIENTED_EDGE('',*,*,#27977,.F.) ;
#39193=ORIENTED_EDGE('',*,*,#27978,.F.) ;
#39194=ORIENTED_EDGE('',*,*,#27973,.T.) ;
#39195=ORIENTED_EDGE('',*,*,#27950,.F.) ;
#39196=ORIENTED_EDGE('',*,*,#27625,.T.) ;
#39197=ORIENTED_EDGE('',*,*,#27979,.F.) ;
#39198=ORIENTED_EDGE('',*,*,#27980,.T.) ;
#39199=ORIENTED_EDGE('',*,*,#27981,.T.) ;
#39200=ORIENTED_EDGE('',*,*,#27982,.T.) ;
#39201=ORIENTED_EDGE('',*,*,#27983,.T.) ;
#39202=ORIENTED_EDGE('',*,*,#27984,.T.) ;
#39203=ORIENTED_EDGE('',*,*,#27985,.T.) ;
#39204=ORIENTED_EDGE('',*,*,#27986,.T.) ;
#39205=ORIENTED_EDGE('',*,*,#27987,.T.) ;
#39206=ORIENTED_EDGE('',*,*,#27981,.F.) ;
#39207=ORIENTED_EDGE('',*,*,#27988,.T.) ;
#39208=ORIENTED_EDGE('',*,*,#27989,.T.) ;
#39209=ORIENTED_EDGE('',*,*,#27990,.T.) ;
#39210=ORIENTED_EDGE('',*,*,#27986,.F.) ;
#39211=ORIENTED_EDGE('',*,*,#27991,.T.) ;
#39212=ORIENTED_EDGE('',*,*,#27992,.T.) ;
#39213=ORIENTED_EDGE('',*,*,#27993,.T.) ;
#39214=ORIENTED_EDGE('',*,*,#27989,.F.) ;
#39215=ORIENTED_EDGE('',*,*,#27994,.T.) ;
#39216=ORIENTED_EDGE('',*,*,#27995,.T.) ;
#39217=ORIENTED_EDGE('',*,*,#27996,.T.) ;
#39218=ORIENTED_EDGE('',*,*,#27992,.F.) ;
#39219=ORIENTED_EDGE('',*,*,#27997,.T.) ;
#39220=ORIENTED_EDGE('',*,*,#27995,.F.) ;
#39221=ORIENTED_EDGE('',*,*,#27998,.T.) ;
#39222=ORIENTED_EDGE('',*,*,#27999,.T.) ;
#39223=ORIENTED_EDGE('',*,*,#28000,.T.) ;
#39224=ORIENTED_EDGE('',*,*,#27998,.F.) ;
#39225=ORIENTED_EDGE('',*,*,#27997,.F.) ;
#39226=ORIENTED_EDGE('',*,*,#27994,.F.) ;
#39227=ORIENTED_EDGE('',*,*,#28001,.T.) ;
#39228=ORIENTED_EDGE('',*,*,#28002,.F.) ;
#39229=ORIENTED_EDGE('',*,*,#28003,.F.) ;
#39230=ORIENTED_EDGE('',*,*,#28004,.T.) ;
#39231=ORIENTED_EDGE('',*,*,#27993,.F.) ;
#39232=ORIENTED_EDGE('',*,*,#28005,.F.) ;
#39233=ORIENTED_EDGE('',*,*,#28006,.F.) ;
#39234=ORIENTED_EDGE('',*,*,#28007,.T.) ;
#39235=ORIENTED_EDGE('',*,*,#28008,.F.) ;
#39236=ORIENTED_EDGE('',*,*,#28009,.F.) ;
#39237=ORIENTED_EDGE('',*,*,#28010,.F.) ;
#39238=ORIENTED_EDGE('',*,*,#27987,.F.) ;
#39239=ORIENTED_EDGE('',*,*,#27990,.F.) ;
#39240=ORIENTED_EDGE('',*,*,#27991,.F.) ;
#39241=ORIENTED_EDGE('',*,*,#28011,.F.) ;
#39242=ORIENTED_EDGE('',*,*,#28001,.F.) ;
#39243=ORIENTED_EDGE('',*,*,#27988,.F.) ;
#39244=ORIENTED_EDGE('',*,*,#27985,.F.) ;
#39245=ORIENTED_EDGE('',*,*,#27984,.F.) ;
#39246=ORIENTED_EDGE('',*,*,#28012,.T.) ;
#39247=ORIENTED_EDGE('',*,*,#28013,.F.) ;
#39248=ORIENTED_EDGE('',*,*,#28011,.T.) ;
#39249=ORIENTED_EDGE('',*,*,#27629,.T.) ;
#39250=ORIENTED_EDGE('',*,*,#28014,.T.) ;
#39251=ORIENTED_EDGE('',*,*,#28015,.T.) ;
#39252=ORIENTED_EDGE('',*,*,#28016,.T.) ;
#39253=ORIENTED_EDGE('',*,*,#28017,.T.) ;
#39254=ORIENTED_EDGE('',*,*,#28018,.T.) ;
#39255=ORIENTED_EDGE('',*,*,#27630,.T.) ;
#39256=ORIENTED_EDGE('',*,*,#28016,.F.) ;
#39257=ORIENTED_EDGE('',*,*,#27631,.T.) ;
#39258=ORIENTED_EDGE('',*,*,#28018,.F.) ;
#39259=ORIENTED_EDGE('',*,*,#28019,.T.) ;
#39260=ORIENTED_EDGE('',*,*,#28020,.T.) ;
#39261=ORIENTED_EDGE('',*,*,#27632,.T.) ;
#39262=ORIENTED_EDGE('',*,*,#28020,.F.) ;
#39263=ORIENTED_EDGE('',*,*,#28021,.T.) ;
#39264=ORIENTED_EDGE('',*,*,#28014,.F.) ;
#39265=ORIENTED_EDGE('',*,*,#28017,.F.) ;
#39266=ORIENTED_EDGE('',*,*,#28022,.F.) ;
#39267=ORIENTED_EDGE('',*,*,#28023,.F.) ;
#39268=ORIENTED_EDGE('',*,*,#28024,.T.) ;
#39269=ORIENTED_EDGE('',*,*,#28015,.F.) ;
#39270=ORIENTED_EDGE('',*,*,#28025,.T.) ;
#39271=ORIENTED_EDGE('',*,*,#28026,.F.) ;
#39272=ORIENTED_EDGE('',*,*,#28022,.T.) ;
#39273=ORIENTED_EDGE('',*,*,#27530,.T.) ;
#39274=ORIENTED_EDGE('',*,*,#27552,.T.) ;
#39275=ORIENTED_EDGE('',*,*,#27549,.T.) ;
#39276=ORIENTED_EDGE('',*,*,#27546,.T.) ;
#39277=ORIENTED_EDGE('',*,*,#27543,.T.) ;
#39278=ORIENTED_EDGE('',*,*,#27540,.T.) ;
#39279=ORIENTED_EDGE('',*,*,#27537,.T.) ;
#39280=ORIENTED_EDGE('',*,*,#27534,.T.) ;
#39281=ORIENTED_EDGE('',*,*,#28027,.T.) ;
#39282=ORIENTED_EDGE('',*,*,#28028,.T.) ;
#39283=ORIENTED_EDGE('',*,*,#28029,.T.) ;
#39284=ORIENTED_EDGE('',*,*,#28030,.T.) ;
#39285=ORIENTED_EDGE('',*,*,#28031,.T.) ;
#39286=ORIENTED_EDGE('',*,*,#28027,.F.) ;
#39287=ORIENTED_EDGE('',*,*,#28032,.T.) ;
#39288=ORIENTED_EDGE('',*,*,#28033,.T.) ;
#39289=ORIENTED_EDGE('',*,*,#28034,.T.) ;
#39290=ORIENTED_EDGE('',*,*,#28030,.F.) ;
#39291=ORIENTED_EDGE('',*,*,#28035,.T.) ;
#39292=ORIENTED_EDGE('',*,*,#28035,.F.) ;
#39293=ORIENTED_EDGE('',*,*,#28036,.F.) ;
#39294=ORIENTED_EDGE('',*,*,#28037,.T.) ;
#39295=ORIENTED_EDGE('',*,*,#28038,.T.) ;
#39296=ORIENTED_EDGE('',*,*,#28039,.T.) ;
#39297=ORIENTED_EDGE('',*,*,#28040,.T.) ;
#39298=ORIENTED_EDGE('',*,*,#28032,.F.) ;
#39299=ORIENTED_EDGE('',*,*,#28029,.F.) ;
#39300=ORIENTED_EDGE('',*,*,#28041,.T.) ;
#39301=ORIENTED_EDGE('',*,*,#28042,.T.) ;
#39302=ORIENTED_EDGE('',*,*,#28036,.T.) ;
#39303=ORIENTED_EDGE('',*,*,#28028,.F.) ;
#39304=ORIENTED_EDGE('',*,*,#28043,.T.) ;
#39305=ORIENTED_EDGE('',*,*,#28044,.F.) ;
#39306=ORIENTED_EDGE('',*,*,#28045,.T.) ;
#39307=ORIENTED_EDGE('',*,*,#28046,.F.) ;
#39308=ORIENTED_EDGE('',*,*,#28047,.F.) ;
#39309=ORIENTED_EDGE('',*,*,#28048,.F.) ;
#39310=ORIENTED_EDGE('',*,*,#27780,.T.) ;
#39311=ORIENTED_EDGE('',*,*,#28049,.T.) ;
#39312=ORIENTED_EDGE('',*,*,#28047,.T.) ;
#39313=ORIENTED_EDGE('',*,*,#28050,.T.) ;
#39314=ORIENTED_EDGE('',*,*,#27912,.T.) ;
#39315=ORIENTED_EDGE('',*,*,#28051,.T.) ;
#39316=ORIENTED_EDGE('',*,*,#28048,.T.) ;
#39317=ORIENTED_EDGE('',*,*,#28052,.T.) ;
#39318=ORIENTED_EDGE('',*,*,#28053,.F.) ;
#39319=ORIENTED_EDGE('',*,*,#28054,.F.) ;
#39320=ORIENTED_EDGE('',*,*,#28055,.T.) ;
#39321=ORIENTED_EDGE('',*,*,#28056,.F.) ;
#39322=ORIENTED_EDGE('',*,*,#27914,.F.) ;
#39323=ORIENTED_EDGE('',*,*,#28057,.T.) ;
#39324=ORIENTED_EDGE('',*,*,#28054,.T.) ;
#39325=ORIENTED_EDGE('',*,*,#28058,.T.) ;
#39326=ORIENTED_EDGE('',*,*,#27782,.T.) ;
#39327=ORIENTED_EDGE('',*,*,#28059,.T.) ;
#39328=ORIENTED_EDGE('',*,*,#28056,.T.) ;
#39329=ORIENTED_EDGE('',*,*,#28060,.T.) ;
#39330=ORIENTED_EDGE('',*,*,#28046,.T.) ;
#39331=ORIENTED_EDGE('',*,*,#28061,.T.) ;
#39332=ORIENTED_EDGE('',*,*,#28053,.T.) ;
#39333=ORIENTED_EDGE('',*,*,#28062,.T.) ;
#39334=ORIENTED_EDGE('',*,*,#27908,.T.) ;
#39335=ORIENTED_EDGE('',*,*,#28052,.F.) ;
#39336=ORIENTED_EDGE('',*,*,#28049,.F.) ;
#39337=ORIENTED_EDGE('',*,*,#27779,.T.) ;
#39338=ORIENTED_EDGE('',*,*,#28063,.F.) ;
#39339=ORIENTED_EDGE('',*,*,#28064,.F.) ;
#39340=ORIENTED_EDGE('',*,*,#28065,.F.) ;
#39341=ORIENTED_EDGE('',*,*,#28066,.T.) ;
#39342=ORIENTED_EDGE('',*,*,#28067,.T.) ;
#39343=ORIENTED_EDGE('',*,*,#28068,.T.) ;
#39344=ORIENTED_EDGE('',*,*,#28069,.F.) ;
#39345=ORIENTED_EDGE('',*,*,#28070,.F.) ;
#39346=ORIENTED_EDGE('',*,*,#28071,.F.) ;
#39347=ORIENTED_EDGE('',*,*,#28072,.F.) ;
#39348=ORIENTED_EDGE('',*,*,#28073,.F.) ;
#39349=ORIENTED_EDGE('',*,*,#28074,.F.) ;
#39350=ORIENTED_EDGE('',*,*,#28075,.F.) ;
#39351=ORIENTED_EDGE('',*,*,#28076,.F.) ;
#39352=ORIENTED_EDGE('',*,*,#28077,.F.) ;
#39353=ORIENTED_EDGE('',*,*,#28078,.F.) ;
#39354=ORIENTED_EDGE('',*,*,#28079,.F.) ;
#39355=ORIENTED_EDGE('',*,*,#28080,.F.) ;
#39356=ORIENTED_EDGE('',*,*,#28081,.F.) ;
#39357=ORIENTED_EDGE('',*,*,#28082,.T.) ;
#39358=ORIENTED_EDGE('',*,*,#28083,.T.) ;
#39359=ORIENTED_EDGE('',*,*,#28084,.T.) ;
#39360=ORIENTED_EDGE('',*,*,#28085,.T.) ;
#39361=ORIENTED_EDGE('',*,*,#28086,.F.) ;
#39362=ORIENTED_EDGE('',*,*,#28087,.F.) ;
#39363=ORIENTED_EDGE('',*,*,#28088,.F.) ;
#39364=ORIENTED_EDGE('',*,*,#28089,.F.) ;
#39365=ORIENTED_EDGE('',*,*,#28090,.F.) ;
#39366=ORIENTED_EDGE('',*,*,#28091,.F.) ;
#39367=ORIENTED_EDGE('',*,*,#28092,.T.) ;
#39368=ORIENTED_EDGE('',*,*,#28093,.T.) ;
#39369=ORIENTED_EDGE('',*,*,#28094,.T.) ;
#39370=ORIENTED_EDGE('',*,*,#28095,.T.) ;
#39371=ORIENTED_EDGE('',*,*,#28096,.T.) ;
#39372=ORIENTED_EDGE('',*,*,#28097,.T.) ;
#39373=ORIENTED_EDGE('',*,*,#28098,.F.) ;
#39374=ORIENTED_EDGE('',*,*,#28099,.F.) ;
#39375=ORIENTED_EDGE('',*,*,#28100,.T.) ;
#39376=ORIENTED_EDGE('',*,*,#28101,.T.) ;
#39377=ORIENTED_EDGE('',*,*,#28102,.T.) ;
#39378=ORIENTED_EDGE('',*,*,#28103,.T.) ;
#39379=ORIENTED_EDGE('',*,*,#28104,.T.) ;
#39380=ORIENTED_EDGE('',*,*,#28105,.T.) ;
#39381=ORIENTED_EDGE('',*,*,#28106,.F.) ;
#39382=ORIENTED_EDGE('',*,*,#28107,.T.) ;
#39383=ORIENTED_EDGE('',*,*,#28108,.T.) ;
#39384=ORIENTED_EDGE('',*,*,#28109,.T.) ;
#39385=ORIENTED_EDGE('',*,*,#28110,.T.) ;
#39386=ORIENTED_EDGE('',*,*,#28111,.T.) ;
#39387=ORIENTED_EDGE('',*,*,#28112,.T.) ;
#39388=ORIENTED_EDGE('',*,*,#28113,.T.) ;
#39389=ORIENTED_EDGE('',*,*,#28114,.T.) ;
#39390=ORIENTED_EDGE('',*,*,#28115,.T.) ;
#39391=ORIENTED_EDGE('',*,*,#28116,.T.) ;
#39392=ORIENTED_EDGE('',*,*,#28117,.T.) ;
#39393=ORIENTED_EDGE('',*,*,#28118,.F.) ;
#39394=ORIENTED_EDGE('',*,*,#28119,.T.) ;
#39395=ORIENTED_EDGE('',*,*,#28120,.T.) ;
#39396=ORIENTED_EDGE('',*,*,#28121,.T.) ;
#39397=ORIENTED_EDGE('',*,*,#28039,.F.) ;
#39398=ORIENTED_EDGE('',*,*,#28122,.T.) ;
#39399=ORIENTED_EDGE('',*,*,#28123,.F.) ;
#39400=ORIENTED_EDGE('',*,*,#28124,.F.) ;
#39401=ORIENTED_EDGE('',*,*,#28125,.F.) ;
#39402=ORIENTED_EDGE('',*,*,#28126,.F.) ;
#39403=ORIENTED_EDGE('',*,*,#28127,.F.) ;
#39404=ORIENTED_EDGE('',*,*,#28128,.T.) ;
#39405=ORIENTED_EDGE('',*,*,#28129,.F.) ;
#39406=ORIENTED_EDGE('',*,*,#28130,.T.) ;
#39407=ORIENTED_EDGE('',*,*,#28131,.F.) ;
#39408=ORIENTED_EDGE('',*,*,#28132,.F.) ;
#39409=ORIENTED_EDGE('',*,*,#28133,.T.) ;
#39410=ORIENTED_EDGE('',*,*,#28134,.F.) ;
#39411=ORIENTED_EDGE('',*,*,#28135,.T.) ;
#39412=ORIENTED_EDGE('',*,*,#28136,.F.) ;
#39413=ORIENTED_EDGE('',*,*,#28137,.F.) ;
#39414=ORIENTED_EDGE('',*,*,#28138,.T.) ;
#39415=ORIENTED_EDGE('',*,*,#28139,.F.) ;
#39416=ORIENTED_EDGE('',*,*,#28140,.T.) ;
#39417=ORIENTED_EDGE('',*,*,#28141,.T.) ;
#39418=ORIENTED_EDGE('',*,*,#28142,.T.) ;
#39419=ORIENTED_EDGE('',*,*,#28143,.F.) ;
#39420=ORIENTED_EDGE('',*,*,#28144,.F.) ;
#39421=ORIENTED_EDGE('',*,*,#28145,.F.) ;
#39422=ORIENTED_EDGE('',*,*,#28146,.F.) ;
#39423=ORIENTED_EDGE('',*,*,#28147,.F.) ;
#39424=ORIENTED_EDGE('',*,*,#28148,.F.) ;
#39425=ORIENTED_EDGE('',*,*,#28149,.F.) ;
#39426=ORIENTED_EDGE('',*,*,#28150,.F.) ;
#39427=ORIENTED_EDGE('',*,*,#28151,.F.) ;
#39428=ORIENTED_EDGE('',*,*,#28152,.T.) ;
#39429=ORIENTED_EDGE('',*,*,#27906,.T.) ;
#39430=ORIENTED_EDGE('',*,*,#27891,.F.) ;
#39431=ORIENTED_EDGE('',*,*,#27921,.F.) ;
#39432=ORIENTED_EDGE('',*,*,#28153,.F.) ;
#39433=ORIENTED_EDGE('',*,*,#28154,.F.) ;
#39434=ORIENTED_EDGE('',*,*,#28155,.F.) ;
#39435=ORIENTED_EDGE('',*,*,#28156,.F.) ;
#39436=ORIENTED_EDGE('',*,*,#28157,.F.) ;
#39437=ORIENTED_EDGE('',*,*,#28158,.F.) ;
#39438=ORIENTED_EDGE('',*,*,#28159,.F.) ;
#39439=ORIENTED_EDGE('',*,*,#28160,.F.) ;
#39440=ORIENTED_EDGE('',*,*,#28161,.F.) ;
#39441=ORIENTED_EDGE('',*,*,#28162,.T.) ;
#39442=ORIENTED_EDGE('',*,*,#28163,.T.) ;
#39443=ORIENTED_EDGE('',*,*,#28164,.T.) ;
#39444=ORIENTED_EDGE('',*,*,#27916,.T.) ;
#39445=ORIENTED_EDGE('',*,*,#28165,.F.) ;
#39446=ORIENTED_EDGE('',*,*,#28166,.F.) ;
#39447=ORIENTED_EDGE('',*,*,#28167,.F.) ;
#39448=ORIENTED_EDGE('',*,*,#28168,.F.) ;
#39449=ORIENTED_EDGE('',*,*,#28169,.F.) ;
#39450=ORIENTED_EDGE('',*,*,#28170,.F.) ;
#39451=ORIENTED_EDGE('',*,*,#28171,.F.) ;
#39452=ORIENTED_EDGE('',*,*,#28172,.F.) ;
#39453=ORIENTED_EDGE('',*,*,#28173,.F.) ;
#39454=ORIENTED_EDGE('',*,*,#28174,.F.) ;
#39455=ORIENTED_EDGE('',*,*,#28175,.F.) ;
#39456=ORIENTED_EDGE('',*,*,#28176,.F.) ;
#39457=ORIENTED_EDGE('',*,*,#28177,.F.) ;
#39458=ORIENTED_EDGE('',*,*,#28178,.F.) ;
#39459=ORIENTED_EDGE('',*,*,#28179,.F.) ;
#39460=ORIENTED_EDGE('',*,*,#28180,.F.) ;
#39461=ORIENTED_EDGE('',*,*,#28181,.F.) ;
#39462=ORIENTED_EDGE('',*,*,#28182,.F.) ;
#39463=ORIENTED_EDGE('',*,*,#28183,.F.) ;
#39464=ORIENTED_EDGE('',*,*,#28184,.F.) ;
#39465=ORIENTED_EDGE('',*,*,#28185,.F.) ;
#39466=ORIENTED_EDGE('',*,*,#28186,.F.) ;
#39467=ORIENTED_EDGE('',*,*,#28187,.F.) ;
#39468=ORIENTED_EDGE('',*,*,#28188,.F.) ;
#39469=ORIENTED_EDGE('',*,*,#28189,.F.) ;
#39470=ORIENTED_EDGE('',*,*,#28190,.F.) ;
#39471=ORIENTED_EDGE('',*,*,#28191,.F.) ;
#39472=ORIENTED_EDGE('',*,*,#28192,.F.) ;
#39473=ORIENTED_EDGE('',*,*,#28193,.F.) ;
#39474=ORIENTED_EDGE('',*,*,#28194,.F.) ;
#39475=ORIENTED_EDGE('',*,*,#28195,.F.) ;
#39476=ORIENTED_EDGE('',*,*,#28196,.F.) ;
#39477=ORIENTED_EDGE('',*,*,#28197,.F.) ;
#39478=ORIENTED_EDGE('',*,*,#28198,.F.) ;
#39479=ORIENTED_EDGE('',*,*,#28199,.F.) ;
#39480=ORIENTED_EDGE('',*,*,#28200,.F.) ;
#39481=ORIENTED_EDGE('',*,*,#28201,.F.) ;
#39482=ORIENTED_EDGE('',*,*,#28202,.F.) ;
#39483=ORIENTED_EDGE('',*,*,#27637,.F.) ;
#39484=ORIENTED_EDGE('',*,*,#27635,.F.) ;
#39485=ORIENTED_EDGE('',*,*,#28203,.F.) ;
#39486=ORIENTED_EDGE('',*,*,#28204,.F.) ;
#39487=ORIENTED_EDGE('',*,*,#28205,.F.) ;
#39488=ORIENTED_EDGE('',*,*,#28206,.F.) ;
#39489=ORIENTED_EDGE('',*,*,#28207,.F.) ;
#39490=ORIENTED_EDGE('',*,*,#28208,.F.) ;
#39491=ORIENTED_EDGE('',*,*,#28209,.F.) ;
#39492=ORIENTED_EDGE('',*,*,#28210,.F.) ;
#39493=ORIENTED_EDGE('',*,*,#28211,.F.) ;
#39494=ORIENTED_EDGE('',*,*,#28212,.F.) ;
#39495=ORIENTED_EDGE('',*,*,#28213,.F.) ;
#39496=ORIENTED_EDGE('',*,*,#28214,.F.) ;
#39497=ORIENTED_EDGE('',*,*,#28215,.F.) ;
#39498=ORIENTED_EDGE('',*,*,#28216,.F.) ;
#39499=ORIENTED_EDGE('',*,*,#28217,.F.) ;
#39500=ORIENTED_EDGE('',*,*,#28218,.F.) ;
#39501=ORIENTED_EDGE('',*,*,#28219,.F.) ;
#39502=ORIENTED_EDGE('',*,*,#28220,.F.) ;
#39503=ORIENTED_EDGE('',*,*,#28221,.F.) ;
#39504=ORIENTED_EDGE('',*,*,#28222,.F.) ;
#39505=ORIENTED_EDGE('',*,*,#28223,.F.) ;
#39506=ORIENTED_EDGE('',*,*,#28224,.F.) ;
#39507=ORIENTED_EDGE('',*,*,#28225,.F.) ;
#39508=ORIENTED_EDGE('',*,*,#28226,.F.) ;
#39509=ORIENTED_EDGE('',*,*,#28227,.F.) ;
#39510=ORIENTED_EDGE('',*,*,#28050,.F.) ;
#39511=ORIENTED_EDGE('',*,*,#28062,.F.) ;
#39512=ORIENTED_EDGE('',*,*,#28059,.F.) ;
#39513=ORIENTED_EDGE('',*,*,#27781,.T.) ;
#39514=ORIENTED_EDGE('',*,*,#28228,.T.) ;
#39515=ORIENTED_EDGE('',*,*,#28229,.F.) ;
#39516=ORIENTED_EDGE('',*,*,#28230,.F.) ;
#39517=ORIENTED_EDGE('',*,*,#28231,.F.) ;
#39518=ORIENTED_EDGE('',*,*,#27867,.F.) ;
#39519=ORIENTED_EDGE('',*,*,#27903,.T.) ;
#39520=ORIENTED_EDGE('',*,*,#28232,.T.) ;
#39521=ORIENTED_EDGE('',*,*,#28229,.T.) ;
#39522=ORIENTED_EDGE('',*,*,#28233,.T.) ;
#39523=ORIENTED_EDGE('',*,*,#28234,.T.) ;
#39524=ORIENTED_EDGE('',*,*,#28126,.T.) ;
#39525=ORIENTED_EDGE('',*,*,#28230,.T.) ;
#39526=ORIENTED_EDGE('',*,*,#28235,.T.) ;
#39527=ORIENTED_EDGE('',*,*,#28236,.T.) ;
#39528=ORIENTED_EDGE('',*,*,#28237,.T.) ;
#39529=ORIENTED_EDGE('',*,*,#28231,.T.) ;
#39530=ORIENTED_EDGE('',*,*,#28125,.T.) ;
#39531=ORIENTED_EDGE('',*,*,#28238,.T.) ;
#39532=ORIENTED_EDGE('',*,*,#28239,.T.) ;
#39533=ORIENTED_EDGE('',*,*,#28236,.F.) ;
#39534=ORIENTED_EDGE('',*,*,#28124,.T.) ;
#39535=ORIENTED_EDGE('',*,*,#28235,.F.) ;
#39536=ORIENTED_EDGE('',*,*,#28232,.F.) ;
#39537=ORIENTED_EDGE('',*,*,#27902,.F.) ;
#39538=ORIENTED_EDGE('',*,*,#28240,.F.) ;
#39539=ORIENTED_EDGE('',*,*,#27868,.F.) ;
#39540=ORIENTED_EDGE('',*,*,#28233,.F.) ;
#39541=ORIENTED_EDGE('',*,*,#28228,.F.) ;
#39542=ORIENTED_EDGE('',*,*,#28237,.F.) ;
#39543=ORIENTED_EDGE('',*,*,#28241,.T.) ;
#39544=ORIENTED_EDGE('',*,*,#28242,.F.) ;
#39545=ORIENTED_EDGE('',*,*,#28243,.F.) ;
#39546=ORIENTED_EDGE('',*,*,#28239,.F.) ;
#39547=ORIENTED_EDGE('',*,*,#28244,.F.) ;
#39548=ORIENTED_EDGE('',*,*,#28245,.T.) ;
#39549=ORIENTED_EDGE('',*,*,#28041,.F.) ;
#39550=ORIENTED_EDGE('',*,*,#28045,.F.) ;
#39551=ORIENTED_EDGE('',*,*,#28246,.T.) ;
#39552=ORIENTED_EDGE('',*,*,#28247,.F.) ;
#39553=ORIENTED_EDGE('',*,*,#28241,.F.) ;
#39554=ORIENTED_EDGE('',*,*,#27905,.F.) ;
#39555=ORIENTED_EDGE('',*,*,#28248,.T.) ;
#39556=ORIENTED_EDGE('',*,*,#28151,.T.) ;
#39557=ORIENTED_EDGE('',*,*,#28249,.T.) ;
#39558=ORIENTED_EDGE('',*,*,#28250,.T.) ;
#39559=ORIENTED_EDGE('',*,*,#28251,.F.) ;
#39560=ORIENTED_EDGE('',*,*,#28252,.F.) ;
#39561=ORIENTED_EDGE('',*,*,#28253,.F.) ;
#39562=ORIENTED_EDGE('',*,*,#28254,.F.) ;
#39563=ORIENTED_EDGE('',*,*,#27767,.F.) ;
#39564=ORIENTED_EDGE('',*,*,#28255,.T.) ;
#39565=ORIENTED_EDGE('',*,*,#28256,.T.) ;
#39566=ORIENTED_EDGE('',*,*,#28257,.T.) ;
#39567=ORIENTED_EDGE('',*,*,#28258,.T.) ;
#39568=ORIENTED_EDGE('',*,*,#28259,.T.) ;
#39569=ORIENTED_EDGE('',*,*,#28256,.F.) ;
#39570=ORIENTED_EDGE('',*,*,#28260,.T.) ;
#39571=ORIENTED_EDGE('',*,*,#28261,.T.) ;
#39572=ORIENTED_EDGE('',*,*,#28262,.T.) ;
#39573=ORIENTED_EDGE('',*,*,#28258,.F.) ;
#39574=ORIENTED_EDGE('',*,*,#28263,.T.) ;
#39575=ORIENTED_EDGE('',*,*,#28264,.T.) ;
#39576=ORIENTED_EDGE('',*,*,#28265,.T.) ;
#39577=ORIENTED_EDGE('',*,*,#28261,.F.) ;
#39578=ORIENTED_EDGE('',*,*,#28266,.T.) ;
#39579=ORIENTED_EDGE('',*,*,#28253,.T.) ;
#39580=ORIENTED_EDGE('',*,*,#28267,.T.) ;
#39581=ORIENTED_EDGE('',*,*,#28264,.F.) ;
#39582=ORIENTED_EDGE('',*,*,#28268,.T.) ;
#39583=ORIENTED_EDGE('',*,*,#28269,.T.) ;
#39584=ORIENTED_EDGE('',*,*,#28270,.T.) ;
#39585=ORIENTED_EDGE('',*,*,#28271,.T.) ;
#39586=ORIENTED_EDGE('',*,*,#28272,.T.) ;
#39587=ORIENTED_EDGE('',*,*,#28273,.T.) ;
#39588=ORIENTED_EDGE('',*,*,#28274,.T.) ;
#39589=ORIENTED_EDGE('',*,*,#28271,.F.) ;
#39590=ORIENTED_EDGE('',*,*,#28275,.T.) ;
#39591=ORIENTED_EDGE('',*,*,#28254,.T.) ;
#39592=ORIENTED_EDGE('',*,*,#28276,.T.) ;
#39593=ORIENTED_EDGE('',*,*,#28273,.F.) ;
#39594=ORIENTED_EDGE('',*,*,#28277,.T.) ;
#39595=ORIENTED_EDGE('',*,*,#28278,.F.) ;
#39596=ORIENTED_EDGE('',*,*,#28279,.F.) ;
#39597=ORIENTED_EDGE('',*,*,#28280,.T.) ;
#39598=ORIENTED_EDGE('',*,*,#28281,.F.) ;
#39599=ORIENTED_EDGE('',*,*,#27923,.F.) ;
#39600=ORIENTED_EDGE('',*,*,#28282,.T.) ;
#39601=ORIENTED_EDGE('',*,*,#28283,.T.) ;
#39602=ORIENTED_EDGE('',*,*,#28153,.T.) ;
#39603=ORIENTED_EDGE('',*,*,#27924,.F.) ;
#39604=ORIENTED_EDGE('',*,*,#28284,.T.) ;
#39605=ORIENTED_EDGE('',*,*,#28154,.T.) ;
#39606=ORIENTED_EDGE('',*,*,#28283,.F.) ;
#39607=ORIENTED_EDGE('',*,*,#28285,.T.) ;
#39608=ORIENTED_EDGE('',*,*,#28286,.T.) ;
#39609=ORIENTED_EDGE('',*,*,#28155,.T.) ;
#39610=ORIENTED_EDGE('',*,*,#28284,.F.) ;
#39611=ORIENTED_EDGE('',*,*,#28287,.T.) ;
#39612=ORIENTED_EDGE('',*,*,#28288,.T.) ;
#39613=ORIENTED_EDGE('',*,*,#28156,.T.) ;
#39614=ORIENTED_EDGE('',*,*,#28286,.F.) ;
#39615=ORIENTED_EDGE('',*,*,#28289,.T.) ;
#39616=ORIENTED_EDGE('',*,*,#28288,.F.) ;
#39617=ORIENTED_EDGE('',*,*,#28290,.T.) ;
#39618=ORIENTED_EDGE('',*,*,#28279,.T.) ;
#39619=ORIENTED_EDGE('',*,*,#28157,.T.) ;
#39620=ORIENTED_EDGE('',*,*,#28281,.T.) ;
#39621=ORIENTED_EDGE('',*,*,#28291,.T.) ;
#39622=ORIENTED_EDGE('',*,*,#28252,.T.) ;
#39623=ORIENTED_EDGE('',*,*,#28292,.T.) ;
#39624=ORIENTED_EDGE('',*,*,#28293,.T.) ;
#39625=ORIENTED_EDGE('',*,*,#28158,.T.) ;
#39626=ORIENTED_EDGE('',*,*,#28278,.T.) ;
#39627=ORIENTED_EDGE('',*,*,#28294,.T.) ;
#39628=ORIENTED_EDGE('',*,*,#28295,.T.) ;
#39629=ORIENTED_EDGE('',*,*,#28159,.T.) ;
#39630=ORIENTED_EDGE('',*,*,#28293,.F.) ;
#39631=ORIENTED_EDGE('',*,*,#28296,.T.) ;
#39632=ORIENTED_EDGE('',*,*,#28297,.T.) ;
#39633=ORIENTED_EDGE('',*,*,#28160,.T.) ;
#39634=ORIENTED_EDGE('',*,*,#28295,.F.) ;
#39635=ORIENTED_EDGE('',*,*,#28298,.T.) ;
#39636=ORIENTED_EDGE('',*,*,#28299,.F.) ;
#39637=ORIENTED_EDGE('',*,*,#28161,.T.) ;
#39638=ORIENTED_EDGE('',*,*,#28297,.F.) ;
#39639=ORIENTED_EDGE('',*,*,#28300,.F.) ;
#39640=ORIENTED_EDGE('',*,*,#27770,.F.) ;
#39641=ORIENTED_EDGE('',*,*,#27783,.T.) ;
#39642=ORIENTED_EDGE('',*,*,#28060,.F.) ;
#39643=ORIENTED_EDGE('',*,*,#28055,.F.) ;
#39644=ORIENTED_EDGE('',*,*,#28057,.F.) ;
#39645=ORIENTED_EDGE('',*,*,#27913,.F.) ;
#39646=ORIENTED_EDGE('',*,*,#27918,.F.) ;
#39647=ORIENTED_EDGE('',*,*,#28301,.T.) ;
#39648=ORIENTED_EDGE('',*,*,#28302,.T.) ;
#39649=ORIENTED_EDGE('',*,*,#28303,.T.) ;
#39650=ORIENTED_EDGE('',*,*,#28272,.F.) ;
#39651=ORIENTED_EDGE('',*,*,#28274,.F.) ;
#39652=ORIENTED_EDGE('',*,*,#28276,.F.) ;
#39653=ORIENTED_EDGE('',*,*,#28268,.F.) ;
#39654=ORIENTED_EDGE('',*,*,#28266,.F.) ;
#39655=ORIENTED_EDGE('',*,*,#28263,.F.) ;
#39656=ORIENTED_EDGE('',*,*,#28260,.F.) ;
#39657=ORIENTED_EDGE('',*,*,#28255,.F.) ;
#39658=ORIENTED_EDGE('',*,*,#27771,.F.) ;
#39659=ORIENTED_EDGE('',*,*,#28257,.F.) ;
#39660=ORIENTED_EDGE('',*,*,#28304,.T.) ;
#39661=ORIENTED_EDGE('',*,*,#28305,.F.) ;
#39662=ORIENTED_EDGE('',*,*,#28306,.F.) ;
#39663=ORIENTED_EDGE('',*,*,#28307,.F.) ;
#39664=ORIENTED_EDGE('',*,*,#28259,.F.) ;
#39665=ORIENTED_EDGE('',*,*,#28308,.T.) ;
#39666=ORIENTED_EDGE('',*,*,#28309,.F.) ;
#39667=ORIENTED_EDGE('',*,*,#28304,.F.) ;
#39668=ORIENTED_EDGE('',*,*,#28262,.F.) ;
#39669=ORIENTED_EDGE('',*,*,#28310,.F.) ;
#39670=ORIENTED_EDGE('',*,*,#28311,.F.) ;
#39671=ORIENTED_EDGE('',*,*,#28308,.F.) ;
#39672=ORIENTED_EDGE('',*,*,#28265,.F.) ;
#39673=ORIENTED_EDGE('',*,*,#28312,.T.) ;
#39674=ORIENTED_EDGE('',*,*,#28313,.F.) ;
#39675=ORIENTED_EDGE('',*,*,#28310,.T.) ;
#39676=ORIENTED_EDGE('',*,*,#28267,.F.) ;
#39677=ORIENTED_EDGE('',*,*,#28291,.F.) ;
#39678=ORIENTED_EDGE('',*,*,#28280,.F.) ;
#39679=ORIENTED_EDGE('',*,*,#28290,.F.) ;
#39680=ORIENTED_EDGE('',*,*,#28314,.T.) ;
#39681=ORIENTED_EDGE('',*,*,#28315,.F.) ;
#39682=ORIENTED_EDGE('',*,*,#28316,.F.) ;
#39683=ORIENTED_EDGE('',*,*,#28317,.F.) ;
#39684=ORIENTED_EDGE('',*,*,#28318,.F.) ;
#39685=ORIENTED_EDGE('',*,*,#28319,.F.) ;
#39686=ORIENTED_EDGE('',*,*,#28320,.F.) ;
#39687=ORIENTED_EDGE('',*,*,#28321,.F.) ;
#39688=ORIENTED_EDGE('',*,*,#28312,.F.) ;
#39689=ORIENTED_EDGE('',*,*,#28289,.F.) ;
#39690=ORIENTED_EDGE('',*,*,#28322,.T.) ;
#39691=ORIENTED_EDGE('',*,*,#28323,.F.) ;
#39692=ORIENTED_EDGE('',*,*,#28314,.F.) ;
#39693=ORIENTED_EDGE('',*,*,#28287,.F.) ;
#39694=ORIENTED_EDGE('',*,*,#28324,.T.) ;
#39695=ORIENTED_EDGE('',*,*,#28325,.F.) ;
#39696=ORIENTED_EDGE('',*,*,#28322,.F.) ;
#39697=ORIENTED_EDGE('',*,*,#28285,.F.) ;
#39698=ORIENTED_EDGE('',*,*,#28326,.F.) ;
#39699=ORIENTED_EDGE('',*,*,#28327,.F.) ;
#39700=ORIENTED_EDGE('',*,*,#28324,.F.) ;
#39701=ORIENTED_EDGE('',*,*,#28282,.F.) ;
#39702=ORIENTED_EDGE('',*,*,#27927,.T.) ;
#39703=ORIENTED_EDGE('',*,*,#28328,.F.) ;
#39704=ORIENTED_EDGE('',*,*,#28329,.F.) ;
#39705=ORIENTED_EDGE('',*,*,#28330,.F.) ;
#39706=ORIENTED_EDGE('',*,*,#28326,.T.) ;
#39707=ORIENTED_EDGE('',*,*,#28331,.F.) ;
#39708=ORIENTED_EDGE('',*,*,#28332,.F.) ;
#39709=ORIENTED_EDGE('',*,*,#28333,.F.) ;
#39710=ORIENTED_EDGE('',*,*,#28334,.T.) ;
#39711=ORIENTED_EDGE('',*,*,#28335,.F.) ;
#39712=ORIENTED_EDGE('',*,*,#28336,.T.) ;
#39713=ORIENTED_EDGE('',*,*,#28332,.T.) ;
#39714=ORIENTED_EDGE('',*,*,#28337,.T.) ;
#39715=ORIENTED_EDGE('',*,*,#28338,.F.) ;
#39716=ORIENTED_EDGE('',*,*,#28339,.F.) ;
#39717=ORIENTED_EDGE('',*,*,#28340,.T.) ;
#39718=ORIENTED_EDGE('',*,*,#28341,.F.) ;
#39719=ORIENTED_EDGE('',*,*,#28342,.T.) ;
#39720=ORIENTED_EDGE('',*,*,#28343,.T.) ;
#39721=ORIENTED_EDGE('',*,*,#28339,.T.) ;
#39722=ORIENTED_EDGE('',*,*,#28344,.T.) ;
#39723=ORIENTED_EDGE('',*,*,#28342,.F.) ;
#39724=ORIENTED_EDGE('',*,*,#28345,.T.) ;
#39725=ORIENTED_EDGE('',*,*,#28331,.T.) ;
#39726=ORIENTED_EDGE('',*,*,#28346,.T.) ;
#39727=ORIENTED_EDGE('',*,*,#28347,.T.) ;
#39728=ORIENTED_EDGE('',*,*,#28348,.F.) ;
#39729=ORIENTED_EDGE('',*,*,#28349,.F.) ;
#39730=ORIENTED_EDGE('',*,*,#28350,.F.) ;
#39731=ORIENTED_EDGE('',*,*,#28351,.F.) ;
#39732=ORIENTED_EDGE('',*,*,#28352,.F.) ;
#39733=ORIENTED_EDGE('',*,*,#28353,.T.) ;
#39734=ORIENTED_EDGE('',*,*,#28354,.F.) ;
#39735=ORIENTED_EDGE('',*,*,#28355,.T.) ;
#39736=ORIENTED_EDGE('',*,*,#28356,.T.) ;
#39737=ORIENTED_EDGE('',*,*,#28352,.T.) ;
#39738=ORIENTED_EDGE('',*,*,#28357,.T.) ;
#39739=ORIENTED_EDGE('',*,*,#28348,.T.) ;
#39740=ORIENTED_EDGE('',*,*,#28358,.T.) ;
#39741=ORIENTED_EDGE('',*,*,#28355,.F.) ;
#39742=ORIENTED_EDGE('',*,*,#28359,.T.) ;
#39743=ORIENTED_EDGE('',*,*,#28360,.T.) ;
#39744=ORIENTED_EDGE('',*,*,#28361,.T.) ;
#39745=ORIENTED_EDGE('',*,*,#28354,.T.) ;
#39746=ORIENTED_EDGE('',*,*,#28362,.T.) ;
#39747=ORIENTED_EDGE('',*,*,#28363,.T.) ;
#39748=ORIENTED_EDGE('',*,*,#28364,.T.) ;
#39749=ORIENTED_EDGE('',*,*,#28360,.F.) ;
#39750=ORIENTED_EDGE('',*,*,#28365,.T.) ;
#39751=ORIENTED_EDGE('',*,*,#28366,.T.) ;
#39752=ORIENTED_EDGE('',*,*,#28367,.T.) ;
#39753=ORIENTED_EDGE('',*,*,#28363,.F.) ;
#39754=ORIENTED_EDGE('',*,*,#27708,.T.) ;
#39755=ORIENTED_EDGE('',*,*,#27825,.F.) ;
#39756=ORIENTED_EDGE('',*,*,#28368,.T.) ;
#39757=ORIENTED_EDGE('',*,*,#28366,.F.) ;
#39758=ORIENTED_EDGE('',*,*,#27707,.T.) ;
#39759=ORIENTED_EDGE('',*,*,#28369,.F.) ;
#39760=ORIENTED_EDGE('',*,*,#28370,.T.) ;
#39761=ORIENTED_EDGE('',*,*,#28351,.T.) ;
#39762=ORIENTED_EDGE('',*,*,#28371,.T.) ;
#39763=ORIENTED_EDGE('',*,*,#28372,.T.) ;
#39764=ORIENTED_EDGE('',*,*,#28373,.T.) ;
#39765=ORIENTED_EDGE('',*,*,#27827,.F.) ;
#39766=ORIENTED_EDGE('',*,*,#27752,.T.) ;
#39767=ORIENTED_EDGE('',*,*,#28374,.T.) ;
#39768=ORIENTED_EDGE('',*,*,#28375,.T.) ;
#39769=ORIENTED_EDGE('',*,*,#28372,.F.) ;
#39770=ORIENTED_EDGE('',*,*,#27751,.T.) ;
#39771=ORIENTED_EDGE('',*,*,#28376,.T.) ;
#39772=ORIENTED_EDGE('',*,*,#28377,.T.) ;
#39773=ORIENTED_EDGE('',*,*,#28374,.F.) ;
#39774=ORIENTED_EDGE('',*,*,#27750,.T.) ;
#39775=ORIENTED_EDGE('',*,*,#27811,.F.) ;
#39776=ORIENTED_EDGE('',*,*,#28378,.T.) ;
#39777=ORIENTED_EDGE('',*,*,#28376,.F.) ;
#39778=ORIENTED_EDGE('',*,*,#27749,.T.) ;
#39779=ORIENTED_EDGE('',*,*,#28379,.F.) ;
#39780=ORIENTED_EDGE('',*,*,#28380,.T.) ;
#39781=ORIENTED_EDGE('',*,*,#28349,.T.) ;
#39782=ORIENTED_EDGE('',*,*,#28381,.T.) ;
#39783=ORIENTED_EDGE('',*,*,#28382,.T.) ;
#39784=ORIENTED_EDGE('',*,*,#28383,.T.) ;
#39785=ORIENTED_EDGE('',*,*,#28350,.T.) ;
#39786=ORIENTED_EDGE('',*,*,#28384,.T.) ;
#39787=ORIENTED_EDGE('',*,*,#28385,.T.) ;
#39788=ORIENTED_EDGE('',*,*,#28386,.T.) ;
#39789=ORIENTED_EDGE('',*,*,#28382,.F.) ;
#39790=ORIENTED_EDGE('',*,*,#28387,.T.) ;
#39791=ORIENTED_EDGE('',*,*,#28388,.T.) ;
#39792=ORIENTED_EDGE('',*,*,#28389,.T.) ;
#39793=ORIENTED_EDGE('',*,*,#28385,.F.) ;
#39794=ORIENTED_EDGE('',*,*,#28390,.T.) ;
#39795=ORIENTED_EDGE('',*,*,#28391,.T.) ;
#39796=ORIENTED_EDGE('',*,*,#28392,.T.) ;
#39797=ORIENTED_EDGE('',*,*,#28388,.F.) ;
#39798=ORIENTED_EDGE('',*,*,#28393,.T.) ;
#39799=ORIENTED_EDGE('',*,*,#28394,.T.) ;
#39800=ORIENTED_EDGE('',*,*,#28395,.T.) ;
#39801=ORIENTED_EDGE('',*,*,#28391,.F.) ;
#39802=ORIENTED_EDGE('',*,*,#28396,.T.) ;
#39803=ORIENTED_EDGE('',*,*,#28397,.T.) ;
#39804=ORIENTED_EDGE('',*,*,#28398,.T.) ;
#39805=ORIENTED_EDGE('',*,*,#28394,.F.) ;
#39806=ORIENTED_EDGE('',*,*,#28399,.T.) ;
#39807=ORIENTED_EDGE('',*,*,#28400,.T.) ;
#39808=ORIENTED_EDGE('',*,*,#28401,.T.) ;
#39809=ORIENTED_EDGE('',*,*,#28397,.F.) ;
#39810=ORIENTED_EDGE('',*,*,#28402,.T.) ;
#39811=ORIENTED_EDGE('',*,*,#28403,.T.) ;
#39812=ORIENTED_EDGE('',*,*,#28404,.T.) ;
#39813=ORIENTED_EDGE('',*,*,#28400,.F.) ;
#39814=ORIENTED_EDGE('',*,*,#28405,.T.) ;
#39815=ORIENTED_EDGE('',*,*,#28341,.T.) ;
#39816=ORIENTED_EDGE('',*,*,#28406,.T.) ;
#39817=ORIENTED_EDGE('',*,*,#28403,.F.) ;
#39818=ORIENTED_EDGE('',*,*,#28407,.T.) ;
#39819=ORIENTED_EDGE('',*,*,#28408,.T.) ;
#39820=ORIENTED_EDGE('',*,*,#28409,.T.) ;
#39821=ORIENTED_EDGE('',*,*,#28333,.T.) ;
#39822=ORIENTED_EDGE('',*,*,#28410,.T.) ;
#39823=ORIENTED_EDGE('',*,*,#28408,.F.) ;
#39824=ORIENTED_EDGE('',*,*,#28411,.T.) ;
#39825=ORIENTED_EDGE('',*,*,#28412,.T.) ;
#39826=ORIENTED_EDGE('',*,*,#28413,.T.) ;
#39827=ORIENTED_EDGE('',*,*,#27817,.T.) ;
#39828=ORIENTED_EDGE('',*,*,#27822,.T.) ;
#39829=ORIENTED_EDGE('',*,*,#28412,.F.) ;
#39830=ORIENTED_EDGE('',*,*,#28414,.T.) ;
#39831=ORIENTED_EDGE('',*,*,#28415,.F.) ;
#39832=ORIENTED_EDGE('',*,*,#28416,.T.) ;
#39833=ORIENTED_EDGE('',*,*,#28338,.T.) ;
#39834=ORIENTED_EDGE('',*,*,#28417,.T.) ;
#39835=ORIENTED_EDGE('',*,*,#28346,.F.) ;
#39836=ORIENTED_EDGE('',*,*,#28334,.F.) ;
#39837=ORIENTED_EDGE('',*,*,#28409,.F.) ;
#39838=ORIENTED_EDGE('',*,*,#28413,.F.) ;
#39839=ORIENTED_EDGE('',*,*,#27821,.T.) ;
#39840=ORIENTED_EDGE('',*,*,#28418,.F.) ;
#39841=ORIENTED_EDGE('',*,*,#28419,.T.) ;
#39842=ORIENTED_EDGE('',*,*,#28365,.F.) ;
#39843=ORIENTED_EDGE('',*,*,#28362,.F.) ;
#39844=ORIENTED_EDGE('',*,*,#28353,.F.) ;
#39845=ORIENTED_EDGE('',*,*,#28356,.F.) ;
#39846=ORIENTED_EDGE('',*,*,#28420,.T.) ;
#39847=ORIENTED_EDGE('',*,*,#28421,.T.) ;
#39848=ORIENTED_EDGE('',*,*,#27709,.T.) ;
#39849=ORIENTED_EDGE('',*,*,#28364,.F.) ;
#39850=ORIENTED_EDGE('',*,*,#28367,.F.) ;
#39851=ORIENTED_EDGE('',*,*,#28422,.T.) ;
#39852=ORIENTED_EDGE('',*,*,#28423,.T.) ;
#39853=ORIENTED_EDGE('',*,*,#28424,.T.) ;
#39854=ORIENTED_EDGE('',*,*,#28373,.F.) ;
#39855=ORIENTED_EDGE('',*,*,#28425,.F.) ;
#39856=ORIENTED_EDGE('',*,*,#28165,.T.) ;
#39857=ORIENTED_EDGE('',*,*,#28426,.T.) ;
#39858=ORIENTED_EDGE('',*,*,#28375,.F.) ;
#39859=ORIENTED_EDGE('',*,*,#28427,.F.) ;
#39860=ORIENTED_EDGE('',*,*,#28166,.T.) ;
#39861=ORIENTED_EDGE('',*,*,#28425,.T.) ;
#39862=ORIENTED_EDGE('',*,*,#28377,.F.) ;
#39863=ORIENTED_EDGE('',*,*,#28428,.F.) ;
#39864=ORIENTED_EDGE('',*,*,#28167,.T.) ;
#39865=ORIENTED_EDGE('',*,*,#28427,.T.) ;
#39866=ORIENTED_EDGE('',*,*,#28414,.F.) ;
#39867=ORIENTED_EDGE('',*,*,#28411,.F.) ;
#39868=ORIENTED_EDGE('',*,*,#28429,.T.) ;
#39869=ORIENTED_EDGE('',*,*,#28430,.T.) ;
#39870=ORIENTED_EDGE('',*,*,#28431,.T.) ;
#39871=ORIENTED_EDGE('',*,*,#27824,.F.) ;
#39872=ORIENTED_EDGE('',*,*,#27828,.F.) ;
#39873=ORIENTED_EDGE('',*,*,#28426,.F.) ;
#39874=ORIENTED_EDGE('',*,*,#28172,.T.) ;
#39875=ORIENTED_EDGE('',*,*,#28432,.T.) ;
#39876=ORIENTED_EDGE('',*,*,#28390,.F.) ;
#39877=ORIENTED_EDGE('',*,*,#28433,.F.) ;
#39878=ORIENTED_EDGE('',*,*,#28434,.T.) ;
#39879=ORIENTED_EDGE('',*,*,#28422,.F.) ;
#39880=ORIENTED_EDGE('',*,*,#28368,.F.) ;
#39881=ORIENTED_EDGE('',*,*,#28410,.F.) ;
#39882=ORIENTED_EDGE('',*,*,#28336,.F.) ;
#39883=ORIENTED_EDGE('',*,*,#28435,.T.) ;
#39884=ORIENTED_EDGE('',*,*,#28429,.F.) ;
#39885=ORIENTED_EDGE('',*,*,#27814,.F.) ;
#39886=ORIENTED_EDGE('',*,*,#27818,.F.) ;
#39887=ORIENTED_EDGE('',*,*,#28431,.F.) ;
#39888=ORIENTED_EDGE('',*,*,#28436,.T.) ;
#39889=ORIENTED_EDGE('',*,*,#28437,.F.) ;
#39890=ORIENTED_EDGE('',*,*,#28402,.F.) ;
#39891=ORIENTED_EDGE('',*,*,#28438,.F.) ;
#39892=ORIENTED_EDGE('',*,*,#28168,.T.) ;
#39893=ORIENTED_EDGE('',*,*,#28428,.T.) ;
#39894=ORIENTED_EDGE('',*,*,#28378,.F.) ;
#39895=ORIENTED_EDGE('',*,*,#28337,.F.) ;
#39896=ORIENTED_EDGE('',*,*,#28345,.F.) ;
#39897=ORIENTED_EDGE('',*,*,#28344,.F.) ;
#39898=ORIENTED_EDGE('',*,*,#28416,.F.) ;
#39899=ORIENTED_EDGE('',*,*,#28439,.T.) ;
#39900=ORIENTED_EDGE('',*,*,#28335,.T.) ;
#39901=ORIENTED_EDGE('',*,*,#28439,.F.) ;
#39902=ORIENTED_EDGE('',*,*,#28415,.T.) ;
#39903=ORIENTED_EDGE('',*,*,#28440,.F.) ;
#39904=ORIENTED_EDGE('',*,*,#28441,.F.) ;
#39905=ORIENTED_EDGE('',*,*,#28436,.F.) ;
#39906=ORIENTED_EDGE('',*,*,#28430,.F.) ;
#39907=ORIENTED_EDGE('',*,*,#28435,.F.) ;
#39908=ORIENTED_EDGE('',*,*,#28442,.T.) ;
#39909=ORIENTED_EDGE('',*,*,#28443,.T.) ;
#39910=ORIENTED_EDGE('',*,*,#28444,.T.) ;
#39911=ORIENTED_EDGE('',*,*,#28445,.T.) ;
#39912=ORIENTED_EDGE('',*,*,#28443,.F.) ;
#39913=ORIENTED_EDGE('',*,*,#28446,.F.) ;
#39914=ORIENTED_EDGE('',*,*,#28447,.F.) ;
#39915=ORIENTED_EDGE('',*,*,#28448,.F.) ;
#39916=ORIENTED_EDGE('',*,*,#28449,.T.) ;
#39917=ORIENTED_EDGE('',*,*,#28447,.T.) ;
#39918=ORIENTED_EDGE('',*,*,#28450,.T.) ;
#39919=ORIENTED_EDGE('',*,*,#28451,.T.) ;
#39920=ORIENTED_EDGE('',*,*,#28452,.T.) ;
#39921=ORIENTED_EDGE('',*,*,#28453,.F.) ;
#39922=ORIENTED_EDGE('',*,*,#28454,.F.) ;
#39923=ORIENTED_EDGE('',*,*,#28455,.F.) ;
#39924=ORIENTED_EDGE('',*,*,#28456,.F.) ;
#39925=ORIENTED_EDGE('',*,*,#28457,.F.) ;
#39926=ORIENTED_EDGE('',*,*,#28458,.T.) ;
#39927=ORIENTED_EDGE('',*,*,#28459,.F.) ;
#39928=ORIENTED_EDGE('',*,*,#28453,.T.) ;
#39929=ORIENTED_EDGE('',*,*,#28460,.T.) ;
#39930=ORIENTED_EDGE('',*,*,#28457,.T.) ;
#39931=ORIENTED_EDGE('',*,*,#28461,.T.) ;
#39932=ORIENTED_EDGE('',*,*,#28462,.T.) ;
#39933=ORIENTED_EDGE('',*,*,#28463,.T.) ;
#39934=ORIENTED_EDGE('',*,*,#28464,.T.) ;
#39935=ORIENTED_EDGE('',*,*,#28465,.T.) ;
#39936=ORIENTED_EDGE('',*,*,#28466,.T.) ;
#39937=ORIENTED_EDGE('',*,*,#28467,.T.) ;
#39938=ORIENTED_EDGE('',*,*,#28462,.F.) ;
#39939=ORIENTED_EDGE('',*,*,#28468,.T.) ;
#39940=ORIENTED_EDGE('',*,*,#28459,.T.) ;
#39941=ORIENTED_EDGE('',*,*,#28469,.T.) ;
#39942=ORIENTED_EDGE('',*,*,#28466,.F.) ;
#39943=ORIENTED_EDGE('',*,*,#28470,.T.) ;
#39944=ORIENTED_EDGE('',*,*,#28471,.F.) ;
#39945=ORIENTED_EDGE('',*,*,#28472,.T.) ;
#39946=ORIENTED_EDGE('',*,*,#28456,.T.) ;
#39947=ORIENTED_EDGE('',*,*,#28473,.T.) ;
#39948=ORIENTED_EDGE('',*,*,#28474,.F.) ;
#39949=ORIENTED_EDGE('',*,*,#28475,.T.) ;
#39950=ORIENTED_EDGE('',*,*,#28454,.T.) ;
#39951=ORIENTED_EDGE('',*,*,#28476,.T.) ;
#39952=ORIENTED_EDGE('',*,*,#28477,.T.) ;
#39953=ORIENTED_EDGE('',*,*,#28478,.T.) ;
#39954=ORIENTED_EDGE('',*,*,#28455,.T.) ;
#39955=ORIENTED_EDGE('',*,*,#28479,.T.) ;
#39956=ORIENTED_EDGE('',*,*,#28480,.T.) ;
#39957=ORIENTED_EDGE('',*,*,#28481,.T.) ;
#39958=ORIENTED_EDGE('',*,*,#28477,.F.) ;
#39959=ORIENTED_EDGE('',*,*,#28482,.T.) ;
#39960=ORIENTED_EDGE('',*,*,#28483,.T.) ;
#39961=ORIENTED_EDGE('',*,*,#28484,.T.) ;
#39962=ORIENTED_EDGE('',*,*,#28480,.F.) ;
#39963=ORIENTED_EDGE('',*,*,#28485,.T.) ;
#39964=ORIENTED_EDGE('',*,*,#28467,.F.) ;
#39965=ORIENTED_EDGE('',*,*,#28486,.T.) ;
#39966=ORIENTED_EDGE('',*,*,#28487,.F.) ;
#39967=ORIENTED_EDGE('',*,*,#28488,.F.) ;
#39968=ORIENTED_EDGE('',*,*,#28469,.F.) ;
#39969=ORIENTED_EDGE('',*,*,#28458,.F.) ;
#39970=ORIENTED_EDGE('',*,*,#28460,.F.) ;
#39971=ORIENTED_EDGE('',*,*,#28452,.F.) ;
#39972=ORIENTED_EDGE('',*,*,#28478,.F.) ;
#39973=ORIENTED_EDGE('',*,*,#28489,.F.) ;
#39974=ORIENTED_EDGE('',*,*,#28490,.F.) ;
#39975=ORIENTED_EDGE('',*,*,#28491,.F.) ;
#39976=ORIENTED_EDGE('',*,*,#28492,.F.) ;
#39977=ORIENTED_EDGE('',*,*,#28493,.F.) ;
#39978=ORIENTED_EDGE('',*,*,#28494,.F.) ;
#39979=ORIENTED_EDGE('',*,*,#28495,.F.) ;
#39980=ORIENTED_EDGE('',*,*,#28496,.F.) ;
#39981=ORIENTED_EDGE('',*,*,#28497,.F.) ;
#39982=ORIENTED_EDGE('',*,*,#28498,.F.) ;
#39983=ORIENTED_EDGE('',*,*,#28499,.F.) ;
#39984=ORIENTED_EDGE('',*,*,#28486,.F.) ;
#39985=ORIENTED_EDGE('',*,*,#28481,.F.) ;
#39986=ORIENTED_EDGE('',*,*,#28500,.F.) ;
#39987=ORIENTED_EDGE('',*,*,#28501,.F.) ;
#39988=ORIENTED_EDGE('',*,*,#28489,.T.) ;
#39989=ORIENTED_EDGE('',*,*,#27829,.F.) ;
#39990=ORIENTED_EDGE('',*,*,#27731,.F.) ;
#39991=ORIENTED_EDGE('',*,*,#28502,.F.) ;
#39992=ORIENTED_EDGE('',*,*,#28503,.T.) ;
#39993=ORIENTED_EDGE('',*,*,#28504,.F.) ;
#39994=ORIENTED_EDGE('',*,*,#28505,.F.) ;
#39995=ORIENTED_EDGE('',*,*,#28506,.F.) ;
#39996=ORIENTED_EDGE('',*,*,#28500,.T.) ;
#39997=ORIENTED_EDGE('',*,*,#28484,.F.) ;
#39998=ORIENTED_EDGE('',*,*,#28507,.T.) ;
#39999=ORIENTED_EDGE('',*,*,#28463,.F.) ;
#40000=ORIENTED_EDGE('',*,*,#28488,.T.) ;
#40001=ORIENTED_EDGE('',*,*,#28508,.F.) ;
#40002=ORIENTED_EDGE('',*,*,#28305,.T.) ;
#40003=ORIENTED_EDGE('',*,*,#28509,.T.) ;
#40004=ORIENTED_EDGE('',*,*,#28510,.T.) ;
#40005=ORIENTED_EDGE('',*,*,#28511,.T.) ;
#40006=ORIENTED_EDGE('',*,*,#27772,.F.) ;
#40007=ORIENTED_EDGE('',*,*,#28307,.T.) ;
#40008=ORIENTED_EDGE('',*,*,#28512,.T.) ;
#40009=ORIENTED_EDGE('',*,*,#28513,.T.) ;
#40010=ORIENTED_EDGE('',*,*,#27787,.F.) ;
#40011=ORIENTED_EDGE('',*,*,#28514,.T.) ;
#40012=ORIENTED_EDGE('',*,*,#28512,.F.) ;
#40013=ORIENTED_EDGE('',*,*,#28306,.T.) ;
#40014=ORIENTED_EDGE('',*,*,#28511,.F.) ;
#40015=ORIENTED_EDGE('',*,*,#28515,.T.) ;
#40016=ORIENTED_EDGE('',*,*,#28516,.T.) ;
#40017=ORIENTED_EDGE('',*,*,#28509,.F.) ;
#40018=ORIENTED_EDGE('',*,*,#28309,.T.) ;
#40019=ORIENTED_EDGE('',*,*,#28517,.T.) ;
#40020=ORIENTED_EDGE('',*,*,#28518,.T.) ;
#40021=ORIENTED_EDGE('',*,*,#28515,.F.) ;
#40022=ORIENTED_EDGE('',*,*,#28311,.T.) ;
#40023=ORIENTED_EDGE('',*,*,#28519,.T.) ;
#40024=ORIENTED_EDGE('',*,*,#28520,.T.) ;
#40025=ORIENTED_EDGE('',*,*,#28517,.F.) ;
#40026=ORIENTED_EDGE('',*,*,#28313,.T.) ;
#40027=ORIENTED_EDGE('',*,*,#28521,.T.) ;
#40028=ORIENTED_EDGE('',*,*,#28522,.T.) ;
#40029=ORIENTED_EDGE('',*,*,#28519,.F.) ;
#40030=ORIENTED_EDGE('',*,*,#28321,.T.) ;
#40031=ORIENTED_EDGE('',*,*,#28523,.T.) ;
#40032=ORIENTED_EDGE('',*,*,#28524,.T.) ;
#40033=ORIENTED_EDGE('',*,*,#28521,.F.) ;
#40034=ORIENTED_EDGE('',*,*,#28320,.T.) ;
#40035=ORIENTED_EDGE('',*,*,#28525,.T.) ;
#40036=ORIENTED_EDGE('',*,*,#28526,.T.) ;
#40037=ORIENTED_EDGE('',*,*,#28523,.F.) ;
#40038=ORIENTED_EDGE('',*,*,#28319,.T.) ;
#40039=ORIENTED_EDGE('',*,*,#28527,.T.) ;
#40040=ORIENTED_EDGE('',*,*,#28528,.T.) ;
#40041=ORIENTED_EDGE('',*,*,#28525,.F.) ;
#40042=ORIENTED_EDGE('',*,*,#28318,.T.) ;
#40043=ORIENTED_EDGE('',*,*,#28529,.T.) ;
#40044=ORIENTED_EDGE('',*,*,#28530,.T.) ;
#40045=ORIENTED_EDGE('',*,*,#28527,.F.) ;
#40046=ORIENTED_EDGE('',*,*,#28317,.T.) ;
#40047=ORIENTED_EDGE('',*,*,#28531,.T.) ;
#40048=ORIENTED_EDGE('',*,*,#28532,.T.) ;
#40049=ORIENTED_EDGE('',*,*,#28529,.F.) ;
#40050=ORIENTED_EDGE('',*,*,#28316,.T.) ;
#40051=ORIENTED_EDGE('',*,*,#28533,.T.) ;
#40052=ORIENTED_EDGE('',*,*,#28534,.T.) ;
#40053=ORIENTED_EDGE('',*,*,#28531,.F.) ;
#40054=ORIENTED_EDGE('',*,*,#28315,.T.) ;
#40055=ORIENTED_EDGE('',*,*,#28535,.T.) ;
#40056=ORIENTED_EDGE('',*,*,#28536,.T.) ;
#40057=ORIENTED_EDGE('',*,*,#28533,.F.) ;
#40058=ORIENTED_EDGE('',*,*,#28323,.T.) ;
#40059=ORIENTED_EDGE('',*,*,#28537,.T.) ;
#40060=ORIENTED_EDGE('',*,*,#28538,.T.) ;
#40061=ORIENTED_EDGE('',*,*,#28535,.F.) ;
#40062=ORIENTED_EDGE('',*,*,#28325,.T.) ;
#40063=ORIENTED_EDGE('',*,*,#28539,.T.) ;
#40064=ORIENTED_EDGE('',*,*,#28540,.T.) ;
#40065=ORIENTED_EDGE('',*,*,#28537,.F.) ;
#40066=ORIENTED_EDGE('',*,*,#28327,.T.) ;
#40067=ORIENTED_EDGE('',*,*,#28541,.T.) ;
#40068=ORIENTED_EDGE('',*,*,#28542,.T.) ;
#40069=ORIENTED_EDGE('',*,*,#28539,.F.) ;
#40070=ORIENTED_EDGE('',*,*,#28330,.T.) ;
#40071=ORIENTED_EDGE('',*,*,#28543,.T.) ;
#40072=ORIENTED_EDGE('',*,*,#28544,.T.) ;
#40073=ORIENTED_EDGE('',*,*,#28541,.F.) ;
#40074=ORIENTED_EDGE('',*,*,#28329,.T.) ;
#40075=ORIENTED_EDGE('',*,*,#28545,.T.) ;
#40076=ORIENTED_EDGE('',*,*,#27615,.T.) ;
#40077=ORIENTED_EDGE('',*,*,#28543,.F.) ;
#40078=ORIENTED_EDGE('',*,*,#28328,.T.) ;
#40079=ORIENTED_EDGE('',*,*,#28546,.T.) ;
#40080=ORIENTED_EDGE('',*,*,#27616,.T.) ;
#40081=ORIENTED_EDGE('',*,*,#28545,.F.) ;
#40082=ORIENTED_EDGE('',*,*,#27926,.T.) ;
#40083=ORIENTED_EDGE('',*,*,#28547,.T.) ;
#40084=ORIENTED_EDGE('',*,*,#27617,.T.) ;
#40085=ORIENTED_EDGE('',*,*,#28546,.F.) ;
#40086=ORIENTED_EDGE('',*,*,#28548,.T.) ;
#40087=ORIENTED_EDGE('',*,*,#28549,.T.) ;
#40088=ORIENTED_EDGE('',*,*,#27618,.T.) ;
#40089=ORIENTED_EDGE('',*,*,#28547,.F.) ;
#40090=ORIENTED_EDGE('',*,*,#28550,.T.) ;
#40091=ORIENTED_EDGE('',*,*,#28551,.T.) ;
#40092=ORIENTED_EDGE('',*,*,#27619,.T.) ;
#40093=ORIENTED_EDGE('',*,*,#28549,.F.) ;
#40094=ORIENTED_EDGE('',*,*,#28552,.T.) ;
#40095=ORIENTED_EDGE('',*,*,#28553,.T.) ;
#40096=ORIENTED_EDGE('',*,*,#27620,.T.) ;
#40097=ORIENTED_EDGE('',*,*,#28551,.F.) ;
#40098=ORIENTED_EDGE('',*,*,#28554,.T.) ;
#40099=ORIENTED_EDGE('',*,*,#28555,.T.) ;
#40100=ORIENTED_EDGE('',*,*,#27621,.T.) ;
#40101=ORIENTED_EDGE('',*,*,#28553,.F.) ;
#40102=ORIENTED_EDGE('',*,*,#28556,.T.) ;
#40103=ORIENTED_EDGE('',*,*,#28557,.T.) ;
#40104=ORIENTED_EDGE('',*,*,#27622,.T.) ;
#40105=ORIENTED_EDGE('',*,*,#28555,.F.) ;
#40106=ORIENTED_EDGE('',*,*,#28242,.T.) ;
#40107=ORIENTED_EDGE('',*,*,#28558,.T.) ;
#40108=ORIENTED_EDGE('',*,*,#27623,.T.) ;
#40109=ORIENTED_EDGE('',*,*,#28557,.F.) ;
#40110=ORIENTED_EDGE('',*,*,#28247,.T.) ;
#40111=ORIENTED_EDGE('',*,*,#27979,.T.) ;
#40112=ORIENTED_EDGE('',*,*,#27624,.T.) ;
#40113=ORIENTED_EDGE('',*,*,#28558,.F.) ;
#40114=ORIENTED_EDGE('',*,*,#28559,.T.) ;
#40115=ORIENTED_EDGE('',*,*,#27980,.F.) ;
#40116=ORIENTED_EDGE('',*,*,#28560,.F.) ;
#40117=ORIENTED_EDGE('',*,*,#28561,.F.) ;
#40118=ORIENTED_EDGE('',*,*,#27977,.T.) ;
#40119=ORIENTED_EDGE('',*,*,#28559,.F.) ;
#40120=ORIENTED_EDGE('',*,*,#28246,.F.) ;
#40121=ORIENTED_EDGE('',*,*,#28562,.F.) ;
#40122=ORIENTED_EDGE('',*,*,#28560,.T.) ;
#40123=ORIENTED_EDGE('',*,*,#27873,.F.) ;
#40124=ORIENTED_EDGE('',*,*,#28243,.T.) ;
#40125=ORIENTED_EDGE('',*,*,#28556,.F.) ;
#40126=ORIENTED_EDGE('',*,*,#28563,.F.) ;
#40127=ORIENTED_EDGE('',*,*,#27876,.F.) ;
#40128=ORIENTED_EDGE('',*,*,#28563,.T.) ;
#40129=ORIENTED_EDGE('',*,*,#28554,.F.) ;
#40130=ORIENTED_EDGE('',*,*,#28564,.T.) ;
#40131=ORIENTED_EDGE('',*,*,#27879,.F.) ;
#40132=ORIENTED_EDGE('',*,*,#28564,.F.) ;
#40133=ORIENTED_EDGE('',*,*,#28552,.F.) ;
#40134=ORIENTED_EDGE('',*,*,#28565,.F.) ;
#40135=ORIENTED_EDGE('',*,*,#27882,.F.) ;
#40136=ORIENTED_EDGE('',*,*,#28565,.T.) ;
#40137=ORIENTED_EDGE('',*,*,#28550,.F.) ;
#40138=ORIENTED_EDGE('',*,*,#28566,.F.) ;
#40139=ORIENTED_EDGE('',*,*,#27885,.F.) ;
#40140=ORIENTED_EDGE('',*,*,#28566,.T.) ;
#40141=ORIENTED_EDGE('',*,*,#28548,.F.) ;
#40142=ORIENTED_EDGE('',*,*,#27925,.F.) ;
#40143=ORIENTED_EDGE('',*,*,#27830,.F.) ;
#40144=ORIENTED_EDGE('',*,*,#28508,.T.) ;
#40145=ORIENTED_EDGE('',*,*,#28567,.T.) ;
#40146=ORIENTED_EDGE('',*,*,#28568,.T.) ;
#40147=ORIENTED_EDGE('',*,*,#27713,.F.) ;
#40148=ORIENTED_EDGE('',*,*,#27759,.T.) ;
#40149=ORIENTED_EDGE('',*,*,#28569,.T.) ;
#40150=ORIENTED_EDGE('',*,*,#28502,.T.) ;
#40151=ORIENTED_EDGE('',*,*,#27714,.F.) ;
#40152=ORIENTED_EDGE('',*,*,#28570,.T.) ;
#40153=ORIENTED_EDGE('',*,*,#28571,.T.) ;
#40154=ORIENTED_EDGE('',*,*,#27756,.T.) ;
#40155=ORIENTED_EDGE('',*,*,#27761,.F.) ;
#40156=ORIENTED_EDGE('',*,*,#28572,.T.) ;
#40157=ORIENTED_EDGE('',*,*,#27757,.T.) ;
#40158=ORIENTED_EDGE('',*,*,#28571,.F.) ;
#40159=ORIENTED_EDGE('',*,*,#28573,.T.) ;
#40160=ORIENTED_EDGE('',*,*,#27758,.T.) ;
#40161=ORIENTED_EDGE('',*,*,#28572,.F.) ;
#40162=ORIENTED_EDGE('',*,*,#28574,.T.) ;
#40163=ORIENTED_EDGE('',*,*,#28569,.F.) ;
#40164=ORIENTED_EDGE('',*,*,#28575,.T.) ;
#40165=ORIENTED_EDGE('',*,*,#28576,.T.) ;
#40166=ORIENTED_EDGE('',*,*,#28567,.F.) ;
#40167=ORIENTED_EDGE('',*,*,#28487,.T.) ;
#40168=ORIENTED_EDGE('',*,*,#28577,.T.) ;
#40169=ORIENTED_EDGE('',*,*,#28578,.T.) ;
#40170=ORIENTED_EDGE('',*,*,#28575,.F.) ;
#40171=ORIENTED_EDGE('',*,*,#28499,.T.) ;
#40172=ORIENTED_EDGE('',*,*,#28579,.T.) ;
#40173=ORIENTED_EDGE('',*,*,#28580,.T.) ;
#40174=ORIENTED_EDGE('',*,*,#28577,.F.) ;
#40175=ORIENTED_EDGE('',*,*,#28498,.T.) ;
#40176=ORIENTED_EDGE('',*,*,#28581,.T.) ;
#40177=ORIENTED_EDGE('',*,*,#27820,.T.) ;
#40178=ORIENTED_EDGE('',*,*,#28579,.F.) ;
#40179=ORIENTED_EDGE('',*,*,#28497,.T.) ;
#40180=ORIENTED_EDGE('',*,*,#28582,.T.) ;
#40181=ORIENTED_EDGE('',*,*,#28418,.T.) ;
#40182=ORIENTED_EDGE('',*,*,#28581,.F.) ;
#40183=ORIENTED_EDGE('',*,*,#28496,.T.) ;
#40184=ORIENTED_EDGE('',*,*,#28583,.T.) ;
#40185=ORIENTED_EDGE('',*,*,#28584,.T.) ;
#40186=ORIENTED_EDGE('',*,*,#28582,.F.) ;
#40187=ORIENTED_EDGE('',*,*,#28495,.T.) ;
#40188=ORIENTED_EDGE('',*,*,#28585,.T.) ;
#40189=ORIENTED_EDGE('',*,*,#28586,.T.) ;
#40190=ORIENTED_EDGE('',*,*,#28583,.F.) ;
#40191=ORIENTED_EDGE('',*,*,#28494,.T.) ;
#40192=ORIENTED_EDGE('',*,*,#28587,.T.) ;
#40193=ORIENTED_EDGE('',*,*,#28585,.F.) ;
#40194=ORIENTED_EDGE('',*,*,#28493,.T.) ;
#40195=ORIENTED_EDGE('',*,*,#28588,.T.) ;
#40196=ORIENTED_EDGE('',*,*,#28589,.T.) ;
#40197=ORIENTED_EDGE('',*,*,#28590,.T.) ;
#40198=ORIENTED_EDGE('',*,*,#28591,.T.) ;
#40199=ORIENTED_EDGE('',*,*,#28592,.T.) ;
#40200=ORIENTED_EDGE('',*,*,#28593,.T.) ;
#40201=ORIENTED_EDGE('',*,*,#28594,.T.) ;
#40202=ORIENTED_EDGE('',*,*,#28591,.F.) ;
#40203=ORIENTED_EDGE('',*,*,#28595,.T.) ;
#40204=ORIENTED_EDGE('',*,*,#28596,.T.) ;
#40205=ORIENTED_EDGE('',*,*,#28506,.T.) ;
#40206=ORIENTED_EDGE('',*,*,#28593,.F.) ;
#40207=ORIENTED_EDGE('',*,*,#28597,.T.) ;
#40208=ORIENTED_EDGE('',*,*,#28598,.T.) ;
#40209=ORIENTED_EDGE('',*,*,#28501,.T.) ;
#40210=ORIENTED_EDGE('',*,*,#28596,.F.) ;
#40211=ORIENTED_EDGE('',*,*,#28599,.T.) ;
#40212=ORIENTED_EDGE('',*,*,#28600,.T.) ;
#40213=ORIENTED_EDGE('',*,*,#28490,.T.) ;
#40214=ORIENTED_EDGE('',*,*,#28598,.F.) ;
#40215=ORIENTED_EDGE('',*,*,#28601,.T.) ;
#40216=ORIENTED_EDGE('',*,*,#28602,.T.) ;
#40217=ORIENTED_EDGE('',*,*,#28491,.T.) ;
#40218=ORIENTED_EDGE('',*,*,#28600,.F.) ;
#40219=ORIENTED_EDGE('',*,*,#28603,.T.) ;
#40220=ORIENTED_EDGE('',*,*,#28492,.T.) ;
#40221=ORIENTED_EDGE('',*,*,#28602,.F.) ;
#40222=ORIENTED_EDGE('',*,*,#28604,.T.) ;
#40223=ORIENTED_EDGE('',*,*,#28588,.F.) ;
#40224=ORIENTED_EDGE('',*,*,#27739,.F.) ;
#40225=ORIENTED_EDGE('',*,*,#27844,.F.) ;
#40226=ORIENTED_EDGE('',*,*,#27843,.F.) ;
#40227=ORIENTED_EDGE('',*,*,#27840,.F.) ;
#40228=ORIENTED_EDGE('',*,*,#27762,.F.) ;
#40229=ORIENTED_EDGE('',*,*,#27834,.F.) ;
#40230=ORIENTED_EDGE('',*,*,#28568,.F.) ;
#40231=ORIENTED_EDGE('',*,*,#28576,.F.) ;
#40232=ORIENTED_EDGE('',*,*,#28578,.F.) ;
#40233=ORIENTED_EDGE('',*,*,#28605,.F.) ;
#40234=ORIENTED_EDGE('',*,*,#27833,.F.) ;
#40235=ORIENTED_EDGE('',*,*,#28605,.T.) ;
#40236=ORIENTED_EDGE('',*,*,#28580,.F.) ;
#40237=ORIENTED_EDGE('',*,*,#27819,.T.) ;
#40238=ORIENTED_EDGE('',*,*,#28343,.F.) ;
#40239=ORIENTED_EDGE('',*,*,#28419,.F.) ;
#40240=ORIENTED_EDGE('',*,*,#28584,.F.) ;
#40241=ORIENTED_EDGE('',*,*,#28606,.F.) ;
#40242=ORIENTED_EDGE('',*,*,#28607,.F.) ;
#40243=ORIENTED_EDGE('',*,*,#28608,.F.) ;
#40244=ORIENTED_EDGE('',*,*,#28609,.F.) ;
#40245=ORIENTED_EDGE('',*,*,#28610,.F.) ;
#40246=ORIENTED_EDGE('',*,*,#28611,.F.) ;
#40247=ORIENTED_EDGE('',*,*,#28420,.F.) ;
#40248=ORIENTED_EDGE('',*,*,#28358,.F.) ;
#40249=ORIENTED_EDGE('',*,*,#28347,.F.) ;
#40250=ORIENTED_EDGE('',*,*,#28383,.F.) ;
#40251=ORIENTED_EDGE('',*,*,#28386,.F.) ;
#40252=ORIENTED_EDGE('',*,*,#28389,.F.) ;
#40253=ORIENTED_EDGE('',*,*,#28392,.F.) ;
#40254=ORIENTED_EDGE('',*,*,#28395,.F.) ;
#40255=ORIENTED_EDGE('',*,*,#28398,.F.) ;
#40256=ORIENTED_EDGE('',*,*,#28401,.F.) ;
#40257=ORIENTED_EDGE('',*,*,#28404,.F.) ;
#40258=ORIENTED_EDGE('',*,*,#28406,.F.) ;
#40259=ORIENTED_EDGE('',*,*,#28340,.F.) ;
#40260=ORIENTED_EDGE('',*,*,#28612,.F.) ;
#40261=ORIENTED_EDGE('',*,*,#28613,.F.) ;
#40262=ORIENTED_EDGE('',*,*,#28614,.F.) ;
#40263=ORIENTED_EDGE('',*,*,#28615,.F.) ;
#40264=ORIENTED_EDGE('',*,*,#28616,.F.) ;
#40265=ORIENTED_EDGE('',*,*,#28617,.F.) ;
#40266=ORIENTED_EDGE('',*,*,#28618,.F.) ;
#40267=ORIENTED_EDGE('',*,*,#28619,.F.) ;
#40268=ORIENTED_EDGE('',*,*,#28620,.F.) ;
#40269=ORIENTED_EDGE('',*,*,#28621,.F.) ;
#40270=ORIENTED_EDGE('',*,*,#28622,.F.) ;
#40271=ORIENTED_EDGE('',*,*,#28623,.F.) ;
#40272=ORIENTED_EDGE('',*,*,#28624,.F.) ;
#40273=ORIENTED_EDGE('',*,*,#28625,.F.) ;
#40274=ORIENTED_EDGE('',*,*,#28586,.F.) ;
#40275=ORIENTED_EDGE('',*,*,#28626,.T.) ;
#40276=ORIENTED_EDGE('',*,*,#28627,.T.) ;
#40277=ORIENTED_EDGE('',*,*,#28606,.T.) ;
#40278=ORIENTED_EDGE('',*,*,#28587,.F.) ;
#40279=ORIENTED_EDGE('',*,*,#28628,.T.) ;
#40280=ORIENTED_EDGE('',*,*,#28629,.F.) ;
#40281=ORIENTED_EDGE('',*,*,#28630,.F.) ;
#40282=ORIENTED_EDGE('',*,*,#28626,.F.) ;
#40283=ORIENTED_EDGE('',*,*,#28604,.F.) ;
#40284=ORIENTED_EDGE('',*,*,#28631,.F.) ;
#40285=ORIENTED_EDGE('',*,*,#28632,.T.) ;
#40286=ORIENTED_EDGE('',*,*,#28100,.F.) ;
#40287=ORIENTED_EDGE('',*,*,#28633,.F.) ;
#40288=ORIENTED_EDGE('',*,*,#28634,.F.) ;
#40289=ORIENTED_EDGE('',*,*,#28628,.F.) ;
#40290=ORIENTED_EDGE('',*,*,#28635,.T.) ;
#40291=ORIENTED_EDGE('',*,*,#28603,.F.) ;
#40292=ORIENTED_EDGE('',*,*,#28636,.T.) ;
#40293=ORIENTED_EDGE('',*,*,#28637,.T.) ;
#40294=ORIENTED_EDGE('',*,*,#28631,.T.) ;
#40295=ORIENTED_EDGE('',*,*,#28601,.F.) ;
#40296=ORIENTED_EDGE('',*,*,#28599,.F.) ;
#40297=ORIENTED_EDGE('',*,*,#28597,.F.) ;
#40298=ORIENTED_EDGE('',*,*,#28595,.F.) ;
#40299=ORIENTED_EDGE('',*,*,#28590,.F.) ;
#40300=ORIENTED_EDGE('',*,*,#28638,.T.) ;
#40301=ORIENTED_EDGE('',*,*,#28639,.T.) ;
#40302=ORIENTED_EDGE('',*,*,#28640,.F.) ;
#40303=ORIENTED_EDGE('',*,*,#28641,.F.) ;
#40304=ORIENTED_EDGE('',*,*,#28636,.F.) ;
#40305=ORIENTED_EDGE('',*,*,#28589,.F.) ;
#40306=ORIENTED_EDGE('',*,*,#28642,.T.) ;
#40307=ORIENTED_EDGE('',*,*,#28104,.F.) ;
#40308=ORIENTED_EDGE('',*,*,#28643,.F.) ;
#40309=ORIENTED_EDGE('',*,*,#28638,.F.) ;
#40310=ORIENTED_EDGE('',*,*,#28644,.T.) ;
#40311=ORIENTED_EDGE('',*,*,#28645,.F.) ;
#40312=ORIENTED_EDGE('',*,*,#28646,.F.) ;
#40313=ORIENTED_EDGE('',*,*,#28647,.F.) ;
#40314=ORIENTED_EDGE('',*,*,#28648,.T.) ;
#40315=ORIENTED_EDGE('',*,*,#28649,.F.) ;
#40316=ORIENTED_EDGE('',*,*,#28650,.F.) ;
#40317=ORIENTED_EDGE('',*,*,#28651,.F.) ;
#40318=ORIENTED_EDGE('',*,*,#27947,.F.) ;
#40319=ORIENTED_EDGE('',*,*,#28652,.T.) ;
#40320=ORIENTED_EDGE('',*,*,#28653,.T.) ;
#40321=ORIENTED_EDGE('',*,*,#28654,.T.) ;
#40322=ORIENTED_EDGE('',*,*,#28655,.T.) ;
#40323=ORIENTED_EDGE('',*,*,#28656,.T.) ;
#40324=ORIENTED_EDGE('',*,*,#28653,.F.) ;
#40325=ORIENTED_EDGE('',*,*,#28657,.T.) ;
#40326=ORIENTED_EDGE('',*,*,#28658,.T.) ;
#40327=ORIENTED_EDGE('',*,*,#28659,.T.) ;
#40328=ORIENTED_EDGE('',*,*,#28655,.F.) ;
#40329=ORIENTED_EDGE('',*,*,#28660,.T.) ;
#40330=ORIENTED_EDGE('',*,*,#28649,.T.) ;
#40331=ORIENTED_EDGE('',*,*,#28661,.T.) ;
#40332=ORIENTED_EDGE('',*,*,#28658,.F.) ;
#40333=ORIENTED_EDGE('',*,*,#28662,.T.) ;
#40334=ORIENTED_EDGE('',*,*,#28663,.F.) ;
#40335=ORIENTED_EDGE('',*,*,#28664,.T.) ;
#40336=ORIENTED_EDGE('',*,*,#28650,.T.) ;
#40337=ORIENTED_EDGE('',*,*,#28665,.T.) ;
#40338=ORIENTED_EDGE('',*,*,#28645,.T.) ;
#40339=ORIENTED_EDGE('',*,*,#28666,.T.) ;
#40340=ORIENTED_EDGE('',*,*,#28651,.T.) ;
#40341=ORIENTED_EDGE('',*,*,#28667,.T.) ;
#40342=ORIENTED_EDGE('',*,*,#28668,.F.) ;
#40343=ORIENTED_EDGE('',*,*,#28669,.T.) ;
#40344=ORIENTED_EDGE('',*,*,#28646,.T.) ;
#40345=ORIENTED_EDGE('',*,*,#28670,.T.) ;
#40346=ORIENTED_EDGE('',*,*,#28671,.T.) ;
#40347=ORIENTED_EDGE('',*,*,#28672,.T.) ;
#40348=ORIENTED_EDGE('',*,*,#28647,.T.) ;
#40349=ORIENTED_EDGE('',*,*,#28673,.T.) ;
#40350=ORIENTED_EDGE('',*,*,#28674,.T.) ;
#40351=ORIENTED_EDGE('',*,*,#28675,.T.) ;
#40352=ORIENTED_EDGE('',*,*,#28671,.F.) ;
#40353=ORIENTED_EDGE('',*,*,#28003,.T.) ;
#40354=ORIENTED_EDGE('',*,*,#28013,.T.) ;
#40355=ORIENTED_EDGE('',*,*,#28676,.T.) ;
#40356=ORIENTED_EDGE('',*,*,#28674,.F.) ;
#40357=ORIENTED_EDGE('',*,*,#28002,.T.) ;
#40358=ORIENTED_EDGE('',*,*,#28657,.F.) ;
#40359=ORIENTED_EDGE('',*,*,#28652,.F.) ;
#40360=ORIENTED_EDGE('',*,*,#27946,.F.) ;
#40361=ORIENTED_EDGE('',*,*,#28677,.T.) ;
#40362=ORIENTED_EDGE('',*,*,#28678,.T.) ;
#40363=ORIENTED_EDGE('',*,*,#28679,.T.) ;
#40364=ORIENTED_EDGE('',*,*,#27944,.F.) ;
#40365=ORIENTED_EDGE('',*,*,#28654,.F.) ;
#40366=ORIENTED_EDGE('',*,*,#28680,.F.) ;
#40367=ORIENTED_EDGE('',*,*,#27941,.F.) ;
#40368=ORIENTED_EDGE('',*,*,#28680,.T.) ;
#40369=ORIENTED_EDGE('',*,*,#28656,.F.) ;
#40370=ORIENTED_EDGE('',*,*,#28659,.F.) ;
#40371=ORIENTED_EDGE('',*,*,#28681,.T.) ;
#40372=ORIENTED_EDGE('',*,*,#27965,.F.) ;
#40373=ORIENTED_EDGE('',*,*,#27936,.F.) ;
#40374=ORIENTED_EDGE('',*,*,#27939,.F.) ;
#40375=ORIENTED_EDGE('',*,*,#27963,.F.) ;
#40376=ORIENTED_EDGE('',*,*,#28681,.F.) ;
#40377=ORIENTED_EDGE('',*,*,#28661,.F.) ;
#40378=ORIENTED_EDGE('',*,*,#28648,.F.) ;
#40379=ORIENTED_EDGE('',*,*,#28666,.F.) ;
#40380=ORIENTED_EDGE('',*,*,#28644,.F.) ;
#40381=ORIENTED_EDGE('',*,*,#28672,.F.) ;
#40382=ORIENTED_EDGE('',*,*,#28675,.F.) ;
#40383=ORIENTED_EDGE('',*,*,#28682,.F.) ;
#40384=ORIENTED_EDGE('',*,*,#28683,.T.) ;
#40385=ORIENTED_EDGE('',*,*,#28684,.F.) ;
#40386=ORIENTED_EDGE('',*,*,#28676,.F.) ;
#40387=ORIENTED_EDGE('',*,*,#28012,.F.) ;
#40388=ORIENTED_EDGE('',*,*,#28685,.T.) ;
#40389=ORIENTED_EDGE('',*,*,#28686,.F.) ;
#40390=ORIENTED_EDGE('',*,*,#28687,.T.) ;
#40391=ORIENTED_EDGE('',*,*,#28688,.T.) ;
#40392=ORIENTED_EDGE('',*,*,#28682,.T.) ;
#40393=ORIENTED_EDGE('',*,*,#28689,.T.) ;
#40394=ORIENTED_EDGE('',*,*,#28690,.T.) ;
#40395=ORIENTED_EDGE('',*,*,#28006,.T.) ;
#40396=ORIENTED_EDGE('',*,*,#28691,.T.) ;
#40397=ORIENTED_EDGE('',*,*,#27996,.F.) ;
#40398=ORIENTED_EDGE('',*,*,#28692,.T.) ;
#40399=ORIENTED_EDGE('',*,*,#28693,.T.) ;
#40400=ORIENTED_EDGE('',*,*,#28694,.T.) ;
#40401=ORIENTED_EDGE('',*,*,#28695,.T.) ;
#40402=ORIENTED_EDGE('',*,*,#28691,.F.) ;
#40403=ORIENTED_EDGE('',*,*,#28005,.T.) ;
#40404=ORIENTED_EDGE('',*,*,#27791,.F.) ;
#40405=ORIENTED_EDGE('',*,*,#28696,.F.) ;
#40406=ORIENTED_EDGE('',*,*,#28689,.F.) ;
#40407=ORIENTED_EDGE('',*,*,#28695,.F.) ;
#40408=ORIENTED_EDGE('',*,*,#28697,.F.) ;
#40409=ORIENTED_EDGE('',*,*,#28698,.T.) ;
#40410=ORIENTED_EDGE('',*,*,#28699,.F.) ;
#40411=ORIENTED_EDGE('',*,*,#28700,.T.) ;
#40412=ORIENTED_EDGE('',*,*,#27665,.T.) ;
#40413=ORIENTED_EDGE('',*,*,#27642,.F.) ;
#40414=ORIENTED_EDGE('',*,*,#28694,.F.) ;
#40415=ORIENTED_EDGE('',*,*,#28701,.T.) ;
#40416=ORIENTED_EDGE('',*,*,#28702,.F.) ;
#40417=ORIENTED_EDGE('',*,*,#28697,.T.) ;
#40418=ORIENTED_EDGE('',*,*,#28669,.F.) ;
#40419=ORIENTED_EDGE('',*,*,#28703,.F.) ;
#40420=ORIENTED_EDGE('',*,*,#28701,.F.) ;
#40421=ORIENTED_EDGE('',*,*,#28693,.F.) ;
#40422=ORIENTED_EDGE('',*,*,#28704,.F.) ;
#40423=ORIENTED_EDGE('',*,*,#27999,.F.) ;
#40424=ORIENTED_EDGE('',*,*,#28004,.F.) ;
#40425=ORIENTED_EDGE('',*,*,#28673,.F.) ;
#40426=ORIENTED_EDGE('',*,*,#27671,.F.) ;
#40427=ORIENTED_EDGE('',*,*,#28705,.T.) ;
#40428=ORIENTED_EDGE('',*,*,#28706,.F.) ;
#40429=ORIENTED_EDGE('',*,*,#27699,.F.) ;
#40430=ORIENTED_EDGE('',*,*,#27698,.T.) ;
#40431=ORIENTED_EDGE('',*,*,#28707,.T.) ;
#40432=ORIENTED_EDGE('',*,*,#27701,.T.) ;
#40433=ORIENTED_EDGE('',*,*,#28708,.T.) ;
#40434=ORIENTED_EDGE('',*,*,#27802,.T.) ;
#40435=ORIENTED_EDGE('',*,*,#28706,.T.) ;
#40436=ORIENTED_EDGE('',*,*,#28709,.T.) ;
#40437=ORIENTED_EDGE('',*,*,#28708,.F.) ;
#40438=ORIENTED_EDGE('',*,*,#27700,.T.) ;
#40439=ORIENTED_EDGE('',*,*,#28710,.T.) ;
#40440=ORIENTED_EDGE('',*,*,#27702,.T.) ;
#40441=ORIENTED_EDGE('',*,*,#28707,.F.) ;
#40442=ORIENTED_EDGE('',*,*,#28711,.T.) ;
#40443=ORIENTED_EDGE('',*,*,#28712,.T.) ;
#40444=ORIENTED_EDGE('',*,*,#27703,.T.) ;
#40445=ORIENTED_EDGE('',*,*,#28710,.F.) ;
#40446=ORIENTED_EDGE('',*,*,#28713,.T.) ;
#40447=ORIENTED_EDGE('',*,*,#28714,.T.) ;
#40448=ORIENTED_EDGE('',*,*,#27859,.T.) ;
#40449=ORIENTED_EDGE('',*,*,#28712,.F.) ;
#40450=ORIENTED_EDGE('',*,*,#28715,.T.) ;
#40451=ORIENTED_EDGE('',*,*,#27670,.F.) ;
#40452=ORIENTED_EDGE('',*,*,#28716,.T.) ;
#40453=ORIENTED_EDGE('',*,*,#27794,.F.) ;
#40454=ORIENTED_EDGE('',*,*,#27803,.T.) ;
#40455=ORIENTED_EDGE('',*,*,#28709,.F.) ;
#40456=ORIENTED_EDGE('',*,*,#28705,.F.) ;
#40457=ORIENTED_EDGE('',*,*,#27695,.F.) ;
#40458=ORIENTED_EDGE('',*,*,#27711,.T.) ;
#40459=ORIENTED_EDGE('',*,*,#28717,.T.) ;
#40460=ORIENTED_EDGE('',*,*,#28718,.T.) ;
#40461=ORIENTED_EDGE('',*,*,#28719,.T.) ;
#40462=ORIENTED_EDGE('',*,*,#28720,.T.) ;
#40463=ORIENTED_EDGE('',*,*,#28721,.F.) ;
#40464=ORIENTED_EDGE('',*,*,#28722,.F.) ;
#40465=ORIENTED_EDGE('',*,*,#27696,.F.) ;
#40466=ORIENTED_EDGE('',*,*,#28723,.F.) ;
#40467=ORIENTED_EDGE('',*,*,#28721,.T.) ;
#40468=ORIENTED_EDGE('',*,*,#28724,.T.) ;
#40469=ORIENTED_EDGE('',*,*,#28725,.T.) ;
#40470=ORIENTED_EDGE('',*,*,#27792,.T.) ;
#40471=ORIENTED_EDGE('',*,*,#27651,.F.) ;
#40472=ORIENTED_EDGE('',*,*,#27656,.T.) ;
#40473=ORIENTED_EDGE('',*,*,#27655,.T.) ;
#40474=ORIENTED_EDGE('',*,*,#28726,.T.) ;
#40475=ORIENTED_EDGE('',*,*,#28727,.T.) ;
#40476=ORIENTED_EDGE('',*,*,#28724,.F.) ;
#40477=ORIENTED_EDGE('',*,*,#28728,.T.) ;
#40478=ORIENTED_EDGE('',*,*,#28729,.T.) ;
#40479=ORIENTED_EDGE('',*,*,#28730,.T.) ;
#40480=ORIENTED_EDGE('',*,*,#28726,.F.) ;
#40481=ORIENTED_EDGE('',*,*,#28731,.T.) ;
#40482=ORIENTED_EDGE('',*,*,#28008,.T.) ;
#40483=ORIENTED_EDGE('',*,*,#28729,.F.) ;
#40484=ORIENTED_EDGE('',*,*,#28732,.T.) ;
#40485=ORIENTED_EDGE('',*,*,#28733,.T.) ;
#40486=ORIENTED_EDGE('',*,*,#28530,.F.) ;
#40487=ORIENTED_EDGE('',*,*,#28734,.F.) ;
#40488=ORIENTED_EDGE('',*,*,#28735,.T.) ;
#40489=ORIENTED_EDGE('',*,*,#28736,.T.) ;
#40490=ORIENTED_EDGE('',*,*,#28737,.T.) ;
#40491=ORIENTED_EDGE('',*,*,#28738,.T.) ;
#40492=ORIENTED_EDGE('',*,*,#28739,.T.) ;
#40493=ORIENTED_EDGE('',*,*,#28687,.F.) ;
#40494=ORIENTED_EDGE('',*,*,#28740,.F.) ;
#40495=ORIENTED_EDGE('',*,*,#28741,.F.) ;
#40496=ORIENTED_EDGE('',*,*,#28742,.F.) ;
#40497=ORIENTED_EDGE('',*,*,#28743,.F.) ;
#40498=ORIENTED_EDGE('',*,*,#28744,.F.) ;
#40499=ORIENTED_EDGE('',*,*,#28745,.F.) ;
#40500=ORIENTED_EDGE('',*,*,#28746,.F.) ;
#40501=ORIENTED_EDGE('',*,*,#28747,.F.) ;
#40502=ORIENTED_EDGE('',*,*,#28748,.F.) ;
#40503=ORIENTED_EDGE('',*,*,#28749,.F.) ;
#40504=ORIENTED_EDGE('',*,*,#28750,.F.) ;
#40505=ORIENTED_EDGE('',*,*,#28751,.F.) ;
#40506=ORIENTED_EDGE('',*,*,#28752,.F.) ;
#40507=ORIENTED_EDGE('',*,*,#28753,.T.) ;
#40508=ORIENTED_EDGE('',*,*,#28754,.F.) ;
#40509=ORIENTED_EDGE('',*,*,#28755,.F.) ;
#40510=ORIENTED_EDGE('',*,*,#28756,.F.) ;
#40511=ORIENTED_EDGE('',*,*,#28757,.F.) ;
#40512=ORIENTED_EDGE('',*,*,#28758,.F.) ;
#40513=ORIENTED_EDGE('',*,*,#28759,.F.) ;
#40514=ORIENTED_EDGE('',*,*,#28760,.F.) ;
#40515=ORIENTED_EDGE('',*,*,#28761,.F.) ;
#40516=ORIENTED_EDGE('',*,*,#28762,.F.) ;
#40517=ORIENTED_EDGE('',*,*,#28763,.F.) ;
#40518=ORIENTED_EDGE('',*,*,#28764,.F.) ;
#40519=ORIENTED_EDGE('',*,*,#28765,.F.) ;
#40520=ORIENTED_EDGE('',*,*,#28766,.F.) ;
#40521=ORIENTED_EDGE('',*,*,#28767,.F.) ;
#40522=ORIENTED_EDGE('',*,*,#28528,.F.) ;
#40523=ORIENTED_EDGE('',*,*,#28741,.T.) ;
#40524=ORIENTED_EDGE('',*,*,#28768,.F.) ;
#40525=ORIENTED_EDGE('',*,*,#28732,.F.) ;
#40526=ORIENTED_EDGE('',*,*,#28731,.F.) ;
#40527=ORIENTED_EDGE('',*,*,#28769,.T.) ;
#40528=ORIENTED_EDGE('',*,*,#28526,.F.) ;
#40529=ORIENTED_EDGE('',*,*,#28769,.F.) ;
#40530=ORIENTED_EDGE('',*,*,#28728,.F.) ;
#40531=ORIENTED_EDGE('',*,*,#28720,.F.) ;
#40532=ORIENTED_EDGE('',*,*,#28770,.F.) ;
#40533=ORIENTED_EDGE('',*,*,#28771,.F.) ;
#40534=ORIENTED_EDGE('',*,*,#28772,.T.) ;
#40535=ORIENTED_EDGE('',*,*,#28009,.T.) ;
#40536=ORIENTED_EDGE('',*,*,#28733,.F.) ;
#40537=ORIENTED_EDGE('',*,*,#28768,.T.) ;
#40538=ORIENTED_EDGE('',*,*,#28740,.T.) ;
#40539=ORIENTED_EDGE('',*,*,#27982,.F.) ;
#40540=ORIENTED_EDGE('',*,*,#28010,.T.) ;
#40541=ORIENTED_EDGE('',*,*,#28772,.F.) ;
#40542=ORIENTED_EDGE('',*,*,#28686,.T.) ;
#40543=ORIENTED_EDGE('',*,*,#28685,.F.) ;
#40544=ORIENTED_EDGE('',*,*,#27983,.F.) ;
#40545=ORIENTED_EDGE('',*,*,#28711,.F.) ;
#40546=ORIENTED_EDGE('',*,*,#27801,.T.) ;
#40547=ORIENTED_EDGE('',*,*,#27805,.F.) ;
#40548=ORIENTED_EDGE('',*,*,#28773,.F.) ;
#40549=ORIENTED_EDGE('',*,*,#28774,.F.) ;
#40550=ORIENTED_EDGE('',*,*,#28713,.F.) ;
#40551=ORIENTED_EDGE('',*,*,#28774,.T.) ;
#40552=ORIENTED_EDGE('',*,*,#28775,.T.) ;
#40553=ORIENTED_EDGE('',*,*,#28776,.T.) ;
#40554=ORIENTED_EDGE('',*,*,#28715,.F.) ;
#40555=ORIENTED_EDGE('',*,*,#28777,.T.) ;
#40556=ORIENTED_EDGE('',*,*,#28778,.T.) ;
#40557=ORIENTED_EDGE('',*,*,#28773,.T.) ;
#40558=ORIENTED_EDGE('',*,*,#27810,.T.) ;
#40559=ORIENTED_EDGE('',*,*,#27681,.F.) ;
#40560=ORIENTED_EDGE('',*,*,#27799,.F.) ;
#40561=ORIENTED_EDGE('',*,*,#28716,.F.) ;
#40562=ORIENTED_EDGE('',*,*,#27675,.F.) ;
#40563=ORIENTED_EDGE('',*,*,#27678,.F.) ;
#40564=ORIENTED_EDGE('',*,*,#28714,.F.) ;
#40565=ORIENTED_EDGE('',*,*,#28776,.F.) ;
#40566=ORIENTED_EDGE('',*,*,#28779,.F.) ;
#40567=ORIENTED_EDGE('',*,*,#28780,.T.) ;
#40568=ORIENTED_EDGE('',*,*,#27860,.T.) ;
#40569=ORIENTED_EDGE('',*,*,#28781,.F.) ;
#40570=ORIENTED_EDGE('',*,*,#27854,.T.) ;
#40571=ORIENTED_EDGE('',*,*,#28780,.F.) ;
#40572=ORIENTED_EDGE('',*,*,#28782,.F.) ;
#40573=ORIENTED_EDGE('',*,*,#27937,.F.) ;
#40574=ORIENTED_EDGE('',*,*,#27855,.T.) ;
#40575=ORIENTED_EDGE('',*,*,#28781,.T.) ;
#40576=ORIENTED_EDGE('',*,*,#28783,.T.) ;
#40577=ORIENTED_EDGE('',*,*,#27942,.F.) ;
#40578=ORIENTED_EDGE('',*,*,#28783,.F.) ;
#40579=ORIENTED_EDGE('',*,*,#28782,.T.) ;
#40580=ORIENTED_EDGE('',*,*,#28779,.T.) ;
#40581=ORIENTED_EDGE('',*,*,#28775,.F.) ;
#40582=ORIENTED_EDGE('',*,*,#28778,.F.) ;
#40583=ORIENTED_EDGE('',*,*,#28784,.F.) ;
#40584=ORIENTED_EDGE('',*,*,#28785,.F.) ;
#40585=ORIENTED_EDGE('',*,*,#27948,.F.) ;
#40586=ORIENTED_EDGE('',*,*,#27945,.F.) ;
#40587=ORIENTED_EDGE('',*,*,#28722,.T.) ;
#40588=ORIENTED_EDGE('',*,*,#28723,.T.) ;
#40589=ORIENTED_EDGE('',*,*,#27654,.T.) ;
#40590=ORIENTED_EDGE('',*,*,#27662,.F.) ;
#40591=ORIENTED_EDGE('',*,*,#28786,.F.) ;
#40592=ORIENTED_EDGE('',*,*,#28787,.T.) ;
#40593=ORIENTED_EDGE('',*,*,#27691,.T.) ;
#40594=ORIENTED_EDGE('',*,*,#27667,.T.) ;
#40595=ORIENTED_EDGE('',*,*,#27660,.T.) ;
#40596=ORIENTED_EDGE('',*,*,#28788,.T.) ;
#40597=ORIENTED_EDGE('',*,*,#28699,.T.) ;
#40598=ORIENTED_EDGE('',*,*,#28789,.F.) ;
#40599=ORIENTED_EDGE('',*,*,#28544,.F.) ;
#40600=ORIENTED_EDGE('',*,*,#27614,.T.) ;
#40601=ORIENTED_EDGE('',*,*,#28790,.T.) ;
#40602=ORIENTED_EDGE('',*,*,#28791,.T.) ;
#40603=ORIENTED_EDGE('',*,*,#28790,.F.) ;
#40604=ORIENTED_EDGE('',*,*,#27613,.F.) ;
#40605=ORIENTED_EDGE('',*,*,#28792,.F.) ;
#40606=ORIENTED_EDGE('',*,*,#28683,.F.) ;
#40607=ORIENTED_EDGE('',*,*,#28688,.F.) ;
#40608=ORIENTED_EDGE('',*,*,#28739,.F.) ;
#40609=ORIENTED_EDGE('',*,*,#28793,.T.) ;
#40610=ORIENTED_EDGE('',*,*,#28794,.T.) ;
#40611=ORIENTED_EDGE('',*,*,#28795,.F.) ;
#40612=ORIENTED_EDGE('',*,*,#28735,.F.) ;
#40613=ORIENTED_EDGE('',*,*,#28796,.F.) ;
#40614=ORIENTED_EDGE('',*,*,#28797,.F.) ;
#40615=ORIENTED_EDGE('',*,*,#27790,.T.) ;
#40616=ORIENTED_EDGE('',*,*,#27793,.T.) ;
#40617=ORIENTED_EDGE('',*,*,#28725,.F.) ;
#40618=ORIENTED_EDGE('',*,*,#28727,.F.) ;
#40619=ORIENTED_EDGE('',*,*,#28730,.F.) ;
#40620=ORIENTED_EDGE('',*,*,#28007,.F.) ;
#40621=ORIENTED_EDGE('',*,*,#28690,.F.) ;
#40622=ORIENTED_EDGE('',*,*,#28696,.T.) ;
#40623=ORIENTED_EDGE('',*,*,#28532,.F.) ;
#40624=ORIENTED_EDGE('',*,*,#28798,.T.) ;
#40625=ORIENTED_EDGE('',*,*,#28796,.T.) ;
#40626=ORIENTED_EDGE('',*,*,#28734,.T.) ;
#40627=ORIENTED_EDGE('',*,*,#28660,.F.) ;
#40628=ORIENTED_EDGE('',*,*,#28679,.F.) ;
#40629=ORIENTED_EDGE('',*,*,#28799,.F.) ;
#40630=ORIENTED_EDGE('',*,*,#28665,.F.) ;
#40631=ORIENTED_EDGE('',*,*,#28662,.F.) ;
#40632=ORIENTED_EDGE('',*,*,#27960,.F.) ;
#40633=ORIENTED_EDGE('',*,*,#28684,.T.) ;
#40634=ORIENTED_EDGE('',*,*,#28792,.T.) ;
#40635=ORIENTED_EDGE('',*,*,#27612,.T.) ;
#40636=ORIENTED_EDGE('',*,*,#28800,.F.) ;
#40637=ORIENTED_EDGE('',*,*,#28801,.F.) ;
#40638=ORIENTED_EDGE('',*,*,#28802,.F.) ;
#40639=ORIENTED_EDGE('',*,*,#28803,.T.) ;
#40640=ORIENTED_EDGE('',*,*,#28115,.F.) ;
#40641=ORIENTED_EDGE('',*,*,#28804,.F.) ;
#40642=ORIENTED_EDGE('',*,*,#28116,.F.) ;
#40643=ORIENTED_EDGE('',*,*,#28803,.F.) ;
#40644=ORIENTED_EDGE('',*,*,#28805,.F.) ;
#40645=ORIENTED_EDGE('',*,*,#28806,.F.) ;
#40646=ORIENTED_EDGE('',*,*,#28120,.F.) ;
#40647=ORIENTED_EDGE('',*,*,#28807,.F.) ;
#40648=ORIENTED_EDGE('',*,*,#28808,.T.) ;
#40649=ORIENTED_EDGE('',*,*,#28809,.T.) ;
#40650=ORIENTED_EDGE('',*,*,#28121,.F.) ;
#40651=ORIENTED_EDGE('',*,*,#28809,.F.) ;
#40652=ORIENTED_EDGE('',*,*,#28810,.T.) ;
#40653=ORIENTED_EDGE('',*,*,#28033,.F.) ;
#40654=ORIENTED_EDGE('',*,*,#28040,.F.) ;
#40655=ORIENTED_EDGE('',*,*,#28811,.F.) ;
#40656=ORIENTED_EDGE('',*,*,#28812,.F.) ;
#40657=ORIENTED_EDGE('',*,*,#28813,.F.) ;
#40658=ORIENTED_EDGE('',*,*,#28801,.T.) ;
#40659=ORIENTED_EDGE('',*,*,#28119,.F.) ;
#40660=ORIENTED_EDGE('',*,*,#28814,.F.) ;
#40661=ORIENTED_EDGE('',*,*,#28815,.F.) ;
#40662=ORIENTED_EDGE('',*,*,#28807,.T.) ;
#40663=ORIENTED_EDGE('',*,*,#28804,.T.) ;
#40664=ORIENTED_EDGE('',*,*,#28114,.F.) ;
#40665=ORIENTED_EDGE('',*,*,#28816,.F.) ;
#40666=ORIENTED_EDGE('',*,*,#28817,.T.) ;
#40667=ORIENTED_EDGE('',*,*,#28814,.T.) ;
#40668=ORIENTED_EDGE('',*,*,#28118,.T.) ;
#40669=ORIENTED_EDGE('',*,*,#28818,.T.) ;
#40670=ORIENTED_EDGE('',*,*,#28819,.T.) ;
#40671=ORIENTED_EDGE('',*,*,#28806,.T.) ;
#40672=ORIENTED_EDGE('',*,*,#28820,.T.) ;
#40673=ORIENTED_EDGE('',*,*,#28818,.F.) ;
#40674=ORIENTED_EDGE('',*,*,#28117,.F.) ;
#40675=ORIENTED_EDGE('',*,*,#28810,.F.) ;
#40676=ORIENTED_EDGE('',*,*,#28808,.F.) ;
#40677=ORIENTED_EDGE('',*,*,#28815,.T.) ;
#40678=ORIENTED_EDGE('',*,*,#28819,.F.) ;
#40679=ORIENTED_EDGE('',*,*,#28820,.F.) ;
#40680=ORIENTED_EDGE('',*,*,#28805,.T.) ;
#40681=ORIENTED_EDGE('',*,*,#28802,.T.) ;
#40682=ORIENTED_EDGE('',*,*,#28813,.T.) ;
#40683=ORIENTED_EDGE('',*,*,#28821,.F.) ;
#40684=ORIENTED_EDGE('',*,*,#28822,.F.) ;
#40685=ORIENTED_EDGE('',*,*,#28823,.F.) ;
#40686=ORIENTED_EDGE('',*,*,#28824,.F.) ;
#40687=ORIENTED_EDGE('',*,*,#28825,.F.) ;
#40688=ORIENTED_EDGE('',*,*,#28043,.F.) ;
#40689=ORIENTED_EDGE('',*,*,#28031,.F.) ;
#40690=ORIENTED_EDGE('',*,*,#28034,.F.) ;
#40691=ORIENTED_EDGE('',*,*,#28026,.T.) ;
#40692=ORIENTED_EDGE('',*,*,#28826,.T.) ;
#40693=ORIENTED_EDGE('',*,*,#28827,.T.) ;
#40694=ORIENTED_EDGE('',*,*,#28023,.T.) ;
#40695=ORIENTED_EDGE('',*,*,#28823,.T.) ;
#40696=ORIENTED_EDGE('',*,*,#28828,.T.) ;
#40697=ORIENTED_EDGE('',*,*,#27978,.T.) ;
#40698=ORIENTED_EDGE('',*,*,#28829,.T.) ;
#40699=ORIENTED_EDGE('',*,*,#28561,.T.) ;
#40700=ORIENTED_EDGE('',*,*,#28830,.T.) ;
#40701=ORIENTED_EDGE('',*,*,#28824,.T.) ;
#40702=ORIENTED_EDGE('',*,*,#28829,.F.) ;
#40703=ORIENTED_EDGE('',*,*,#28044,.T.) ;
#40704=ORIENTED_EDGE('',*,*,#28825,.T.) ;
#40705=ORIENTED_EDGE('',*,*,#28830,.F.) ;
#40706=ORIENTED_EDGE('',*,*,#28562,.T.) ;
#40707=ORIENTED_EDGE('',*,*,#28831,.T.) ;
#40708=ORIENTED_EDGE('',*,*,#27974,.T.) ;
#40709=ORIENTED_EDGE('',*,*,#28828,.F.) ;
#40710=ORIENTED_EDGE('',*,*,#28822,.T.) ;
#40711=ORIENTED_EDGE('',*,*,#28832,.F.) ;
#40712=ORIENTED_EDGE('',*,*,#27975,.T.) ;
#40713=ORIENTED_EDGE('',*,*,#28831,.F.) ;
#40714=ORIENTED_EDGE('',*,*,#28821,.T.) ;
#40715=ORIENTED_EDGE('',*,*,#28812,.T.) ;
#40716=ORIENTED_EDGE('',*,*,#28445,.F.) ;
#40717=ORIENTED_EDGE('',*,*,#28833,.F.) ;
#40718=ORIENTED_EDGE('',*,*,#28834,.F.) ;
#40719=ORIENTED_EDGE('',*,*,#28835,.F.) ;
#40720=ORIENTED_EDGE('',*,*,#28451,.F.) ;
#40721=ORIENTED_EDGE('',*,*,#28836,.F.) ;
#40722=ORIENTED_EDGE('',*,*,#28837,.F.) ;
#40723=ORIENTED_EDGE('',*,*,#28838,.F.) ;
#40724=ORIENTED_EDGE('',*,*,#28839,.F.) ;
#40725=ORIENTED_EDGE('',*,*,#28837,.T.) ;
#40726=ORIENTED_EDGE('',*,*,#28840,.F.) ;
#40727=ORIENTED_EDGE('',*,*,#28834,.T.) ;
#40728=ORIENTED_EDGE('',*,*,#28475,.F.) ;
#40729=ORIENTED_EDGE('',*,*,#28841,.T.) ;
#40730=ORIENTED_EDGE('',*,*,#28485,.F.) ;
#40731=ORIENTED_EDGE('',*,*,#28482,.F.) ;
#40732=ORIENTED_EDGE('',*,*,#28479,.F.) ;
#40733=ORIENTED_EDGE('',*,*,#28838,.T.) ;
#40734=ORIENTED_EDGE('',*,*,#28839,.T.) ;
#40735=ORIENTED_EDGE('',*,*,#28833,.T.) ;
#40736=ORIENTED_EDGE('',*,*,#28444,.F.) ;
#40737=ORIENTED_EDGE('',*,*,#28448,.T.) ;
#40738=ORIENTED_EDGE('',*,*,#28449,.F.) ;
#40739=ORIENTED_EDGE('',*,*,#28472,.F.) ;
#40740=ORIENTED_EDGE('',*,*,#28842,.T.) ;
#40741=ORIENTED_EDGE('',*,*,#28476,.F.) ;
#40742=ORIENTED_EDGE('',*,*,#28461,.F.) ;
#40743=ORIENTED_EDGE('',*,*,#28465,.F.) ;
#40744=ORIENTED_EDGE('',*,*,#28843,.T.) ;
#40745=ORIENTED_EDGE('',*,*,#28473,.F.) ;
#40746=ORIENTED_EDGE('',*,*,#28470,.F.) ;
#40747=ORIENTED_EDGE('',*,*,#28468,.F.) ;
#40748=ORIENTED_EDGE('',*,*,#28836,.T.) ;
#40749=ORIENTED_EDGE('',*,*,#28450,.F.) ;
#40750=ORIENTED_EDGE('',*,*,#28446,.T.) ;
#40751=ORIENTED_EDGE('',*,*,#28442,.F.) ;
#40752=ORIENTED_EDGE('',*,*,#28835,.T.) ;
#40753=ORIENTED_EDGE('',*,*,#28840,.T.) ;
#40754=ORIENTED_EDGE('',*,*,#28471,.T.) ;
#40755=ORIENTED_EDGE('',*,*,#28843,.F.) ;
#40756=ORIENTED_EDGE('',*,*,#28464,.F.) ;
#40757=ORIENTED_EDGE('',*,*,#28507,.F.) ;
#40758=ORIENTED_EDGE('',*,*,#28483,.F.) ;
#40759=ORIENTED_EDGE('',*,*,#28841,.F.) ;
#40760=ORIENTED_EDGE('',*,*,#28474,.T.) ;
#40761=ORIENTED_EDGE('',*,*,#28842,.F.) ;
#40762=ORIENTED_EDGE('',*,*,#28844,.T.) ;
#40763=ORIENTED_EDGE('',*,*,#28845,.T.) ;
#40764=ORIENTED_EDGE('',*,*,#28846,.T.) ;
#40765=ORIENTED_EDGE('',*,*,#28847,.F.) ;
#40766=ORIENTED_EDGE('',*,*,#28848,.T.) ;
#40767=ORIENTED_EDGE('',*,*,#28849,.T.) ;
#40768=ORIENTED_EDGE('',*,*,#28850,.T.) ;
#40769=ORIENTED_EDGE('',*,*,#28845,.F.) ;
#40770=ORIENTED_EDGE('',*,*,#28851,.T.) ;
#40771=ORIENTED_EDGE('',*,*,#28852,.T.) ;
#40772=ORIENTED_EDGE('',*,*,#28853,.T.) ;
#40773=ORIENTED_EDGE('',*,*,#28849,.F.) ;
#40774=ORIENTED_EDGE('',*,*,#28854,.T.) ;
#40775=ORIENTED_EDGE('',*,*,#28852,.F.) ;
#40776=ORIENTED_EDGE('',*,*,#28855,.T.) ;
#40777=ORIENTED_EDGE('',*,*,#28856,.T.) ;
#40778=ORIENTED_EDGE('',*,*,#28857,.T.) ;
#40779=ORIENTED_EDGE('',*,*,#28856,.F.) ;
#40780=ORIENTED_EDGE('',*,*,#28858,.T.) ;
#40781=ORIENTED_EDGE('',*,*,#28859,.T.) ;
#40782=ORIENTED_EDGE('',*,*,#28860,.T.) ;
#40783=ORIENTED_EDGE('',*,*,#28859,.F.) ;
#40784=ORIENTED_EDGE('',*,*,#28861,.T.) ;
#40785=ORIENTED_EDGE('',*,*,#28862,.T.) ;
#40786=ORIENTED_EDGE('',*,*,#28863,.T.) ;
#40787=ORIENTED_EDGE('',*,*,#28862,.F.) ;
#40788=ORIENTED_EDGE('',*,*,#28864,.T.) ;
#40789=ORIENTED_EDGE('',*,*,#28847,.T.) ;
#40790=ORIENTED_EDGE('',*,*,#28857,.F.) ;
#40791=ORIENTED_EDGE('',*,*,#28865,.F.) ;
#40792=ORIENTED_EDGE('',*,*,#28866,.F.) ;
#40793=ORIENTED_EDGE('',*,*,#28867,.T.) ;
#40794=ORIENTED_EDGE('',*,*,#28860,.F.) ;
#40795=ORIENTED_EDGE('',*,*,#28868,.F.) ;
#40796=ORIENTED_EDGE('',*,*,#28869,.F.) ;
#40797=ORIENTED_EDGE('',*,*,#28865,.T.) ;
#40798=ORIENTED_EDGE('',*,*,#28863,.F.) ;
#40799=ORIENTED_EDGE('',*,*,#28870,.F.) ;
#40800=ORIENTED_EDGE('',*,*,#28871,.F.) ;
#40801=ORIENTED_EDGE('',*,*,#28868,.T.) ;
#40802=ORIENTED_EDGE('',*,*,#28846,.F.) ;
#40803=ORIENTED_EDGE('',*,*,#28872,.F.) ;
#40804=ORIENTED_EDGE('',*,*,#28873,.F.) ;
#40805=ORIENTED_EDGE('',*,*,#28870,.T.) ;
#40806=ORIENTED_EDGE('',*,*,#28844,.F.) ;
#40807=ORIENTED_EDGE('',*,*,#28864,.F.) ;
#40808=ORIENTED_EDGE('',*,*,#28861,.F.) ;
#40809=ORIENTED_EDGE('',*,*,#28858,.F.) ;
#40810=ORIENTED_EDGE('',*,*,#28855,.F.) ;
#40811=ORIENTED_EDGE('',*,*,#28851,.F.) ;
#40812=ORIENTED_EDGE('',*,*,#28848,.F.) ;
#40813=ORIENTED_EDGE('',*,*,#28874,.T.) ;
#40814=ORIENTED_EDGE('',*,*,#28875,.T.) ;
#40815=ORIENTED_EDGE('',*,*,#28876,.T.) ;
#40816=ORIENTED_EDGE('',*,*,#28877,.F.) ;
#40817=ORIENTED_EDGE('',*,*,#28878,.T.) ;
#40818=ORIENTED_EDGE('',*,*,#28879,.T.) ;
#40819=ORIENTED_EDGE('',*,*,#28880,.T.) ;
#40820=ORIENTED_EDGE('',*,*,#28875,.F.) ;
#40821=ORIENTED_EDGE('',*,*,#28881,.T.) ;
#40822=ORIENTED_EDGE('',*,*,#28882,.T.) ;
#40823=ORIENTED_EDGE('',*,*,#28883,.T.) ;
#40824=ORIENTED_EDGE('',*,*,#28879,.F.) ;
#40825=ORIENTED_EDGE('',*,*,#28884,.T.) ;
#40826=ORIENTED_EDGE('',*,*,#28882,.F.) ;
#40827=ORIENTED_EDGE('',*,*,#28885,.T.) ;
#40828=ORIENTED_EDGE('',*,*,#28886,.T.) ;
#40829=ORIENTED_EDGE('',*,*,#28887,.T.) ;
#40830=ORIENTED_EDGE('',*,*,#28886,.F.) ;
#40831=ORIENTED_EDGE('',*,*,#28888,.T.) ;
#40832=ORIENTED_EDGE('',*,*,#28889,.T.) ;
#40833=ORIENTED_EDGE('',*,*,#28890,.T.) ;
#40834=ORIENTED_EDGE('',*,*,#28889,.F.) ;
#40835=ORIENTED_EDGE('',*,*,#28891,.T.) ;
#40836=ORIENTED_EDGE('',*,*,#28892,.T.) ;
#40837=ORIENTED_EDGE('',*,*,#28893,.T.) ;
#40838=ORIENTED_EDGE('',*,*,#28892,.F.) ;
#40839=ORIENTED_EDGE('',*,*,#28894,.T.) ;
#40840=ORIENTED_EDGE('',*,*,#28877,.T.) ;
#40841=ORIENTED_EDGE('',*,*,#28887,.F.) ;
#40842=ORIENTED_EDGE('',*,*,#28895,.F.) ;
#40843=ORIENTED_EDGE('',*,*,#28896,.F.) ;
#40844=ORIENTED_EDGE('',*,*,#28897,.T.) ;
#40845=ORIENTED_EDGE('',*,*,#28890,.F.) ;
#40846=ORIENTED_EDGE('',*,*,#28898,.F.) ;
#40847=ORIENTED_EDGE('',*,*,#28899,.F.) ;
#40848=ORIENTED_EDGE('',*,*,#28895,.T.) ;
#40849=ORIENTED_EDGE('',*,*,#28893,.F.) ;
#40850=ORIENTED_EDGE('',*,*,#28900,.F.) ;
#40851=ORIENTED_EDGE('',*,*,#28901,.F.) ;
#40852=ORIENTED_EDGE('',*,*,#28898,.T.) ;
#40853=ORIENTED_EDGE('',*,*,#28876,.F.) ;
#40854=ORIENTED_EDGE('',*,*,#28902,.F.) ;
#40855=ORIENTED_EDGE('',*,*,#28903,.F.) ;
#40856=ORIENTED_EDGE('',*,*,#28900,.T.) ;
#40857=ORIENTED_EDGE('',*,*,#28874,.F.) ;
#40858=ORIENTED_EDGE('',*,*,#28894,.F.) ;
#40859=ORIENTED_EDGE('',*,*,#28891,.F.) ;
#40860=ORIENTED_EDGE('',*,*,#28888,.F.) ;
#40861=ORIENTED_EDGE('',*,*,#28885,.F.) ;
#40862=ORIENTED_EDGE('',*,*,#28881,.F.) ;
#40863=ORIENTED_EDGE('',*,*,#28878,.F.) ;
#40864=ORIENTED_EDGE('',*,*,#28904,.T.) ;
#40865=ORIENTED_EDGE('',*,*,#28905,.T.) ;
#40866=ORIENTED_EDGE('',*,*,#28906,.T.) ;
#40867=ORIENTED_EDGE('',*,*,#28907,.F.) ;
#40868=ORIENTED_EDGE('',*,*,#28908,.T.) ;
#40869=ORIENTED_EDGE('',*,*,#28909,.T.) ;
#40870=ORIENTED_EDGE('',*,*,#28910,.T.) ;
#40871=ORIENTED_EDGE('',*,*,#28905,.F.) ;
#40872=ORIENTED_EDGE('',*,*,#28911,.T.) ;
#40873=ORIENTED_EDGE('',*,*,#28912,.T.) ;
#40874=ORIENTED_EDGE('',*,*,#28913,.T.) ;
#40875=ORIENTED_EDGE('',*,*,#28909,.F.) ;
#40876=ORIENTED_EDGE('',*,*,#28914,.T.) ;
#40877=ORIENTED_EDGE('',*,*,#28912,.F.) ;
#40878=ORIENTED_EDGE('',*,*,#28915,.T.) ;
#40879=ORIENTED_EDGE('',*,*,#28916,.T.) ;
#40880=ORIENTED_EDGE('',*,*,#28917,.T.) ;
#40881=ORIENTED_EDGE('',*,*,#28916,.F.) ;
#40882=ORIENTED_EDGE('',*,*,#28918,.T.) ;
#40883=ORIENTED_EDGE('',*,*,#28919,.T.) ;
#40884=ORIENTED_EDGE('',*,*,#28920,.T.) ;
#40885=ORIENTED_EDGE('',*,*,#28919,.F.) ;
#40886=ORIENTED_EDGE('',*,*,#28921,.T.) ;
#40887=ORIENTED_EDGE('',*,*,#28922,.T.) ;
#40888=ORIENTED_EDGE('',*,*,#28923,.T.) ;
#40889=ORIENTED_EDGE('',*,*,#28922,.F.) ;
#40890=ORIENTED_EDGE('',*,*,#28924,.T.) ;
#40891=ORIENTED_EDGE('',*,*,#28907,.T.) ;
#40892=ORIENTED_EDGE('',*,*,#28917,.F.) ;
#40893=ORIENTED_EDGE('',*,*,#28925,.F.) ;
#40894=ORIENTED_EDGE('',*,*,#28926,.F.) ;
#40895=ORIENTED_EDGE('',*,*,#28927,.T.) ;
#40896=ORIENTED_EDGE('',*,*,#28920,.F.) ;
#40897=ORIENTED_EDGE('',*,*,#28928,.F.) ;
#40898=ORIENTED_EDGE('',*,*,#28929,.F.) ;
#40899=ORIENTED_EDGE('',*,*,#28925,.T.) ;
#40900=ORIENTED_EDGE('',*,*,#28923,.F.) ;
#40901=ORIENTED_EDGE('',*,*,#28930,.F.) ;
#40902=ORIENTED_EDGE('',*,*,#28931,.F.) ;
#40903=ORIENTED_EDGE('',*,*,#28928,.T.) ;
#40904=ORIENTED_EDGE('',*,*,#28906,.F.) ;
#40905=ORIENTED_EDGE('',*,*,#28932,.F.) ;
#40906=ORIENTED_EDGE('',*,*,#28933,.F.) ;
#40907=ORIENTED_EDGE('',*,*,#28930,.T.) ;
#40908=ORIENTED_EDGE('',*,*,#28904,.F.) ;
#40909=ORIENTED_EDGE('',*,*,#28924,.F.) ;
#40910=ORIENTED_EDGE('',*,*,#28921,.F.) ;
#40911=ORIENTED_EDGE('',*,*,#28918,.F.) ;
#40912=ORIENTED_EDGE('',*,*,#28915,.F.) ;
#40913=ORIENTED_EDGE('',*,*,#28911,.F.) ;
#40914=ORIENTED_EDGE('',*,*,#28908,.F.) ;
#40915=ORIENTED_EDGE('',*,*,#28934,.T.) ;
#40916=ORIENTED_EDGE('',*,*,#28935,.T.) ;
#40917=ORIENTED_EDGE('',*,*,#28936,.T.) ;
#40918=ORIENTED_EDGE('',*,*,#28937,.F.) ;
#40919=ORIENTED_EDGE('',*,*,#28938,.T.) ;
#40920=ORIENTED_EDGE('',*,*,#28935,.F.) ;
#40921=ORIENTED_EDGE('',*,*,#28939,.T.) ;
#40922=ORIENTED_EDGE('',*,*,#28940,.T.) ;
#40923=ORIENTED_EDGE('',*,*,#28941,.T.) ;
#40924=ORIENTED_EDGE('',*,*,#28940,.F.) ;
#40925=ORIENTED_EDGE('',*,*,#28942,.T.) ;
#40926=ORIENTED_EDGE('',*,*,#28943,.T.) ;
#40927=ORIENTED_EDGE('',*,*,#28944,.T.) ;
#40928=ORIENTED_EDGE('',*,*,#28943,.F.) ;
#40929=ORIENTED_EDGE('',*,*,#28945,.T.) ;
#40930=ORIENTED_EDGE('',*,*,#28937,.T.) ;
#40931=ORIENTED_EDGE('',*,*,#28944,.F.) ;
#40932=ORIENTED_EDGE('',*,*,#28946,.F.) ;
#40933=ORIENTED_EDGE('',*,*,#28947,.F.) ;
#40934=ORIENTED_EDGE('',*,*,#28948,.T.) ;
#40935=ORIENTED_EDGE('',*,*,#28936,.F.) ;
#40936=ORIENTED_EDGE('',*,*,#28949,.F.) ;
#40937=ORIENTED_EDGE('',*,*,#28950,.F.) ;
#40938=ORIENTED_EDGE('',*,*,#28946,.T.) ;
#40939=ORIENTED_EDGE('',*,*,#28934,.F.) ;
#40940=ORIENTED_EDGE('',*,*,#28945,.F.) ;
#40941=ORIENTED_EDGE('',*,*,#28942,.F.) ;
#40942=ORIENTED_EDGE('',*,*,#28939,.F.) ;
#40943=ORIENTED_EDGE('',*,*,#28951,.T.) ;
#40944=ORIENTED_EDGE('',*,*,#28952,.T.) ;
#40945=ORIENTED_EDGE('',*,*,#28953,.T.) ;
#40946=ORIENTED_EDGE('',*,*,#28954,.F.) ;
#40947=ORIENTED_EDGE('',*,*,#28955,.T.) ;
#40948=ORIENTED_EDGE('',*,*,#28956,.T.) ;
#40949=ORIENTED_EDGE('',*,*,#28957,.T.) ;
#40950=ORIENTED_EDGE('',*,*,#28952,.F.) ;
#40951=ORIENTED_EDGE('',*,*,#28958,.T.) ;
#40952=ORIENTED_EDGE('',*,*,#28959,.T.) ;
#40953=ORIENTED_EDGE('',*,*,#28960,.T.) ;
#40954=ORIENTED_EDGE('',*,*,#28956,.F.) ;
#40955=ORIENTED_EDGE('',*,*,#28961,.T.) ;
#40956=ORIENTED_EDGE('',*,*,#28959,.F.) ;
#40957=ORIENTED_EDGE('',*,*,#28962,.T.) ;
#40958=ORIENTED_EDGE('',*,*,#28963,.T.) ;
#40959=ORIENTED_EDGE('',*,*,#28964,.T.) ;
#40960=ORIENTED_EDGE('',*,*,#28963,.F.) ;
#40961=ORIENTED_EDGE('',*,*,#28965,.T.) ;
#40962=ORIENTED_EDGE('',*,*,#28966,.T.) ;
#40963=ORIENTED_EDGE('',*,*,#28967,.T.) ;
#40964=ORIENTED_EDGE('',*,*,#28966,.F.) ;
#40965=ORIENTED_EDGE('',*,*,#28968,.T.) ;
#40966=ORIENTED_EDGE('',*,*,#28969,.T.) ;
#40967=ORIENTED_EDGE('',*,*,#28970,.T.) ;
#40968=ORIENTED_EDGE('',*,*,#28969,.F.) ;
#40969=ORIENTED_EDGE('',*,*,#28971,.T.) ;
#40970=ORIENTED_EDGE('',*,*,#28954,.T.) ;
#40971=ORIENTED_EDGE('',*,*,#28964,.F.) ;
#40972=ORIENTED_EDGE('',*,*,#28972,.F.) ;
#40973=ORIENTED_EDGE('',*,*,#28973,.F.) ;
#40974=ORIENTED_EDGE('',*,*,#28974,.T.) ;
#40975=ORIENTED_EDGE('',*,*,#28967,.F.) ;
#40976=ORIENTED_EDGE('',*,*,#28975,.F.) ;
#40977=ORIENTED_EDGE('',*,*,#28976,.F.) ;
#40978=ORIENTED_EDGE('',*,*,#28972,.T.) ;
#40979=ORIENTED_EDGE('',*,*,#28970,.F.) ;
#40980=ORIENTED_EDGE('',*,*,#28977,.F.) ;
#40981=ORIENTED_EDGE('',*,*,#28978,.F.) ;
#40982=ORIENTED_EDGE('',*,*,#28975,.T.) ;
#40983=ORIENTED_EDGE('',*,*,#28953,.F.) ;
#40984=ORIENTED_EDGE('',*,*,#28979,.F.) ;
#40985=ORIENTED_EDGE('',*,*,#28980,.F.) ;
#40986=ORIENTED_EDGE('',*,*,#28977,.T.) ;
#40987=ORIENTED_EDGE('',*,*,#28951,.F.) ;
#40988=ORIENTED_EDGE('',*,*,#28971,.F.) ;
#40989=ORIENTED_EDGE('',*,*,#28968,.F.) ;
#40990=ORIENTED_EDGE('',*,*,#28965,.F.) ;
#40991=ORIENTED_EDGE('',*,*,#28962,.F.) ;
#40992=ORIENTED_EDGE('',*,*,#28958,.F.) ;
#40993=ORIENTED_EDGE('',*,*,#28955,.F.) ;
#40994=ORIENTED_EDGE('',*,*,#28981,.T.) ;
#40995=ORIENTED_EDGE('',*,*,#28982,.T.) ;
#40996=ORIENTED_EDGE('',*,*,#28983,.T.) ;
#40997=ORIENTED_EDGE('',*,*,#28984,.F.) ;
#40998=ORIENTED_EDGE('',*,*,#28985,.T.) ;
#40999=ORIENTED_EDGE('',*,*,#28982,.F.) ;
#41000=ORIENTED_EDGE('',*,*,#28986,.T.) ;
#41001=ORIENTED_EDGE('',*,*,#28987,.T.) ;
#41002=ORIENTED_EDGE('',*,*,#28988,.T.) ;
#41003=ORIENTED_EDGE('',*,*,#28987,.F.) ;
#41004=ORIENTED_EDGE('',*,*,#28989,.T.) ;
#41005=ORIENTED_EDGE('',*,*,#28990,.T.) ;
#41006=ORIENTED_EDGE('',*,*,#28991,.T.) ;
#41007=ORIENTED_EDGE('',*,*,#28990,.F.) ;
#41008=ORIENTED_EDGE('',*,*,#28992,.T.) ;
#41009=ORIENTED_EDGE('',*,*,#28984,.T.) ;
#41010=ORIENTED_EDGE('',*,*,#28991,.F.) ;
#41011=ORIENTED_EDGE('',*,*,#28993,.F.) ;
#41012=ORIENTED_EDGE('',*,*,#28994,.F.) ;
#41013=ORIENTED_EDGE('',*,*,#28995,.T.) ;
#41014=ORIENTED_EDGE('',*,*,#28983,.F.) ;
#41015=ORIENTED_EDGE('',*,*,#28996,.F.) ;
#41016=ORIENTED_EDGE('',*,*,#28997,.F.) ;
#41017=ORIENTED_EDGE('',*,*,#28993,.T.) ;
#41018=ORIENTED_EDGE('',*,*,#28981,.F.) ;
#41019=ORIENTED_EDGE('',*,*,#28992,.F.) ;
#41020=ORIENTED_EDGE('',*,*,#28989,.F.) ;
#41021=ORIENTED_EDGE('',*,*,#28986,.F.) ;
#41022=ORIENTED_EDGE('',*,*,#28998,.T.) ;
#41023=ORIENTED_EDGE('',*,*,#28999,.T.) ;
#41024=ORIENTED_EDGE('',*,*,#29000,.T.) ;
#41025=ORIENTED_EDGE('',*,*,#29001,.F.) ;
#41026=ORIENTED_EDGE('',*,*,#29002,.T.) ;
#41027=ORIENTED_EDGE('',*,*,#29003,.T.) ;
#41028=ORIENTED_EDGE('',*,*,#29004,.T.) ;
#41029=ORIENTED_EDGE('',*,*,#28999,.F.) ;
#41030=ORIENTED_EDGE('',*,*,#29005,.T.) ;
#41031=ORIENTED_EDGE('',*,*,#29006,.T.) ;
#41032=ORIENTED_EDGE('',*,*,#29007,.T.) ;
#41033=ORIENTED_EDGE('',*,*,#29003,.F.) ;
#41034=ORIENTED_EDGE('',*,*,#29008,.T.) ;
#41035=ORIENTED_EDGE('',*,*,#29009,.T.) ;
#41036=ORIENTED_EDGE('',*,*,#29006,.F.) ;
#41037=ORIENTED_EDGE('',*,*,#29010,.T.) ;
#41038=ORIENTED_EDGE('',*,*,#29011,.T.) ;
#41039=ORIENTED_EDGE('',*,*,#29008,.F.) ;
#41040=ORIENTED_EDGE('',*,*,#29012,.T.) ;
#41041=ORIENTED_EDGE('',*,*,#29013,.T.) ;
#41042=ORIENTED_EDGE('',*,*,#29014,.T.) ;
#41043=ORIENTED_EDGE('',*,*,#29013,.F.) ;
#41044=ORIENTED_EDGE('',*,*,#29015,.T.) ;
#41045=ORIENTED_EDGE('',*,*,#29016,.T.) ;
#41046=ORIENTED_EDGE('',*,*,#29017,.T.) ;
#41047=ORIENTED_EDGE('',*,*,#29018,.T.) ;
#41048=ORIENTED_EDGE('',*,*,#29019,.T.) ;
#41049=ORIENTED_EDGE('',*,*,#29016,.F.) ;
#41050=ORIENTED_EDGE('',*,*,#29020,.T.) ;
#41051=ORIENTED_EDGE('',*,*,#29021,.T.) ;
#41052=ORIENTED_EDGE('',*,*,#29018,.F.) ;
#41053=ORIENTED_EDGE('',*,*,#29022,.T.) ;
#41054=ORIENTED_EDGE('',*,*,#29023,.T.) ;
#41055=ORIENTED_EDGE('',*,*,#29020,.F.) ;
#41056=ORIENTED_EDGE('',*,*,#29024,.T.) ;
#41057=ORIENTED_EDGE('',*,*,#29025,.T.) ;
#41058=ORIENTED_EDGE('',*,*,#29026,.T.) ;
#41059=ORIENTED_EDGE('',*,*,#29025,.F.) ;
#41060=ORIENTED_EDGE('',*,*,#29027,.T.) ;
#41061=ORIENTED_EDGE('',*,*,#29028,.T.) ;
#41062=ORIENTED_EDGE('',*,*,#29029,.T.) ;
#41063=ORIENTED_EDGE('',*,*,#29028,.F.) ;
#41064=ORIENTED_EDGE('',*,*,#29030,.T.) ;
#41065=ORIENTED_EDGE('',*,*,#29001,.T.) ;
#41066=ORIENTED_EDGE('',*,*,#29019,.F.) ;
#41067=ORIENTED_EDGE('',*,*,#29031,.F.) ;
#41068=ORIENTED_EDGE('',*,*,#29032,.F.) ;
#41069=ORIENTED_EDGE('',*,*,#29033,.T.) ;
#41070=ORIENTED_EDGE('',*,*,#29021,.F.) ;
#41071=ORIENTED_EDGE('',*,*,#29034,.F.) ;
#41072=ORIENTED_EDGE('',*,*,#29035,.F.) ;
#41073=ORIENTED_EDGE('',*,*,#29031,.T.) ;
#41074=ORIENTED_EDGE('',*,*,#29023,.F.) ;
#41075=ORIENTED_EDGE('',*,*,#29036,.F.) ;
#41076=ORIENTED_EDGE('',*,*,#29037,.F.) ;
#41077=ORIENTED_EDGE('',*,*,#29034,.T.) ;
#41078=ORIENTED_EDGE('',*,*,#29026,.F.) ;
#41079=ORIENTED_EDGE('',*,*,#29038,.F.) ;
#41080=ORIENTED_EDGE('',*,*,#29039,.F.) ;
#41081=ORIENTED_EDGE('',*,*,#29036,.T.) ;
#41082=ORIENTED_EDGE('',*,*,#29029,.F.) ;
#41083=ORIENTED_EDGE('',*,*,#29040,.F.) ;
#41084=ORIENTED_EDGE('',*,*,#29041,.F.) ;
#41085=ORIENTED_EDGE('',*,*,#29038,.T.) ;
#41086=ORIENTED_EDGE('',*,*,#29000,.F.) ;
#41087=ORIENTED_EDGE('',*,*,#29042,.F.) ;
#41088=ORIENTED_EDGE('',*,*,#29043,.F.) ;
#41089=ORIENTED_EDGE('',*,*,#29040,.T.) ;
#41090=ORIENTED_EDGE('',*,*,#28998,.F.) ;
#41091=ORIENTED_EDGE('',*,*,#29030,.F.) ;
#41092=ORIENTED_EDGE('',*,*,#29027,.F.) ;
#41093=ORIENTED_EDGE('',*,*,#29024,.F.) ;
#41094=ORIENTED_EDGE('',*,*,#29022,.F.) ;
#41095=ORIENTED_EDGE('',*,*,#29017,.F.) ;
#41096=ORIENTED_EDGE('',*,*,#29015,.F.) ;
#41097=ORIENTED_EDGE('',*,*,#29012,.F.) ;
#41098=ORIENTED_EDGE('',*,*,#29010,.F.) ;
#41099=ORIENTED_EDGE('',*,*,#29005,.F.) ;
#41100=ORIENTED_EDGE('',*,*,#29002,.F.) ;
#41101=ORIENTED_EDGE('',*,*,#29044,.T.) ;
#41102=ORIENTED_EDGE('',*,*,#29045,.T.) ;
#41103=ORIENTED_EDGE('',*,*,#29046,.T.) ;
#41104=ORIENTED_EDGE('',*,*,#29047,.F.) ;
#41105=ORIENTED_EDGE('',*,*,#29048,.T.) ;
#41106=ORIENTED_EDGE('',*,*,#29049,.T.) ;
#41107=ORIENTED_EDGE('',*,*,#29050,.T.) ;
#41108=ORIENTED_EDGE('',*,*,#29045,.F.) ;
#41109=ORIENTED_EDGE('',*,*,#29051,.T.) ;
#41110=ORIENTED_EDGE('',*,*,#29052,.T.) ;
#41111=ORIENTED_EDGE('',*,*,#29049,.F.) ;
#41112=ORIENTED_EDGE('',*,*,#29053,.T.) ;
#41113=ORIENTED_EDGE('',*,*,#29054,.T.) ;
#41114=ORIENTED_EDGE('',*,*,#29051,.F.) ;
#41115=ORIENTED_EDGE('',*,*,#29055,.T.) ;
#41116=ORIENTED_EDGE('',*,*,#29056,.T.) ;
#41117=ORIENTED_EDGE('',*,*,#29057,.T.) ;
#41118=ORIENTED_EDGE('',*,*,#29058,.T.) ;
#41119=ORIENTED_EDGE('',*,*,#29059,.T.) ;
#41120=ORIENTED_EDGE('',*,*,#29056,.F.) ;
#41121=ORIENTED_EDGE('',*,*,#29060,.T.) ;
#41122=ORIENTED_EDGE('',*,*,#29061,.T.) ;
#41123=ORIENTED_EDGE('',*,*,#29062,.T.) ;
#41124=ORIENTED_EDGE('',*,*,#29058,.F.) ;
#41125=ORIENTED_EDGE('',*,*,#29063,.T.) ;
#41126=ORIENTED_EDGE('',*,*,#29064,.T.) ;
#41127=ORIENTED_EDGE('',*,*,#29061,.F.) ;
#41128=ORIENTED_EDGE('',*,*,#29065,.T.) ;
#41129=ORIENTED_EDGE('',*,*,#29066,.T.) ;
#41130=ORIENTED_EDGE('',*,*,#29063,.F.) ;
#41131=ORIENTED_EDGE('',*,*,#29067,.T.) ;
#41132=ORIENTED_EDGE('',*,*,#29068,.T.) ;
#41133=ORIENTED_EDGE('',*,*,#29069,.T.) ;
#41134=ORIENTED_EDGE('',*,*,#29068,.F.) ;
#41135=ORIENTED_EDGE('',*,*,#29070,.T.) ;
#41136=ORIENTED_EDGE('',*,*,#29071,.T.) ;
#41137=ORIENTED_EDGE('',*,*,#29072,.T.) ;
#41138=ORIENTED_EDGE('',*,*,#29071,.F.) ;
#41139=ORIENTED_EDGE('',*,*,#29073,.T.) ;
#41140=ORIENTED_EDGE('',*,*,#29074,.T.) ;
#41141=ORIENTED_EDGE('',*,*,#29075,.T.) ;
#41142=ORIENTED_EDGE('',*,*,#29074,.F.) ;
#41143=ORIENTED_EDGE('',*,*,#29076,.T.) ;
#41144=ORIENTED_EDGE('',*,*,#29047,.T.) ;
#41145=ORIENTED_EDGE('',*,*,#29064,.F.) ;
#41146=ORIENTED_EDGE('',*,*,#29077,.F.) ;
#41147=ORIENTED_EDGE('',*,*,#29078,.F.) ;
#41148=ORIENTED_EDGE('',*,*,#29079,.T.) ;
#41149=ORIENTED_EDGE('',*,*,#29066,.F.) ;
#41150=ORIENTED_EDGE('',*,*,#29080,.F.) ;
#41151=ORIENTED_EDGE('',*,*,#29081,.F.) ;
#41152=ORIENTED_EDGE('',*,*,#29077,.T.) ;
#41153=ORIENTED_EDGE('',*,*,#29069,.F.) ;
#41154=ORIENTED_EDGE('',*,*,#29082,.F.) ;
#41155=ORIENTED_EDGE('',*,*,#29083,.F.) ;
#41156=ORIENTED_EDGE('',*,*,#29080,.T.) ;
#41157=ORIENTED_EDGE('',*,*,#29072,.F.) ;
#41158=ORIENTED_EDGE('',*,*,#29084,.F.) ;
#41159=ORIENTED_EDGE('',*,*,#29085,.F.) ;
#41160=ORIENTED_EDGE('',*,*,#29082,.T.) ;
#41161=ORIENTED_EDGE('',*,*,#29075,.F.) ;
#41162=ORIENTED_EDGE('',*,*,#29086,.F.) ;
#41163=ORIENTED_EDGE('',*,*,#29087,.F.) ;
#41164=ORIENTED_EDGE('',*,*,#29084,.T.) ;
#41165=ORIENTED_EDGE('',*,*,#29046,.F.) ;
#41166=ORIENTED_EDGE('',*,*,#29088,.F.) ;
#41167=ORIENTED_EDGE('',*,*,#29089,.F.) ;
#41168=ORIENTED_EDGE('',*,*,#29086,.T.) ;
#41169=ORIENTED_EDGE('',*,*,#29044,.F.) ;
#41170=ORIENTED_EDGE('',*,*,#29076,.F.) ;
#41171=ORIENTED_EDGE('',*,*,#29073,.F.) ;
#41172=ORIENTED_EDGE('',*,*,#29070,.F.) ;
#41173=ORIENTED_EDGE('',*,*,#29067,.F.) ;
#41174=ORIENTED_EDGE('',*,*,#29065,.F.) ;
#41175=ORIENTED_EDGE('',*,*,#29060,.F.) ;
#41176=ORIENTED_EDGE('',*,*,#29057,.F.) ;
#41177=ORIENTED_EDGE('',*,*,#29055,.F.) ;
#41178=ORIENTED_EDGE('',*,*,#29053,.F.) ;
#41179=ORIENTED_EDGE('',*,*,#29048,.F.) ;
#41180=ORIENTED_EDGE('',*,*,#28612,.T.) ;
#41181=ORIENTED_EDGE('',*,*,#29090,.T.) ;
#41182=ORIENTED_EDGE('',*,*,#29091,.T.) ;
#41183=ORIENTED_EDGE('',*,*,#29092,.F.) ;
#41184=ORIENTED_EDGE('',*,*,#29093,.T.) ;
#41185=ORIENTED_EDGE('',*,*,#29094,.T.) ;
#41186=ORIENTED_EDGE('',*,*,#28613,.T.) ;
#41187=ORIENTED_EDGE('',*,*,#29092,.T.) ;
#41188=ORIENTED_EDGE('',*,*,#28618,.T.) ;
#41189=ORIENTED_EDGE('',*,*,#29095,.T.) ;
#41190=ORIENTED_EDGE('',*,*,#28873,.T.) ;
#41191=ORIENTED_EDGE('',*,*,#29090,.F.) ;
#41192=ORIENTED_EDGE('',*,*,#28617,.T.) ;
#41193=ORIENTED_EDGE('',*,*,#29096,.T.) ;
#41194=ORIENTED_EDGE('',*,*,#28871,.T.) ;
#41195=ORIENTED_EDGE('',*,*,#29095,.F.) ;
#41196=ORIENTED_EDGE('',*,*,#28616,.T.) ;
#41197=ORIENTED_EDGE('',*,*,#29097,.T.) ;
#41198=ORIENTED_EDGE('',*,*,#28869,.T.) ;
#41199=ORIENTED_EDGE('',*,*,#29096,.F.) ;
#41200=ORIENTED_EDGE('',*,*,#28866,.T.) ;
#41201=ORIENTED_EDGE('',*,*,#29097,.F.) ;
#41202=ORIENTED_EDGE('',*,*,#28615,.T.) ;
#41203=ORIENTED_EDGE('',*,*,#29098,.T.) ;
#41204=ORIENTED_EDGE('',*,*,#29099,.T.) ;
#41205=ORIENTED_EDGE('',*,*,#29098,.F.) ;
#41206=ORIENTED_EDGE('',*,*,#28614,.T.) ;
#41207=ORIENTED_EDGE('',*,*,#29094,.F.) ;
#41208=ORIENTED_EDGE('',*,*,#28854,.F.) ;
#41209=ORIENTED_EDGE('',*,*,#28867,.F.) ;
#41210=ORIENTED_EDGE('',*,*,#29099,.F.) ;
#41211=ORIENTED_EDGE('',*,*,#29100,.T.) ;
#41212=ORIENTED_EDGE('',*,*,#28853,.F.) ;
#41213=ORIENTED_EDGE('',*,*,#29100,.F.) ;
#41214=ORIENTED_EDGE('',*,*,#29093,.F.) ;
#41215=ORIENTED_EDGE('',*,*,#29101,.T.) ;
#41216=ORIENTED_EDGE('',*,*,#28850,.F.) ;
#41217=ORIENTED_EDGE('',*,*,#29101,.F.) ;
#41218=ORIENTED_EDGE('',*,*,#29091,.F.) ;
#41219=ORIENTED_EDGE('',*,*,#28872,.T.) ;
#41220=ORIENTED_EDGE('',*,*,#28622,.T.) ;
#41221=ORIENTED_EDGE('',*,*,#29102,.T.) ;
#41222=ORIENTED_EDGE('',*,*,#28899,.T.) ;
#41223=ORIENTED_EDGE('',*,*,#29103,.F.) ;
#41224=ORIENTED_EDGE('',*,*,#28621,.T.) ;
#41225=ORIENTED_EDGE('',*,*,#29104,.T.) ;
#41226=ORIENTED_EDGE('',*,*,#28896,.T.) ;
#41227=ORIENTED_EDGE('',*,*,#29102,.F.) ;
#41228=ORIENTED_EDGE('',*,*,#28619,.T.) ;
#41229=ORIENTED_EDGE('',*,*,#29105,.T.) ;
#41230=ORIENTED_EDGE('',*,*,#29106,.T.) ;
#41231=ORIENTED_EDGE('',*,*,#29107,.T.) ;
#41232=ORIENTED_EDGE('',*,*,#29108,.T.) ;
#41233=ORIENTED_EDGE('',*,*,#29105,.F.) ;
#41234=ORIENTED_EDGE('',*,*,#28625,.T.) ;
#41235=ORIENTED_EDGE('',*,*,#29109,.T.) ;
#41236=ORIENTED_EDGE('',*,*,#28620,.T.) ;
#41237=ORIENTED_EDGE('',*,*,#29107,.F.) ;
#41238=ORIENTED_EDGE('',*,*,#29110,.T.) ;
#41239=ORIENTED_EDGE('',*,*,#29104,.F.) ;
#41240=ORIENTED_EDGE('',*,*,#28903,.T.) ;
#41241=ORIENTED_EDGE('',*,*,#29109,.F.) ;
#41242=ORIENTED_EDGE('',*,*,#28624,.T.) ;
#41243=ORIENTED_EDGE('',*,*,#29111,.T.) ;
#41244=ORIENTED_EDGE('',*,*,#28901,.T.) ;
#41245=ORIENTED_EDGE('',*,*,#29111,.F.) ;
#41246=ORIENTED_EDGE('',*,*,#28623,.T.) ;
#41247=ORIENTED_EDGE('',*,*,#29103,.T.) ;
#41248=ORIENTED_EDGE('',*,*,#28884,.F.) ;
#41249=ORIENTED_EDGE('',*,*,#28897,.F.) ;
#41250=ORIENTED_EDGE('',*,*,#29110,.F.) ;
#41251=ORIENTED_EDGE('',*,*,#29112,.T.) ;
#41252=ORIENTED_EDGE('',*,*,#28883,.F.) ;
#41253=ORIENTED_EDGE('',*,*,#29112,.F.) ;
#41254=ORIENTED_EDGE('',*,*,#29106,.F.) ;
#41255=ORIENTED_EDGE('',*,*,#29113,.T.) ;
#41256=ORIENTED_EDGE('',*,*,#29114,.T.) ;
#41257=ORIENTED_EDGE('',*,*,#29115,.T.) ;
#41258=ORIENTED_EDGE('',*,*,#29116,.T.) ;
#41259=ORIENTED_EDGE('',*,*,#29117,.F.) ;
#41260=ORIENTED_EDGE('',*,*,#29118,.T.) ;
#41261=ORIENTED_EDGE('',*,*,#29119,.T.) ;
#41262=ORIENTED_EDGE('',*,*,#29120,.T.) ;
#41263=ORIENTED_EDGE('',*,*,#29117,.T.) ;
#41264=ORIENTED_EDGE('',*,*,#29121,.T.) ;
#41265=ORIENTED_EDGE('',*,*,#29122,.T.) ;
#41266=ORIENTED_EDGE('',*,*,#28933,.T.) ;
#41267=ORIENTED_EDGE('',*,*,#29115,.F.) ;
#41268=ORIENTED_EDGE('',*,*,#29123,.T.) ;
#41269=ORIENTED_EDGE('',*,*,#29124,.T.) ;
#41270=ORIENTED_EDGE('',*,*,#28931,.T.) ;
#41271=ORIENTED_EDGE('',*,*,#29122,.F.) ;
#41272=ORIENTED_EDGE('',*,*,#29125,.T.) ;
#41273=ORIENTED_EDGE('',*,*,#29126,.T.) ;
#41274=ORIENTED_EDGE('',*,*,#28929,.T.) ;
#41275=ORIENTED_EDGE('',*,*,#29124,.F.) ;
#41276=ORIENTED_EDGE('',*,*,#28926,.T.) ;
#41277=ORIENTED_EDGE('',*,*,#29126,.F.) ;
#41278=ORIENTED_EDGE('',*,*,#29127,.T.) ;
#41279=ORIENTED_EDGE('',*,*,#29128,.T.) ;
#41280=ORIENTED_EDGE('',*,*,#29129,.T.) ;
#41281=ORIENTED_EDGE('',*,*,#29128,.F.) ;
#41282=ORIENTED_EDGE('',*,*,#29130,.T.) ;
#41283=ORIENTED_EDGE('',*,*,#29119,.F.) ;
#41284=ORIENTED_EDGE('',*,*,#28914,.F.) ;
#41285=ORIENTED_EDGE('',*,*,#28927,.F.) ;
#41286=ORIENTED_EDGE('',*,*,#29129,.F.) ;
#41287=ORIENTED_EDGE('',*,*,#29131,.T.) ;
#41288=ORIENTED_EDGE('',*,*,#28913,.F.) ;
#41289=ORIENTED_EDGE('',*,*,#29131,.F.) ;
#41290=ORIENTED_EDGE('',*,*,#29118,.F.) ;
#41291=ORIENTED_EDGE('',*,*,#29132,.T.) ;
#41292=ORIENTED_EDGE('',*,*,#28910,.F.) ;
#41293=ORIENTED_EDGE('',*,*,#29132,.F.) ;
#41294=ORIENTED_EDGE('',*,*,#29116,.F.) ;
#41295=ORIENTED_EDGE('',*,*,#28932,.T.) ;
#41296=ORIENTED_EDGE('',*,*,#29133,.F.) ;
#41297=ORIENTED_EDGE('',*,*,#29134,.F.) ;
#41298=ORIENTED_EDGE('',*,*,#29135,.F.) ;
#41299=ORIENTED_EDGE('',*,*,#29136,.F.) ;
#41300=ORIENTED_EDGE('',*,*,#28718,.F.) ;
#41301=ORIENTED_EDGE('',*,*,#29137,.F.) ;
#41302=ORIENTED_EDGE('',*,*,#29138,.F.) ;
#41303=ORIENTED_EDGE('',*,*,#29139,.F.) ;
#41304=ORIENTED_EDGE('',*,*,#29140,.F.) ;
#41305=ORIENTED_EDGE('',*,*,#27528,.F.) ;
#41306=ORIENTED_EDGE('',*,*,#29141,.F.) ;
#41307=ORIENTED_EDGE('',*,*,#29142,.F.) ;
#41308=ORIENTED_EDGE('',*,*,#29143,.F.) ;
#41309=ORIENTED_EDGE('',*,*,#29144,.F.) ;
#41310=ORIENTED_EDGE('',*,*,#29145,.F.) ;
#41311=ORIENTED_EDGE('',*,*,#29146,.F.) ;
#41312=ORIENTED_EDGE('',*,*,#29147,.F.) ;
#41313=ORIENTED_EDGE('',*,*,#29148,.F.) ;
#41314=ORIENTED_EDGE('',*,*,#29149,.F.) ;
#41315=ORIENTED_EDGE('',*,*,#29150,.F.) ;
#41316=ORIENTED_EDGE('',*,*,#29151,.F.) ;
#41317=ORIENTED_EDGE('',*,*,#29152,.F.) ;
#41318=ORIENTED_EDGE('',*,*,#29153,.F.) ;
#41319=ORIENTED_EDGE('',*,*,#29154,.F.) ;
#41320=ORIENTED_EDGE('',*,*,#29114,.F.) ;
#41321=ORIENTED_EDGE('',*,*,#29120,.F.) ;
#41322=ORIENTED_EDGE('',*,*,#29130,.F.) ;
#41323=ORIENTED_EDGE('',*,*,#29127,.F.) ;
#41324=ORIENTED_EDGE('',*,*,#29125,.F.) ;
#41325=ORIENTED_EDGE('',*,*,#29123,.F.) ;
#41326=ORIENTED_EDGE('',*,*,#29121,.F.) ;
#41327=ORIENTED_EDGE('',*,*,#29144,.T.) ;
#41328=ORIENTED_EDGE('',*,*,#29155,.T.) ;
#41329=ORIENTED_EDGE('',*,*,#28950,.T.) ;
#41330=ORIENTED_EDGE('',*,*,#29156,.T.) ;
#41331=ORIENTED_EDGE('',*,*,#29147,.T.) ;
#41332=ORIENTED_EDGE('',*,*,#29157,.T.) ;
#41333=ORIENTED_EDGE('',*,*,#28947,.T.) ;
#41334=ORIENTED_EDGE('',*,*,#29155,.F.) ;
#41335=ORIENTED_EDGE('',*,*,#29158,.T.) ;
#41336=ORIENTED_EDGE('',*,*,#29157,.F.) ;
#41337=ORIENTED_EDGE('',*,*,#29146,.T.) ;
#41338=ORIENTED_EDGE('',*,*,#29159,.T.) ;
#41339=ORIENTED_EDGE('',*,*,#29145,.T.) ;
#41340=ORIENTED_EDGE('',*,*,#29156,.F.) ;
#41341=ORIENTED_EDGE('',*,*,#29160,.T.) ;
#41342=ORIENTED_EDGE('',*,*,#29159,.F.) ;
#41343=ORIENTED_EDGE('',*,*,#28938,.F.) ;
#41344=ORIENTED_EDGE('',*,*,#29161,.F.) ;
#41345=ORIENTED_EDGE('',*,*,#29160,.F.) ;
#41346=ORIENTED_EDGE('',*,*,#28949,.T.) ;
#41347=ORIENTED_EDGE('',*,*,#29148,.T.) ;
#41348=ORIENTED_EDGE('',*,*,#29162,.T.) ;
#41349=ORIENTED_EDGE('',*,*,#29163,.T.) ;
#41350=ORIENTED_EDGE('',*,*,#29164,.T.) ;
#41351=ORIENTED_EDGE('',*,*,#29154,.T.) ;
#41352=ORIENTED_EDGE('',*,*,#29165,.T.) ;
#41353=ORIENTED_EDGE('',*,*,#29166,.T.) ;
#41354=ORIENTED_EDGE('',*,*,#29162,.F.) ;
#41355=ORIENTED_EDGE('',*,*,#29153,.T.) ;
#41356=ORIENTED_EDGE('',*,*,#29167,.T.) ;
#41357=ORIENTED_EDGE('',*,*,#28980,.T.) ;
#41358=ORIENTED_EDGE('',*,*,#29165,.F.) ;
#41359=ORIENTED_EDGE('',*,*,#29152,.T.) ;
#41360=ORIENTED_EDGE('',*,*,#29168,.T.) ;
#41361=ORIENTED_EDGE('',*,*,#28978,.T.) ;
#41362=ORIENTED_EDGE('',*,*,#29167,.F.) ;
#41363=ORIENTED_EDGE('',*,*,#28976,.T.) ;
#41364=ORIENTED_EDGE('',*,*,#29168,.F.) ;
#41365=ORIENTED_EDGE('',*,*,#29151,.T.) ;
#41366=ORIENTED_EDGE('',*,*,#29169,.T.) ;
#41367=ORIENTED_EDGE('',*,*,#28973,.T.) ;
#41368=ORIENTED_EDGE('',*,*,#29169,.F.) ;
#41369=ORIENTED_EDGE('',*,*,#29150,.T.) ;
#41370=ORIENTED_EDGE('',*,*,#29170,.T.) ;
#41371=ORIENTED_EDGE('',*,*,#29171,.T.) ;
#41372=ORIENTED_EDGE('',*,*,#29170,.F.) ;
#41373=ORIENTED_EDGE('',*,*,#29149,.T.) ;
#41374=ORIENTED_EDGE('',*,*,#29164,.F.) ;
#41375=ORIENTED_EDGE('',*,*,#28961,.F.) ;
#41376=ORIENTED_EDGE('',*,*,#28974,.F.) ;
#41377=ORIENTED_EDGE('',*,*,#29171,.F.) ;
#41378=ORIENTED_EDGE('',*,*,#29172,.T.) ;
#41379=ORIENTED_EDGE('',*,*,#28960,.F.) ;
#41380=ORIENTED_EDGE('',*,*,#29172,.F.) ;
#41381=ORIENTED_EDGE('',*,*,#29163,.F.) ;
#41382=ORIENTED_EDGE('',*,*,#29173,.T.) ;
#41383=ORIENTED_EDGE('',*,*,#28764,.T.) ;
#41384=ORIENTED_EDGE('',*,*,#29174,.T.) ;
#41385=ORIENTED_EDGE('',*,*,#28994,.T.) ;
#41386=ORIENTED_EDGE('',*,*,#29175,.F.) ;
#41387=ORIENTED_EDGE('',*,*,#28767,.T.) ;
#41388=ORIENTED_EDGE('',*,*,#29176,.T.) ;
#41389=ORIENTED_EDGE('',*,*,#29177,.T.) ;
#41390=ORIENTED_EDGE('',*,*,#29174,.F.) ;
#41391=ORIENTED_EDGE('',*,*,#28997,.T.) ;
#41392=ORIENTED_EDGE('',*,*,#29178,.T.) ;
#41393=ORIENTED_EDGE('',*,*,#28765,.T.) ;
#41394=ORIENTED_EDGE('',*,*,#29175,.T.) ;
#41395=ORIENTED_EDGE('',*,*,#28766,.T.) ;
#41396=ORIENTED_EDGE('',*,*,#29178,.F.) ;
#41397=ORIENTED_EDGE('',*,*,#29179,.T.) ;
#41398=ORIENTED_EDGE('',*,*,#29176,.F.) ;
#41399=ORIENTED_EDGE('',*,*,#29180,.T.) ;
#41400=ORIENTED_EDGE('',*,*,#29181,.T.) ;
#41401=ORIENTED_EDGE('',*,*,#28761,.T.) ;
#41402=ORIENTED_EDGE('',*,*,#29182,.T.) ;
#41403=ORIENTED_EDGE('',*,*,#28760,.T.) ;
#41404=ORIENTED_EDGE('',*,*,#29183,.T.) ;
#41405=ORIENTED_EDGE('',*,*,#29184,.T.) ;
#41406=ORIENTED_EDGE('',*,*,#29182,.F.) ;
#41407=ORIENTED_EDGE('',*,*,#28759,.T.) ;
#41408=ORIENTED_EDGE('',*,*,#29185,.T.) ;
#41409=ORIENTED_EDGE('',*,*,#29043,.T.) ;
#41410=ORIENTED_EDGE('',*,*,#29183,.F.) ;
#41411=ORIENTED_EDGE('',*,*,#28758,.T.) ;
#41412=ORIENTED_EDGE('',*,*,#29186,.T.) ;
#41413=ORIENTED_EDGE('',*,*,#29041,.T.) ;
#41414=ORIENTED_EDGE('',*,*,#29185,.F.) ;
#41415=ORIENTED_EDGE('',*,*,#28757,.T.) ;
#41416=ORIENTED_EDGE('',*,*,#29187,.T.) ;
#41417=ORIENTED_EDGE('',*,*,#29039,.T.) ;
#41418=ORIENTED_EDGE('',*,*,#29186,.F.) ;
#41419=ORIENTED_EDGE('',*,*,#29188,.T.) ;
#41420=ORIENTED_EDGE('',*,*,#28754,.T.) ;
#41421=ORIENTED_EDGE('',*,*,#29189,.T.) ;
#41422=ORIENTED_EDGE('',*,*,#29032,.T.) ;
#41423=ORIENTED_EDGE('',*,*,#29190,.T.) ;
#41424=ORIENTED_EDGE('',*,*,#28755,.T.) ;
#41425=ORIENTED_EDGE('',*,*,#29188,.F.) ;
#41426=ORIENTED_EDGE('',*,*,#29035,.T.) ;
#41427=ORIENTED_EDGE('',*,*,#28756,.T.) ;
#41428=ORIENTED_EDGE('',*,*,#29190,.F.) ;
#41429=ORIENTED_EDGE('',*,*,#29037,.T.) ;
#41430=ORIENTED_EDGE('',*,*,#29187,.F.) ;
#41431=ORIENTED_EDGE('',*,*,#29191,.T.) ;
#41432=ORIENTED_EDGE('',*,*,#28762,.T.) ;
#41433=ORIENTED_EDGE('',*,*,#29181,.F.) ;
#41434=ORIENTED_EDGE('',*,*,#29192,.T.) ;
#41435=ORIENTED_EDGE('',*,*,#29193,.T.) ;
#41436=ORIENTED_EDGE('',*,*,#28763,.T.) ;
#41437=ORIENTED_EDGE('',*,*,#29191,.F.) ;
#41438=ORIENTED_EDGE('',*,*,#29194,.T.) ;
#41439=ORIENTED_EDGE('',*,*,#29011,.F.) ;
#41440=ORIENTED_EDGE('',*,*,#29195,.F.) ;
#41441=ORIENTED_EDGE('',*,*,#29194,.F.) ;
#41442=ORIENTED_EDGE('',*,*,#29196,.T.) ;
#41443=ORIENTED_EDGE('',*,*,#29009,.F.) ;
#41444=ORIENTED_EDGE('',*,*,#29196,.F.) ;
#41445=ORIENTED_EDGE('',*,*,#29192,.F.) ;
#41446=ORIENTED_EDGE('',*,*,#29197,.T.) ;
#41447=ORIENTED_EDGE('',*,*,#29007,.F.) ;
#41448=ORIENTED_EDGE('',*,*,#29197,.F.) ;
#41449=ORIENTED_EDGE('',*,*,#29180,.F.) ;
#41450=ORIENTED_EDGE('',*,*,#29198,.T.) ;
#41451=ORIENTED_EDGE('',*,*,#29004,.F.) ;
#41452=ORIENTED_EDGE('',*,*,#29198,.F.) ;
#41453=ORIENTED_EDGE('',*,*,#29184,.F.) ;
#41454=ORIENTED_EDGE('',*,*,#29042,.T.) ;
#41455=ORIENTED_EDGE('',*,*,#28745,.T.) ;
#41456=ORIENTED_EDGE('',*,*,#29199,.T.) ;
#41457=ORIENTED_EDGE('',*,*,#29200,.T.) ;
#41458=ORIENTED_EDGE('',*,*,#29201,.T.) ;
#41459=ORIENTED_EDGE('',*,*,#29202,.T.) ;
#41460=ORIENTED_EDGE('',*,*,#29203,.T.) ;
#41461=ORIENTED_EDGE('',*,*,#28742,.T.) ;
#41462=ORIENTED_EDGE('',*,*,#29204,.T.) ;
#41463=ORIENTED_EDGE('',*,*,#28752,.T.) ;
#41464=ORIENTED_EDGE('',*,*,#29205,.T.) ;
#41465=ORIENTED_EDGE('',*,*,#29089,.T.) ;
#41466=ORIENTED_EDGE('',*,*,#29204,.F.) ;
#41467=ORIENTED_EDGE('',*,*,#28751,.T.) ;
#41468=ORIENTED_EDGE('',*,*,#29206,.T.) ;
#41469=ORIENTED_EDGE('',*,*,#29087,.T.) ;
#41470=ORIENTED_EDGE('',*,*,#29205,.F.) ;
#41471=ORIENTED_EDGE('',*,*,#29085,.T.) ;
#41472=ORIENTED_EDGE('',*,*,#29206,.F.) ;
#41473=ORIENTED_EDGE('',*,*,#28750,.T.) ;
#41474=ORIENTED_EDGE('',*,*,#29207,.T.) ;
#41475=ORIENTED_EDGE('',*,*,#29083,.T.) ;
#41476=ORIENTED_EDGE('',*,*,#29207,.F.) ;
#41477=ORIENTED_EDGE('',*,*,#28749,.T.) ;
#41478=ORIENTED_EDGE('',*,*,#29208,.T.) ;
#41479=ORIENTED_EDGE('',*,*,#29209,.T.) ;
#41480=ORIENTED_EDGE('',*,*,#28743,.T.) ;
#41481=ORIENTED_EDGE('',*,*,#29203,.F.) ;
#41482=ORIENTED_EDGE('',*,*,#29210,.T.) ;
#41483=ORIENTED_EDGE('',*,*,#28744,.T.) ;
#41484=ORIENTED_EDGE('',*,*,#29209,.F.) ;
#41485=ORIENTED_EDGE('',*,*,#29211,.T.) ;
#41486=ORIENTED_EDGE('',*,*,#29199,.F.) ;
#41487=ORIENTED_EDGE('',*,*,#29212,.T.) ;
#41488=ORIENTED_EDGE('',*,*,#29213,.T.) ;
#41489=ORIENTED_EDGE('',*,*,#28746,.T.) ;
#41490=ORIENTED_EDGE('',*,*,#29201,.F.) ;
#41491=ORIENTED_EDGE('',*,*,#29214,.T.) ;
#41492=ORIENTED_EDGE('',*,*,#28747,.T.) ;
#41493=ORIENTED_EDGE('',*,*,#29213,.F.) ;
#41494=ORIENTED_EDGE('',*,*,#29078,.T.) ;
#41495=ORIENTED_EDGE('',*,*,#28748,.T.) ;
#41496=ORIENTED_EDGE('',*,*,#29214,.F.) ;
#41497=ORIENTED_EDGE('',*,*,#29081,.T.) ;
#41498=ORIENTED_EDGE('',*,*,#29208,.F.) ;
#41499=ORIENTED_EDGE('',*,*,#29062,.F.) ;
#41500=ORIENTED_EDGE('',*,*,#29079,.F.) ;
#41501=ORIENTED_EDGE('',*,*,#29212,.F.) ;
#41502=ORIENTED_EDGE('',*,*,#29215,.T.) ;
#41503=ORIENTED_EDGE('',*,*,#29059,.F.) ;
#41504=ORIENTED_EDGE('',*,*,#29215,.F.) ;
#41505=ORIENTED_EDGE('',*,*,#29200,.F.) ;
#41506=ORIENTED_EDGE('',*,*,#29216,.T.) ;
#41507=ORIENTED_EDGE('',*,*,#29054,.F.) ;
#41508=ORIENTED_EDGE('',*,*,#29216,.F.) ;
#41509=ORIENTED_EDGE('',*,*,#29211,.F.) ;
#41510=ORIENTED_EDGE('',*,*,#29217,.T.) ;
#41511=ORIENTED_EDGE('',*,*,#29052,.F.) ;
#41512=ORIENTED_EDGE('',*,*,#29217,.F.) ;
#41513=ORIENTED_EDGE('',*,*,#29210,.F.) ;
#41514=ORIENTED_EDGE('',*,*,#29218,.T.) ;
#41515=ORIENTED_EDGE('',*,*,#29050,.F.) ;
#41516=ORIENTED_EDGE('',*,*,#29218,.F.) ;
#41517=ORIENTED_EDGE('',*,*,#29202,.F.) ;
#41518=ORIENTED_EDGE('',*,*,#29088,.T.) ;
#41519=ORIENTED_EDGE('',*,*,#29014,.F.) ;
#41520=ORIENTED_EDGE('',*,*,#29033,.F.) ;
#41521=ORIENTED_EDGE('',*,*,#29189,.F.) ;
#41522=ORIENTED_EDGE('',*,*,#28753,.F.) ;
#41523=ORIENTED_EDGE('',*,*,#29193,.F.) ;
#41524=ORIENTED_EDGE('',*,*,#29195,.T.) ;
#41525=ORIENTED_EDGE('',*,*,#28988,.F.) ;
#41526=ORIENTED_EDGE('',*,*,#28995,.F.) ;
#41527=ORIENTED_EDGE('',*,*,#29177,.F.) ;
#41528=ORIENTED_EDGE('',*,*,#29219,.T.) ;
#41529=ORIENTED_EDGE('',*,*,#28985,.F.) ;
#41530=ORIENTED_EDGE('',*,*,#29219,.F.) ;
#41531=ORIENTED_EDGE('',*,*,#29179,.F.) ;
#41532=ORIENTED_EDGE('',*,*,#28996,.T.) ;
#41533=ORIENTED_EDGE('',*,*,#28941,.F.) ;
#41534=ORIENTED_EDGE('',*,*,#28948,.F.) ;
#41535=ORIENTED_EDGE('',*,*,#29158,.F.) ;
#41536=ORIENTED_EDGE('',*,*,#29161,.T.) ;
#41537=ORIENTED_EDGE('',*,*,#28880,.F.) ;
#41538=ORIENTED_EDGE('',*,*,#29113,.F.) ;
#41539=ORIENTED_EDGE('',*,*,#29108,.F.) ;
#41540=ORIENTED_EDGE('',*,*,#28902,.T.) ;
#41541=ORIENTED_EDGE('',*,*,#28957,.F.) ;
#41542=ORIENTED_EDGE('',*,*,#29173,.F.) ;
#41543=ORIENTED_EDGE('',*,*,#29166,.F.) ;
#41544=ORIENTED_EDGE('',*,*,#28979,.T.) ;
#41545=ORIENTED_EDGE('',*,*,#28042,.F.) ;
#41546=ORIENTED_EDGE('',*,*,#28245,.F.) ;
#41547=ORIENTED_EDGE('',*,*,#29220,.T.) ;
#41548=ORIENTED_EDGE('',*,*,#29221,.T.) ;
#41549=ORIENTED_EDGE('',*,*,#28037,.F.) ;
#41550=ORIENTED_EDGE('',*,*,#28522,.F.) ;
#41551=ORIENTED_EDGE('',*,*,#29222,.F.) ;
#41552=ORIENTED_EDGE('',*,*,#29223,.F.) ;
#41553=ORIENTED_EDGE('',*,*,#29224,.F.) ;
#41554=ORIENTED_EDGE('',*,*,#29225,.F.) ;
#41555=ORIENTED_EDGE('',*,*,#29226,.F.) ;
#41556=ORIENTED_EDGE('',*,*,#29227,.F.) ;
#41557=ORIENTED_EDGE('',*,*,#28510,.F.) ;
#41558=ORIENTED_EDGE('',*,*,#28516,.F.) ;
#41559=ORIENTED_EDGE('',*,*,#28518,.F.) ;
#41560=ORIENTED_EDGE('',*,*,#28520,.F.) ;
#41561=ORIENTED_EDGE('',*,*,#28637,.F.) ;
#41562=ORIENTED_EDGE('',*,*,#28641,.T.) ;
#41563=ORIENTED_EDGE('',*,*,#29228,.T.) ;
#41564=ORIENTED_EDGE('',*,*,#28101,.F.) ;
#41565=ORIENTED_EDGE('',*,*,#28632,.F.) ;
#41566=ORIENTED_EDGE('',*,*,#28113,.F.) ;
#41567=ORIENTED_EDGE('',*,*,#29229,.F.) ;
#41568=ORIENTED_EDGE('',*,*,#29230,.F.) ;
#41569=ORIENTED_EDGE('',*,*,#28816,.T.) ;
#41570=ORIENTED_EDGE('',*,*,#28112,.F.) ;
#41571=ORIENTED_EDGE('',*,*,#29231,.F.) ;
#41572=ORIENTED_EDGE('',*,*,#29232,.T.) ;
#41573=ORIENTED_EDGE('',*,*,#29229,.T.) ;
#41574=ORIENTED_EDGE('',*,*,#28111,.F.) ;
#41575=ORIENTED_EDGE('',*,*,#29233,.F.) ;
#41576=ORIENTED_EDGE('',*,*,#29234,.T.) ;
#41577=ORIENTED_EDGE('',*,*,#29231,.T.) ;
#41578=ORIENTED_EDGE('',*,*,#28110,.F.) ;
#41579=ORIENTED_EDGE('',*,*,#29235,.F.) ;
#41580=ORIENTED_EDGE('',*,*,#29236,.T.) ;
#41581=ORIENTED_EDGE('',*,*,#29233,.T.) ;
#41582=ORIENTED_EDGE('',*,*,#28109,.F.) ;
#41583=ORIENTED_EDGE('',*,*,#29237,.F.) ;
#41584=ORIENTED_EDGE('',*,*,#29238,.T.) ;
#41585=ORIENTED_EDGE('',*,*,#29235,.T.) ;
#41586=ORIENTED_EDGE('',*,*,#28108,.F.) ;
#41587=ORIENTED_EDGE('',*,*,#29239,.F.) ;
#41588=ORIENTED_EDGE('',*,*,#29240,.F.) ;
#41589=ORIENTED_EDGE('',*,*,#29237,.T.) ;
#41590=ORIENTED_EDGE('',*,*,#28800,.T.) ;
#41591=ORIENTED_EDGE('',*,*,#28817,.F.) ;
#41592=ORIENTED_EDGE('',*,*,#29230,.T.) ;
#41593=ORIENTED_EDGE('',*,*,#29232,.F.) ;
#41594=ORIENTED_EDGE('',*,*,#29234,.F.) ;
#41595=ORIENTED_EDGE('',*,*,#29236,.F.) ;
#41596=ORIENTED_EDGE('',*,*,#29238,.F.) ;
#41597=ORIENTED_EDGE('',*,*,#29240,.T.) ;
#41598=ORIENTED_EDGE('',*,*,#29241,.F.) ;
#41599=ORIENTED_EDGE('',*,*,#29242,.F.) ;
#41600=ORIENTED_EDGE('',*,*,#27847,.F.) ;
#41601=ORIENTED_EDGE('',*,*,#27968,.T.) ;
#41602=ORIENTED_EDGE('',*,*,#27970,.F.) ;
#41603=ORIENTED_EDGE('',*,*,#27972,.F.) ;
#41604=ORIENTED_EDGE('',*,*,#27976,.F.) ;
#41605=ORIENTED_EDGE('',*,*,#28832,.T.) ;
#41606=ORIENTED_EDGE('',*,*,#28811,.T.) ;
#41607=ORIENTED_EDGE('',*,*,#29243,.T.) ;
#41608=ORIENTED_EDGE('',*,*,#29244,.F.) ;
#41609=ORIENTED_EDGE('',*,*,#27848,.F.) ;
#41610=ORIENTED_EDGE('',*,*,#29242,.T.) ;
#41611=ORIENTED_EDGE('',*,*,#29245,.T.) ;
#41612=ORIENTED_EDGE('',*,*,#29246,.F.) ;
#41613=ORIENTED_EDGE('',*,*,#29243,.F.) ;
#41614=ORIENTED_EDGE('',*,*,#29241,.T.) ;
#41615=ORIENTED_EDGE('',*,*,#29239,.T.) ;
#41616=ORIENTED_EDGE('',*,*,#28103,.F.) ;
#41617=ORIENTED_EDGE('',*,*,#29247,.F.) ;
#41618=ORIENTED_EDGE('',*,*,#28639,.F.) ;
#41619=ORIENTED_EDGE('',*,*,#28643,.T.) ;
#41620=ORIENTED_EDGE('',*,*,#28102,.F.) ;
#41621=ORIENTED_EDGE('',*,*,#29228,.F.) ;
#41622=ORIENTED_EDGE('',*,*,#28640,.T.) ;
#41623=ORIENTED_EDGE('',*,*,#29247,.T.) ;
#41624=ORIENTED_EDGE('',*,*,#28592,.F.) ;
#41625=ORIENTED_EDGE('',*,*,#29248,.T.) ;
#41626=ORIENTED_EDGE('',*,*,#29249,.F.) ;
#41627=ORIENTED_EDGE('',*,*,#29250,.F.) ;
#41628=ORIENTED_EDGE('',*,*,#28642,.F.) ;
#41629=ORIENTED_EDGE('',*,*,#28736,.F.) ;
#41630=ORIENTED_EDGE('',*,*,#28795,.T.) ;
#41631=ORIENTED_EDGE('',*,*,#29251,.T.) ;
#41632=ORIENTED_EDGE('',*,*,#29252,.F.) ;
#41633=ORIENTED_EDGE('',*,*,#28737,.F.) ;
#41634=ORIENTED_EDGE('',*,*,#29252,.T.) ;
#41635=ORIENTED_EDGE('',*,*,#29253,.T.) ;
#41636=ORIENTED_EDGE('',*,*,#29254,.F.) ;
#41637=ORIENTED_EDGE('',*,*,#28738,.F.) ;
#41638=ORIENTED_EDGE('',*,*,#29254,.T.) ;
#41639=ORIENTED_EDGE('',*,*,#29255,.T.) ;
#41640=ORIENTED_EDGE('',*,*,#28793,.F.) ;
#41641=ORIENTED_EDGE('',*,*,#29251,.F.) ;
#41642=ORIENTED_EDGE('',*,*,#28794,.F.) ;
#41643=ORIENTED_EDGE('',*,*,#29255,.F.) ;
#41644=ORIENTED_EDGE('',*,*,#29253,.F.) ;
#41645=ORIENTED_EDGE('',*,*,#29256,.F.) ;
#41646=ORIENTED_EDGE('',*,*,#29257,.T.) ;
#41647=ORIENTED_EDGE('',*,*,#29258,.F.) ;
#41648=ORIENTED_EDGE('',*,*,#29259,.F.) ;
#41649=ORIENTED_EDGE('',*,*,#28573,.F.) ;
#41650=ORIENTED_EDGE('',*,*,#29260,.T.) ;
#41651=ORIENTED_EDGE('',*,*,#29261,.F.) ;
#41652=ORIENTED_EDGE('',*,*,#29262,.F.) ;
#41653=ORIENTED_EDGE('',*,*,#28574,.F.) ;
#41654=ORIENTED_EDGE('',*,*,#29262,.T.) ;
#41655=ORIENTED_EDGE('',*,*,#29263,.F.) ;
#41656=ORIENTED_EDGE('',*,*,#29257,.F.) ;
#41657=ORIENTED_EDGE('',*,*,#28503,.F.) ;
#41658=ORIENTED_EDGE('',*,*,#28570,.F.) ;
#41659=ORIENTED_EDGE('',*,*,#27850,.F.) ;
#41660=ORIENTED_EDGE('',*,*,#29259,.T.) ;
#41661=ORIENTED_EDGE('',*,*,#29264,.F.) ;
#41662=ORIENTED_EDGE('',*,*,#29260,.F.) ;
#41663=ORIENTED_EDGE('',*,*,#29264,.T.) ;
#41664=ORIENTED_EDGE('',*,*,#29258,.T.) ;
#41665=ORIENTED_EDGE('',*,*,#29263,.T.) ;
#41666=ORIENTED_EDGE('',*,*,#29261,.T.) ;
#41667=ORIENTED_EDGE('',*,*,#28677,.F.) ;
#41668=ORIENTED_EDGE('',*,*,#27949,.F.) ;
#41669=ORIENTED_EDGE('',*,*,#28785,.T.) ;
#41670=ORIENTED_EDGE('',*,*,#29265,.T.) ;
#41671=ORIENTED_EDGE('',*,*,#29266,.F.) ;
#41672=ORIENTED_EDGE('',*,*,#28542,.F.) ;
#41673=ORIENTED_EDGE('',*,*,#28791,.F.) ;
#41674=ORIENTED_EDGE('',*,*,#28797,.T.) ;
#41675=ORIENTED_EDGE('',*,*,#28798,.F.) ;
#41676=ORIENTED_EDGE('',*,*,#28534,.F.) ;
#41677=ORIENTED_EDGE('',*,*,#28536,.F.) ;
#41678=ORIENTED_EDGE('',*,*,#28538,.F.) ;
#41679=ORIENTED_EDGE('',*,*,#28540,.F.) ;
#41680=ORIENTED_EDGE('',*,*,#28788,.F.) ;
#41681=ORIENTED_EDGE('',*,*,#27659,.T.) ;
#41682=ORIENTED_EDGE('',*,*,#27664,.F.) ;
#41683=ORIENTED_EDGE('',*,*,#27666,.T.) ;
#41684=ORIENTED_EDGE('',*,*,#28700,.F.) ;
#41685=ORIENTED_EDGE('',*,*,#29267,.F.) ;
#41686=ORIENTED_EDGE('',*,*,#27806,.F.) ;
#41687=ORIENTED_EDGE('',*,*,#27687,.T.) ;
#41688=ORIENTED_EDGE('',*,*,#27690,.F.) ;
#41689=ORIENTED_EDGE('',*,*,#27692,.T.) ;
#41690=ORIENTED_EDGE('',*,*,#28663,.T.) ;
#41691=ORIENTED_EDGE('',*,*,#28799,.T.) ;
#41692=ORIENTED_EDGE('',*,*,#28678,.F.) ;
#41693=ORIENTED_EDGE('',*,*,#29266,.T.) ;
#41694=ORIENTED_EDGE('',*,*,#29268,.T.) ;
#41695=ORIENTED_EDGE('',*,*,#27808,.F.) ;
#41696=ORIENTED_EDGE('',*,*,#29269,.F.) ;
#41697=ORIENTED_EDGE('',*,*,#28786,.T.) ;
#41698=ORIENTED_EDGE('',*,*,#27661,.T.) ;
#41699=ORIENTED_EDGE('',*,*,#28789,.T.) ;
#41700=ORIENTED_EDGE('',*,*,#28698,.F.) ;
#41701=ORIENTED_EDGE('',*,*,#28702,.T.) ;
#41702=ORIENTED_EDGE('',*,*,#28703,.T.) ;
#41703=ORIENTED_EDGE('',*,*,#28668,.T.) ;
#41704=ORIENTED_EDGE('',*,*,#29270,.T.) ;
#41705=ORIENTED_EDGE('',*,*,#29265,.F.) ;
#41706=ORIENTED_EDGE('',*,*,#28784,.T.) ;
#41707=ORIENTED_EDGE('',*,*,#28777,.F.) ;
#41708=ORIENTED_EDGE('',*,*,#27809,.T.) ;
#41709=ORIENTED_EDGE('',*,*,#29268,.F.) ;
#41710=ORIENTED_EDGE('',*,*,#28387,.F.) ;
#41711=ORIENTED_EDGE('',*,*,#29271,.T.) ;
#41712=ORIENTED_EDGE('',*,*,#29272,.T.) ;
#41713=ORIENTED_EDGE('',*,*,#28433,.T.) ;
#41714=ORIENTED_EDGE('',*,*,#28380,.F.) ;
#41715=ORIENTED_EDGE('',*,*,#29273,.T.) ;
#41716=ORIENTED_EDGE('',*,*,#29271,.F.) ;
#41717=ORIENTED_EDGE('',*,*,#28384,.F.) ;
#41718=ORIENTED_EDGE('',*,*,#28405,.F.) ;
#41719=ORIENTED_EDGE('',*,*,#28437,.T.) ;
#41720=ORIENTED_EDGE('',*,*,#28441,.T.) ;
#41721=ORIENTED_EDGE('',*,*,#29274,.T.) ;
#41722=ORIENTED_EDGE('',*,*,#29267,.T.) ;
#41723=ORIENTED_EDGE('',*,*,#28787,.F.) ;
#41724=ORIENTED_EDGE('',*,*,#29269,.T.) ;
#41725=ORIENTED_EDGE('',*,*,#27807,.F.) ;
#41726=ORIENTED_EDGE('',*,*,#28019,.F.) ;
#41727=ORIENTED_EDGE('',*,*,#28024,.F.) ;
#41728=ORIENTED_EDGE('',*,*,#28827,.F.) ;
#41729=ORIENTED_EDGE('',*,*,#29275,.T.) ;
#41730=ORIENTED_EDGE('',*,*,#28021,.F.) ;
#41731=ORIENTED_EDGE('',*,*,#29275,.F.) ;
#41732=ORIENTED_EDGE('',*,*,#28826,.F.) ;
#41733=ORIENTED_EDGE('',*,*,#28025,.F.) ;
#41734=ORIENTED_EDGE('',*,*,#28664,.F.) ;
#41735=ORIENTED_EDGE('',*,*,#29270,.F.) ;
#41736=ORIENTED_EDGE('',*,*,#28670,.F.) ;
#41737=ORIENTED_EDGE('',*,*,#28667,.F.) ;
#41738=ORIENTED_EDGE('',*,*,#28000,.F.) ;
#41739=ORIENTED_EDGE('',*,*,#28704,.T.) ;
#41740=ORIENTED_EDGE('',*,*,#28692,.F.) ;
#41741=ORIENTED_EDGE('',*,*,#29226,.T.) ;
#41742=ORIENTED_EDGE('',*,*,#29276,.T.) ;
#41743=ORIENTED_EDGE('',*,*,#29277,.T.) ;
#41744=ORIENTED_EDGE('',*,*,#29278,.T.) ;
#41745=ORIENTED_EDGE('',*,*,#29279,.F.) ;
#41746=ORIENTED_EDGE('',*,*,#29280,.F.) ;
#41747=ORIENTED_EDGE('',*,*,#29281,.F.) ;
#41748=ORIENTED_EDGE('',*,*,#29225,.T.) ;
#41749=ORIENTED_EDGE('',*,*,#29282,.T.) ;
#41750=ORIENTED_EDGE('',*,*,#29283,.T.) ;
#41751=ORIENTED_EDGE('',*,*,#29276,.F.) ;
#41752=ORIENTED_EDGE('',*,*,#27513,.T.) ;
#41753=ORIENTED_EDGE('',*,*,#29284,.F.) ;
#41754=ORIENTED_EDGE('',*,*,#29141,.T.) ;
#41755=ORIENTED_EDGE('',*,*,#27527,.F.) ;
#41756=ORIENTED_EDGE('',*,*,#29284,.T.) ;
#41757=ORIENTED_EDGE('',*,*,#27516,.T.) ;
#41758=ORIENTED_EDGE('',*,*,#29285,.T.) ;
#41759=ORIENTED_EDGE('',*,*,#29280,.T.) ;
#41760=ORIENTED_EDGE('',*,*,#29142,.T.) ;
#41761=ORIENTED_EDGE('',*,*,#29286,.T.) ;
#41762=ORIENTED_EDGE('',*,*,#29287,.F.) ;
#41763=ORIENTED_EDGE('',*,*,#29288,.F.) ;
#41764=ORIENTED_EDGE('',*,*,#29289,.F.) ;
#41765=ORIENTED_EDGE('',*,*,#29290,.T.) ;
#41766=ORIENTED_EDGE('',*,*,#29223,.T.) ;
#41767=ORIENTED_EDGE('',*,*,#29287,.T.) ;
#41768=ORIENTED_EDGE('',*,*,#29291,.T.) ;
#41769=ORIENTED_EDGE('',*,*,#29224,.T.) ;
#41770=ORIENTED_EDGE('',*,*,#29290,.F.) ;
#41771=ORIENTED_EDGE('',*,*,#29292,.T.) ;
#41772=ORIENTED_EDGE('',*,*,#29282,.F.) ;
#41773=ORIENTED_EDGE('',*,*,#28524,.F.) ;
#41774=ORIENTED_EDGE('',*,*,#28771,.T.) ;
#41775=ORIENTED_EDGE('',*,*,#29288,.T.) ;
#41776=ORIENTED_EDGE('',*,*,#29222,.T.) ;
#41777=ORIENTED_EDGE('',*,*,#29293,.F.) ;
#41778=ORIENTED_EDGE('',*,*,#28627,.F.) ;
#41779=ORIENTED_EDGE('',*,*,#29294,.F.) ;
#41780=ORIENTED_EDGE('',*,*,#29295,.T.) ;
#41781=ORIENTED_EDGE('',*,*,#29296,.T.) ;
#41782=ORIENTED_EDGE('',*,*,#29294,.T.) ;
#41783=ORIENTED_EDGE('',*,*,#28630,.T.) ;
#41784=ORIENTED_EDGE('',*,*,#28634,.T.) ;
#41785=ORIENTED_EDGE('',*,*,#29297,.T.) ;
#41786=ORIENTED_EDGE('',*,*,#29295,.F.) ;
#41787=ORIENTED_EDGE('',*,*,#28629,.T.) ;
#41788=ORIENTED_EDGE('',*,*,#29298,.T.) ;
#41789=ORIENTED_EDGE('',*,*,#29299,.T.) ;
#41790=ORIENTED_EDGE('',*,*,#29139,.T.) ;
#41791=ORIENTED_EDGE('',*,*,#29300,.T.) ;
#41792=ORIENTED_EDGE('',*,*,#28719,.F.) ;
#41793=ORIENTED_EDGE('',*,*,#29301,.F.) ;
#41794=ORIENTED_EDGE('',*,*,#29302,.T.) ;
#41795=ORIENTED_EDGE('',*,*,#29303,.F.) ;
#41796=ORIENTED_EDGE('',*,*,#29304,.T.) ;
#41797=ORIENTED_EDGE('',*,*,#29305,.T.) ;
#41798=ORIENTED_EDGE('',*,*,#29135,.T.) ;
#41799=ORIENTED_EDGE('',*,*,#29306,.T.) ;
#41800=ORIENTED_EDGE('',*,*,#29301,.T.) ;
#41801=ORIENTED_EDGE('',*,*,#29136,.T.) ;
#41802=ORIENTED_EDGE('',*,*,#29305,.F.) ;
#41803=ORIENTED_EDGE('',*,*,#29307,.T.) ;
#41804=ORIENTED_EDGE('',*,*,#29289,.T.) ;
#41805=ORIENTED_EDGE('',*,*,#28770,.T.) ;
#41806=ORIENTED_EDGE('',*,*,#29303,.T.) ;
#41807=ORIENTED_EDGE('',*,*,#29308,.T.) ;
#41808=ORIENTED_EDGE('',*,*,#29309,.T.) ;
#41809=ORIENTED_EDGE('',*,*,#29310,.F.) ;
#41810=ORIENTED_EDGE('',*,*,#28717,.F.) ;
#41811=ORIENTED_EDGE('',*,*,#29311,.F.) ;
#41812=ORIENTED_EDGE('',*,*,#29312,.T.) ;
#41813=ORIENTED_EDGE('',*,*,#29137,.T.) ;
#41814=ORIENTED_EDGE('',*,*,#29310,.T.) ;
#41815=ORIENTED_EDGE('',*,*,#29313,.T.) ;
#41816=ORIENTED_EDGE('',*,*,#29138,.T.) ;
#41817=ORIENTED_EDGE('',*,*,#29312,.F.) ;
#41818=ORIENTED_EDGE('',*,*,#29314,.T.) ;
#41819=ORIENTED_EDGE('',*,*,#29300,.F.) ;
#41820=ORIENTED_EDGE('',*,*,#28421,.F.) ;
#41821=ORIENTED_EDGE('',*,*,#29315,.F.) ;
#41822=ORIENTED_EDGE('',*,*,#29316,.T.) ;
#41823=ORIENTED_EDGE('',*,*,#29317,.F.) ;
#41824=ORIENTED_EDGE('',*,*,#29318,.T.) ;
#41825=ORIENTED_EDGE('',*,*,#29319,.T.) ;
#41826=ORIENTED_EDGE('',*,*,#28610,.T.) ;
#41827=ORIENTED_EDGE('',*,*,#29320,.T.) ;
#41828=ORIENTED_EDGE('',*,*,#29315,.T.) ;
#41829=ORIENTED_EDGE('',*,*,#28611,.T.) ;
#41830=ORIENTED_EDGE('',*,*,#29319,.F.) ;
#41831=ORIENTED_EDGE('',*,*,#29321,.T.) ;
#41832=ORIENTED_EDGE('',*,*,#29311,.T.) ;
#41833=ORIENTED_EDGE('',*,*,#27710,.T.) ;
#41834=ORIENTED_EDGE('',*,*,#29317,.T.) ;
#41835=ORIENTED_EDGE('',*,*,#29322,.T.) ;
#41836=ORIENTED_EDGE('',*,*,#29323,.T.) ;
#41837=ORIENTED_EDGE('',*,*,#29324,.T.) ;
#41838=ORIENTED_EDGE('',*,*,#29325,.T.) ;
#41839=ORIENTED_EDGE('',*,*,#28608,.T.) ;
#41840=ORIENTED_EDGE('',*,*,#28609,.T.) ;
#41841=ORIENTED_EDGE('',*,*,#29325,.F.) ;
#41842=ORIENTED_EDGE('',*,*,#29326,.T.) ;
#41843=ORIENTED_EDGE('',*,*,#29320,.F.) ;
#41844=ORIENTED_EDGE('',*,*,#29293,.T.) ;
#41845=ORIENTED_EDGE('',*,*,#29327,.T.) ;
#41846=ORIENTED_EDGE('',*,*,#29323,.F.) ;
#41847=ORIENTED_EDGE('',*,*,#28607,.T.) ;
#41848=ORIENTED_EDGE('',*,*,#27525,.T.) ;
#41849=ORIENTED_EDGE('',*,*,#27529,.T.) ;
#41850=ORIENTED_EDGE('',*,*,#29140,.T.) ;
#41851=ORIENTED_EDGE('',*,*,#29299,.F.) ;
#41852=ORIENTED_EDGE('',*,*,#29328,.T.) ;
#41853=ORIENTED_EDGE('',*,*,#29329,.T.) ;
#41854=ORIENTED_EDGE('',*,*,#29330,.T.) ;
#41855=ORIENTED_EDGE('',*,*,#29331,.T.) ;
#41856=ORIENTED_EDGE('',*,*,#29133,.T.) ;
#41857=ORIENTED_EDGE('',*,*,#29134,.T.) ;
#41858=ORIENTED_EDGE('',*,*,#29331,.F.) ;
#41859=ORIENTED_EDGE('',*,*,#29332,.T.) ;
#41860=ORIENTED_EDGE('',*,*,#29306,.F.) ;
#41861=ORIENTED_EDGE('',*,*,#29333,.T.) ;
#41862=ORIENTED_EDGE('',*,*,#29334,.T.) ;
#41863=ORIENTED_EDGE('',*,*,#29335,.T.) ;
#41864=ORIENTED_EDGE('',*,*,#29336,.T.) ;
#41865=ORIENTED_EDGE('',*,*,#27518,.T.) ;
#41866=ORIENTED_EDGE('',*,*,#27523,.T.) ;
#41867=ORIENTED_EDGE('',*,*,#29337,.T.) ;
#41868=ORIENTED_EDGE('',*,*,#29335,.F.) ;
#41869=ORIENTED_EDGE('',*,*,#29338,.T.) ;
#41870=ORIENTED_EDGE('',*,*,#29279,.T.) ;
#41871=ORIENTED_EDGE('',*,*,#29339,.T.) ;
#41872=ORIENTED_EDGE('',*,*,#29329,.F.) ;
#41873=ORIENTED_EDGE('',*,*,#29143,.T.) ;
#41874=ORIENTED_EDGE('',*,*,#29340,.T.) ;
#41875=ORIENTED_EDGE('',*,*,#29341,.T.) ;
#41876=ORIENTED_EDGE('',*,*,#29281,.T.) ;
#41877=ORIENTED_EDGE('',*,*,#29342,.T.) ;
#41878=ORIENTED_EDGE('',*,*,#29343,.T.) ;
#41879=ORIENTED_EDGE('',*,*,#29344,.T.) ;
#41880=ORIENTED_EDGE('',*,*,#29340,.F.) ;
#41881=ORIENTED_EDGE('',*,*,#29345,.T.) ;
#41882=ORIENTED_EDGE('',*,*,#28513,.F.) ;
#41883=ORIENTED_EDGE('',*,*,#29346,.T.) ;
#41884=ORIENTED_EDGE('',*,*,#29347,.T.) ;
#41885=ORIENTED_EDGE('',*,*,#29348,.T.) ;
#41886=ORIENTED_EDGE('',*,*,#29349,.T.) ;
#41887=ORIENTED_EDGE('',*,*,#29350,.T.) ;
#41888=ORIENTED_EDGE('',*,*,#29347,.F.) ;
#41889=ORIENTED_EDGE('',*,*,#29351,.T.) ;
#41890=ORIENTED_EDGE('',*,*,#29352,.T.) ;
#41891=ORIENTED_EDGE('',*,*,#29349,.F.) ;
#41892=ORIENTED_EDGE('',*,*,#29353,.T.) ;
#41893=ORIENTED_EDGE('',*,*,#29278,.F.) ;
#41894=ORIENTED_EDGE('',*,*,#29318,.F.) ;
#41895=ORIENTED_EDGE('',*,*,#29354,.F.) ;
#41896=ORIENTED_EDGE('',*,*,#28095,.F.) ;
#41897=ORIENTED_EDGE('',*,*,#29355,.T.) ;
#41898=ORIENTED_EDGE('',*,*,#29326,.F.) ;
#41899=ORIENTED_EDGE('',*,*,#29356,.F.) ;
#41900=ORIENTED_EDGE('',*,*,#28096,.F.) ;
#41901=ORIENTED_EDGE('',*,*,#29354,.T.) ;
#41902=ORIENTED_EDGE('',*,*,#29324,.F.) ;
#41903=ORIENTED_EDGE('',*,*,#29357,.F.) ;
#41904=ORIENTED_EDGE('',*,*,#28097,.F.) ;
#41905=ORIENTED_EDGE('',*,*,#29356,.T.) ;
#41906=ORIENTED_EDGE('',*,*,#29327,.F.) ;
#41907=ORIENTED_EDGE('',*,*,#29296,.F.) ;
#41908=ORIENTED_EDGE('',*,*,#29358,.T.) ;
#41909=ORIENTED_EDGE('',*,*,#28098,.T.) ;
#41910=ORIENTED_EDGE('',*,*,#29357,.T.) ;
#41911=ORIENTED_EDGE('',*,*,#29297,.F.) ;
#41912=ORIENTED_EDGE('',*,*,#28633,.T.) ;
#41913=ORIENTED_EDGE('',*,*,#28099,.T.) ;
#41914=ORIENTED_EDGE('',*,*,#29358,.F.) ;
#41915=ORIENTED_EDGE('',*,*,#28514,.F.) ;
#41916=ORIENTED_EDGE('',*,*,#29227,.T.) ;
#41917=ORIENTED_EDGE('',*,*,#29353,.F.) ;
#41918=ORIENTED_EDGE('',*,*,#29351,.F.) ;
#41919=ORIENTED_EDGE('',*,*,#29346,.F.) ;
#41920=ORIENTED_EDGE('',*,*,#28594,.F.) ;
#41921=ORIENTED_EDGE('',*,*,#28505,.T.) ;
#41922=ORIENTED_EDGE('',*,*,#29359,.F.) ;
#41923=ORIENTED_EDGE('',*,*,#29248,.F.) ;
#41924=ORIENTED_EDGE('',*,*,#29298,.F.) ;
#41925=ORIENTED_EDGE('',*,*,#29360,.T.) ;
#41926=ORIENTED_EDGE('',*,*,#28092,.F.) ;
#41927=ORIENTED_EDGE('',*,*,#29361,.T.) ;
#41928=ORIENTED_EDGE('',*,*,#29332,.F.) ;
#41929=ORIENTED_EDGE('',*,*,#29362,.F.) ;
#41930=ORIENTED_EDGE('',*,*,#28084,.F.) ;
#41931=ORIENTED_EDGE('',*,*,#29363,.T.) ;
#41932=ORIENTED_EDGE('',*,*,#29364,.T.) ;
#41933=ORIENTED_EDGE('',*,*,#28139,.T.) ;
#41934=ORIENTED_EDGE('',*,*,#29365,.T.) ;
#41935=ORIENTED_EDGE('',*,*,#29366,.T.) ;
#41936=ORIENTED_EDGE('',*,*,#29367,.T.) ;
#41937=ORIENTED_EDGE('',*,*,#29365,.F.) ;
#41938=ORIENTED_EDGE('',*,*,#28138,.F.) ;
#41939=ORIENTED_EDGE('',*,*,#29368,.T.) ;
#41940=ORIENTED_EDGE('',*,*,#29369,.T.) ;
#41941=ORIENTED_EDGE('',*,*,#29368,.F.) ;
#41942=ORIENTED_EDGE('',*,*,#28137,.T.) ;
#41943=ORIENTED_EDGE('',*,*,#29370,.T.) ;
#41944=ORIENTED_EDGE('',*,*,#29371,.T.) ;
#41945=ORIENTED_EDGE('',*,*,#29370,.F.) ;
#41946=ORIENTED_EDGE('',*,*,#28136,.T.) ;
#41947=ORIENTED_EDGE('',*,*,#29372,.T.) ;
#41948=ORIENTED_EDGE('',*,*,#29373,.T.) ;
#41949=ORIENTED_EDGE('',*,*,#29372,.F.) ;
#41950=ORIENTED_EDGE('',*,*,#28135,.F.) ;
#41951=ORIENTED_EDGE('',*,*,#29374,.T.) ;
#41952=ORIENTED_EDGE('',*,*,#29375,.T.) ;
#41953=ORIENTED_EDGE('',*,*,#29374,.F.) ;
#41954=ORIENTED_EDGE('',*,*,#28134,.T.) ;
#41955=ORIENTED_EDGE('',*,*,#29376,.T.) ;
#41956=ORIENTED_EDGE('',*,*,#29377,.T.) ;
#41957=ORIENTED_EDGE('',*,*,#29376,.F.) ;
#41958=ORIENTED_EDGE('',*,*,#28133,.F.) ;
#41959=ORIENTED_EDGE('',*,*,#29378,.T.) ;
#41960=ORIENTED_EDGE('',*,*,#29379,.T.) ;
#41961=ORIENTED_EDGE('',*,*,#29378,.F.) ;
#41962=ORIENTED_EDGE('',*,*,#28132,.T.) ;
#41963=ORIENTED_EDGE('',*,*,#29380,.T.) ;
#41964=ORIENTED_EDGE('',*,*,#29381,.T.) ;
#41965=ORIENTED_EDGE('',*,*,#29380,.F.) ;
#41966=ORIENTED_EDGE('',*,*,#28131,.T.) ;
#41967=ORIENTED_EDGE('',*,*,#29382,.T.) ;
#41968=ORIENTED_EDGE('',*,*,#28107,.F.) ;
#41969=ORIENTED_EDGE('',*,*,#29383,.T.) ;
#41970=ORIENTED_EDGE('',*,*,#29384,.F.) ;
#41971=ORIENTED_EDGE('',*,*,#29245,.F.) ;
#41972=ORIENTED_EDGE('',*,*,#28106,.T.) ;
#41973=ORIENTED_EDGE('',*,*,#29385,.T.) ;
#41974=ORIENTED_EDGE('',*,*,#29386,.F.) ;
#41975=ORIENTED_EDGE('',*,*,#29383,.F.) ;
#41976=ORIENTED_EDGE('',*,*,#28105,.F.) ;
#41977=ORIENTED_EDGE('',*,*,#29250,.T.) ;
#41978=ORIENTED_EDGE('',*,*,#29387,.F.) ;
#41979=ORIENTED_EDGE('',*,*,#29385,.F.) ;
#41980=ORIENTED_EDGE('',*,*,#28393,.F.) ;
#41981=ORIENTED_EDGE('',*,*,#28432,.F.) ;
#41982=ORIENTED_EDGE('',*,*,#28171,.T.) ;
#41983=ORIENTED_EDGE('',*,*,#29388,.T.) ;
#41984=ORIENTED_EDGE('',*,*,#28396,.F.) ;
#41985=ORIENTED_EDGE('',*,*,#29388,.F.) ;
#41986=ORIENTED_EDGE('',*,*,#28170,.T.) ;
#41987=ORIENTED_EDGE('',*,*,#29389,.T.) ;
#41988=ORIENTED_EDGE('',*,*,#29390,.T.) ;
#41989=ORIENTED_EDGE('',*,*,#28399,.F.) ;
#41990=ORIENTED_EDGE('',*,*,#29389,.F.) ;
#41991=ORIENTED_EDGE('',*,*,#28169,.T.) ;
#41992=ORIENTED_EDGE('',*,*,#28438,.T.) ;
#41993=ORIENTED_EDGE('',*,*,#28173,.T.) ;
#41994=ORIENTED_EDGE('',*,*,#29391,.T.) ;
#41995=ORIENTED_EDGE('',*,*,#29392,.T.) ;
#41996=ORIENTED_EDGE('',*,*,#29391,.F.) ;
#41997=ORIENTED_EDGE('',*,*,#29393,.T.) ;
#41998=ORIENTED_EDGE('',*,*,#28081,.T.) ;
#41999=ORIENTED_EDGE('',*,*,#29394,.T.) ;
#42000=ORIENTED_EDGE('',*,*,#29395,.T.) ;
#42001=ORIENTED_EDGE('',*,*,#29396,.T.) ;
#42002=ORIENTED_EDGE('',*,*,#29394,.F.) ;
#42003=ORIENTED_EDGE('',*,*,#28080,.T.) ;
#42004=ORIENTED_EDGE('',*,*,#29397,.T.) ;
#42005=ORIENTED_EDGE('',*,*,#29398,.T.) ;
#42006=ORIENTED_EDGE('',*,*,#29397,.F.) ;
#42007=ORIENTED_EDGE('',*,*,#28079,.T.) ;
#42008=ORIENTED_EDGE('',*,*,#29399,.T.) ;
#42009=ORIENTED_EDGE('',*,*,#29400,.T.) ;
#42010=ORIENTED_EDGE('',*,*,#29399,.F.) ;
#42011=ORIENTED_EDGE('',*,*,#28078,.T.) ;
#42012=ORIENTED_EDGE('',*,*,#29401,.T.) ;
#42013=ORIENTED_EDGE('',*,*,#29402,.T.) ;
#42014=ORIENTED_EDGE('',*,*,#29401,.F.) ;
#42015=ORIENTED_EDGE('',*,*,#28077,.T.) ;
#42016=ORIENTED_EDGE('',*,*,#29403,.T.) ;
#42017=ORIENTED_EDGE('',*,*,#29404,.T.) ;
#42018=ORIENTED_EDGE('',*,*,#29405,.F.) ;
#42019=ORIENTED_EDGE('',*,*,#28181,.T.) ;
#42020=ORIENTED_EDGE('',*,*,#29406,.T.) ;
#42021=ORIENTED_EDGE('',*,*,#29407,.T.) ;
#42022=ORIENTED_EDGE('',*,*,#29406,.F.) ;
#42023=ORIENTED_EDGE('',*,*,#28180,.T.) ;
#42024=ORIENTED_EDGE('',*,*,#29408,.T.) ;
#42025=ORIENTED_EDGE('',*,*,#29409,.T.) ;
#42026=ORIENTED_EDGE('',*,*,#29408,.F.) ;
#42027=ORIENTED_EDGE('',*,*,#28179,.T.) ;
#42028=ORIENTED_EDGE('',*,*,#29410,.T.) ;
#42029=ORIENTED_EDGE('',*,*,#29411,.T.) ;
#42030=ORIENTED_EDGE('',*,*,#29410,.F.) ;
#42031=ORIENTED_EDGE('',*,*,#28178,.T.) ;
#42032=ORIENTED_EDGE('',*,*,#29412,.T.) ;
#42033=ORIENTED_EDGE('',*,*,#29413,.T.) ;
#42034=ORIENTED_EDGE('',*,*,#29412,.F.) ;
#42035=ORIENTED_EDGE('',*,*,#28177,.T.) ;
#42036=ORIENTED_EDGE('',*,*,#29414,.T.) ;
#42037=ORIENTED_EDGE('',*,*,#29415,.T.) ;
#42038=ORIENTED_EDGE('',*,*,#29414,.F.) ;
#42039=ORIENTED_EDGE('',*,*,#28176,.T.) ;
#42040=ORIENTED_EDGE('',*,*,#29416,.T.) ;
#42041=ORIENTED_EDGE('',*,*,#29417,.T.) ;
#42042=ORIENTED_EDGE('',*,*,#29416,.F.) ;
#42043=ORIENTED_EDGE('',*,*,#28175,.T.) ;
#42044=ORIENTED_EDGE('',*,*,#29418,.T.) ;
#42045=ORIENTED_EDGE('',*,*,#28188,.T.) ;
#42046=ORIENTED_EDGE('',*,*,#29419,.T.) ;
#42047=ORIENTED_EDGE('',*,*,#29420,.T.) ;
#42048=ORIENTED_EDGE('',*,*,#29419,.F.) ;
#42049=ORIENTED_EDGE('',*,*,#29421,.T.) ;
#42050=ORIENTED_EDGE('',*,*,#29422,.F.) ;
#42051=ORIENTED_EDGE('',*,*,#28195,.T.) ;
#42052=ORIENTED_EDGE('',*,*,#29423,.T.) ;
#42053=ORIENTED_EDGE('',*,*,#29424,.T.) ;
#42054=ORIENTED_EDGE('',*,*,#29423,.F.) ;
#42055=ORIENTED_EDGE('',*,*,#28194,.T.) ;
#42056=ORIENTED_EDGE('',*,*,#29425,.T.) ;
#42057=ORIENTED_EDGE('',*,*,#29426,.T.) ;
#42058=ORIENTED_EDGE('',*,*,#29425,.F.) ;
#42059=ORIENTED_EDGE('',*,*,#28193,.T.) ;
#42060=ORIENTED_EDGE('',*,*,#29427,.T.) ;
#42061=ORIENTED_EDGE('',*,*,#29428,.T.) ;
#42062=ORIENTED_EDGE('',*,*,#29427,.F.) ;
#42063=ORIENTED_EDGE('',*,*,#28192,.T.) ;
#42064=ORIENTED_EDGE('',*,*,#29429,.T.) ;
#42065=ORIENTED_EDGE('',*,*,#29430,.T.) ;
#42066=ORIENTED_EDGE('',*,*,#29429,.F.) ;
#42067=ORIENTED_EDGE('',*,*,#28191,.T.) ;
#42068=ORIENTED_EDGE('',*,*,#29431,.T.) ;
#42069=ORIENTED_EDGE('',*,*,#29432,.T.) ;
#42070=ORIENTED_EDGE('',*,*,#29431,.F.) ;
#42071=ORIENTED_EDGE('',*,*,#28190,.T.) ;
#42072=ORIENTED_EDGE('',*,*,#29433,.T.) ;
#42073=ORIENTED_EDGE('',*,*,#29434,.T.) ;
#42074=ORIENTED_EDGE('',*,*,#29435,.F.) ;
#42075=ORIENTED_EDGE('',*,*,#28207,.T.) ;
#42076=ORIENTED_EDGE('',*,*,#29436,.T.) ;
#42077=ORIENTED_EDGE('',*,*,#29437,.T.) ;
#42078=ORIENTED_EDGE('',*,*,#29436,.F.) ;
#42079=ORIENTED_EDGE('',*,*,#28206,.T.) ;
#42080=ORIENTED_EDGE('',*,*,#29438,.T.) ;
#42081=ORIENTED_EDGE('',*,*,#29439,.T.) ;
#42082=ORIENTED_EDGE('',*,*,#29438,.F.) ;
#42083=ORIENTED_EDGE('',*,*,#28205,.T.) ;
#42084=ORIENTED_EDGE('',*,*,#29440,.T.) ;
#42085=ORIENTED_EDGE('',*,*,#29441,.T.) ;
#42086=ORIENTED_EDGE('',*,*,#29440,.F.) ;
#42087=ORIENTED_EDGE('',*,*,#28204,.T.) ;
#42088=ORIENTED_EDGE('',*,*,#29442,.T.) ;
#42089=ORIENTED_EDGE('',*,*,#27634,.F.) ;
#42090=ORIENTED_EDGE('',*,*,#29443,.T.) ;
#42091=ORIENTED_EDGE('',*,*,#29442,.F.) ;
#42092=ORIENTED_EDGE('',*,*,#28203,.T.) ;
#42093=ORIENTED_EDGE('',*,*,#29444,.T.) ;
#42094=ORIENTED_EDGE('',*,*,#27638,.F.) ;
#42095=ORIENTED_EDGE('',*,*,#28202,.T.) ;
#42096=ORIENTED_EDGE('',*,*,#29445,.T.) ;
#42097=ORIENTED_EDGE('',*,*,#29446,.T.) ;
#42098=ORIENTED_EDGE('',*,*,#29447,.F.) ;
#42099=ORIENTED_EDGE('',*,*,#28144,.T.) ;
#42100=ORIENTED_EDGE('',*,*,#29448,.T.) ;
#42101=ORIENTED_EDGE('',*,*,#29449,.T.) ;
#42102=ORIENTED_EDGE('',*,*,#29448,.F.) ;
#42103=ORIENTED_EDGE('',*,*,#28143,.T.) ;
#42104=ORIENTED_EDGE('',*,*,#29450,.F.) ;
#42105=ORIENTED_EDGE('',*,*,#27898,.T.) ;
#42106=ORIENTED_EDGE('',*,*,#29451,.T.) ;
#42107=ORIENTED_EDGE('',*,*,#29452,.T.) ;
#42108=ORIENTED_EDGE('',*,*,#29451,.F.) ;
#42109=ORIENTED_EDGE('',*,*,#27897,.F.) ;
#42110=ORIENTED_EDGE('',*,*,#29453,.T.) ;
#42111=ORIENTED_EDGE('',*,*,#29454,.T.) ;
#42112=ORIENTED_EDGE('',*,*,#29453,.F.) ;
#42113=ORIENTED_EDGE('',*,*,#27896,.T.) ;
#42114=ORIENTED_EDGE('',*,*,#29455,.T.) ;
#42115=ORIENTED_EDGE('',*,*,#29456,.T.) ;
#42116=ORIENTED_EDGE('',*,*,#29455,.F.) ;
#42117=ORIENTED_EDGE('',*,*,#27895,.F.) ;
#42118=ORIENTED_EDGE('',*,*,#28251,.T.) ;
#42119=ORIENTED_EDGE('',*,*,#29457,.T.) ;
#42120=ORIENTED_EDGE('',*,*,#29458,.F.) ;
#42121=ORIENTED_EDGE('',*,*,#28221,.T.) ;
#42122=ORIENTED_EDGE('',*,*,#29459,.T.) ;
#42123=ORIENTED_EDGE('',*,*,#29460,.T.) ;
#42124=ORIENTED_EDGE('',*,*,#29459,.F.) ;
#42125=ORIENTED_EDGE('',*,*,#28220,.T.) ;
#42126=ORIENTED_EDGE('',*,*,#29461,.T.) ;
#42127=ORIENTED_EDGE('',*,*,#29462,.T.) ;
#42128=ORIENTED_EDGE('',*,*,#29461,.F.) ;
#42129=ORIENTED_EDGE('',*,*,#28219,.T.) ;
#42130=ORIENTED_EDGE('',*,*,#29463,.T.) ;
#42131=ORIENTED_EDGE('',*,*,#29464,.T.) ;
#42132=ORIENTED_EDGE('',*,*,#29463,.F.) ;
#42133=ORIENTED_EDGE('',*,*,#28218,.T.) ;
#42134=ORIENTED_EDGE('',*,*,#29465,.T.) ;
#42135=ORIENTED_EDGE('',*,*,#29466,.T.) ;
#42136=ORIENTED_EDGE('',*,*,#29465,.F.) ;
#42137=ORIENTED_EDGE('',*,*,#28217,.T.) ;
#42138=ORIENTED_EDGE('',*,*,#29467,.T.) ;
#42139=ORIENTED_EDGE('',*,*,#29468,.T.) ;
#42140=ORIENTED_EDGE('',*,*,#29467,.F.) ;
#42141=ORIENTED_EDGE('',*,*,#28216,.T.) ;
#42142=ORIENTED_EDGE('',*,*,#29469,.T.) ;
#42143=ORIENTED_EDGE('',*,*,#29470,.T.) ;
#42144=ORIENTED_EDGE('',*,*,#29469,.F.) ;
#42145=ORIENTED_EDGE('',*,*,#28215,.T.) ;
#42146=ORIENTED_EDGE('',*,*,#29471,.T.) ;
#42147=ORIENTED_EDGE('',*,*,#29472,.T.) ;
#42148=ORIENTED_EDGE('',*,*,#29471,.F.) ;
#42149=ORIENTED_EDGE('',*,*,#28214,.T.) ;
#42150=ORIENTED_EDGE('',*,*,#29473,.T.) ;
#42151=ORIENTED_EDGE('',*,*,#29474,.T.) ;
#42152=ORIENTED_EDGE('',*,*,#29473,.F.) ;
#42153=ORIENTED_EDGE('',*,*,#28227,.T.) ;
#42154=ORIENTED_EDGE('',*,*,#29475,.T.) ;
#42155=ORIENTED_EDGE('',*,*,#29476,.T.) ;
#42156=ORIENTED_EDGE('',*,*,#29475,.F.) ;
#42157=ORIENTED_EDGE('',*,*,#28226,.T.) ;
#42158=ORIENTED_EDGE('',*,*,#29477,.T.) ;
#42159=ORIENTED_EDGE('',*,*,#29478,.T.) ;
#42160=ORIENTED_EDGE('',*,*,#29477,.F.) ;
#42161=ORIENTED_EDGE('',*,*,#28225,.T.) ;
#42162=ORIENTED_EDGE('',*,*,#29479,.T.) ;
#42163=ORIENTED_EDGE('',*,*,#29480,.T.) ;
#42164=ORIENTED_EDGE('',*,*,#29479,.F.) ;
#42165=ORIENTED_EDGE('',*,*,#28224,.T.) ;
#42166=ORIENTED_EDGE('',*,*,#29481,.T.) ;
#42167=ORIENTED_EDGE('',*,*,#29482,.T.) ;
#42168=ORIENTED_EDGE('',*,*,#29481,.F.) ;
#42169=ORIENTED_EDGE('',*,*,#28223,.T.) ;
#42170=ORIENTED_EDGE('',*,*,#29483,.T.) ;
#42171=ORIENTED_EDGE('',*,*,#29484,.T.) ;
#42172=ORIENTED_EDGE('',*,*,#29483,.F.) ;
#42173=ORIENTED_EDGE('',*,*,#28222,.T.) ;
#42174=ORIENTED_EDGE('',*,*,#29458,.T.) ;
#42175=ORIENTED_EDGE('',*,*,#29472,.F.) ;
#42176=ORIENTED_EDGE('',*,*,#29474,.F.) ;
#42177=ORIENTED_EDGE('',*,*,#29476,.F.) ;
#42178=ORIENTED_EDGE('',*,*,#29478,.F.) ;
#42179=ORIENTED_EDGE('',*,*,#29480,.F.) ;
#42180=ORIENTED_EDGE('',*,*,#29482,.F.) ;
#42181=ORIENTED_EDGE('',*,*,#29484,.F.) ;
#42182=ORIENTED_EDGE('',*,*,#29457,.F.) ;
#42183=ORIENTED_EDGE('',*,*,#29460,.F.) ;
#42184=ORIENTED_EDGE('',*,*,#29462,.F.) ;
#42185=ORIENTED_EDGE('',*,*,#29464,.F.) ;
#42186=ORIENTED_EDGE('',*,*,#29466,.F.) ;
#42187=ORIENTED_EDGE('',*,*,#29468,.F.) ;
#42188=ORIENTED_EDGE('',*,*,#29470,.F.) ;
#42189=ORIENTED_EDGE('',*,*,#29485,.T.) ;
#42190=ORIENTED_EDGE('',*,*,#29433,.F.) ;
#42191=ORIENTED_EDGE('',*,*,#28189,.T.) ;
#42192=ORIENTED_EDGE('',*,*,#29486,.T.) ;
#42193=ORIENTED_EDGE('',*,*,#29487,.T.) ;
#42194=ORIENTED_EDGE('',*,*,#29486,.F.) ;
#42195=ORIENTED_EDGE('',*,*,#28200,.T.) ;
#42196=ORIENTED_EDGE('',*,*,#29488,.T.) ;
#42197=ORIENTED_EDGE('',*,*,#29489,.T.) ;
#42198=ORIENTED_EDGE('',*,*,#29488,.F.) ;
#42199=ORIENTED_EDGE('',*,*,#28199,.T.) ;
#42200=ORIENTED_EDGE('',*,*,#29490,.T.) ;
#42201=ORIENTED_EDGE('',*,*,#29491,.T.) ;
#42202=ORIENTED_EDGE('',*,*,#29490,.F.) ;
#42203=ORIENTED_EDGE('',*,*,#28198,.T.) ;
#42204=ORIENTED_EDGE('',*,*,#29492,.T.) ;
#42205=ORIENTED_EDGE('',*,*,#29493,.T.) ;
#42206=ORIENTED_EDGE('',*,*,#29492,.F.) ;
#42207=ORIENTED_EDGE('',*,*,#28197,.T.) ;
#42208=ORIENTED_EDGE('',*,*,#29494,.T.) ;
#42209=ORIENTED_EDGE('',*,*,#29495,.T.) ;
#42210=ORIENTED_EDGE('',*,*,#29494,.F.) ;
#42211=ORIENTED_EDGE('',*,*,#28196,.T.) ;
#42212=ORIENTED_EDGE('',*,*,#29422,.T.) ;
#42213=ORIENTED_EDGE('',*,*,#29485,.F.) ;
#42214=ORIENTED_EDGE('',*,*,#29487,.F.) ;
#42215=ORIENTED_EDGE('',*,*,#29489,.F.) ;
#42216=ORIENTED_EDGE('',*,*,#29491,.F.) ;
#42217=ORIENTED_EDGE('',*,*,#29493,.F.) ;
#42218=ORIENTED_EDGE('',*,*,#29495,.F.) ;
#42219=ORIENTED_EDGE('',*,*,#29421,.F.) ;
#42220=ORIENTED_EDGE('',*,*,#29424,.F.) ;
#42221=ORIENTED_EDGE('',*,*,#29426,.F.) ;
#42222=ORIENTED_EDGE('',*,*,#29428,.F.) ;
#42223=ORIENTED_EDGE('',*,*,#29430,.F.) ;
#42224=ORIENTED_EDGE('',*,*,#29432,.F.) ;
#42225=ORIENTED_EDGE('',*,*,#29496,.T.) ;
#42226=ORIENTED_EDGE('',*,*,#29445,.F.) ;
#42227=ORIENTED_EDGE('',*,*,#28201,.T.) ;
#42228=ORIENTED_EDGE('',*,*,#29497,.T.) ;
#42229=ORIENTED_EDGE('',*,*,#29498,.T.) ;
#42230=ORIENTED_EDGE('',*,*,#29497,.F.) ;
#42231=ORIENTED_EDGE('',*,*,#28213,.T.) ;
#42232=ORIENTED_EDGE('',*,*,#29499,.T.) ;
#42233=ORIENTED_EDGE('',*,*,#29500,.T.) ;
#42234=ORIENTED_EDGE('',*,*,#29499,.F.) ;
#42235=ORIENTED_EDGE('',*,*,#28212,.T.) ;
#42236=ORIENTED_EDGE('',*,*,#29501,.T.) ;
#42237=ORIENTED_EDGE('',*,*,#29502,.T.) ;
#42238=ORIENTED_EDGE('',*,*,#29501,.F.) ;
#42239=ORIENTED_EDGE('',*,*,#28211,.T.) ;
#42240=ORIENTED_EDGE('',*,*,#29503,.T.) ;
#42241=ORIENTED_EDGE('',*,*,#29504,.T.) ;
#42242=ORIENTED_EDGE('',*,*,#29503,.F.) ;
#42243=ORIENTED_EDGE('',*,*,#28210,.T.) ;
#42244=ORIENTED_EDGE('',*,*,#29505,.T.) ;
#42245=ORIENTED_EDGE('',*,*,#29506,.T.) ;
#42246=ORIENTED_EDGE('',*,*,#29505,.F.) ;
#42247=ORIENTED_EDGE('',*,*,#28209,.T.) ;
#42248=ORIENTED_EDGE('',*,*,#29507,.T.) ;
#42249=ORIENTED_EDGE('',*,*,#29508,.T.) ;
#42250=ORIENTED_EDGE('',*,*,#29507,.F.) ;
#42251=ORIENTED_EDGE('',*,*,#28208,.T.) ;
#42252=ORIENTED_EDGE('',*,*,#29435,.T.) ;
#42253=ORIENTED_EDGE('',*,*,#27633,.T.) ;
#42254=ORIENTED_EDGE('',*,*,#27639,.F.) ;
#42255=ORIENTED_EDGE('',*,*,#29444,.F.) ;
#42256=ORIENTED_EDGE('',*,*,#29496,.F.) ;
#42257=ORIENTED_EDGE('',*,*,#29498,.F.) ;
#42258=ORIENTED_EDGE('',*,*,#29500,.F.) ;
#42259=ORIENTED_EDGE('',*,*,#29502,.F.) ;
#42260=ORIENTED_EDGE('',*,*,#29504,.F.) ;
#42261=ORIENTED_EDGE('',*,*,#29506,.F.) ;
#42262=ORIENTED_EDGE('',*,*,#29508,.F.) ;
#42263=ORIENTED_EDGE('',*,*,#29434,.F.) ;
#42264=ORIENTED_EDGE('',*,*,#29437,.F.) ;
#42265=ORIENTED_EDGE('',*,*,#29439,.F.) ;
#42266=ORIENTED_EDGE('',*,*,#29441,.F.) ;
#42267=ORIENTED_EDGE('',*,*,#29443,.F.) ;
#42268=ORIENTED_EDGE('',*,*,#29509,.T.) ;
#42269=ORIENTED_EDGE('',*,*,#29403,.F.) ;
#42270=ORIENTED_EDGE('',*,*,#28076,.T.) ;
#42271=ORIENTED_EDGE('',*,*,#29510,.T.) ;
#42272=ORIENTED_EDGE('',*,*,#29511,.T.) ;
#42273=ORIENTED_EDGE('',*,*,#29510,.F.) ;
#42274=ORIENTED_EDGE('',*,*,#28075,.T.) ;
#42275=ORIENTED_EDGE('',*,*,#29512,.T.) ;
#42276=ORIENTED_EDGE('',*,*,#29513,.T.) ;
#42277=ORIENTED_EDGE('',*,*,#29512,.F.) ;
#42278=ORIENTED_EDGE('',*,*,#28074,.T.) ;
#42279=ORIENTED_EDGE('',*,*,#29514,.T.) ;
#42280=ORIENTED_EDGE('',*,*,#29515,.T.) ;
#42281=ORIENTED_EDGE('',*,*,#29514,.F.) ;
#42282=ORIENTED_EDGE('',*,*,#28073,.T.) ;
#42283=ORIENTED_EDGE('',*,*,#29516,.T.) ;
#42284=ORIENTED_EDGE('',*,*,#29517,.T.) ;
#42285=ORIENTED_EDGE('',*,*,#29516,.F.) ;
#42286=ORIENTED_EDGE('',*,*,#28072,.T.) ;
#42287=ORIENTED_EDGE('',*,*,#29518,.T.) ;
#42288=ORIENTED_EDGE('',*,*,#29519,.T.) ;
#42289=ORIENTED_EDGE('',*,*,#29518,.F.) ;
#42290=ORIENTED_EDGE('',*,*,#28071,.T.) ;
#42291=ORIENTED_EDGE('',*,*,#29520,.T.) ;
#42292=ORIENTED_EDGE('',*,*,#29521,.T.) ;
#42293=ORIENTED_EDGE('',*,*,#29520,.F.) ;
#42294=ORIENTED_EDGE('',*,*,#28070,.T.) ;
#42295=ORIENTED_EDGE('',*,*,#29522,.T.) ;
#42296=ORIENTED_EDGE('',*,*,#29523,.T.) ;
#42297=ORIENTED_EDGE('',*,*,#29395,.F.) ;
#42298=ORIENTED_EDGE('',*,*,#29396,.F.) ;
#42299=ORIENTED_EDGE('',*,*,#29398,.F.) ;
#42300=ORIENTED_EDGE('',*,*,#29400,.F.) ;
#42301=ORIENTED_EDGE('',*,*,#29402,.F.) ;
#42302=ORIENTED_EDGE('',*,*,#29509,.F.) ;
#42303=ORIENTED_EDGE('',*,*,#29511,.F.) ;
#42304=ORIENTED_EDGE('',*,*,#29513,.F.) ;
#42305=ORIENTED_EDGE('',*,*,#29515,.F.) ;
#42306=ORIENTED_EDGE('',*,*,#29517,.F.) ;
#42307=ORIENTED_EDGE('',*,*,#29519,.F.) ;
#42308=ORIENTED_EDGE('',*,*,#29521,.F.) ;
#42309=ORIENTED_EDGE('',*,*,#29524,.F.) ;
#42310=ORIENTED_EDGE('',*,*,#29525,.T.) ;
#42311=ORIENTED_EDGE('',*,*,#29418,.F.) ;
#42312=ORIENTED_EDGE('',*,*,#28174,.T.) ;
#42313=ORIENTED_EDGE('',*,*,#29526,.T.) ;
#42314=ORIENTED_EDGE('',*,*,#29527,.T.) ;
#42315=ORIENTED_EDGE('',*,*,#29526,.F.) ;
#42316=ORIENTED_EDGE('',*,*,#28187,.T.) ;
#42317=ORIENTED_EDGE('',*,*,#29528,.T.) ;
#42318=ORIENTED_EDGE('',*,*,#29529,.T.) ;
#42319=ORIENTED_EDGE('',*,*,#29528,.F.) ;
#42320=ORIENTED_EDGE('',*,*,#28186,.T.) ;
#42321=ORIENTED_EDGE('',*,*,#29530,.T.) ;
#42322=ORIENTED_EDGE('',*,*,#29531,.T.) ;
#42323=ORIENTED_EDGE('',*,*,#29530,.F.) ;
#42324=ORIENTED_EDGE('',*,*,#28185,.T.) ;
#42325=ORIENTED_EDGE('',*,*,#29532,.T.) ;
#42326=ORIENTED_EDGE('',*,*,#29533,.T.) ;
#42327=ORIENTED_EDGE('',*,*,#29532,.F.) ;
#42328=ORIENTED_EDGE('',*,*,#28184,.T.) ;
#42329=ORIENTED_EDGE('',*,*,#29534,.T.) ;
#42330=ORIENTED_EDGE('',*,*,#29535,.T.) ;
#42331=ORIENTED_EDGE('',*,*,#29534,.F.) ;
#42332=ORIENTED_EDGE('',*,*,#28183,.T.) ;
#42333=ORIENTED_EDGE('',*,*,#29536,.T.) ;
#42334=ORIENTED_EDGE('',*,*,#29537,.T.) ;
#42335=ORIENTED_EDGE('',*,*,#29536,.F.) ;
#42336=ORIENTED_EDGE('',*,*,#28182,.T.) ;
#42337=ORIENTED_EDGE('',*,*,#29405,.T.) ;
#42338=ORIENTED_EDGE('',*,*,#29525,.F.) ;
#42339=ORIENTED_EDGE('',*,*,#29527,.F.) ;
#42340=ORIENTED_EDGE('',*,*,#29529,.F.) ;
#42341=ORIENTED_EDGE('',*,*,#29531,.F.) ;
#42342=ORIENTED_EDGE('',*,*,#29533,.F.) ;
#42343=ORIENTED_EDGE('',*,*,#29535,.F.) ;
#42344=ORIENTED_EDGE('',*,*,#29537,.F.) ;
#42345=ORIENTED_EDGE('',*,*,#29404,.F.) ;
#42346=ORIENTED_EDGE('',*,*,#29407,.F.) ;
#42347=ORIENTED_EDGE('',*,*,#29409,.F.) ;
#42348=ORIENTED_EDGE('',*,*,#29411,.F.) ;
#42349=ORIENTED_EDGE('',*,*,#29413,.F.) ;
#42350=ORIENTED_EDGE('',*,*,#29415,.F.) ;
#42351=ORIENTED_EDGE('',*,*,#29417,.F.) ;
#42352=ORIENTED_EDGE('',*,*,#29538,.T.) ;
#42353=ORIENTED_EDGE('',*,*,#28249,.F.) ;
#42354=ORIENTED_EDGE('',*,*,#28150,.T.) ;
#42355=ORIENTED_EDGE('',*,*,#29539,.T.) ;
#42356=ORIENTED_EDGE('',*,*,#29540,.T.) ;
#42357=ORIENTED_EDGE('',*,*,#29539,.F.) ;
#42358=ORIENTED_EDGE('',*,*,#28149,.T.) ;
#42359=ORIENTED_EDGE('',*,*,#29541,.T.) ;
#42360=ORIENTED_EDGE('',*,*,#29542,.T.) ;
#42361=ORIENTED_EDGE('',*,*,#29541,.F.) ;
#42362=ORIENTED_EDGE('',*,*,#28148,.T.) ;
#42363=ORIENTED_EDGE('',*,*,#29543,.T.) ;
#42364=ORIENTED_EDGE('',*,*,#29544,.T.) ;
#42365=ORIENTED_EDGE('',*,*,#29543,.F.) ;
#42366=ORIENTED_EDGE('',*,*,#28147,.T.) ;
#42367=ORIENTED_EDGE('',*,*,#29545,.T.) ;
#42368=ORIENTED_EDGE('',*,*,#29546,.T.) ;
#42369=ORIENTED_EDGE('',*,*,#29545,.F.) ;
#42370=ORIENTED_EDGE('',*,*,#28146,.T.) ;
#42371=ORIENTED_EDGE('',*,*,#29547,.T.) ;
#42372=ORIENTED_EDGE('',*,*,#29548,.T.) ;
#42373=ORIENTED_EDGE('',*,*,#29547,.F.) ;
#42374=ORIENTED_EDGE('',*,*,#28145,.T.) ;
#42375=ORIENTED_EDGE('',*,*,#29447,.T.) ;
#42376=ORIENTED_EDGE('',*,*,#29538,.F.) ;
#42377=ORIENTED_EDGE('',*,*,#29540,.F.) ;
#42378=ORIENTED_EDGE('',*,*,#29542,.F.) ;
#42379=ORIENTED_EDGE('',*,*,#29544,.F.) ;
#42380=ORIENTED_EDGE('',*,*,#29546,.F.) ;
#42381=ORIENTED_EDGE('',*,*,#29548,.F.) ;
#42382=ORIENTED_EDGE('',*,*,#29446,.F.) ;
#42383=ORIENTED_EDGE('',*,*,#29449,.F.) ;
#42384=ORIENTED_EDGE('',*,*,#29452,.F.) ;
#42385=ORIENTED_EDGE('',*,*,#29454,.F.) ;
#42386=ORIENTED_EDGE('',*,*,#29456,.F.) ;
#42387=ORIENTED_EDGE('',*,*,#28250,.F.) ;
#42388=ORIENTED_EDGE('',*,*,#29392,.F.) ;
#42389=ORIENTED_EDGE('',*,*,#29549,.T.) ;
#42390=ORIENTED_EDGE('',*,*,#29382,.F.) ;
#42391=ORIENTED_EDGE('',*,*,#28130,.F.) ;
#42392=ORIENTED_EDGE('',*,*,#29550,.T.) ;
#42393=ORIENTED_EDGE('',*,*,#29551,.T.) ;
#42394=ORIENTED_EDGE('',*,*,#29550,.F.) ;
#42395=ORIENTED_EDGE('',*,*,#28129,.T.) ;
#42396=ORIENTED_EDGE('',*,*,#29552,.T.) ;
#42397=ORIENTED_EDGE('',*,*,#29420,.F.) ;
#42398=ORIENTED_EDGE('',*,*,#29336,.F.) ;
#42399=ORIENTED_EDGE('',*,*,#29553,.F.) ;
#42400=ORIENTED_EDGE('',*,*,#28089,.T.) ;
#42401=ORIENTED_EDGE('',*,*,#29554,.T.) ;
#42402=ORIENTED_EDGE('',*,*,#29333,.F.) ;
#42403=ORIENTED_EDGE('',*,*,#29554,.F.) ;
#42404=ORIENTED_EDGE('',*,*,#28088,.T.) ;
#42405=ORIENTED_EDGE('',*,*,#29555,.F.) ;
#42406=ORIENTED_EDGE('',*,*,#29343,.F.) ;
#42407=ORIENTED_EDGE('',*,*,#29556,.F.) ;
#42408=ORIENTED_EDGE('',*,*,#29344,.F.) ;
#42409=ORIENTED_EDGE('',*,*,#29555,.T.) ;
#42410=ORIENTED_EDGE('',*,*,#28087,.T.) ;
#42411=ORIENTED_EDGE('',*,*,#29557,.F.) ;
#42412=ORIENTED_EDGE('',*,*,#29277,.F.) ;
#42413=ORIENTED_EDGE('',*,*,#29558,.F.) ;
#42414=ORIENTED_EDGE('',*,*,#28065,.T.) ;
#42415=ORIENTED_EDGE('',*,*,#29559,.F.) ;
#42416=ORIENTED_EDGE('',*,*,#29352,.F.) ;
#42417=ORIENTED_EDGE('',*,*,#27911,.F.) ;
#42418=ORIENTED_EDGE('',*,*,#28058,.F.) ;
#42419=ORIENTED_EDGE('',*,*,#28061,.F.) ;
#42420=ORIENTED_EDGE('',*,*,#28051,.F.) ;
#42421=ORIENTED_EDGE('',*,*,#28164,.F.) ;
#42422=ORIENTED_EDGE('',*,*,#29560,.F.) ;
#42423=ORIENTED_EDGE('',*,*,#28301,.F.) ;
#42424=ORIENTED_EDGE('',*,*,#27917,.T.) ;
#42425=ORIENTED_EDGE('',*,*,#28277,.F.) ;
#42426=ORIENTED_EDGE('',*,*,#29561,.T.) ;
#42427=ORIENTED_EDGE('',*,*,#28294,.F.) ;
#42428=ORIENTED_EDGE('',*,*,#28292,.F.) ;
#42429=ORIENTED_EDGE('',*,*,#28275,.F.) ;
#42430=ORIENTED_EDGE('',*,*,#29562,.T.) ;
#42431=ORIENTED_EDGE('',*,*,#28296,.F.) ;
#42432=ORIENTED_EDGE('',*,*,#29561,.F.) ;
#42433=ORIENTED_EDGE('',*,*,#28270,.F.) ;
#42434=ORIENTED_EDGE('',*,*,#29563,.T.) ;
#42435=ORIENTED_EDGE('',*,*,#28298,.F.) ;
#42436=ORIENTED_EDGE('',*,*,#29562,.F.) ;
#42437=ORIENTED_EDGE('',*,*,#28269,.F.) ;
#42438=ORIENTED_EDGE('',*,*,#28303,.F.) ;
#42439=ORIENTED_EDGE('',*,*,#29564,.T.) ;
#42440=ORIENTED_EDGE('',*,*,#28162,.F.) ;
#42441=ORIENTED_EDGE('',*,*,#28299,.T.) ;
#42442=ORIENTED_EDGE('',*,*,#28300,.T.) ;
#42443=ORIENTED_EDGE('',*,*,#29563,.F.) ;
#42444=ORIENTED_EDGE('',*,*,#28163,.F.) ;
#42445=ORIENTED_EDGE('',*,*,#29564,.F.) ;
#42446=ORIENTED_EDGE('',*,*,#28302,.F.) ;
#42447=ORIENTED_EDGE('',*,*,#29560,.T.) ;
#42448=ORIENTED_EDGE('',*,*,#29565,.T.) ;
#42449=ORIENTED_EDGE('',*,*,#29366,.F.) ;
#42450=ORIENTED_EDGE('',*,*,#29367,.F.) ;
#42451=ORIENTED_EDGE('',*,*,#29369,.F.) ;
#42452=ORIENTED_EDGE('',*,*,#29371,.F.) ;
#42453=ORIENTED_EDGE('',*,*,#29373,.F.) ;
#42454=ORIENTED_EDGE('',*,*,#29375,.F.) ;
#42455=ORIENTED_EDGE('',*,*,#29377,.F.) ;
#42456=ORIENTED_EDGE('',*,*,#29379,.F.) ;
#42457=ORIENTED_EDGE('',*,*,#29381,.F.) ;
#42458=ORIENTED_EDGE('',*,*,#29549,.F.) ;
#42459=ORIENTED_EDGE('',*,*,#29551,.F.) ;
#42460=ORIENTED_EDGE('',*,*,#29566,.F.) ;
#42461=ORIENTED_EDGE('',*,*,#29567,.T.) ;
#42462=ORIENTED_EDGE('',*,*,#29566,.T.) ;
#42463=ORIENTED_EDGE('',*,*,#29552,.F.) ;
#42464=ORIENTED_EDGE('',*,*,#28128,.F.) ;
#42465=ORIENTED_EDGE('',*,*,#27904,.F.) ;
#42466=ORIENTED_EDGE('',*,*,#27907,.T.) ;
#42467=ORIENTED_EDGE('',*,*,#28152,.F.) ;
#42468=ORIENTED_EDGE('',*,*,#28248,.F.) ;
#42469=ORIENTED_EDGE('',*,*,#28240,.T.) ;
#42470=ORIENTED_EDGE('',*,*,#27901,.T.) ;
#42471=ORIENTED_EDGE('',*,*,#29568,.T.) ;
#42472=ORIENTED_EDGE('',*,*,#28140,.F.) ;
#42473=ORIENTED_EDGE('',*,*,#29364,.F.) ;
#42474=ORIENTED_EDGE('',*,*,#29565,.F.) ;
#42475=ORIENTED_EDGE('',*,*,#29567,.F.) ;
#42476=ORIENTED_EDGE('',*,*,#28127,.T.) ;
#42477=ORIENTED_EDGE('',*,*,#28234,.F.) ;
#42478=ORIENTED_EDGE('',*,*,#28141,.F.) ;
#42479=ORIENTED_EDGE('',*,*,#29568,.F.) ;
#42480=ORIENTED_EDGE('',*,*,#27900,.F.) ;
#42481=ORIENTED_EDGE('',*,*,#29569,.T.) ;
#42482=ORIENTED_EDGE('',*,*,#28142,.F.) ;
#42483=ORIENTED_EDGE('',*,*,#29569,.F.) ;
#42484=ORIENTED_EDGE('',*,*,#27899,.T.) ;
#42485=ORIENTED_EDGE('',*,*,#29450,.T.) ;
#42486=ORIENTED_EDGE('',*,*,#29220,.F.) ;
#42487=ORIENTED_EDGE('',*,*,#28244,.T.) ;
#42488=ORIENTED_EDGE('',*,*,#28238,.F.) ;
#42489=ORIENTED_EDGE('',*,*,#28123,.T.) ;
#42490=ORIENTED_EDGE('',*,*,#29570,.T.) ;
#42491=ORIENTED_EDGE('',*,*,#29570,.F.) ;
#42492=ORIENTED_EDGE('',*,*,#28122,.F.) ;
#42493=ORIENTED_EDGE('',*,*,#28038,.F.) ;
#42494=ORIENTED_EDGE('',*,*,#29221,.F.) ;
#42495=ORIENTED_EDGE('',*,*,#29330,.F.) ;
#42496=ORIENTED_EDGE('',*,*,#29571,.F.) ;
#42497=ORIENTED_EDGE('',*,*,#28085,.F.) ;
#42498=ORIENTED_EDGE('',*,*,#29362,.T.) ;
#42499=ORIENTED_EDGE('',*,*,#29341,.F.) ;
#42500=ORIENTED_EDGE('',*,*,#29557,.T.) ;
#42501=ORIENTED_EDGE('',*,*,#28086,.T.) ;
#42502=ORIENTED_EDGE('',*,*,#29571,.T.) ;
#42503=ORIENTED_EDGE('',*,*,#29339,.F.) ;
#42504=ORIENTED_EDGE('',*,*,#27788,.F.) ;
#42505=ORIENTED_EDGE('',*,*,#29348,.F.) ;
#42506=ORIENTED_EDGE('',*,*,#29572,.F.) ;
#42507=ORIENTED_EDGE('',*,*,#28063,.T.) ;
#42508=ORIENTED_EDGE('',*,*,#27778,.T.) ;
#42509=ORIENTED_EDGE('',*,*,#27786,.T.) ;
#42510=ORIENTED_EDGE('',*,*,#29350,.F.) ;
#42511=ORIENTED_EDGE('',*,*,#29559,.T.) ;
#42512=ORIENTED_EDGE('',*,*,#28064,.T.) ;
#42513=ORIENTED_EDGE('',*,*,#29572,.T.) ;
#42514=ORIENTED_EDGE('',*,*,#29334,.F.) ;
#42515=ORIENTED_EDGE('',*,*,#29556,.T.) ;
#42516=ORIENTED_EDGE('',*,*,#29345,.F.) ;
#42517=ORIENTED_EDGE('',*,*,#29342,.F.) ;
#42518=ORIENTED_EDGE('',*,*,#29285,.F.) ;
#42519=ORIENTED_EDGE('',*,*,#27515,.F.) ;
#42520=ORIENTED_EDGE('',*,*,#27519,.F.) ;
#42521=ORIENTED_EDGE('',*,*,#29338,.F.) ;
#42522=ORIENTED_EDGE('',*,*,#29328,.F.) ;
#42523=ORIENTED_EDGE('',*,*,#29361,.F.) ;
#42524=ORIENTED_EDGE('',*,*,#28091,.T.) ;
#42525=ORIENTED_EDGE('',*,*,#29573,.F.) ;
#42526=ORIENTED_EDGE('',*,*,#27521,.F.) ;
#42527=ORIENTED_EDGE('',*,*,#27526,.F.) ;
#42528=ORIENTED_EDGE('',*,*,#27522,.F.) ;
#42529=ORIENTED_EDGE('',*,*,#29573,.T.) ;
#42530=ORIENTED_EDGE('',*,*,#28090,.T.) ;
#42531=ORIENTED_EDGE('',*,*,#29553,.T.) ;
#42532=ORIENTED_EDGE('',*,*,#29337,.F.) ;
#42533=ORIENTED_EDGE('',*,*,#28635,.F.) ;
#42534=ORIENTED_EDGE('',*,*,#29574,.T.) ;
#42535=ORIENTED_EDGE('',*,*,#29390,.F.) ;
#42536=ORIENTED_EDGE('',*,*,#29574,.F.) ;
#42537=ORIENTED_EDGE('',*,*,#29575,.T.) ;
#42538=ORIENTED_EDGE('',*,*,#29524,.T.) ;
#42539=ORIENTED_EDGE('',*,*,#29522,.F.) ;
#42540=ORIENTED_EDGE('',*,*,#28069,.T.) ;
#42541=ORIENTED_EDGE('',*,*,#29283,.F.) ;
#42542=ORIENTED_EDGE('',*,*,#29576,.T.) ;
#42543=ORIENTED_EDGE('',*,*,#28066,.F.) ;
#42544=ORIENTED_EDGE('',*,*,#29558,.T.) ;
#42545=ORIENTED_EDGE('',*,*,#29304,.F.) ;
#42546=ORIENTED_EDGE('',*,*,#29363,.F.) ;
#42547=ORIENTED_EDGE('',*,*,#28083,.F.) ;
#42548=ORIENTED_EDGE('',*,*,#29577,.T.) ;
#42549=ORIENTED_EDGE('',*,*,#29307,.F.) ;
#42550=ORIENTED_EDGE('',*,*,#29577,.F.) ;
#42551=ORIENTED_EDGE('',*,*,#28082,.F.) ;
#42552=ORIENTED_EDGE('',*,*,#29393,.F.) ;
#42553=ORIENTED_EDGE('',*,*,#29523,.F.) ;
#42554=ORIENTED_EDGE('',*,*,#29575,.F.) ;
#42555=ORIENTED_EDGE('',*,*,#28068,.F.) ;
#42556=ORIENTED_EDGE('',*,*,#29578,.T.) ;
#42557=ORIENTED_EDGE('',*,*,#29291,.F.) ;
#42558=ORIENTED_EDGE('',*,*,#29286,.F.) ;
#42559=ORIENTED_EDGE('',*,*,#29308,.F.) ;
#42560=ORIENTED_EDGE('',*,*,#29302,.F.) ;
#42561=ORIENTED_EDGE('',*,*,#29292,.F.) ;
#42562=ORIENTED_EDGE('',*,*,#29578,.F.) ;
#42563=ORIENTED_EDGE('',*,*,#28067,.F.) ;
#42564=ORIENTED_EDGE('',*,*,#29576,.F.) ;
#42565=ORIENTED_EDGE('',*,*,#29314,.F.) ;
#42566=ORIENTED_EDGE('',*,*,#29579,.F.) ;
#42567=ORIENTED_EDGE('',*,*,#28093,.F.) ;
#42568=ORIENTED_EDGE('',*,*,#29360,.F.) ;
#42569=ORIENTED_EDGE('',*,*,#29321,.F.) ;
#42570=ORIENTED_EDGE('',*,*,#29355,.F.) ;
#42571=ORIENTED_EDGE('',*,*,#28094,.F.) ;
#42572=ORIENTED_EDGE('',*,*,#29579,.T.) ;
#42573=ORIENTED_EDGE('',*,*,#29313,.F.) ;
#42574=ORIENTED_EDGE('',*,*,#29309,.F.) ;
#42575=ORIENTED_EDGE('',*,*,#29322,.F.) ;
#42576=ORIENTED_EDGE('',*,*,#29316,.F.) ;
#42577=ORIENTED_EDGE('',*,*,#28369,.T.) ;
#42578=ORIENTED_EDGE('',*,*,#29580,.F.) ;
#42579=ORIENTED_EDGE('',*,*,#28423,.F.) ;
#42580=ORIENTED_EDGE('',*,*,#28434,.F.) ;
#42581=ORIENTED_EDGE('',*,*,#29272,.F.) ;
#42582=ORIENTED_EDGE('',*,*,#29273,.F.) ;
#42583=ORIENTED_EDGE('',*,*,#28379,.T.) ;
#42584=ORIENTED_EDGE('',*,*,#29581,.F.) ;
#42585=ORIENTED_EDGE('',*,*,#28370,.F.) ;
#42586=ORIENTED_EDGE('',*,*,#29581,.T.) ;
#42587=ORIENTED_EDGE('',*,*,#28381,.F.) ;
#42588=ORIENTED_EDGE('',*,*,#28359,.F.) ;
#42589=ORIENTED_EDGE('',*,*,#28357,.F.) ;
#42590=ORIENTED_EDGE('',*,*,#28407,.F.) ;
#42591=ORIENTED_EDGE('',*,*,#29274,.F.) ;
#42592=ORIENTED_EDGE('',*,*,#28440,.T.) ;
#42593=ORIENTED_EDGE('',*,*,#28417,.F.) ;
#42594=ORIENTED_EDGE('',*,*,#29244,.T.) ;
#42595=ORIENTED_EDGE('',*,*,#29246,.T.) ;
#42596=ORIENTED_EDGE('',*,*,#29384,.T.) ;
#42597=ORIENTED_EDGE('',*,*,#29386,.T.) ;
#42598=ORIENTED_EDGE('',*,*,#29387,.T.) ;
#42599=ORIENTED_EDGE('',*,*,#29249,.T.) ;
#42600=ORIENTED_EDGE('',*,*,#29359,.T.) ;
#42601=ORIENTED_EDGE('',*,*,#28504,.T.) ;
#42602=ORIENTED_EDGE('',*,*,#29256,.T.) ;
#42603=ORIENTED_EDGE('',*,*,#27849,.T.) ;
#42604=ORIENTED_EDGE('',*,*,#28361,.F.) ;
#42605=ORIENTED_EDGE('',*,*,#28424,.F.) ;
#42606=ORIENTED_EDGE('',*,*,#29580,.T.) ;
#42607=ORIENTED_EDGE('',*,*,#28371,.F.) ;
#45715=TOROIDAL_SURFACE('',#52557,0.48,0.24) ;
#45716=TOROIDAL_SURFACE('',#52583,0.48,0.24) ;
#45717=TOROIDAL_SURFACE('',#52659,0.14,0.1) ;
#45718=TOROIDAL_SURFACE('',#52669,0.14,0.1) ;
#45719=TOROIDAL_SURFACE('',#52677,0.2,0.1) ;
#45720=TOROIDAL_SURFACE('',#52681,0.45,0.3) ;
#45721=TOROIDAL_SURFACE('',#52685,0.2,0.1) ;
#45722=TOROIDAL_SURFACE('',#52691,0.45,0.3) ;
#45723=TOROIDAL_SURFACE('',#52709,4.09999999999997,0.1) ;
#45724=TOROIDAL_SURFACE('',#52715,0.9,0.1) ;
#45725=TOROIDAL_SURFACE('',#52719,0.700000000000129,0.1) ;
#45726=TOROIDAL_SURFACE('',#52725,0.500000000000129,0.1) ;
#45727=TOROIDAL_SURFACE('',#52732,0.2,0.1) ;
#45728=TOROIDAL_SURFACE('',#52754,0.200000000000002,0.100000000000002) ;
#45729=TOROIDAL_SURFACE('',#52761,0.800000000000003,0.1) ;
#45730=TOROIDAL_SURFACE('',#52773,3.79999999999997,0.1) ;
#45731=TOROIDAL_SURFACE('',#52779,3.79999999999982,0.1) ;
#45732=TOROIDAL_SURFACE('',#52784,0.65,0.1) ;
#45733=TOROIDAL_SURFACE('',#52790,0.65,0.1) ;
#45734=TOROIDAL_SURFACE('',#52826,1.9,0.1) ;
#45735=TOROIDAL_SURFACE('',#52838,0.2,0.1) ;
#45736=TOROIDAL_SURFACE('',#52854,0.199999999999969,0.0999999999999847) ;
#45737=TOROIDAL_SURFACE('',#52931,3.,0.1) ;
#45738=TOROIDAL_SURFACE('',#52933,4.09999999999997,0.1) ;
#45739=TOROIDAL_SURFACE('',#52949,0.699999999999915,0.1) ;
#45740=TOROIDAL_SURFACE('',#52955,0.9,0.1) ;
#45741=TOROIDAL_SURFACE('',#52962,0.600000000000114,0.1) ;
#45742=TOROIDAL_SURFACE('',#52971,1.1,0.1) ;
#45743=TOROIDAL_SURFACE('',#52978,0.3999999999999,0.1) ;
#45744=TOROIDAL_SURFACE('',#52985,0.400000000000114,0.1) ;
#45745=TOROIDAL_SURFACE('',#53015,0.200000000000031,0.100000000000016) ;
#45746=TOROIDAL_SURFACE('',#53022,0.6,0.1) ;
#45747=TOROIDAL_SURFACE('',#53025,0.200000000000031,0.0999999999999979) ;
#45748=TOROIDAL_SURFACE('',#53032,0.6,0.1) ;
#45749=TOROIDAL_SURFACE('',#53045,0.299999999999996,0.1) ;
#45750=TOROIDAL_SURFACE('',#53050,0.300000000000031,0.1) ;
#45751=TOROIDAL_SURFACE('',#53058,0.3,0.1) ;
#45752=TOROIDAL_SURFACE('',#53064,0.300000000000031,0.1) ;
#45753=TOROIDAL_SURFACE('',#53070,0.3,0.1) ;
#45754=TOROIDAL_SURFACE('',#53076,0.3,0.1) ;
#45755=TOROIDAL_SURFACE('',#53110,0.199999999999996,0.0999999999999979) ;
#45756=TOROIDAL_SURFACE('',#53115,0.199999999999996,0.0999999999999979) ;
#45757=TOROIDAL_SURFACE('',#53124,0.400000000000007,0.1) ;
#45758=TOROIDAL_SURFACE('',#53135,0.400000000000007,0.1) ;
#45759=TOROIDAL_SURFACE('',#53157,0.699999999999915,0.1) ;
#45760=TOROIDAL_SURFACE('',#53162,0.9,0.1) ;
#45761=TOROIDAL_SURFACE('',#53167,0.6,0.1) ;
#45762=TOROIDAL_SURFACE('',#53172,0.65,0.1) ;
#45763=TOROIDAL_SURFACE('',#53177,0.85,0.1) ;
#45764=TOROIDAL_SURFACE('',#53191,1.1,0.1) ;
#45765=TOROIDAL_SURFACE('',#53195,0.500000000000129,0.1) ;
#45766=TOROIDAL_SURFACE('',#53200,0.700000000000129,0.1) ;
#45767=TOROIDAL_SURFACE('',#53203,0.9,0.1) ;
#45768=TOROIDAL_SURFACE('',#53208,4.09999999999997,0.1) ;
#45769=TOROIDAL_SURFACE('',#53212,1.40000000000004,0.1) ;
#45770=TOROIDAL_SURFACE('',#53228,1.4,0.1) ;
#45771=TOROIDAL_SURFACE('',#53232,0.400000000000007,0.1) ;
#45772=TOROIDAL_SURFACE('',#53237,0.65,0.1) ;
#45773=TOROIDAL_SURFACE('',#53242,0.6,0.1) ;
#45774=TOROIDAL_SURFACE('',#53246,0.4,0.1) ;
#45775=TOROIDAL_SURFACE('',#53254,0.400000000000043,0.1) ;
#45776=TOROIDAL_SURFACE('',#53260,0.400000000000007,0.1) ;
#45777=TOROIDAL_SURFACE('',#53265,0.3,0.1) ;
#45778=TOROIDAL_SURFACE('',#53298,0.65,0.1) ;
#45779=TOROIDAL_SURFACE('',#53399,3.79999999999997,0.1) ;
#45780=TOROIDAL_SURFACE('',#53404,1.40000000000004,0.1) ;
#45781=TOROIDAL_SURFACE('',#53506,0.599999999999972,0.1) ;
#45782=TOROIDAL_SURFACE('',#53516,0.399999999999963,0.1) ;
#45783=TOROIDAL_SURFACE('',#53538,0.599999999999972,0.1) ;
#45784=TOROIDAL_SURFACE('',#53548,0.399999999999963,0.1) ;
#45785=TOROIDAL_SURFACE('',#53656,0.199999999999963,0.1) ;
#45786=TOROIDAL_SURFACE('',#53659,0.799999999999972,0.1) ;
#45787=TOROIDAL_SURFACE('',#53682,0.799999999999972,0.1) ;
#45788=TOROIDAL_SURFACE('',#53688,0.199999999999963,0.1) ;
#45789=TOROIDAL_SURFACE('',#53755,4.56491106406736,0.5) ;
#45790=TOROIDAL_SURFACE('',#53761,4.55,0.5) ;
#45791=TOROIDAL_SURFACE('',#53772,4.56491106406736,0.5) ;
#45792=TOROIDAL_SURFACE('',#53779,4.55,0.5) ;
#45793=TOROIDAL_SURFACE('',#53784,4.55,0.5) ;
#45794=TOROIDAL_SURFACE('',#53792,4.55,0.5) ;
#45795=TOROIDAL_SURFACE('',#53798,4.56491106406736,0.5) ;
#45796=TOROIDAL_SURFACE('',#53805,4.56491106406736,0.5) ;
#47600=ADVANCED_FACE('',(#12382),#2005,.T.) ;
#47601=ADVANCED_FACE('',(#12383),#2006,.T.) ;
#47602=ADVANCED_FACE('',(#12384),#2007,.T.) ;
#47603=ADVANCED_FACE('',(#12385),#2008,.T.) ;
#47604=ADVANCED_FACE('',(#12386),#2009,.T.) ;
#47605=ADVANCED_FACE('',(#12387),#2563,.F.) ;
#47606=ADVANCED_FACE('',(#12388),#2010,.F.) ;
#47607=ADVANCED_FACE('',(#12389),#2011,.F.) ;
#47608=ADVANCED_FACE('',(#12390),#2012,.F.) ;
#47609=ADVANCED_FACE('',(#12391),#2013,.F.) ;
#47610=ADVANCED_FACE('',(#12392),#2014,.F.) ;
#47611=ADVANCED_FACE('',(#12393),#2564,.F.) ;
#47612=ADVANCED_FACE('',(#12394),#2565,.F.) ;
#47613=ADVANCED_FACE('',(#12395),#2566,.F.) ;
#47614=ADVANCED_FACE('',(#12396),#2567,.F.) ;
#47615=ADVANCED_FACE('',(#12397),#2015,.F.) ;
#47616=ADVANCED_FACE('',(#12398),#2016,.F.) ;
#47617=ADVANCED_FACE('',(#12399),#2017,.F.) ;
#47618=ADVANCED_FACE('',(#12400),#2018,.F.) ;
#47619=ADVANCED_FACE('',(#12401),#2568,.F.) ;
#47620=ADVANCED_FACE('',(#12402),#2569,.F.) ;
#47621=ADVANCED_FACE('',(#12403),#2570,.F.) ;
#47622=ADVANCED_FACE('',(#12404),#2019,.F.) ;
#47623=ADVANCED_FACE('',(#12405),#2020,.F.) ;
#47624=ADVANCED_FACE('',(#12406),#2021,.F.) ;
#47625=ADVANCED_FACE('',(#12407),#2022,.F.) ;
#47626=ADVANCED_FACE('',(#12408),#2023,.F.) ;
#47627=ADVANCED_FACE('',(#12409),#2024,.F.) ;
#47628=ADVANCED_FACE('',(#12410),#2025,.F.) ;
#47629=ADVANCED_FACE('',(#12411),#2571,.F.) ;
#47630=ADVANCED_FACE('',(#12412),#2572,.F.) ;
#47631=ADVANCED_FACE('',(#12413),#2573,.F.) ;
#47632=ADVANCED_FACE('',(#12414,#738),#2574,.T.) ;
#47633=ADVANCED_FACE('',(#12415,#739,#740),#2575,.T.) ;
#47634=ADVANCED_FACE('',(#12416),#2026,.T.) ;
#47635=ADVANCED_FACE('',(#12417),#2027,.T.) ;
#47636=ADVANCED_FACE('',(#12418),#45715,.T.) ;
#47637=ADVANCED_FACE('',(#12419),#10134,.T.) ;
#47638=ADVANCED_FACE('',(#12420),#97,.F.) ;
#47639=ADVANCED_FACE('',(#12421),#10135,.T.) ;
#47640=ADVANCED_FACE('',(#12422),#2028,.F.) ;
#47641=ADVANCED_FACE('',(#12423),#2576,.F.) ;
#47642=ADVANCED_FACE('',(#12424),#10136,.T.) ;
#47643=ADVANCED_FACE('',(#12425),#2577,.T.) ;
#47644=ADVANCED_FACE('',(#12426),#2029,.F.) ;
#47645=ADVANCED_FACE('',(#12427),#10137,.T.) ;
#47646=ADVANCED_FACE('',(#12428),#98,.F.) ;
#47647=ADVANCED_FACE('',(#12429),#10138,.T.) ;
#47648=ADVANCED_FACE('',(#12430),#45716,.T.) ;
#47649=ADVANCED_FACE('',(#12431),#2578,.T.) ;
#47650=ADVANCED_FACE('',(#12432),#10139,.T.) ;
#47651=ADVANCED_FACE('',(#12433),#2579,.T.) ;
#47652=ADVANCED_FACE('',(#12434),#2030,.F.) ;
#47653=ADVANCED_FACE('',(#12435),#2580,.T.) ;
#47654=ADVANCED_FACE('',(#12436),#2581,.T.) ;
#47655=ADVANCED_FACE('',(#12437),#2031,.T.) ;
#47656=ADVANCED_FACE('',(#12438),#10140,.F.) ;
#47657=ADVANCED_FACE('',(#12439),#2032,.T.) ;
#47658=ADVANCED_FACE('',(#12440),#2033,.T.) ;
#47659=ADVANCED_FACE('',(#12441),#10141,.T.) ;
#47660=ADVANCED_FACE('',(#12442),#2582,.F.) ;
#47661=ADVANCED_FACE('',(#12443),#10142,.T.) ;
#47662=ADVANCED_FACE('',(#12444),#2034,.T.) ;
#47663=ADVANCED_FACE('',(#12445),#10143,.F.) ;
#47664=ADVANCED_FACE('',(#12446),#2035,.T.) ;
#47665=ADVANCED_FACE('',(#12447),#2036,.T.) ;
#47666=ADVANCED_FACE('',(#12448),#2583,.F.) ;
#47667=ADVANCED_FACE('',(#12449),#10144,.T.) ;
#47668=ADVANCED_FACE('',(#12450),#10145,.T.) ;
#47669=ADVANCED_FACE('',(#12451),#2037,.F.) ;
#47670=ADVANCED_FACE('',(#12452),#10146,.T.) ;
#47671=ADVANCED_FACE('',(#12453),#10147,.T.) ;
#47672=ADVANCED_FACE('',(#12454),#2584,.T.) ;
#47673=ADVANCED_FACE('',(#12455),#2585,.T.) ;
#47674=ADVANCED_FACE('',(#12456),#2586,.T.) ;
#47675=ADVANCED_FACE('',(#12457),#10148,.T.) ;
#47676=ADVANCED_FACE('',(#12458),#10149,.F.) ;
#47677=ADVANCED_FACE('',(#12459),#2587,.T.) ;
#47678=ADVANCED_FACE('',(#12460),#2038,.T.) ;
#47679=ADVANCED_FACE('',(#12461),#10150,.F.) ;
#47680=ADVANCED_FACE('',(#12462),#2588,.T.) ;
#47681=ADVANCED_FACE('',(#12463),#10151,.F.) ;
#47682=ADVANCED_FACE('',(#12464),#2589,.F.) ;
#47683=ADVANCED_FACE('',(#12465),#45717,.T.) ;
#47684=ADVANCED_FACE('',(#12466),#10152,.T.) ;
#47685=ADVANCED_FACE('',(#12467),#10153,.T.) ;
#47686=ADVANCED_FACE('',(#12468),#2590,.T.) ;
#47687=ADVANCED_FACE('',(#12469),#45718,.T.) ;
#47688=ADVANCED_FACE('',(#12470),#10154,.T.) ;
#47689=ADVANCED_FACE('',(#12471),#10155,.T.) ;
#47690=ADVANCED_FACE('',(#12472),#45719,.T.) ;
#47691=ADVANCED_FACE('',(#12473),#45720,.T.) ;
#47692=ADVANCED_FACE('',(#12474),#10156,.T.) ;
#47693=ADVANCED_FACE('',(#12475),#45721,.T.) ;
#47694=ADVANCED_FACE('',(#12476),#10157,.T.) ;
#47695=ADVANCED_FACE('',(#12477),#45722,.T.) ;
#47696=ADVANCED_FACE('',(#12478),#10158,.T.) ;
#47697=ADVANCED_FACE('',(#12479),#2591,.T.) ;
#47698=ADVANCED_FACE('',(#12480),#10159,.T.) ;
#47699=ADVANCED_FACE('',(#12481),#2592,.T.) ;
#47700=ADVANCED_FACE('',(#12482),#10160,.T.) ;
#47701=ADVANCED_FACE('',(#12483),#2211,.T.) ;
#47702=ADVANCED_FACE('',(#12484),#10161,.T.) ;
#47703=ADVANCED_FACE('',(#12485),#45723,.T.) ;
#47704=ADVANCED_FACE('',(#12486),#10162,.T.) ;
#47705=ADVANCED_FACE('',(#12487),#45724,.T.) ;
#47706=ADVANCED_FACE('',(#12488),#45725,.T.) ;
#47707=ADVANCED_FACE('',(#12489),#10163,.T.) ;
#47708=ADVANCED_FACE('',(#12490),#45726,.T.) ;
#47709=ADVANCED_FACE('',(#12491),#10164,.T.) ;
#47710=ADVANCED_FACE('',(#12492),#10165,.T.) ;
#47711=ADVANCED_FACE('',(#12493),#45727,.T.) ;
#47712=ADVANCED_FACE('',(#12494),#2593,.F.) ;
#47713=ADVANCED_FACE('',(#12495),#10166,.T.) ;
#47714=ADVANCED_FACE('',(#12496),#2594,.T.) ;
#47715=ADVANCED_FACE('',(#12497),#10167,.F.) ;
#47716=ADVANCED_FACE('',(#12498),#2039,.T.) ;
#47717=ADVANCED_FACE('',(#12499),#10168,.T.) ;
#47718=ADVANCED_FACE('',(#12500),#10169,.F.) ;
#47719=ADVANCED_FACE('',(#12501),#2040,.T.) ;
#47720=ADVANCED_FACE('',(#12502),#2595,.T.) ;
#47721=ADVANCED_FACE('',(#12503),#45728,.T.) ;
#47722=ADVANCED_FACE('',(#12504),#10170,.T.) ;
#47723=ADVANCED_FACE('',(#12505),#45729,.T.) ;
#47724=ADVANCED_FACE('',(#12506),#10171,.F.) ;
#47725=ADVANCED_FACE('',(#12507),#2041,.T.) ;
#47726=ADVANCED_FACE('',(#12508),#2042,.T.) ;
#47727=ADVANCED_FACE('',(#12509),#10172,.F.) ;
#47728=ADVANCED_FACE('',(#12510),#2043,.T.) ;
#47729=ADVANCED_FACE('',(#12511),#45730,.T.) ;
#47730=ADVANCED_FACE('',(#12512),#10173,.T.) ;
#47731=ADVANCED_FACE('',(#12513),#45731,.T.) ;
#47732=ADVANCED_FACE('',(#12514),#10174,.T.) ;
#47733=ADVANCED_FACE('',(#12515),#45732,.T.) ;
#47734=ADVANCED_FACE('',(#12516),#10175,.T.) ;
#47735=ADVANCED_FACE('',(#12517),#45733,.T.) ;
#47736=ADVANCED_FACE('',(#12518),#10176,.F.) ;
#47737=ADVANCED_FACE('',(#12519),#2596,.T.) ;
#47738=ADVANCED_FACE('',(#12520),#10177,.T.) ;
#47739=ADVANCED_FACE('',(#12521),#2597,.T.) ;
#47740=ADVANCED_FACE('',(#12522),#10178,.T.) ;
#47741=ADVANCED_FACE('',(#12523),#10179,.T.) ;
#47742=ADVANCED_FACE('',(#12524),#2044,.T.) ;
#47743=ADVANCED_FACE('',(#12525),#2045,.T.) ;
#47744=ADVANCED_FACE('',(#12526),#10180,.F.) ;
#47745=ADVANCED_FACE('',(#12527),#2046,.T.) ;
#47746=ADVANCED_FACE('',(#12528),#2047,.T.) ;
#47747=ADVANCED_FACE('',(#12529),#2048,.T.) ;
#47748=ADVANCED_FACE('',(#12530),#10181,.T.) ;
#47749=ADVANCED_FACE('',(#12531),#2598,.T.) ;
#47750=ADVANCED_FACE('',(#12532),#2599,.F.) ;
#47751=ADVANCED_FACE('',(#12533),#10182,.T.) ;
#47752=ADVANCED_FACE('',(#12534),#10183,.T.) ;
#47753=ADVANCED_FACE('',(#12535),#45734,.T.) ;
#47754=ADVANCED_FACE('',(#12536),#10184,.T.) ;
#47755=ADVANCED_FACE('',(#12537),#10185,.T.) ;
#47756=ADVANCED_FACE('',(#12538),#10186,.T.) ;
#47757=ADVANCED_FACE('',(#12539),#2600,.F.) ;
#47758=ADVANCED_FACE('',(#12540),#2601,.T.) ;
#47759=ADVANCED_FACE('',(#12541),#2049,.T.) ;
#47760=ADVANCED_FACE('',(#12542),#45735,.F.) ;
#47761=ADVANCED_FACE('',(#12543),#10187,.F.) ;
#47762=ADVANCED_FACE('',(#12544),#2602,.T.) ;
#47763=ADVANCED_FACE('',(#12545),#10188,.T.) ;
#47764=ADVANCED_FACE('',(#12546),#10189,.T.) ;
#47765=ADVANCED_FACE('',(#12547),#2212,.F.) ;
#47766=ADVANCED_FACE('',(#12548),#10190,.F.) ;
#47767=ADVANCED_FACE('',(#12549),#10191,.F.) ;
#47768=ADVANCED_FACE('',(#12550),#45736,.T.) ;
#47769=ADVANCED_FACE('',(#12551),#10192,.T.) ;
#47770=ADVANCED_FACE('',(#12552),#10193,.T.) ;
#47771=ADVANCED_FACE('',(#12553),#10194,.F.) ;
#47772=ADVANCED_FACE('',(#12554,#741,#742,#743,#744,#745,#746,#747),#2603,
 .F.) ;
#47773=ADVANCED_FACE('',(#12555),#2604,.T.) ;
#47774=ADVANCED_FACE('',(#12556),#2050,.F.) ;
#47775=ADVANCED_FACE('',(#12557),#10195,.T.) ;
#47776=ADVANCED_FACE('',(#12558),#45737,.F.) ;
#47777=ADVANCED_FACE('',(#12559),#45738,.T.) ;
#47778=ADVANCED_FACE('',(#12560),#10196,.T.) ;
#47779=ADVANCED_FACE('',(#12561),#10197,.T.) ;
#47780=ADVANCED_FACE('',(#12562),#10198,.F.) ;
#47781=ADVANCED_FACE('',(#12563),#2605,.T.) ;
#47782=ADVANCED_FACE('',(#12564),#2606,.T.) ;
#47783=ADVANCED_FACE('',(#12565),#2213,.T.) ;
#47784=ADVANCED_FACE('',(#12566),#10199,.T.) ;
#47785=ADVANCED_FACE('',(#12567),#45739,.T.) ;
#47786=ADVANCED_FACE('',(#12568),#10200,.T.) ;
#47787=ADVANCED_FACE('',(#12569),#45740,.T.) ;
#47788=ADVANCED_FACE('',(#12570),#10201,.T.) ;
#47789=ADVANCED_FACE('',(#12571),#10202,.T.) ;
#47790=ADVANCED_FACE('',(#12572),#45741,.T.) ;
#47791=ADVANCED_FACE('',(#12573),#10203,.T.) ;
#47792=ADVANCED_FACE('',(#12574),#2051,.F.) ;
#47793=ADVANCED_FACE('',(#12575),#45742,.T.) ;
#47794=ADVANCED_FACE('',(#12576),#99,.F.) ;
#47795=ADVANCED_FACE('',(#12577),#10204,.T.) ;
#47796=ADVANCED_FACE('',(#12578),#45743,.T.) ;
#47797=ADVANCED_FACE('',(#12579),#10205,.T.) ;
#47798=ADVANCED_FACE('',(#12580),#10206,.T.) ;
#47799=ADVANCED_FACE('',(#12581),#10207,.F.) ;
#47800=ADVANCED_FACE('',(#12582),#45744,.F.) ;
#47801=ADVANCED_FACE('',(#12583),#10208,.F.) ;
#47802=ADVANCED_FACE('',(#12584),#100,.T.) ;
#47803=ADVANCED_FACE('',(#12585),#2607,.F.) ;
#47804=ADVANCED_FACE('',(#12586),#2608,.T.) ;
#47805=ADVANCED_FACE('',(#12587),#10209,.F.) ;
#47806=ADVANCED_FACE('',(#12588),#2609,.T.) ;
#47807=ADVANCED_FACE('',(#12589),#10210,.T.) ;
#47808=ADVANCED_FACE('',(#12590),#2610,.T.) ;
#47809=ADVANCED_FACE('',(#12591),#10211,.T.) ;
#47810=ADVANCED_FACE('',(#12592),#2611,.T.) ;
#47811=ADVANCED_FACE('',(#12593),#10212,.T.) ;
#47812=ADVANCED_FACE('',(#12594),#10213,.F.) ;
#47813=ADVANCED_FACE('',(#12595),#2052,.F.) ;
#47814=ADVANCED_FACE('',(#12596),#10214,.F.) ;
#47815=ADVANCED_FACE('',(#12597),#45745,.T.) ;
#47816=ADVANCED_FACE('',(#12598),#10215,.T.) ;
#47817=ADVANCED_FACE('',(#12599),#45746,.T.) ;
#47818=ADVANCED_FACE('',(#12600),#45747,.T.) ;
#47819=ADVANCED_FACE('',(#12601),#2053,.F.) ;
#47820=ADVANCED_FACE('',(#12602),#45748,.T.) ;
#47821=ADVANCED_FACE('',(#12603),#10216,.T.) ;
#47822=ADVANCED_FACE('',(#12604),#10217,.T.) ;
#47823=ADVANCED_FACE('',(#12605),#2054,.F.) ;
#47824=ADVANCED_FACE('',(#12606),#2055,.F.) ;
#47825=ADVANCED_FACE('',(#12607),#10218,.T.) ;
#47826=ADVANCED_FACE('',(#12608),#10219,.F.) ;
#47827=ADVANCED_FACE('',(#12609),#45749,.T.) ;
#47828=ADVANCED_FACE('',(#12610),#10220,.T.) ;
#47829=ADVANCED_FACE('',(#12611),#45750,.T.) ;
#47830=ADVANCED_FACE('',(#12612),#10221,.T.) ;
#47831=ADVANCED_FACE('',(#12613),#10222,.F.) ;
#47832=ADVANCED_FACE('',(#12614),#10223,.T.) ;
#47833=ADVANCED_FACE('',(#12615),#45751,.T.) ;
#47834=ADVANCED_FACE('',(#12616),#10224,.T.) ;
#47835=ADVANCED_FACE('',(#12617),#45752,.T.) ;
#47836=ADVANCED_FACE('',(#12618),#10225,.T.) ;
#47837=ADVANCED_FACE('',(#12619),#45753,.T.) ;
#47838=ADVANCED_FACE('',(#12620),#10226,.T.) ;
#47839=ADVANCED_FACE('',(#12621),#45754,.T.) ;
#47840=ADVANCED_FACE('',(#12622),#10227,.T.) ;
#47841=ADVANCED_FACE('',(#12623),#10228,.T.) ;
#47842=ADVANCED_FACE('',(#12624),#2056,.F.) ;
#47843=ADVANCED_FACE('',(#12625),#2057,.F.) ;
#47844=ADVANCED_FACE('',(#12626),#10229,.F.) ;
#47845=ADVANCED_FACE('',(#12627),#10230,.F.) ;
#47846=ADVANCED_FACE('',(#12628),#10231,.F.) ;
#47847=ADVANCED_FACE('',(#12629),#10232,.T.) ;
#47848=ADVANCED_FACE('',(#12630),#10233,.F.) ;
#47849=ADVANCED_FACE('',(#12631),#2612,.T.) ;
#47850=ADVANCED_FACE('',(#12632),#10234,.F.) ;
#47851=ADVANCED_FACE('',(#12633),#10235,.T.) ;
#47852=ADVANCED_FACE('',(#12634),#2613,.T.) ;
#47853=ADVANCED_FACE('',(#12635),#2614,.F.) ;
#47854=ADVANCED_FACE('',(#12636),#2615,.T.) ;
#47855=ADVANCED_FACE('',(#12637),#2616,.F.) ;
#47856=ADVANCED_FACE('',(#12638),#2617,.F.) ;
#47857=ADVANCED_FACE('',(#12639),#10236,.T.) ;
#47858=ADVANCED_FACE('',(#12640),#2618,.T.) ;
#47859=ADVANCED_FACE('',(#12641),#10237,.T.) ;
#47860=ADVANCED_FACE('',(#12642),#45755,.T.) ;
#47861=ADVANCED_FACE('',(#12643),#45756,.T.) ;
#47862=ADVANCED_FACE('',(#12644),#10238,.T.) ;
#47863=ADVANCED_FACE('',(#12645),#10239,.T.) ;
#47864=ADVANCED_FACE('',(#12646),#45757,.T.) ;
#47865=ADVANCED_FACE('',(#12647),#10240,.T.) ;
#47866=ADVANCED_FACE('',(#12648),#10241,.F.) ;
#47867=ADVANCED_FACE('',(#12649),#10242,.F.) ;
#47868=ADVANCED_FACE('',(#12650),#10243,.T.) ;
#47869=ADVANCED_FACE('',(#12651),#45758,.T.) ;
#47870=ADVANCED_FACE('',(#12652),#10244,.T.) ;
#47871=ADVANCED_FACE('',(#12653),#10245,.T.) ;
#47872=ADVANCED_FACE('',(#12654),#2619,.T.) ;
#47873=ADVANCED_FACE('',(#12655),#10246,.T.) ;
#47874=ADVANCED_FACE('',(#12656),#2620,.T.) ;
#47875=ADVANCED_FACE('',(#12657),#10247,.T.) ;
#47876=ADVANCED_FACE('',(#12658),#2058,.F.) ;
#47877=ADVANCED_FACE('',(#12659),#10248,.T.) ;
#47878=ADVANCED_FACE('',(#12660),#45759,.T.) ;
#47879=ADVANCED_FACE('',(#12661),#10249,.T.) ;
#47880=ADVANCED_FACE('',(#12662),#45760,.T.) ;
#47881=ADVANCED_FACE('',(#12663),#10250,.T.) ;
#47882=ADVANCED_FACE('',(#12664),#45761,.T.) ;
#47883=ADVANCED_FACE('',(#12665),#10251,.T.) ;
#47884=ADVANCED_FACE('',(#12666),#45762,.T.) ;
#47885=ADVANCED_FACE('',(#12667),#10252,.T.) ;
#47886=ADVANCED_FACE('',(#12668),#45763,.T.) ;
#47887=ADVANCED_FACE('',(#12669),#10253,.T.) ;
#47888=ADVANCED_FACE('',(#12670),#2059,.F.) ;
#47889=ADVANCED_FACE('',(#12671),#10254,.T.) ;
#47890=ADVANCED_FACE('',(#12672),#2060,.F.) ;
#47891=ADVANCED_FACE('',(#12673),#2061,.F.) ;
#47892=ADVANCED_FACE('',(#12674),#2062,.F.) ;
#47893=ADVANCED_FACE('',(#12675),#45764,.T.) ;
#47894=ADVANCED_FACE('',(#12676),#10255,.T.) ;
#47895=ADVANCED_FACE('',(#12677),#45765,.T.) ;
#47896=ADVANCED_FACE('',(#12678),#10256,.T.) ;
#47897=ADVANCED_FACE('',(#12679),#45766,.T.) ;
#47898=ADVANCED_FACE('',(#12680),#45767,.T.) ;
#47899=ADVANCED_FACE('',(#12681),#10257,.T.) ;
#47900=ADVANCED_FACE('',(#12682),#45768,.T.) ;
#47901=ADVANCED_FACE('',(#12683),#10258,.T.) ;
#47902=ADVANCED_FACE('',(#12684),#45769,.T.) ;
#47903=ADVANCED_FACE('',(#12685),#2621,.T.) ;
#47904=ADVANCED_FACE('',(#12686),#10259,.T.) ;
#47905=ADVANCED_FACE('',(#12687),#2622,.T.) ;
#47906=ADVANCED_FACE('',(#12688),#10260,.T.) ;
#47907=ADVANCED_FACE('',(#12689),#10261,.F.) ;
#47908=ADVANCED_FACE('',(#12690),#2623,.T.) ;
#47909=ADVANCED_FACE('',(#12691),#10262,.T.) ;
#47910=ADVANCED_FACE('',(#12692),#10263,.T.) ;
#47911=ADVANCED_FACE('',(#12693),#10264,.T.) ;
#47912=ADVANCED_FACE('',(#12694),#10265,.T.) ;
#47913=ADVANCED_FACE('',(#12695),#45770,.T.) ;
#47914=ADVANCED_FACE('',(#12696),#10266,.T.) ;
#47915=ADVANCED_FACE('',(#12697),#45771,.T.) ;
#47916=ADVANCED_FACE('',(#12698),#10267,.T.) ;
#47917=ADVANCED_FACE('',(#12699),#45772,.T.) ;
#47918=ADVANCED_FACE('',(#12700),#10268,.T.) ;
#47919=ADVANCED_FACE('',(#12701),#45773,.T.) ;
#47920=ADVANCED_FACE('',(#12702),#10269,.T.) ;
#47921=ADVANCED_FACE('',(#12703),#45774,.T.) ;
#47922=ADVANCED_FACE('',(#12704),#10270,.T.) ;
#47923=ADVANCED_FACE('',(#12705),#10271,.T.) ;
#47924=ADVANCED_FACE('',(#12706),#45775,.T.) ;
#47925=ADVANCED_FACE('',(#12707),#10272,.T.) ;
#47926=ADVANCED_FACE('',(#12708),#45776,.T.) ;
#47927=ADVANCED_FACE('',(#12709),#10273,.T.) ;
#47928=ADVANCED_FACE('',(#12710),#45777,.T.) ;
#47929=ADVANCED_FACE('',(#12711),#10274,.T.) ;
#47930=ADVANCED_FACE('',(#12712),#2624,.F.) ;
#47931=ADVANCED_FACE('',(#12713),#2625,.T.) ;
#47932=ADVANCED_FACE('',(#12714),#10275,.T.) ;
#47933=ADVANCED_FACE('',(#12715,#748,#749),#2626,.T.) ;
#47934=ADVANCED_FACE('',(#12716),#10276,.T.) ;
#47935=ADVANCED_FACE('',(#12717),#2627,.T.) ;
#47936=ADVANCED_FACE('',(#12718,#750),#2628,.T.) ;
#47937=ADVANCED_FACE('',(#12719),#10277,.T.) ;
#47938=ADVANCED_FACE('',(#12720),#2629,.F.) ;
#47939=ADVANCED_FACE('',(#12721),#2630,.T.) ;
#47940=ADVANCED_FACE('',(#12722),#2063,.F.) ;
#47941=ADVANCED_FACE('',(#12723),#2064,.F.) ;
#47942=ADVANCED_FACE('',(#12724),#10278,.T.) ;
#47943=ADVANCED_FACE('',(#12725),#2065,.F.) ;
#47944=ADVANCED_FACE('',(#12726),#45778,.T.) ;
#47945=ADVANCED_FACE('',(#12727),#10279,.T.) ;
#47946=ADVANCED_FACE('',(#12728),#10280,.F.) ;
#47947=ADVANCED_FACE('',(#12729),#10281,.T.) ;
#47948=ADVANCED_FACE('',(#12730),#10282,.F.) ;
#47949=ADVANCED_FACE('',(#12731),#10283,.T.) ;
#47950=ADVANCED_FACE('',(#12732),#2066,.F.) ;
#47951=ADVANCED_FACE('',(#12733),#2067,.F.) ;
#47952=ADVANCED_FACE('',(#12734),#10284,.T.) ;
#47953=ADVANCED_FACE('',(#12735),#2631,.F.) ;
#47954=ADVANCED_FACE('',(#12736),#10285,.T.) ;
#47955=ADVANCED_FACE('',(#12737),#2632,.T.) ;
#47956=ADVANCED_FACE('',(#12738),#10286,.F.) ;
#47957=ADVANCED_FACE('',(#12739),#10287,.T.) ;
#47958=ADVANCED_FACE('',(#12740),#10288,.T.) ;
#47959=ADVANCED_FACE('',(#12741),#2633,.F.) ;
#47960=ADVANCED_FACE('',(#12742),#2634,.T.) ;
#47961=ADVANCED_FACE('',(#12743),#2635,.F.) ;
#47962=ADVANCED_FACE('',(#12744),#2068,.F.) ;
#47963=ADVANCED_FACE('',(#12745),#10289,.T.) ;
#47964=ADVANCED_FACE('',(#12746),#2069,.F.) ;
#47965=ADVANCED_FACE('',(#12747),#2070,.F.) ;
#47966=ADVANCED_FACE('',(#12748),#2071,.F.) ;
#47967=ADVANCED_FACE('',(#12749),#2072,.F.) ;
#47968=ADVANCED_FACE('',(#12750),#10290,.F.) ;
#47969=ADVANCED_FACE('',(#12751),#10291,.F.) ;
#47970=ADVANCED_FACE('',(#12752),#2073,.F.) ;
#47971=ADVANCED_FACE('',(#12753),#10292,.T.) ;
#47972=ADVANCED_FACE('',(#12754),#2074,.F.) ;
#47973=ADVANCED_FACE('',(#12755),#2075,.F.) ;
#47974=ADVANCED_FACE('',(#12756,#751,#752,#753),#2636,.T.) ;
#47975=ADVANCED_FACE('',(#12757),#10293,.T.) ;
#47976=ADVANCED_FACE('',(#12758),#2637,.T.) ;
#47977=ADVANCED_FACE('',(#12759),#10294,.T.) ;
#47978=ADVANCED_FACE('',(#12760),#2076,.F.) ;
#47979=ADVANCED_FACE('',(#12761),#2077,.T.) ;
#47980=ADVANCED_FACE('',(#12762),#10295,.F.) ;
#47981=ADVANCED_FACE('',(#12763),#10296,.T.) ;
#47982=ADVANCED_FACE('',(#12764),#2638,.T.) ;
#47983=ADVANCED_FACE('',(#12765),#2078,.F.) ;
#47984=ADVANCED_FACE('',(#12766),#2079,.F.) ;
#47985=ADVANCED_FACE('',(#12767),#10297,.T.) ;
#47986=ADVANCED_FACE('',(#12768),#2639,.T.) ;
#47987=ADVANCED_FACE('',(#12769),#2640,.F.) ;
#47988=ADVANCED_FACE('',(#12770),#2641,.T.) ;
#47989=ADVANCED_FACE('',(#12771),#10298,.T.) ;
#47990=ADVANCED_FACE('',(#12772),#10299,.F.) ;
#47991=ADVANCED_FACE('',(#12773),#2642,.T.) ;
#47992=ADVANCED_FACE('',(#12774),#10300,.F.) ;
#47993=ADVANCED_FACE('',(#12775),#2643,.F.) ;
#47994=ADVANCED_FACE('',(#12776),#10301,.T.) ;
#47995=ADVANCED_FACE('',(#12777),#2644,.F.) ;
#47996=ADVANCED_FACE('',(#12778),#10302,.F.) ;
#47997=ADVANCED_FACE('',(#12779),#2645,.F.) ;
#47998=ADVANCED_FACE('',(#12780),#2080,.F.) ;
#47999=ADVANCED_FACE('',(#12781),#10303,.F.) ;
#48000=ADVANCED_FACE('',(#12782),#10304,.F.) ;
#48001=ADVANCED_FACE('',(#12783),#2646,.T.) ;
#48002=ADVANCED_FACE('',(#12784),#2647,.T.) ;
#48003=ADVANCED_FACE('',(#12785),#2648,.T.) ;
#48004=ADVANCED_FACE('',(#12786,#754),#2649,.F.) ;
#48005=ADVANCED_FACE('',(#12787),#45779,.T.) ;
#48006=ADVANCED_FACE('',(#12788),#10305,.T.) ;
#48007=ADVANCED_FACE('',(#12789),#45780,.T.) ;
#48008=ADVANCED_FACE('',(#12790),#10306,.T.) ;
#48009=ADVANCED_FACE('',(#12791),#2650,.T.) ;
#48010=ADVANCED_FACE('',(#12792),#2651,.T.) ;
#48011=ADVANCED_FACE('',(#12793),#2652,.T.) ;
#48012=ADVANCED_FACE('',(#12794),#2653,.T.) ;
#48013=ADVANCED_FACE('',(#12795,#755),#2654,.F.) ;
#48014=ADVANCED_FACE('',(#12796),#2655,.F.) ;
#48015=ADVANCED_FACE('',(#12797,#756),#2656,.F.) ;
#48016=ADVANCED_FACE('',(#12798),#2657,.F.) ;
#48017=ADVANCED_FACE('',(#12799),#10307,.F.) ;
#48018=ADVANCED_FACE('',(#12800),#2081,.T.) ;
#48019=ADVANCED_FACE('',(#12801),#10308,.F.) ;
#48020=ADVANCED_FACE('',(#12802),#2082,.T.) ;
#48021=ADVANCED_FACE('',(#12803),#10309,.F.) ;
#48022=ADVANCED_FACE('',(#12804),#10310,.F.) ;
#48023=ADVANCED_FACE('',(#12805),#10311,.F.) ;
#48024=ADVANCED_FACE('',(#12806),#2658,.F.) ;
#48025=ADVANCED_FACE('',(#12807),#2659,.F.) ;
#48026=ADVANCED_FACE('',(#12808),#2660,.F.) ;
#48027=ADVANCED_FACE('',(#12809),#2661,.F.) ;
#48028=ADVANCED_FACE('',(#12810),#2662,.T.) ;
#48029=ADVANCED_FACE('',(#12811),#2083,.T.) ;
#48030=ADVANCED_FACE('',(#12812),#10312,.F.) ;
#48031=ADVANCED_FACE('',(#12813),#10313,.F.) ;
#48032=ADVANCED_FACE('',(#12814),#10314,.F.) ;
#48033=ADVANCED_FACE('',(#12815),#10315,.F.) ;
#48034=ADVANCED_FACE('',(#12816),#2084,.T.) ;
#48035=ADVANCED_FACE('',(#12817),#10316,.F.) ;
#48036=ADVANCED_FACE('',(#12818),#2663,.F.) ;
#48037=ADVANCED_FACE('',(#12819),#2085,.F.) ;
#48038=ADVANCED_FACE('',(#12820),#2664,.F.) ;
#48039=ADVANCED_FACE('',(#12821),#2086,.F.) ;
#48040=ADVANCED_FACE('',(#12822),#2665,.T.) ;
#48041=ADVANCED_FACE('',(#12823),#10317,.F.) ;
#48042=ADVANCED_FACE('',(#12824),#10318,.F.) ;
#48043=ADVANCED_FACE('',(#12825),#10319,.F.) ;
#48044=ADVANCED_FACE('',(#12826),#10320,.F.) ;
#48045=ADVANCED_FACE('',(#12827),#10321,.F.) ;
#48046=ADVANCED_FACE('',(#12828),#10322,.F.) ;
#48047=ADVANCED_FACE('',(#12829),#10323,.F.) ;
#48048=ADVANCED_FACE('',(#12830),#2666,.F.) ;
#48049=ADVANCED_FACE('',(#12831),#2667,.F.) ;
#48050=ADVANCED_FACE('',(#12832),#2668,.F.) ;
#48051=ADVANCED_FACE('',(#12833),#2669,.F.) ;
#48052=ADVANCED_FACE('',(#12834),#2670,.F.) ;
#48053=ADVANCED_FACE('',(#12835),#10324,.F.) ;
#48054=ADVANCED_FACE('',(#12836),#10325,.F.) ;
#48055=ADVANCED_FACE('',(#12837),#10326,.F.) ;
#48056=ADVANCED_FACE('',(#12838),#10327,.F.) ;
#48057=ADVANCED_FACE('',(#12839),#2671,.F.) ;
#48058=ADVANCED_FACE('',(#12840),#2672,.F.) ;
#48059=ADVANCED_FACE('',(#12841),#2673,.F.) ;
#48060=ADVANCED_FACE('',(#12842),#10328,.F.) ;
#48061=ADVANCED_FACE('',(#12843),#10329,.F.) ;
#48062=ADVANCED_FACE('',(#12844),#10330,.F.) ;
#48063=ADVANCED_FACE('',(#12845),#10331,.F.) ;
#48064=ADVANCED_FACE('',(#12846),#10332,.F.) ;
#48065=ADVANCED_FACE('',(#12847),#10333,.F.) ;
#48066=ADVANCED_FACE('',(#12848),#10334,.F.) ;
#48067=ADVANCED_FACE('',(#12849),#2674,.F.) ;
#48068=ADVANCED_FACE('',(#12850),#2675,.F.) ;
#48069=ADVANCED_FACE('',(#12851),#2676,.F.) ;
#48070=ADVANCED_FACE('',(#12852),#2677,.F.) ;
#48071=ADVANCED_FACE('',(#12853),#2678,.F.) ;
#48072=ADVANCED_FACE('',(#12854),#10335,.F.) ;
#48073=ADVANCED_FACE('',(#12855),#10336,.F.) ;
#48074=ADVANCED_FACE('',(#12856),#10337,.F.) ;
#48075=ADVANCED_FACE('',(#12857),#10338,.F.) ;
#48076=ADVANCED_FACE('',(#12858),#2679,.F.) ;
#48077=ADVANCED_FACE('',(#12859),#2680,.F.) ;
#48078=ADVANCED_FACE('',(#12860),#2681,.F.) ;
#48079=ADVANCED_FACE('',(#12861),#10339,.F.) ;
#48080=ADVANCED_FACE('',(#12862),#10340,.F.) ;
#48081=ADVANCED_FACE('',(#12863),#10341,.F.) ;
#48082=ADVANCED_FACE('',(#12864),#45781,.F.) ;
#48083=ADVANCED_FACE('',(#12865),#10342,.F.) ;
#48084=ADVANCED_FACE('',(#12866),#10343,.F.) ;
#48085=ADVANCED_FACE('',(#12867),#10344,.F.) ;
#48086=ADVANCED_FACE('',(#12868),#45782,.F.) ;
#48087=ADVANCED_FACE('',(#12869),#10345,.F.) ;
#48088=ADVANCED_FACE('',(#12870),#10346,.F.) ;
#48089=ADVANCED_FACE('',(#12871),#10347,.F.) ;
#48090=ADVANCED_FACE('',(#12872),#2682,.F.) ;
#48091=ADVANCED_FACE('',(#12873),#10348,.T.) ;
#48092=ADVANCED_FACE('',(#12874),#2683,.F.) ;
#48093=ADVANCED_FACE('',(#12875),#2684,.F.) ;
#48094=ADVANCED_FACE('',(#12876),#2685,.F.) ;
#48095=ADVANCED_FACE('',(#12877),#2686,.F.) ;
#48096=ADVANCED_FACE('',(#12878),#2687,.T.) ;
#48097=ADVANCED_FACE('',(#12879),#10349,.F.) ;
#48098=ADVANCED_FACE('',(#12880),#10350,.F.) ;
#48099=ADVANCED_FACE('',(#12881),#45783,.F.) ;
#48100=ADVANCED_FACE('',(#12882),#10351,.F.) ;
#48101=ADVANCED_FACE('',(#12883),#10352,.F.) ;
#48102=ADVANCED_FACE('',(#12884),#10353,.F.) ;
#48103=ADVANCED_FACE('',(#12885),#45784,.F.) ;
#48104=ADVANCED_FACE('',(#12886),#10354,.F.) ;
#48105=ADVANCED_FACE('',(#12887),#10355,.F.) ;
#48106=ADVANCED_FACE('',(#12888),#10356,.F.) ;
#48107=ADVANCED_FACE('',(#12889),#10357,.F.) ;
#48108=ADVANCED_FACE('',(#12890),#10358,.T.) ;
#48109=ADVANCED_FACE('',(#12891),#2688,.F.) ;
#48110=ADVANCED_FACE('',(#12892),#2689,.F.) ;
#48111=ADVANCED_FACE('',(#12893),#2690,.F.) ;
#48112=ADVANCED_FACE('',(#12894),#2691,.F.) ;
#48113=ADVANCED_FACE('',(#12895),#2692,.F.) ;
#48114=ADVANCED_FACE('',(#12896),#2693,.T.) ;
#48115=ADVANCED_FACE('',(#12897),#2087,.F.) ;
#48116=ADVANCED_FACE('',(#12898),#10359,.T.) ;
#48117=ADVANCED_FACE('',(#12899),#10360,.T.) ;
#48118=ADVANCED_FACE('',(#12900),#10361,.T.) ;
#48119=ADVANCED_FACE('',(#12901),#10362,.T.) ;
#48120=ADVANCED_FACE('',(#12902),#10363,.T.) ;
#48121=ADVANCED_FACE('',(#12903),#2088,.F.) ;
#48122=ADVANCED_FACE('',(#12904),#2089,.F.) ;
#48123=ADVANCED_FACE('',(#12905),#2694,.F.) ;
#48124=ADVANCED_FACE('',(#12906),#2090,.F.) ;
#48125=ADVANCED_FACE('',(#12907),#2091,.F.) ;
#48126=ADVANCED_FACE('',(#12908),#10364,.T.) ;
#48127=ADVANCED_FACE('',(#12909),#10365,.T.) ;
#48128=ADVANCED_FACE('',(#12910),#10366,.T.) ;
#48129=ADVANCED_FACE('',(#12911),#10367,.T.) ;
#48130=ADVANCED_FACE('',(#12912),#2092,.F.) ;
#48131=ADVANCED_FACE('',(#12913),#10368,.T.) ;
#48132=ADVANCED_FACE('',(#12914),#2695,.F.) ;
#48133=ADVANCED_FACE('',(#12915),#2696,.F.) ;
#48134=ADVANCED_FACE('',(#12916),#10369,.T.) ;
#48135=ADVANCED_FACE('',(#12917),#10370,.T.) ;
#48136=ADVANCED_FACE('',(#12918),#10371,.T.) ;
#48137=ADVANCED_FACE('',(#12919),#10372,.T.) ;
#48138=ADVANCED_FACE('',(#12920),#10373,.T.) ;
#48139=ADVANCED_FACE('',(#12921),#10374,.T.) ;
#48140=ADVANCED_FACE('',(#12922),#10375,.T.) ;
#48141=ADVANCED_FACE('',(#12923),#2697,.F.) ;
#48142=ADVANCED_FACE('',(#12924),#2698,.F.) ;
#48143=ADVANCED_FACE('',(#12925),#2699,.F.) ;
#48144=ADVANCED_FACE('',(#12926,#757,#758,#759),#2700,.T.) ;
#48145=ADVANCED_FACE('',(#12927),#10376,.T.) ;
#48146=ADVANCED_FACE('',(#12928),#10377,.T.) ;
#48147=ADVANCED_FACE('',(#12929),#10378,.T.) ;
#48148=ADVANCED_FACE('',(#12930),#10379,.T.) ;
#48149=ADVANCED_FACE('',(#12931),#2701,.F.) ;
#48150=ADVANCED_FACE('',(#12932),#10380,.T.) ;
#48151=ADVANCED_FACE('',(#12933),#10381,.T.) ;
#48152=ADVANCED_FACE('',(#12934),#10382,.T.) ;
#48153=ADVANCED_FACE('',(#12935),#10383,.T.) ;
#48154=ADVANCED_FACE('',(#12936),#10384,.T.) ;
#48155=ADVANCED_FACE('',(#12937),#10385,.T.) ;
#48156=ADVANCED_FACE('',(#12938),#10386,.T.) ;
#48157=ADVANCED_FACE('',(#12939),#2702,.F.) ;
#48158=ADVANCED_FACE('',(#12940),#2703,.F.) ;
#48159=ADVANCED_FACE('',(#12941),#10387,.T.) ;
#48160=ADVANCED_FACE('',(#12942),#10388,.T.) ;
#48161=ADVANCED_FACE('',(#12943),#10389,.T.) ;
#48162=ADVANCED_FACE('',(#12944),#10390,.T.) ;
#48163=ADVANCED_FACE('',(#12945),#10391,.T.) ;
#48164=ADVANCED_FACE('',(#12946),#10392,.T.) ;
#48165=ADVANCED_FACE('',(#12947),#10393,.T.) ;
#48166=ADVANCED_FACE('',(#12948),#10394,.T.) ;
#48167=ADVANCED_FACE('',(#12949),#10395,.T.) ;
#48168=ADVANCED_FACE('',(#12950),#10396,.T.) ;
#48169=ADVANCED_FACE('',(#12951),#45785,.T.) ;
#48170=ADVANCED_FACE('',(#12952),#10397,.T.) ;
#48171=ADVANCED_FACE('',(#12953),#45786,.T.) ;
#48172=ADVANCED_FACE('',(#12954),#10398,.T.) ;
#48173=ADVANCED_FACE('',(#12955),#2704,.F.) ;
#48174=ADVANCED_FACE('',(#12956),#10399,.F.) ;
#48175=ADVANCED_FACE('',(#12957),#2705,.F.) ;
#48176=ADVANCED_FACE('',(#12958),#2706,.F.) ;
#48177=ADVANCED_FACE('',(#12959),#10400,.T.) ;
#48178=ADVANCED_FACE('',(#12960),#10401,.T.) ;
#48179=ADVANCED_FACE('',(#12961),#10402,.T.) ;
#48180=ADVANCED_FACE('',(#12962),#10403,.T.) ;
#48181=ADVANCED_FACE('',(#12963),#10404,.T.) ;
#48182=ADVANCED_FACE('',(#12964),#10405,.T.) ;
#48183=ADVANCED_FACE('',(#12965),#45787,.T.) ;
#48184=ADVANCED_FACE('',(#12966),#10406,.T.) ;
#48185=ADVANCED_FACE('',(#12967),#10407,.T.) ;
#48186=ADVANCED_FACE('',(#12968),#45788,.T.) ;
#48187=ADVANCED_FACE('',(#12969),#10408,.T.) ;
#48188=ADVANCED_FACE('',(#12970),#2707,.F.) ;
#48189=ADVANCED_FACE('',(#12971),#2708,.F.) ;
#48190=ADVANCED_FACE('',(#12972),#2709,.F.) ;
#48191=ADVANCED_FACE('',(#12973),#10409,.F.) ;
#48192=ADVANCED_FACE('',(#12974),#2710,.F.) ;
#48193=ADVANCED_FACE('',(#12975),#2711,.F.) ;
#48194=ADVANCED_FACE('',(#12976),#2712,.F.) ;
#48195=ADVANCED_FACE('',(#12977),#2713,.F.) ;
#48196=ADVANCED_FACE('',(#12978),#2714,.F.) ;
#48197=ADVANCED_FACE('',(#12979),#2715,.F.) ;
#48198=ADVANCED_FACE('',(#12980),#2716,.F.) ;
#48199=ADVANCED_FACE('',(#12981),#2717,.F.) ;
#48200=ADVANCED_FACE('',(#12982),#2718,.T.) ;
#48201=ADVANCED_FACE('',(#12983),#2719,.T.) ;
#48202=ADVANCED_FACE('',(#12984),#10410,.F.) ;
#48203=ADVANCED_FACE('',(#12985),#2720,.T.) ;
#48204=ADVANCED_FACE('',(#12986),#10411,.T.) ;
#48205=ADVANCED_FACE('',(#12987),#2721,.T.) ;
#48206=ADVANCED_FACE('',(#12988),#2722,.T.) ;
#48207=ADVANCED_FACE('',(#12989),#2723,.T.) ;
#48208=ADVANCED_FACE('',(#12990),#2724,.F.) ;
#48209=ADVANCED_FACE('',(#12991),#10412,.T.) ;
#48210=ADVANCED_FACE('',(#12992),#2725,.T.) ;
#48211=ADVANCED_FACE('',(#12993),#2726,.T.) ;
#48212=ADVANCED_FACE('',(#12994),#2727,.T.) ;
#48213=ADVANCED_FACE('',(#12995),#2728,.T.) ;
#48214=ADVANCED_FACE('',(#12996),#2729,.F.) ;
#48215=ADVANCED_FACE('',(#12997),#2730,.F.) ;
#48216=ADVANCED_FACE('',(#12998),#2731,.F.) ;
#48217=ADVANCED_FACE('',(#12999),#2732,.T.) ;
#48218=ADVANCED_FACE('',(#13000),#2733,.T.) ;
#48219=ADVANCED_FACE('',(#13001),#10413,.T.) ;
#48220=ADVANCED_FACE('',(#13002),#2734,.T.) ;
#48221=ADVANCED_FACE('',(#13003),#2735,.T.) ;
#48222=ADVANCED_FACE('',(#13004),#2736,.F.) ;
#48223=ADVANCED_FACE('',(#13005),#10414,.F.) ;
#48224=ADVANCED_FACE('',(#13006),#2737,.T.) ;
#48225=ADVANCED_FACE('',(#13007),#2738,.T.) ;
#48226=ADVANCED_FACE('',(#13008),#2739,.T.) ;
#48227=ADVANCED_FACE('',(#13009),#2740,.T.) ;
#48228=ADVANCED_FACE('',(#13010),#2741,.T.) ;
#48229=ADVANCED_FACE('',(#13011),#10415,.T.) ;
#48230=ADVANCED_FACE('',(#13012),#2742,.F.) ;
#48231=ADVANCED_FACE('',(#13013),#10416,.T.) ;
#48232=ADVANCED_FACE('',(#13014),#2743,.T.) ;
#48233=ADVANCED_FACE('',(#13015),#2744,.F.) ;
#48234=ADVANCED_FACE('',(#13016),#2745,.F.) ;
#48235=ADVANCED_FACE('',(#13017),#2746,.F.) ;
#48236=ADVANCED_FACE('',(#13018),#2747,.T.) ;
#48237=ADVANCED_FACE('',(#13019),#10417,.T.) ;
#48238=ADVANCED_FACE('',(#13020),#2214,.T.) ;
#48239=ADVANCED_FACE('',(#13021),#45789,.T.) ;
#48240=ADVANCED_FACE('',(#13022),#2093,.T.) ;
#48241=ADVANCED_FACE('',(#13023),#10418,.T.) ;
#48242=ADVANCED_FACE('',(#13024),#2094,.F.) ;
#48243=ADVANCED_FACE('',(#13025),#45790,.T.) ;
#48244=ADVANCED_FACE('',(#13026),#10419,.T.) ;
#48245=ADVANCED_FACE('',(#13027),#10420,.F.) ;
#48246=ADVANCED_FACE('',(#13028),#2215,.T.) ;
#48247=ADVANCED_FACE('',(#13029),#2095,.F.) ;
#48248=ADVANCED_FACE('',(#13030),#10421,.T.) ;
#48249=ADVANCED_FACE('',(#13031),#45791,.T.) ;
#48250=ADVANCED_FACE('',(#13032),#2096,.F.) ;
#48251=ADVANCED_FACE('',(#13033),#10422,.T.) ;
#48252=ADVANCED_FACE('',(#13034),#45792,.T.) ;
#48253=ADVANCED_FACE('',(#13035),#2097,.F.) ;
#48254=ADVANCED_FACE('',(#13036),#2098,.F.) ;
#48255=ADVANCED_FACE('',(#13037),#45793,.T.) ;
#48256=ADVANCED_FACE('',(#13038),#10423,.T.) ;
#48257=ADVANCED_FACE('',(#13039),#2099,.F.) ;
#48258=ADVANCED_FACE('',(#13040),#10424,.T.) ;
#48259=ADVANCED_FACE('',(#13041),#45794,.T.) ;
#48260=ADVANCED_FACE('',(#13042),#2100,.F.) ;
#48261=ADVANCED_FACE('',(#13043),#10425,.T.) ;
#48262=ADVANCED_FACE('',(#13044),#45795,.T.) ;
#48263=ADVANCED_FACE('',(#13045),#101,.F.) ;
#48264=ADVANCED_FACE('',(#13046),#10426,.T.) ;
#48265=ADVANCED_FACE('',(#13047),#10427,.T.) ;
#48266=ADVANCED_FACE('',(#13048),#45796,.T.) ;
#48267=ADVANCED_FACE('',(#13049),#10428,.T.) ;
#48268=ADVANCED_FACE('',(#13050),#2101,.F.) ;
#48269=ADVANCED_FACE('',(#13051),#102,.F.) ;
#48270=ADVANCED_FACE('',(#13052),#2102,.F.) ;
#48271=ADVANCED_FACE('',(#13053),#10429,.T.) ;
#48272=ADVANCED_FACE('',(#13054),#10430,.T.) ;
#48273=ADVANCED_FACE('',(#13055),#2103,.F.) ;
#48274=ADVANCED_FACE('',(#13056),#10431,.T.) ;
#48275=ADVANCED_FACE('',(#13057),#2748,.F.) ;
#48276=ADVANCED_FACE('',(#13058),#10432,.F.) ;
#48277=ADVANCED_FACE('',(#13059),#2749,.T.) ;
#48278=ADVANCED_FACE('',(#13060),#10433,.T.) ;
#48279=ADVANCED_FACE('',(#13061),#2750,.T.) ;
#48280=ADVANCED_FACE('',(#13062),#2751,.T.) ;
#48281=ADVANCED_FACE('',(#13063),#10434,.T.) ;
#48282=ADVANCED_FACE('',(#13064),#10435,.F.) ;
#48283=ADVANCED_FACE('',(#13065),#10436,.F.) ;
#48284=ADVANCED_FACE('',(#13066),#2752,.T.) ;
#48285=ADVANCED_FACE('',(#13067),#10437,.F.) ;
#48286=ADVANCED_FACE('',(#13068),#2753,.T.) ;
#48287=ADVANCED_FACE('',(#13069),#2754,.T.) ;
#48288=ADVANCED_FACE('',(#13070),#10438,.F.) ;
#48289=ADVANCED_FACE('',(#13071),#2755,.T.) ;
#48290=ADVANCED_FACE('',(#13072),#10439,.F.) ;
#48291=ADVANCED_FACE('',(#13073),#2756,.T.) ;
#48292=ADVANCED_FACE('',(#13074),#2757,.T.) ;
#48293=ADVANCED_FACE('',(#13075),#2104,.T.) ;
#48294=ADVANCED_FACE('',(#13076),#2758,.T.) ;
#48295=ADVANCED_FACE('',(#13077),#2105,.T.) ;
#48296=ADVANCED_FACE('',(#13078),#10440,.F.) ;
#48297=ADVANCED_FACE('',(#13079,#760),#2759,.T.) ;
#48298=ADVANCED_FACE('',(#13080),#10441,.F.) ;
#48299=ADVANCED_FACE('',(#13081),#10442,.F.) ;
#48300=ADVANCED_FACE('',(#13082),#2760,.T.) ;
#48301=ADVANCED_FACE('',(#13083),#10443,.F.) ;
#48302=ADVANCED_FACE('',(#13084),#2761,.T.) ;
#48303=ADVANCED_FACE('',(#13085),#10444,.F.) ;
#48304=ADVANCED_FACE('',(#13086),#2762,.T.) ;
#48305=ADVANCED_FACE('',(#13087),#10445,.F.) ;
#48306=ADVANCED_FACE('',(#13088),#2763,.T.) ;
#48307=ADVANCED_FACE('',(#13089),#10446,.F.) ;
#48308=ADVANCED_FACE('',(#13090),#2764,.T.) ;
#48309=ADVANCED_FACE('',(#13091),#2765,.T.) ;
#48310=ADVANCED_FACE('',(#13092),#10447,.F.) ;
#48311=ADVANCED_FACE('',(#13093),#2766,.T.) ;
#48312=ADVANCED_FACE('',(#13094),#10448,.F.) ;
#48313=ADVANCED_FACE('',(#13095),#2767,.T.) ;
#48314=ADVANCED_FACE('',(#13096),#10449,.F.) ;
#48315=ADVANCED_FACE('',(#13097),#2768,.T.) ;
#48316=ADVANCED_FACE('',(#13098),#10450,.F.) ;
#48317=ADVANCED_FACE('',(#13099),#2769,.T.) ;
#48318=ADVANCED_FACE('',(#13100),#2106,.T.) ;
#48319=ADVANCED_FACE('',(#13101),#10451,.F.) ;
#48320=ADVANCED_FACE('',(#13102),#2770,.T.) ;
#48321=ADVANCED_FACE('',(#13103),#10452,.F.) ;
#48322=ADVANCED_FACE('',(#13104),#2771,.T.) ;
#48323=ADVANCED_FACE('',(#13105),#2772,.T.) ;
#48324=ADVANCED_FACE('',(#13106),#2773,.T.) ;
#48325=ADVANCED_FACE('',(#13107),#10453,.F.) ;
#48326=ADVANCED_FACE('',(#13108),#2774,.T.) ;
#48327=ADVANCED_FACE('',(#13109),#10454,.F.) ;
#48328=ADVANCED_FACE('',(#13110),#2775,.T.) ;
#48329=ADVANCED_FACE('',(#13111),#10455,.F.) ;
#48330=ADVANCED_FACE('',(#13112),#10456,.F.) ;
#48331=ADVANCED_FACE('',(#13113),#2776,.T.) ;
#48332=ADVANCED_FACE('',(#13114),#10457,.F.) ;
#48333=ADVANCED_FACE('',(#13115),#2777,.T.) ;
#48334=ADVANCED_FACE('',(#13116),#2778,.T.) ;
#48335=ADVANCED_FACE('',(#13117),#10458,.F.) ;
#48336=ADVANCED_FACE('',(#13118),#2779,.T.) ;
#48337=ADVANCED_FACE('',(#13119),#10459,.F.) ;
#48338=ADVANCED_FACE('',(#13120),#2780,.T.) ;
#48339=ADVANCED_FACE('',(#13121),#2781,.T.) ;
#48340=ADVANCED_FACE('',(#13122),#10460,.F.) ;
#48341=ADVANCED_FACE('',(#13123),#2782,.T.) ;
#48342=ADVANCED_FACE('',(#13124),#10461,.F.) ;
#48343=ADVANCED_FACE('',(#13125),#2783,.T.) ;
#48344=ADVANCED_FACE('',(#13126),#2784,.F.) ;
#48345=ADVANCED_FACE('',(#13127),#2785,.T.) ;
#48346=ADVANCED_FACE('',(#13128),#2107,.T.) ;
#48347=ADVANCED_FACE('',(#13129),#2786,.T.) ;
#48348=ADVANCED_FACE('',(#13130),#10462,.F.) ;
#48349=ADVANCED_FACE('',(#13131),#2787,.T.) ;
#48350=ADVANCED_FACE('',(#13132),#10463,.F.) ;
#48351=ADVANCED_FACE('',(#13133),#2788,.F.) ;
#48352=ADVANCED_FACE('',(#13134),#2108,.T.) ;
#48353=ADVANCED_FACE('',(#13135),#2789,.T.) ;
#48354=ADVANCED_FACE('',(#13136),#2790,.T.) ;
#48355=ADVANCED_FACE('',(#13137),#10464,.F.) ;
#48356=ADVANCED_FACE('',(#13138),#2791,.T.) ;
#48357=ADVANCED_FACE('',(#13139),#10465,.F.) ;
#48358=ADVANCED_FACE('',(#13140),#2792,.T.) ;
#48359=ADVANCED_FACE('',(#13141),#2793,.F.) ;
#48360=ADVANCED_FACE('',(#13142),#10466,.F.) ;
#48361=ADVANCED_FACE('',(#13143),#2794,.T.) ;
#48362=ADVANCED_FACE('',(#13144),#2795,.T.) ;
#48363=ADVANCED_FACE('',(#13145),#2796,.T.) ;
#48364=ADVANCED_FACE('',(#13146),#2797,.T.) ;
#48365=ADVANCED_FACE('',(#13147),#2798,.T.) ;
#48366=ADVANCED_FACE('',(#13148),#10467,.F.) ;
#48367=ADVANCED_FACE('',(#13149),#2799,.F.) ;
#48368=ADVANCED_FACE('',(#13150),#10468,.F.) ;
#48369=ADVANCED_FACE('',(#13151),#2800,.T.) ;
#48370=ADVANCED_FACE('',(#13152),#2801,.T.) ;
#48371=ADVANCED_FACE('',(#13153),#10469,.F.) ;
#48372=ADVANCED_FACE('',(#13154),#2802,.T.) ;
#48373=ADVANCED_FACE('',(#13155),#10470,.F.) ;
#48374=ADVANCED_FACE('',(#13156),#2803,.T.) ;
#48375=ADVANCED_FACE('',(#13157),#2804,.F.) ;
#48376=ADVANCED_FACE('',(#13158),#10471,.F.) ;
#48377=ADVANCED_FACE('',(#13159),#2805,.T.) ;
#48378=ADVANCED_FACE('',(#13160),#10472,.F.) ;
#48379=ADVANCED_FACE('',(#13161),#2806,.T.) ;
#48380=ADVANCED_FACE('',(#13162),#10473,.F.) ;
#48381=ADVANCED_FACE('',(#13163),#2807,.T.) ;
#48382=ADVANCED_FACE('',(#13164),#2808,.F.) ;
#48383=ADVANCED_FACE('',(#13165),#2809,.F.) ;
#48384=ADVANCED_FACE('',(#13166),#10474,.F.) ;
#48385=ADVANCED_FACE('',(#13167),#2810,.T.) ;
#48386=ADVANCED_FACE('',(#13168),#2811,.F.) ;
#48387=ADVANCED_FACE('',(#13169),#2812,.T.) ;
#48388=ADVANCED_FACE('',(#13170),#2813,.T.) ;
#48389=ADVANCED_FACE('',(#13171),#2814,.T.) ;
#48390=ADVANCED_FACE('',(#13172),#2815,.T.) ;
#48391=ADVANCED_FACE('',(#13173),#2816,.T.) ;
#48392=ADVANCED_FACE('',(#13174),#2817,.T.) ;
#48393=ADVANCED_FACE('',(#13175),#2818,.T.) ;
#48394=ADVANCED_FACE('',(#13176),#10475,.F.) ;
#48395=ADVANCED_FACE('',(#13177),#2819,.T.) ;
#48396=ADVANCED_FACE('',(#13178),#10476,.F.) ;
#48397=ADVANCED_FACE('',(#13179),#2820,.T.) ;
#48398=ADVANCED_FACE('',(#13180),#2821,.F.) ;
#48399=ADVANCED_FACE('',(#13181),#10477,.F.) ;
#48400=ADVANCED_FACE('',(#13182),#2822,.T.) ;
#48401=ADVANCED_FACE('',(#13183),#10478,.T.) ;
#48402=ADVANCED_FACE('',(#13184),#2823,.T.) ;
#48403=ADVANCED_FACE('',(#13185),#2824,.T.) ;
#48404=ADVANCED_FACE('',(#13186),#2825,.F.) ;
#48405=ADVANCED_FACE('',(#13187),#2826,.T.) ;
#48406=ADVANCED_FACE('',(#13188),#2827,.T.) ;
#48407=ADVANCED_FACE('',(#13189),#10479,.T.) ;
#48408=ADVANCED_FACE('',(#13190),#2828,.T.) ;
#48409=ADVANCED_FACE('',(#13191),#10480,.T.) ;
#48410=ADVANCED_FACE('',(#13192),#2829,.T.) ;
#48411=ADVANCED_FACE('',(#13193),#2830,.T.) ;
#48412=ADVANCED_FACE('',(#13194),#10481,.T.) ;
#48413=ADVANCED_FACE('',(#13195),#10482,.F.) ;
#48414=ADVANCED_FACE('',(#13196),#2831,.T.) ;
#48415=ADVANCED_FACE('',(#13197),#10483,.F.) ;
#48416=ADVANCED_FACE('',(#13198),#2832,.F.) ;
#48417=ADVANCED_FACE('',(#13199),#10484,.F.) ;
#48418=ADVANCED_FACE('',(#13200),#2833,.F.) ;
#48419=ADVANCED_FACE('',(#13201),#2834,.F.) ;
#48420=ADVANCED_FACE('',(#13202),#10485,.F.) ;
#48421=ADVANCED_FACE('',(#13203),#2835,.F.) ;
#48422=ADVANCED_FACE('',(#13204),#2836,.F.) ;
#48423=ADVANCED_FACE('',(#13205),#2837,.F.) ;
#48424=ADVANCED_FACE('',(#13206),#2838,.F.) ;
#48425=ADVANCED_FACE('',(#13207),#2839,.F.) ;
#49072=CLOSED_SHELL('',(#47600,#47601,#47602,#47603,#47604,#47605,#47606,
#47607,#47608,#47609,#47610,#47611,#47612,#47613,#47614,#47615,#47616,#47617,
#47618,#47619,#47620,#47621,#47622,#47623,#47624,#47625,#47626,#47627,#47628,
#47629,#47630,#47631,#47632,#47633,#47634,#47635,#47636,#47637,#47638,#47639,
#47640,#47641,#47642,#47643,#47644,#47645,#47646,#47647,#47648,#47649,#47650,
#47651,#47652,#47653,#47654,#47655,#47656,#47657,#47658,#47659,#47660,#47661,
#47662,#47663,#47664,#47665,#47666,#47667,#47668,#47669,#47670,#47671,#47672,
#47673,#47674,#47675,#47676,#47677,#47678,#47679,#47680,#47681,#47682,#47683,
#47684,#47685,#47686,#47687,#47688,#47689,#47690,#47691,#47692,#47693,#47694,
#47695,#47696,#47697,#47698,#47699,#47700,#47701,#47702,#47703,#47704,#47705,
#47706,#47707,#47708,#47709,#47710,#47711,#47712,#47713,#47714,#47715,#47716,
#47717,#47718,#47719,#47720,#47721,#47722,#47723,#47724,#47725,#47726,#47727,
#47728,#47729,#47730,#47731,#47732,#47733,#47734,#47735,#47736,#47737,#47738,
#47739,#47740,#47741,#47742,#47743,#47744,#47745,#47746,#47747,#47748,#47749,
#47750,#47751,#47752,#47753,#47754,#47755,#47756,#47757,#47758,#47759,#47760,
#47761,#47762,#47763,#47764,#47765,#47766,#47767,#47768,#47769,#47770,#47771,
#47772,#47773,#47774,#47775,#47776,#47777,#47778,#47779,#47780,#47781,#47782,
#47783,#47784,#47785,#47786,#47787,#47788,#47789,#47790,#47791,#47792,#47793,
#47794,#47795,#47796,#47797,#47798,#47799,#47800,#47801,#47802,#47803,#47804,
#47805,#47806,#47807,#47808,#47809,#47810,#47811,#47812,#47813,#47814,#47815,
#47816,#47817,#47818,#47819,#47820,#47821,#47822,#47823,#47824,#47825,#47826,
#47827,#47828,#47829,#47830,#47831,#47832,#47833,#47834,#47835,#47836,#47837,
#47838,#47839,#47840,#47841,#47842,#47843,#47844,#47845,#47846,#47847,#47848,
#47849,#47850,#47851,#47852,#47853,#47854,#47855,#47856,#47857,#47858,#47859,
#47860,#47861,#47862,#47863,#47864,#47865,#47866,#47867,#47868,#47869,#47870,
#47871,#47872,#47873,#47874,#47875,#47876,#47877,#47878,#47879,#47880,#47881,
#47882,#47883,#47884,#47885,#47886,#47887,#47888,#47889,#47890,#47891,#47892,
#47893,#47894,#47895,#47896,#47897,#47898,#47899,#47900,#47901,#47902,#47903,
#47904,#47905,#47906,#47907,#47908,#47909,#47910,#47911,#47912,#47913,#47914,
#47915,#47916,#47917,#47918,#47919,#47920,#47921,#47922,#47923,#47924,#47925,
#47926,#47927,#47928,#47929,#47930,#47931,#47932,#47933,#47934,#47935,#47936,
#47937,#47938,#47939,#47940,#47941,#47942,#47943,#47944,#47945,#47946,#47947,
#47948,#47949,#47950,#47951,#47952,#47953,#47954,#47955,#47956,#47957,#47958,
#47959,#47960,#47961,#47962,#47963,#47964,#47965,#47966,#47967,#47968,#47969,
#47970,#47971,#47972,#47973,#47974,#47975,#47976,#47977,#47978,#47979,#47980,
#47981,#47982,#47983,#47984,#47985,#47986,#47987,#47988,#47989,#47990,#47991,
#47992,#47993,#47994,#47995,#47996,#47997,#47998,#47999,#48000,#48001,#48002,
#48003,#48004,#48005,#48006,#48007,#48008,#48009,#48010,#48011,#48012,#48013,
#48014,#48015,#48016,#48017,#48018,#48019,#48020,#48021,#48022,#48023,#48024,
#48025,#48026,#48027,#48028,#48029,#48030,#48031,#48032,#48033,#48034,#48035,
#48036,#48037,#48038,#48039,#48040,#48041,#48042,#48043,#48044,#48045,#48046,
#48047,#48048,#48049,#48050,#48051,#48052,#48053,#48054,#48055,#48056,#48057,
#48058,#48059,#48060,#48061,#48062,#48063,#48064,#48065,#48066,#48067,#48068,
#48069,#48070,#48071,#48072,#48073,#48074,#48075,#48076,#48077,#48078,#48079,
#48080,#48081,#48082,#48083,#48084,#48085,#48086,#48087,#48088,#48089,#48090,
#48091,#48092,#48093,#48094,#48095,#48096,#48097,#48098,#48099,#48100,#48101,
#48102,#48103,#48104,#48105,#48106,#48107,#48108,#48109,#48110,#48111,#48112,
#48113,#48114,#48115,#48116,#48117,#48118,#48119,#48120,#48121,#48122,#48123,
#48124,#48125,#48126,#48127,#48128,#48129,#48130,#48131,#48132,#48133,#48134,
#48135,#48136,#48137,#48138,#48139,#48140,#48141,#48142,#48143,#48144,#48145,
#48146,#48147,#48148,#48149,#48150,#48151,#48152,#48153,#48154,#48155,#48156,
#48157,#48158,#48159,#48160,#48161,#48162,#48163,#48164,#48165,#48166,#48167,
#48168,#48169,#48170,#48171,#48172,#48173,#48174,#48175,#48176,#48177,#48178,
#48179,#48180,#48181,#48182,#48183,#48184,#48185,#48186,#48187,#48188,#48189,
#48190,#48191,#48192,#48193,#48194,#48195,#48196,#48197,#48198,#48199,#48200,
#48201,#48202,#48203,#48204,#48205,#48206,#48207,#48208,#48209,#48210,#48211,
#48212,#48213,#48214,#48215,#48216,#48217,#48218,#48219,#48220,#48221,#48222,
#48223,#48224,#48225,#48226,#48227,#48228,#48229,#48230,#48231,#48232,#48233,
#48234,#48235,#48236,#48237,#48238,#48239,#48240,#48241,#48242,#48243,#48244,
#48245,#48246,#48247,#48248,#48249,#48250,#48251,#48252,#48253,#48254,#48255,
#48256,#48257,#48258,#48259,#48260,#48261,#48262,#48263,#48264,#48265,#48266,
#48267,#48268,#48269,#48270,#48271,#48272,#48273,#48274,#48275,#48276,#48277,
#48278,#48279,#48280,#48281,#48282,#48283,#48284,#48285,#48286,#48287,#48288,
#48289,#48290,#48291,#48292,#48293,#48294,#48295,#48296,#48297,#48298,#48299,
#48300,#48301,#48302,#48303,#48304,#48305,#48306,#48307,#48308,#48309,#48310,
#48311,#48312,#48313,#48314,#48315,#48316,#48317,#48318,#48319,#48320,#48321,
#48322,#48323,#48324,#48325,#48326,#48327,#48328,#48329,#48330,#48331,#48332,
#48333,#48334,#48335,#48336,#48337,#48338,#48339,#48340,#48341,#48342,#48343,
#48344,#48345,#48346,#48347,#48348,#48349,#48350,#48351,#48352,#48353,#48354,
#48355,#48356,#48357,#48358,#48359,#48360,#48361,#48362,#48363,#48364,#48365,
#48366,#48367,#48368,#48369,#48370,#48371,#48372,#48373,#48374,#48375,#48376,
#48377,#48378,#48379,#48380,#48381,#48382,#48383,#48384,#48385,#48386,#48387,
#48388,#48389,#48390,#48391,#48392,#48393,#48394,#48395,#48396,#48397,#48398,
#48399,#48400,#48401,#48402,#48403,#48404,#48405,#48406,#48407,#48408,#48409,
#48410,#48411,#48412,#48413,#48414,#48415,#48416,#48417,#48418,#48419,#48420,
#48421,#48422,#48423,#48424,#48425)) ;
#52526=AXIS2_PLACEMENT_3D('',#88999,#63089,#63090) ;
#52527=AXIS2_PLACEMENT_3D('',#89165,#63091,#63092) ;
#52528=AXIS2_PLACEMENT_3D('',#89259,#63093,#63094) ;
#52529=AXIS2_PLACEMENT_3D('',#89557,#63095,#63096) ;
#52530=AXIS2_PLACEMENT_3D('',#89637,#63097,#63098) ;
#52531=AXIS2_PLACEMENT_3D('',#89873,#63099,#63100) ;
#52532=AXIS2_PLACEMENT_3D('',#89874,#63101,#63102) ;
#52533=AXIS2_PLACEMENT_3D('',#89998,#63112,#63113) ;
#52534=AXIS2_PLACEMENT_3D('',#90004,#63117,#63118) ;
#52535=AXIS2_PLACEMENT_3D('',#90007,#63121,#63122) ;
#52536=AXIS2_PLACEMENT_3D('',#90016,#63127,#63128) ;
#52537=AXIS2_PLACEMENT_3D('',#90114,#63136,#63137) ;
#52538=AXIS2_PLACEMENT_3D('',#90120,#63141,#63142) ;
#52539=AXIS2_PLACEMENT_3D('',#90126,#63146,#63147) ;
#52540=AXIS2_PLACEMENT_3D('',#90293,#63158,#63159) ;
#52541=AXIS2_PLACEMENT_3D('',#90299,#63163,#63164) ;
#52542=AXIS2_PLACEMENT_3D('',#90305,#63168,#63169) ;
#52543=AXIS2_PLACEMENT_3D('',#90308,#63172,#63173) ;
#52544=AXIS2_PLACEMENT_3D('',#90309,#63174,#63175) ;
#52545=AXIS2_PLACEMENT_3D('',#90316,#63178,#63179) ;
#52546=AXIS2_PLACEMENT_3D('',#90320,#63181,#63182) ;
#52547=AXIS2_PLACEMENT_3D('',#90324,#63184,#63185) ;
#52548=AXIS2_PLACEMENT_3D('',#90328,#63187,#63188) ;
#52549=AXIS2_PLACEMENT_3D('',#90330,#63189,#63190) ;
#52550=AXIS2_PLACEMENT_3D('',#90334,#63192,#63193) ;
#52551=AXIS2_PLACEMENT_3D('',#90338,#63195,#63196) ;
#52552=AXIS2_PLACEMENT_3D('',#90342,#63198,#63199) ;
#52553=AXIS2_PLACEMENT_3D('',#90345,#63201,#63202) ;
#52554=AXIS2_PLACEMENT_3D('',#90350,#63204,#63205) ;
#52555=AXIS2_PLACEMENT_3D('',#90364,#63208,#63209) ;
#52556=AXIS2_PLACEMENT_3D('',#90368,#63211,#63212) ;
#52557=AXIS2_PLACEMENT_3D('',#90397,#63215,#63216) ;
#52558=AXIS2_PLACEMENT_3D('',#90400,#63217,#63218) ;
#52559=AXIS2_PLACEMENT_3D('',#90402,#63219,#63220) ;
#52560=AXIS2_PLACEMENT_3D('',#90412,#63221,#63222) ;
#52561=AXIS2_PLACEMENT_3D('',#90413,#63223,#63224) ;
#52562=AXIS2_PLACEMENT_3D('',#90416,#63225,#63226) ;
#52563=AXIS2_PLACEMENT_3D('',#90430,#63229,#63230) ;
#52564=AXIS2_PLACEMENT_3D('',#90431,#63231,#63232) ;
#52565=AXIS2_PLACEMENT_3D('',#90432,#63233,#63234) ;
#52566=AXIS2_PLACEMENT_3D('',#90433,#63235,#63236) ;
#52567=AXIS2_PLACEMENT_3D('',#90436,#63237,#63238) ;
#52568=AXIS2_PLACEMENT_3D('',#90506,#63241,#63242) ;
#52569=AXIS2_PLACEMENT_3D('',#90507,#63243,#63244) ;
#52570=AXIS2_PLACEMENT_3D('',#90517,#63250,#63251) ;
#52571=AXIS2_PLACEMENT_3D('',#90520,#63253,#63254) ;
#52572=AXIS2_PLACEMENT_3D('',#90521,#63255,#63256) ;
#52573=AXIS2_PLACEMENT_3D('',#90559,#63259,#63260) ;
#52574=AXIS2_PLACEMENT_3D('',#90561,#63261,#63262) ;
#52575=AXIS2_PLACEMENT_3D('',#90563,#63263,#63264) ;
#52576=AXIS2_PLACEMENT_3D('',#90591,#63265,#63266) ;
#52577=AXIS2_PLACEMENT_3D('',#90594,#63267,#63268) ;
#52578=AXIS2_PLACEMENT_3D('',#90608,#63271,#63272) ;
#52579=AXIS2_PLACEMENT_3D('',#90609,#63273,#63274) ;
#52580=AXIS2_PLACEMENT_3D('',#90610,#63275,#63276) ;
#52581=AXIS2_PLACEMENT_3D('',#90611,#63277,#63278) ;
#52582=AXIS2_PLACEMENT_3D('',#90614,#63279,#63280) ;
#52583=AXIS2_PLACEMENT_3D('',#90617,#63283,#63284) ;
#52584=AXIS2_PLACEMENT_3D('',#90626,#63285,#63286) ;
#52585=AXIS2_PLACEMENT_3D('',#90627,#63287,#63288) ;
#52586=AXIS2_PLACEMENT_3D('',#90628,#63289,#63290) ;
#52587=AXIS2_PLACEMENT_3D('',#90634,#63294,#63295) ;
#52588=AXIS2_PLACEMENT_3D('',#90637,#63297,#63298) ;
#52589=AXIS2_PLACEMENT_3D('',#90638,#63299,#63300) ;
#52590=AXIS2_PLACEMENT_3D('',#90752,#63304,#63305) ;
#52591=AXIS2_PLACEMENT_3D('',#90753,#63306,#63307) ;
#52592=AXIS2_PLACEMENT_3D('',#90755,#63309,#63310) ;
#52593=AXIS2_PLACEMENT_3D('',#90773,#63311,#63312) ;
#52594=AXIS2_PLACEMENT_3D('',#90783,#63314,#63315) ;
#52595=AXIS2_PLACEMENT_3D('',#90793,#63320,#63321) ;
#52596=AXIS2_PLACEMENT_3D('',#90797,#63323,#63324) ;
#52597=AXIS2_PLACEMENT_3D('',#90826,#63326,#63327) ;
#52598=AXIS2_PLACEMENT_3D('',#90828,#63328,#63329) ;
#52599=AXIS2_PLACEMENT_3D('',#90830,#63330,#63331) ;
#52600=AXIS2_PLACEMENT_3D('',#90832,#63332,#63333) ;
#52601=AXIS2_PLACEMENT_3D('',#90833,#63334,#63335) ;
#52602=AXIS2_PLACEMENT_3D('',#90834,#63336,#63337) ;
#52603=AXIS2_PLACEMENT_3D('',#90837,#63338,#63339) ;
#52604=AXIS2_PLACEMENT_3D('',#90862,#63342,#63343) ;
#52605=AXIS2_PLACEMENT_3D('',#90863,#63344,#63345) ;
#52606=AXIS2_PLACEMENT_3D('',#90864,#63346,#63347) ;
#52607=AXIS2_PLACEMENT_3D('',#90902,#63348,#63349) ;
#52608=AXIS2_PLACEMENT_3D('',#90906,#63351,#63352) ;
#52609=AXIS2_PLACEMENT_3D('',#90908,#63354,#63355) ;
#52610=AXIS2_PLACEMENT_3D('',#90913,#63358,#63359) ;
#52611=AXIS2_PLACEMENT_3D('',#90914,#63360,#63361) ;
#52612=AXIS2_PLACEMENT_3D('',#90917,#63363,#63364) ;
#52613=AXIS2_PLACEMENT_3D('',#90945,#63365,#63366) ;
#52614=AXIS2_PLACEMENT_3D('',#90947,#63367,#63368) ;
#52615=AXIS2_PLACEMENT_3D('',#90949,#63369,#63370) ;
#52616=AXIS2_PLACEMENT_3D('',#90951,#63371,#63372) ;
#52617=AXIS2_PLACEMENT_3D('',#90952,#63373,#63374) ;
#52618=AXIS2_PLACEMENT_3D('',#90953,#63375,#63376) ;
#52619=AXIS2_PLACEMENT_3D('',#90956,#63377,#63378) ;
#52620=AXIS2_PLACEMENT_3D('',#90981,#63381,#63382) ;
#52621=AXIS2_PLACEMENT_3D('',#90982,#63383,#63384) ;
#52622=AXIS2_PLACEMENT_3D('',#90983,#63385,#63386) ;
#52623=AXIS2_PLACEMENT_3D('',#91030,#63387,#63388) ;
#52624=AXIS2_PLACEMENT_3D('',#91036,#63391,#63392) ;
#52625=AXIS2_PLACEMENT_3D('',#91040,#63394,#63395) ;
#52626=AXIS2_PLACEMENT_3D('',#91049,#63400,#63401) ;
#52627=AXIS2_PLACEMENT_3D('',#91053,#63404,#63405) ;
#52628=AXIS2_PLACEMENT_3D('',#91056,#63407,#63408) ;
#52629=AXIS2_PLACEMENT_3D('',#91057,#63409,#63410) ;
#52630=AXIS2_PLACEMENT_3D('',#91061,#63412,#63413) ;
#52631=AXIS2_PLACEMENT_3D('',#91085,#63415,#63416) ;
#52632=AXIS2_PLACEMENT_3D('',#91087,#63417,#63418) ;
#52633=AXIS2_PLACEMENT_3D('',#91088,#63419,#63420) ;
#52634=AXIS2_PLACEMENT_3D('',#91089,#63421,#63422) ;
#52635=AXIS2_PLACEMENT_3D('',#91093,#63424,#63425) ;
#52636=AXIS2_PLACEMENT_3D('',#91095,#63427,#63428) ;
#52637=AXIS2_PLACEMENT_3D('',#91112,#63431,#63432) ;
#52638=AXIS2_PLACEMENT_3D('',#91114,#63434,#63435) ;
#52639=AXIS2_PLACEMENT_3D('',#91124,#63440,#63441) ;
#52640=AXIS2_PLACEMENT_3D('',#91128,#63443,#63444) ;
#52641=AXIS2_PLACEMENT_3D('',#91130,#63446,#63447) ;
#52642=AXIS2_PLACEMENT_3D('',#91132,#63449,#63450) ;
#52643=AXIS2_PLACEMENT_3D('',#91134,#63451,#63452) ;
#52644=AXIS2_PLACEMENT_3D('',#91136,#63454,#63455) ;
#52645=AXIS2_PLACEMENT_3D('',#91138,#63456,#63457) ;
#52646=AXIS2_PLACEMENT_3D('',#91140,#63459,#63460) ;
#52647=AXIS2_PLACEMENT_3D('',#91144,#63462,#63463) ;
#52648=AXIS2_PLACEMENT_3D('',#91146,#63465,#63466) ;
#52649=AXIS2_PLACEMENT_3D('',#91182,#63468,#63469) ;
#52650=AXIS2_PLACEMENT_3D('',#91184,#63470,#63471) ;
#52651=AXIS2_PLACEMENT_3D('',#91186,#63472,#63473) ;
#52652=AXIS2_PLACEMENT_3D('',#91187,#63474,#63475) ;
#52653=AXIS2_PLACEMENT_3D('',#91188,#63476,#63477) ;
#52654=AXIS2_PLACEMENT_3D('',#91191,#63480,#63481) ;
#52655=AXIS2_PLACEMENT_3D('',#91195,#63483,#63484) ;
#52656=AXIS2_PLACEMENT_3D('',#91199,#63487,#63488) ;
#52657=AXIS2_PLACEMENT_3D('',#91202,#63490,#63491) ;
#52658=AXIS2_PLACEMENT_3D('',#91203,#63492,#63493) ;
#52659=AXIS2_PLACEMENT_3D('',#91213,#63499,#63500) ;
#52660=AXIS2_PLACEMENT_3D('',#91215,#63501,#63502) ;
#52661=AXIS2_PLACEMENT_3D('',#91217,#63503,#63504) ;
#52662=AXIS2_PLACEMENT_3D('',#91219,#63505,#63506) ;
#52663=AXIS2_PLACEMENT_3D('',#91220,#63507,#63508) ;
#52664=AXIS2_PLACEMENT_3D('',#91221,#63509,#63510) ;
#52665=AXIS2_PLACEMENT_3D('',#91223,#63512,#63513) ;
#52666=AXIS2_PLACEMENT_3D('',#91227,#63515,#63516) ;
#52667=AXIS2_PLACEMENT_3D('',#91229,#63518,#63519) ;
#52668=AXIS2_PLACEMENT_3D('',#91236,#63523,#63524) ;
#52669=AXIS2_PLACEMENT_3D('',#91237,#63525,#63526) ;
#52670=AXIS2_PLACEMENT_3D('',#91239,#63527,#63528) ;
#52671=AXIS2_PLACEMENT_3D('',#91241,#63529,#63530) ;
#52672=AXIS2_PLACEMENT_3D('',#91242,#63531,#63532) ;
#52673=AXIS2_PLACEMENT_3D('',#91243,#63533,#63534) ;
#52674=AXIS2_PLACEMENT_3D('',#91244,#63535,#63536) ;
#52675=AXIS2_PLACEMENT_3D('',#91245,#63537,#63538) ;
#52676=AXIS2_PLACEMENT_3D('',#91247,#63539,#63540) ;
#52677=AXIS2_PLACEMENT_3D('',#91249,#63542,#63543) ;
#52678=AXIS2_PLACEMENT_3D('',#91251,#63544,#63545) ;
#52679=AXIS2_PLACEMENT_3D('',#91253,#63546,#63547) ;
#52680=AXIS2_PLACEMENT_3D('',#91254,#63548,#63549) ;
#52681=AXIS2_PLACEMENT_3D('',#91255,#63550,#63551) ;
#52682=AXIS2_PLACEMENT_3D('',#91257,#63552,#63553) ;
#52683=AXIS2_PLACEMENT_3D('',#91258,#63554,#63555) ;
#52684=AXIS2_PLACEMENT_3D('',#91259,#63556,#63557) ;
#52685=AXIS2_PLACEMENT_3D('',#91261,#63559,#63560) ;
#52686=AXIS2_PLACEMENT_3D('',#91263,#63561,#63562) ;
#52687=AXIS2_PLACEMENT_3D('',#91265,#63563,#63564) ;
#52688=AXIS2_PLACEMENT_3D('',#91266,#63565,#63566) ;
#52689=AXIS2_PLACEMENT_3D('',#91267,#63567,#63568) ;
#52690=AXIS2_PLACEMENT_3D('',#91270,#63569,#63570) ;
#52691=AXIS2_PLACEMENT_3D('',#91273,#63573,#63574) ;
#52692=AXIS2_PLACEMENT_3D('',#91275,#63575,#63576) ;
#52693=AXIS2_PLACEMENT_3D('',#91276,#63577,#63578) ;
#52694=AXIS2_PLACEMENT_3D('',#91277,#63579,#63580) ;
#52695=AXIS2_PLACEMENT_3D('',#91278,#63581,#63582) ;
#52696=AXIS2_PLACEMENT_3D('',#91280,#63584,#63585) ;
#52697=AXIS2_PLACEMENT_3D('',#91292,#63592,#63593) ;
#52698=AXIS2_PLACEMENT_3D('',#91295,#63595,#63596) ;
#52699=AXIS2_PLACEMENT_3D('',#91296,#63597,#63598) ;
#52700=AXIS2_PLACEMENT_3D('',#91300,#63600,#63601) ;
#52701=AXIS2_PLACEMENT_3D('',#91307,#63605,#63606) ;
#52702=AXIS2_PLACEMENT_3D('',#91308,#63607,#63608) ;
#52703=AXIS2_PLACEMENT_3D('',#91319,#63609,#63610) ;
#52704=AXIS2_PLACEMENT_3D('',#91322,#63611,#63612) ;
#52705=AXIS2_PLACEMENT_3D('',#91324,#63613,#63614) ;
#52706=AXIS2_PLACEMENT_3D('',#91325,#63615,#63616) ;
#52707=AXIS2_PLACEMENT_3D('',#91326,#63617,#63618) ;
#52708=AXIS2_PLACEMENT_3D('',#91329,#63619,#63620) ;
#52709=AXIS2_PLACEMENT_3D('',#91332,#63623,#63624) ;
#52710=AXIS2_PLACEMENT_3D('',#91352,#63625,#63626) ;
#52711=AXIS2_PLACEMENT_3D('',#91354,#63627,#63628) ;
#52712=AXIS2_PLACEMENT_3D('',#91355,#63629,#63630) ;
#52713=AXIS2_PLACEMENT_3D('',#91356,#63631,#63632) ;
#52714=AXIS2_PLACEMENT_3D('',#91359,#63633,#63634) ;
#52715=AXIS2_PLACEMENT_3D('',#91362,#63637,#63638) ;
#52716=AXIS2_PLACEMENT_3D('',#91365,#63639,#63640) ;
#52717=AXIS2_PLACEMENT_3D('',#91366,#63641,#63642) ;
#52718=AXIS2_PLACEMENT_3D('',#91367,#63643,#63644) ;
#52719=AXIS2_PLACEMENT_3D('',#91368,#63645,#63646) ;
#52720=AXIS2_PLACEMENT_3D('',#91371,#63647,#63648) ;
#52721=AXIS2_PLACEMENT_3D('',#91372,#63649,#63650) ;
#52722=AXIS2_PLACEMENT_3D('',#91373,#63651,#63652) ;
#52723=AXIS2_PLACEMENT_3D('',#91374,#63653,#63654) ;
#52724=AXIS2_PLACEMENT_3D('',#91377,#63655,#63656) ;
#52725=AXIS2_PLACEMENT_3D('',#91380,#63659,#63660) ;
#52726=AXIS2_PLACEMENT_3D('',#91383,#63661,#63662) ;
#52727=AXIS2_PLACEMENT_3D('',#91384,#63663,#63664) ;
#52728=AXIS2_PLACEMENT_3D('',#91385,#63665,#63666) ;
#52729=AXIS2_PLACEMENT_3D('',#91386,#63667,#63668) ;
#52730=AXIS2_PLACEMENT_3D('',#91389,#63671,#63672) ;
#52731=AXIS2_PLACEMENT_3D('',#91392,#63673,#63674) ;
#52732=AXIS2_PLACEMENT_3D('',#91395,#63677,#63678) ;
#52733=AXIS2_PLACEMENT_3D('',#91404,#63679,#63680) ;
#52734=AXIS2_PLACEMENT_3D('',#91405,#63681,#63682) ;
#52735=AXIS2_PLACEMENT_3D('',#91406,#63683,#63684) ;
#52736=AXIS2_PLACEMENT_3D('',#91410,#63686,#63687) ;
#52737=AXIS2_PLACEMENT_3D('',#91414,#63689,#63690) ;
#52738=AXIS2_PLACEMENT_3D('',#91422,#63694,#63695) ;
#52739=AXIS2_PLACEMENT_3D('',#91424,#63696,#63697) ;
#52740=AXIS2_PLACEMENT_3D('',#91425,#63698,#63699) ;
#52741=AXIS2_PLACEMENT_3D('',#91426,#63700,#63701) ;
#52742=AXIS2_PLACEMENT_3D('',#91429,#63703,#63704) ;
#52743=AXIS2_PLACEMENT_3D('',#91430,#63705,#63706) ;
#52744=AXIS2_PLACEMENT_3D('',#91434,#63709,#63710) ;
#52745=AXIS2_PLACEMENT_3D('',#91437,#63711,#63712) ;
#52746=AXIS2_PLACEMENT_3D('',#91441,#63714,#63715) ;
#52747=AXIS2_PLACEMENT_3D('',#91444,#63717,#63718) ;
#52748=AXIS2_PLACEMENT_3D('',#91512,#63719,#63720) ;
#52749=AXIS2_PLACEMENT_3D('',#91514,#63721,#63722) ;
#52750=AXIS2_PLACEMENT_3D('',#91517,#63724,#63725) ;
#52751=AXIS2_PLACEMENT_3D('',#91518,#63726,#63727) ;
#52752=AXIS2_PLACEMENT_3D('',#91522,#63729,#63730) ;
#52753=AXIS2_PLACEMENT_3D('',#91572,#63732,#63733) ;
#52754=AXIS2_PLACEMENT_3D('',#91578,#63737,#63738) ;
#52755=AXIS2_PLACEMENT_3D('',#91581,#63739,#63740) ;
#52756=AXIS2_PLACEMENT_3D('',#91582,#63741,#63742) ;
#52757=AXIS2_PLACEMENT_3D('',#91584,#63743,#63744) ;
#52758=AXIS2_PLACEMENT_3D('',#91585,#63745,#63746) ;
#52759=AXIS2_PLACEMENT_3D('',#91586,#63747,#63748) ;
#52760=AXIS2_PLACEMENT_3D('',#91588,#63749,#63750) ;
#52761=AXIS2_PLACEMENT_3D('',#91590,#63752,#63753) ;
#52762=AXIS2_PLACEMENT_3D('',#91591,#63754,#63755) ;
#52763=AXIS2_PLACEMENT_3D('',#91592,#63756,#63757) ;
#52764=AXIS2_PLACEMENT_3D('',#91594,#63758,#63759) ;
#52765=AXIS2_PLACEMENT_3D('',#91622,#63761,#63762) ;
#52766=AXIS2_PLACEMENT_3D('',#91649,#63763,#63764) ;
#52767=AXIS2_PLACEMENT_3D('',#91650,#63765,#63766) ;
#52768=AXIS2_PLACEMENT_3D('',#91651,#63767,#63768) ;
#52769=AXIS2_PLACEMENT_3D('',#91652,#63769,#63770) ;
#52770=AXIS2_PLACEMENT_3D('',#91655,#63771,#63772) ;
#52771=AXIS2_PLACEMENT_3D('',#91695,#63775,#63776) ;
#52772=AXIS2_PLACEMENT_3D('',#91697,#63777,#63778) ;
#52773=AXIS2_PLACEMENT_3D('',#91704,#63779,#63780) ;
#52774=AXIS2_PLACEMENT_3D('',#91706,#63781,#63782) ;
#52775=AXIS2_PLACEMENT_3D('',#91708,#63783,#63784) ;
#52776=AXIS2_PLACEMENT_3D('',#91709,#63785,#63786) ;
#52777=AXIS2_PLACEMENT_3D('',#91710,#63787,#63788) ;
#52778=AXIS2_PLACEMENT_3D('',#91712,#63789,#63790) ;
#52779=AXIS2_PLACEMENT_3D('',#91714,#63792,#63793) ;
#52780=AXIS2_PLACEMENT_3D('',#91716,#63794,#63795) ;
#52781=AXIS2_PLACEMENT_3D('',#91717,#63796,#63797) ;
#52782=AXIS2_PLACEMENT_3D('',#91718,#63798,#63799) ;
#52783=AXIS2_PLACEMENT_3D('',#91720,#63800,#63801) ;
#52784=AXIS2_PLACEMENT_3D('',#91722,#63803,#63804) ;
#52785=AXIS2_PLACEMENT_3D('',#91725,#63805,#63806) ;
#52786=AXIS2_PLACEMENT_3D('',#91726,#63807,#63808) ;
#52787=AXIS2_PLACEMENT_3D('',#91727,#63809,#63810) ;
#52788=AXIS2_PLACEMENT_3D('',#91728,#63811,#63812) ;
#52789=AXIS2_PLACEMENT_3D('',#91731,#63813,#63814) ;
#52790=AXIS2_PLACEMENT_3D('',#91734,#63817,#63818) ;
#52791=AXIS2_PLACEMENT_3D('',#91735,#63819,#63820) ;
#52792=AXIS2_PLACEMENT_3D('',#91736,#63821,#63822) ;
#52793=AXIS2_PLACEMENT_3D('',#91737,#63823,#63824) ;
#52794=AXIS2_PLACEMENT_3D('',#91740,#63826,#63827) ;
#52795=AXIS2_PLACEMENT_3D('',#91741,#63828,#63829) ;
#52796=AXIS2_PLACEMENT_3D('',#91745,#63832,#63833) ;
#52797=AXIS2_PLACEMENT_3D('',#91748,#63835,#63836) ;
#52798=AXIS2_PLACEMENT_3D('',#91749,#63837,#63838) ;
#52799=AXIS2_PLACEMENT_3D('',#91757,#63843,#63844) ;
#52800=AXIS2_PLACEMENT_3D('',#91760,#63846,#63847) ;
#52801=AXIS2_PLACEMENT_3D('',#91761,#63848,#63849) ;
#52802=AXIS2_PLACEMENT_3D('',#91763,#63850,#63851) ;
#52803=AXIS2_PLACEMENT_3D('',#91791,#63853,#63854) ;
#52804=AXIS2_PLACEMENT_3D('',#91853,#63855,#63856) ;
#52805=AXIS2_PLACEMENT_3D('',#91854,#63857,#63858) ;
#52806=AXIS2_PLACEMENT_3D('',#91855,#63859,#63860) ;
#52807=AXIS2_PLACEMENT_3D('',#91856,#63861,#63862) ;
#52808=AXIS2_PLACEMENT_3D('',#91859,#63863,#63864) ;
#52809=AXIS2_PLACEMENT_3D('',#91884,#63867,#63868) ;
#52810=AXIS2_PLACEMENT_3D('',#91885,#63869,#63870) ;
#52811=AXIS2_PLACEMENT_3D('',#91886,#63871,#63872) ;
#52812=AXIS2_PLACEMENT_3D('',#91909,#63873,#63874) ;
#52813=AXIS2_PLACEMENT_3D('',#91910,#63875,#63876) ;
#52814=AXIS2_PLACEMENT_3D('',#91911,#63877,#63878) ;
#52815=AXIS2_PLACEMENT_3D('',#91929,#63879,#63880) ;
#52816=AXIS2_PLACEMENT_3D('',#91941,#63881,#63882) ;
#52817=AXIS2_PLACEMENT_3D('',#91942,#63883,#63884) ;
#52818=AXIS2_PLACEMENT_3D('',#91951,#63886,#63887) ;
#52819=AXIS2_PLACEMENT_3D('',#91953,#63889,#63890) ;
#52820=AXIS2_PLACEMENT_3D('',#91971,#63895,#63896) ;
#52821=AXIS2_PLACEMENT_3D('',#91972,#63897,#63898) ;
#52822=AXIS2_PLACEMENT_3D('',#91974,#63900,#63901) ;
#52823=AXIS2_PLACEMENT_3D('',#91977,#63903,#63904) ;
#52824=AXIS2_PLACEMENT_3D('',#91978,#63905,#63906) ;
#52825=AXIS2_PLACEMENT_3D('',#91980,#63907,#63908) ;
#52826=AXIS2_PLACEMENT_3D('',#91997,#63910,#63911) ;
#52827=AXIS2_PLACEMENT_3D('',#91999,#63912,#63913) ;
#52828=AXIS2_PLACEMENT_3D('',#92014,#63914,#63915) ;
#52829=AXIS2_PLACEMENT_3D('',#92017,#63917,#63918) ;
#52830=AXIS2_PLACEMENT_3D('',#92018,#63919,#63920) ;
#52831=AXIS2_PLACEMENT_3D('',#92020,#63922,#63923) ;
#52832=AXIS2_PLACEMENT_3D('',#92024,#63925,#63926) ;
#52833=AXIS2_PLACEMENT_3D('',#92026,#63928,#63929) ;
#52834=AXIS2_PLACEMENT_3D('',#92030,#63932,#63933) ;
#52835=AXIS2_PLACEMENT_3D('',#92053,#63934,#63935) ;
#52836=AXIS2_PLACEMENT_3D('',#92055,#63936,#63937) ;
#52837=AXIS2_PLACEMENT_3D('',#92056,#63938,#63939) ;
#52838=AXIS2_PLACEMENT_3D('',#92057,#63940,#63941) ;
#52839=AXIS2_PLACEMENT_3D('',#92060,#63942,#63943) ;
#52840=AXIS2_PLACEMENT_3D('',#92061,#63944,#63945) ;
#52841=AXIS2_PLACEMENT_3D('',#92062,#63946,#63947) ;
#52842=AXIS2_PLACEMENT_3D('',#92063,#63948,#63949) ;
#52843=AXIS2_PLACEMENT_3D('',#92090,#63952,#63953) ;
#52844=AXIS2_PLACEMENT_3D('',#92100,#63959,#63960) ;
#52845=AXIS2_PLACEMENT_3D('',#92103,#63962,#63963) ;
#52846=AXIS2_PLACEMENT_3D('',#92104,#63964,#63965) ;
#52847=AXIS2_PLACEMENT_3D('',#92108,#63967,#63968) ;
#52848=AXIS2_PLACEMENT_3D('',#92110,#63970,#63971) ;
#52849=AXIS2_PLACEMENT_3D('',#92113,#63972,#63973) ;
#52850=AXIS2_PLACEMENT_3D('',#92115,#63974,#63975) ;
#52851=AXIS2_PLACEMENT_3D('',#92116,#63976,#63977) ;
#52852=AXIS2_PLACEMENT_3D('',#92117,#63978,#63979) ;
#52853=AXIS2_PLACEMENT_3D('',#92120,#63982,#63983) ;
#52854=AXIS2_PLACEMENT_3D('',#92123,#63986,#63987) ;
#52855=AXIS2_PLACEMENT_3D('',#92126,#63988,#63989) ;
#52856=AXIS2_PLACEMENT_3D('',#92128,#63990,#63991) ;
#52857=AXIS2_PLACEMENT_3D('',#92130,#63992,#63993) ;
#52858=AXIS2_PLACEMENT_3D('',#92131,#63994,#63995) ;
#52859=AXIS2_PLACEMENT_3D('',#92132,#63996,#63997) ;
#52860=AXIS2_PLACEMENT_3D('',#92135,#64000,#64001) ;
#52861=AXIS2_PLACEMENT_3D('',#92138,#64004,#64005) ;
#52862=AXIS2_PLACEMENT_3D('',#92141,#64008,#64009) ;
#52863=AXIS2_PLACEMENT_3D('',#92145,#64011,#64012) ;
#52864=AXIS2_PLACEMENT_3D('',#92149,#64014,#64015) ;
#52865=AXIS2_PLACEMENT_3D('',#92153,#64017,#64018) ;
#52866=AXIS2_PLACEMENT_3D('',#92157,#64020,#64021) ;
#52867=AXIS2_PLACEMENT_3D('',#92169,#64027,#64028) ;
#52868=AXIS2_PLACEMENT_3D('',#92173,#64030,#64031) ;
#52869=AXIS2_PLACEMENT_3D('',#92177,#64033,#64034) ;
#52870=AXIS2_PLACEMENT_3D('',#92181,#64036,#64037) ;
#52871=AXIS2_PLACEMENT_3D('',#92185,#64039,#64040) ;
#52872=AXIS2_PLACEMENT_3D('',#92189,#64042,#64043) ;
#52873=AXIS2_PLACEMENT_3D('',#92197,#64047,#64048) ;
#52874=AXIS2_PLACEMENT_3D('',#92201,#64050,#64051) ;
#52875=AXIS2_PLACEMENT_3D('',#92205,#64053,#64054) ;
#52876=AXIS2_PLACEMENT_3D('',#92209,#64056,#64057) ;
#52877=AXIS2_PLACEMENT_3D('',#92213,#64059,#64060) ;
#52878=AXIS2_PLACEMENT_3D('',#92249,#64071,#64072) ;
#52879=AXIS2_PLACEMENT_3D('',#92253,#64074,#64075) ;
#52880=AXIS2_PLACEMENT_3D('',#92259,#64078,#64079) ;
#52881=AXIS2_PLACEMENT_3D('',#92265,#64082,#64083) ;
#52882=AXIS2_PLACEMENT_3D('',#92282,#64088,#64089) ;
#52883=AXIS2_PLACEMENT_3D('',#92284,#64090,#64091) ;
#52884=AXIS2_PLACEMENT_3D('',#92286,#64092,#64093) ;
#52885=AXIS2_PLACEMENT_3D('',#92288,#64094,#64095) ;
#52886=AXIS2_PLACEMENT_3D('',#92292,#64097,#64098) ;
#52887=AXIS2_PLACEMENT_3D('',#92298,#64101,#64102) ;
#52888=AXIS2_PLACEMENT_3D('',#92302,#64104,#64105) ;
#52889=AXIS2_PLACEMENT_3D('',#92308,#64108,#64109) ;
#52890=AXIS2_PLACEMENT_3D('',#92312,#64111,#64112) ;
#52891=AXIS2_PLACEMENT_3D('',#92320,#64116,#64117) ;
#52892=AXIS2_PLACEMENT_3D('',#92324,#64119,#64120) ;
#52893=AXIS2_PLACEMENT_3D('',#92328,#64122,#64123) ;
#52894=AXIS2_PLACEMENT_3D('',#92332,#64125,#64126) ;
#52895=AXIS2_PLACEMENT_3D('',#92337,#64129,#64130) ;
#52896=AXIS2_PLACEMENT_3D('',#92339,#64131,#64132) ;
#52897=AXIS2_PLACEMENT_3D('',#92343,#64134,#64135) ;
#52898=AXIS2_PLACEMENT_3D('',#92349,#64138,#64139) ;
#52899=AXIS2_PLACEMENT_3D('',#92353,#64141,#64142) ;
#52900=AXIS2_PLACEMENT_3D('',#92355,#64143,#64144) ;
#52901=AXIS2_PLACEMENT_3D('',#92361,#64147,#64148) ;
#52902=AXIS2_PLACEMENT_3D('',#92365,#64150,#64151) ;
#52903=AXIS2_PLACEMENT_3D('',#92369,#64153,#64154) ;
#52904=AXIS2_PLACEMENT_3D('',#92373,#64156,#64157) ;
#52905=AXIS2_PLACEMENT_3D('',#92376,#64159,#64160) ;
#52906=AXIS2_PLACEMENT_3D('',#92379,#64161,#64162) ;
#52907=AXIS2_PLACEMENT_3D('',#92383,#64164,#64165) ;
#52908=AXIS2_PLACEMENT_3D('',#92389,#64168,#64169) ;
#52909=AXIS2_PLACEMENT_3D('',#92393,#64171,#64172) ;
#52910=AXIS2_PLACEMENT_3D('',#92397,#64174,#64175) ;
#52911=AXIS2_PLACEMENT_3D('',#92401,#64177,#64178) ;
#52912=AXIS2_PLACEMENT_3D('',#92406,#64181,#64182) ;
#52913=AXIS2_PLACEMENT_3D('',#92420,#64185,#64186) ;
#52914=AXIS2_PLACEMENT_3D('',#92424,#64188,#64189) ;
#52915=AXIS2_PLACEMENT_3D('',#92428,#64191,#64192) ;
#52916=AXIS2_PLACEMENT_3D('',#92432,#64194,#64195) ;
#52917=AXIS2_PLACEMENT_3D('',#92455,#64200,#64201) ;
#52918=AXIS2_PLACEMENT_3D('',#92459,#64203,#64204) ;
#52919=AXIS2_PLACEMENT_3D('',#92463,#64206,#64207) ;
#52920=AXIS2_PLACEMENT_3D('',#92467,#64209,#64210) ;
#52921=AXIS2_PLACEMENT_3D('',#92473,#64213,#64214) ;
#52922=AXIS2_PLACEMENT_3D('',#92477,#64216,#64217) ;
#52923=AXIS2_PLACEMENT_3D('',#92483,#64220,#64221) ;
#52924=AXIS2_PLACEMENT_3D('',#92487,#64223,#64224) ;
#52925=AXIS2_PLACEMENT_3D('',#92491,#64226,#64227) ;
#52926=AXIS2_PLACEMENT_3D('',#92495,#64229,#64230) ;
#52927=AXIS2_PLACEMENT_3D('',#92499,#64233,#64234) ;
#52928=AXIS2_PLACEMENT_3D('',#92567,#64235,#64236) ;
#52929=AXIS2_PLACEMENT_3D('',#92576,#64237,#64238) ;
#52930=AXIS2_PLACEMENT_3D('',#92577,#64239,#64240) ;
#52931=AXIS2_PLACEMENT_3D('',#92580,#64243,#64244) ;
#52932=AXIS2_PLACEMENT_3D('',#92601,#64245,#64246) ;
#52933=AXIS2_PLACEMENT_3D('',#92602,#64247,#64248) ;
#52934=AXIS2_PLACEMENT_3D('',#92604,#64249,#64250) ;
#52935=AXIS2_PLACEMENT_3D('',#92605,#64251,#64252) ;
#52936=AXIS2_PLACEMENT_3D('',#92606,#64253,#64254) ;
#52937=AXIS2_PLACEMENT_3D('',#92608,#64255,#64256) ;
#52938=AXIS2_PLACEMENT_3D('',#92610,#64258,#64259) ;
#52939=AXIS2_PLACEMENT_3D('',#92612,#64261,#64262) ;
#52940=AXIS2_PLACEMENT_3D('',#92616,#64264,#64265) ;
#52941=AXIS2_PLACEMENT_3D('',#92618,#64267,#64268) ;
#52942=AXIS2_PLACEMENT_3D('',#92625,#64273,#64274) ;
#52943=AXIS2_PLACEMENT_3D('',#92632,#64279,#64280) ;
#52944=AXIS2_PLACEMENT_3D('',#92635,#64281,#64282) ;
#52945=AXIS2_PLACEMENT_3D('',#92637,#64283,#64284) ;
#52946=AXIS2_PLACEMENT_3D('',#92638,#64285,#64286) ;
#52947=AXIS2_PLACEMENT_3D('',#92639,#64287,#64288) ;
#52948=AXIS2_PLACEMENT_3D('',#92643,#64290,#64291) ;
#52949=AXIS2_PLACEMENT_3D('',#92645,#64293,#64294) ;
#52950=AXIS2_PLACEMENT_3D('',#92648,#64295,#64296) ;
#52951=AXIS2_PLACEMENT_3D('',#92649,#64297,#64298) ;
#52952=AXIS2_PLACEMENT_3D('',#92650,#64299,#64300) ;
#52953=AXIS2_PLACEMENT_3D('',#92651,#64301,#64302) ;
#52954=AXIS2_PLACEMENT_3D('',#92654,#64303,#64304) ;
#52955=AXIS2_PLACEMENT_3D('',#92657,#64307,#64308) ;
#52956=AXIS2_PLACEMENT_3D('',#92660,#64309,#64310) ;
#52957=AXIS2_PLACEMENT_3D('',#92661,#64311,#64312) ;
#52958=AXIS2_PLACEMENT_3D('',#92662,#64313,#64314) ;
#52959=AXIS2_PLACEMENT_3D('',#92663,#64315,#64316) ;
#52960=AXIS2_PLACEMENT_3D('',#92666,#64319,#64320) ;
#52961=AXIS2_PLACEMENT_3D('',#92686,#64322,#64323) ;
#52962=AXIS2_PLACEMENT_3D('',#92688,#64325,#64326) ;
#52963=AXIS2_PLACEMENT_3D('',#92691,#64327,#64328) ;
#52964=AXIS2_PLACEMENT_3D('',#92692,#64329,#64330) ;
#52965=AXIS2_PLACEMENT_3D('',#92693,#64331,#64332) ;
#52966=AXIS2_PLACEMENT_3D('',#92694,#64333,#64334) ;
#52967=AXIS2_PLACEMENT_3D('',#92747,#64337,#64338) ;
#52968=AXIS2_PLACEMENT_3D('',#92749,#64339,#64340) ;
#52969=AXIS2_PLACEMENT_3D('',#92751,#64341,#64342) ;
#52970=AXIS2_PLACEMENT_3D('',#92752,#64343,#64344) ;
#52971=AXIS2_PLACEMENT_3D('',#92753,#64345,#64346) ;
#52972=AXIS2_PLACEMENT_3D('',#92755,#64347,#64348) ;
#52973=AXIS2_PLACEMENT_3D('',#92756,#64349,#64350) ;
#52974=AXIS2_PLACEMENT_3D('',#92767,#64351,#64352) ;
#52975=AXIS2_PLACEMENT_3D('',#92768,#64353,#64354) ;
#52976=AXIS2_PLACEMENT_3D('',#92769,#64355,#64356) ;
#52977=AXIS2_PLACEMENT_3D('',#92771,#64357,#64358) ;
#52978=AXIS2_PLACEMENT_3D('',#92773,#64360,#64361) ;
#52979=AXIS2_PLACEMENT_3D('',#92775,#64362,#64363) ;
#52980=AXIS2_PLACEMENT_3D('',#92776,#64364,#64365) ;
#52981=AXIS2_PLACEMENT_3D('',#92777,#64366,#64367) ;
#52982=AXIS2_PLACEMENT_3D('',#92779,#64369,#64370) ;
#52983=AXIS2_PLACEMENT_3D('',#92782,#64373,#64374) ;
#52984=AXIS2_PLACEMENT_3D('',#92784,#64375,#64376) ;
#52985=AXIS2_PLACEMENT_3D('',#92786,#64378,#64379) ;
#52986=AXIS2_PLACEMENT_3D('',#92788,#64380,#64381) ;
#52987=AXIS2_PLACEMENT_3D('',#92789,#64382,#64383) ;
#52988=AXIS2_PLACEMENT_3D('',#92790,#64384,#64385) ;
#52989=AXIS2_PLACEMENT_3D('',#92792,#64386,#64387) ;
#52990=AXIS2_PLACEMENT_3D('',#92839,#64389,#64390) ;
#52991=AXIS2_PLACEMENT_3D('',#92844,#64393,#64394) ;
#52992=AXIS2_PLACEMENT_3D('',#92845,#64395,#64396) ;
#52993=AXIS2_PLACEMENT_3D('',#92852,#64400,#64401) ;
#52994=AXIS2_PLACEMENT_3D('',#92853,#64402,#64403) ;
#52995=AXIS2_PLACEMENT_3D('',#92856,#64405,#64406) ;
#52996=AXIS2_PLACEMENT_3D('',#92857,#64407,#64408) ;
#52997=AXIS2_PLACEMENT_3D('',#92861,#64411,#64412) ;
#52998=AXIS2_PLACEMENT_3D('',#92864,#64414,#64415) ;
#52999=AXIS2_PLACEMENT_3D('',#92865,#64416,#64417) ;
#53000=AXIS2_PLACEMENT_3D('',#92871,#64420,#64421) ;
#53001=AXIS2_PLACEMENT_3D('',#92875,#64423,#64424) ;
#53002=AXIS2_PLACEMENT_3D('',#92879,#64426,#64427) ;
#53003=AXIS2_PLACEMENT_3D('',#92881,#64429,#64430) ;
#53004=AXIS2_PLACEMENT_3D('',#92884,#64432,#64433) ;
#53005=AXIS2_PLACEMENT_3D('',#92885,#64434,#64435) ;
#53006=AXIS2_PLACEMENT_3D('',#92889,#64438,#64439) ;
#53007=AXIS2_PLACEMENT_3D('',#92892,#64441,#64442) ;
#53008=AXIS2_PLACEMENT_3D('',#92893,#64443,#64444) ;
#53009=AXIS2_PLACEMENT_3D('',#92895,#64445,#64446) ;
#53010=AXIS2_PLACEMENT_3D('',#92901,#64447,#64448) ;
#53011=AXIS2_PLACEMENT_3D('',#92934,#64449,#64450) ;
#53012=AXIS2_PLACEMENT_3D('',#92962,#64451,#64452) ;
#53013=AXIS2_PLACEMENT_3D('',#92969,#64453,#64454) ;
#53014=AXIS2_PLACEMENT_3D('',#92972,#64455,#64456) ;
#53015=AXIS2_PLACEMENT_3D('',#92975,#64459,#64460) ;
#53016=AXIS2_PLACEMENT_3D('',#92978,#64461,#64462) ;
#53017=AXIS2_PLACEMENT_3D('',#92980,#64463,#64464) ;
#53018=AXIS2_PLACEMENT_3D('',#92982,#64465,#64466) ;
#53019=AXIS2_PLACEMENT_3D('',#92983,#64467,#64468) ;
#53020=AXIS2_PLACEMENT_3D('',#92984,#64469,#64470) ;
#53021=AXIS2_PLACEMENT_3D('',#92987,#64471,#64472) ;
#53022=AXIS2_PLACEMENT_3D('',#92990,#64475,#64476) ;
#53023=AXIS2_PLACEMENT_3D('',#92991,#64477,#64478) ;
#53024=AXIS2_PLACEMENT_3D('',#92992,#64479,#64480) ;
#53025=AXIS2_PLACEMENT_3D('',#92993,#64481,#64482) ;
#53026=AXIS2_PLACEMENT_3D('',#92996,#64483,#64484) ;
#53027=AXIS2_PLACEMENT_3D('',#92998,#64485,#64486) ;
#53028=AXIS2_PLACEMENT_3D('',#93000,#64487,#64488) ;
#53029=AXIS2_PLACEMENT_3D('',#93001,#64489,#64490) ;
#53030=AXIS2_PLACEMENT_3D('',#93060,#64491,#64492) ;
#53031=AXIS2_PLACEMENT_3D('',#93068,#64493,#64494) ;
#53032=AXIS2_PLACEMENT_3D('',#93069,#64495,#64496) ;
#53033=AXIS2_PLACEMENT_3D('',#93072,#64497,#64498) ;
#53034=AXIS2_PLACEMENT_3D('',#93073,#64499,#64500) ;
#53035=AXIS2_PLACEMENT_3D('',#93074,#64501,#64502) ;
#53036=AXIS2_PLACEMENT_3D('',#93075,#64503,#64504) ;
#53037=AXIS2_PLACEMENT_3D('',#93078,#64507,#64508) ;
#53038=AXIS2_PLACEMENT_3D('',#93081,#64509,#64510) ;
#53039=AXIS2_PLACEMENT_3D('',#93110,#64513,#64514) ;
#53040=AXIS2_PLACEMENT_3D('',#93142,#64515,#64516) ;
#53041=AXIS2_PLACEMENT_3D('',#93143,#64517,#64518) ;
#53042=AXIS2_PLACEMENT_3D('',#93144,#64519,#64520) ;
#53043=AXIS2_PLACEMENT_3D('',#93146,#64522,#64523) ;
#53044=AXIS2_PLACEMENT_3D('',#93149,#64524,#64525) ;
#53045=AXIS2_PLACEMENT_3D('',#93152,#64528,#64529) ;
#53046=AXIS2_PLACEMENT_3D('',#93154,#64530,#64531) ;
#53047=AXIS2_PLACEMENT_3D('',#93155,#64532,#64533) ;
#53048=AXIS2_PLACEMENT_3D('',#93156,#64534,#64535) ;
#53049=AXIS2_PLACEMENT_3D('',#93158,#64536,#64537) ;
#53050=AXIS2_PLACEMENT_3D('',#93160,#64539,#64540) ;
#53051=AXIS2_PLACEMENT_3D('',#93162,#64541,#64542) ;
#53052=AXIS2_PLACEMENT_3D('',#93163,#64543,#64544) ;
#53053=AXIS2_PLACEMENT_3D('',#93164,#64545,#64546) ;
#53054=AXIS2_PLACEMENT_3D('',#93166,#64548,#64549) ;
#53055=AXIS2_PLACEMENT_3D('',#93169,#64550,#64551) ;
#53056=AXIS2_PLACEMENT_3D('',#93172,#64554,#64555) ;
#53057=AXIS2_PLACEMENT_3D('',#93175,#64556,#64557) ;
#53058=AXIS2_PLACEMENT_3D('',#93178,#64560,#64561) ;
#53059=AXIS2_PLACEMENT_3D('',#93181,#64562,#64563) ;
#53060=AXIS2_PLACEMENT_3D('',#93182,#64564,#64565) ;
#53061=AXIS2_PLACEMENT_3D('',#93183,#64566,#64567) ;
#53062=AXIS2_PLACEMENT_3D('',#93184,#64568,#64569) ;
#53063=AXIS2_PLACEMENT_3D('',#93187,#64570,#64571) ;
#53064=AXIS2_PLACEMENT_3D('',#93190,#64574,#64575) ;
#53065=AXIS2_PLACEMENT_3D('',#93193,#64576,#64577) ;
#53066=AXIS2_PLACEMENT_3D('',#93194,#64578,#64579) ;
#53067=AXIS2_PLACEMENT_3D('',#93195,#64580,#64581) ;
#53068=AXIS2_PLACEMENT_3D('',#93196,#64582,#64583) ;
#53069=AXIS2_PLACEMENT_3D('',#93199,#64584,#64585) ;
#53070=AXIS2_PLACEMENT_3D('',#93202,#64588,#64589) ;
#53071=AXIS2_PLACEMENT_3D('',#93205,#64590,#64591) ;
#53072=AXIS2_PLACEMENT_3D('',#93206,#64592,#64593) ;
#53073=AXIS2_PLACEMENT_3D('',#93207,#64594,#64595) ;
#53074=AXIS2_PLACEMENT_3D('',#93208,#64596,#64597) ;
#53075=AXIS2_PLACEMENT_3D('',#93211,#64598,#64599) ;
#53076=AXIS2_PLACEMENT_3D('',#93214,#64602,#64603) ;
#53077=AXIS2_PLACEMENT_3D('',#93217,#64604,#64605) ;
#53078=AXIS2_PLACEMENT_3D('',#93218,#64606,#64607) ;
#53079=AXIS2_PLACEMENT_3D('',#93219,#64608,#64609) ;
#53080=AXIS2_PLACEMENT_3D('',#93220,#64610,#64611) ;
#53081=AXIS2_PLACEMENT_3D('',#93223,#64614,#64615) ;
#53082=AXIS2_PLACEMENT_3D('',#93226,#64616,#64617) ;
#53083=AXIS2_PLACEMENT_3D('',#93260,#64620,#64621) ;
#53084=AXIS2_PLACEMENT_3D('',#93286,#64622,#64623) ;
#53085=AXIS2_PLACEMENT_3D('',#93287,#64624,#64625) ;
#53086=AXIS2_PLACEMENT_3D('',#93290,#64626,#64627) ;
#53087=AXIS2_PLACEMENT_3D('',#93293,#64630,#64631) ;
#53088=AXIS2_PLACEMENT_3D('',#93295,#64632,#64633) ;
#53089=AXIS2_PLACEMENT_3D('',#93297,#64635,#64636) ;
#53090=AXIS2_PLACEMENT_3D('',#93304,#64638,#64639) ;
#53091=AXIS2_PLACEMENT_3D('',#93308,#64641,#64642) ;
#53092=AXIS2_PLACEMENT_3D('',#93310,#64644,#64645) ;
#53093=AXIS2_PLACEMENT_3D('',#93313,#64648,#64649) ;
#53094=AXIS2_PLACEMENT_3D('',#93315,#64651,#64652) ;
#53095=AXIS2_PLACEMENT_3D('',#93317,#64654,#64655) ;
#53096=AXIS2_PLACEMENT_3D('',#93321,#64657,#64658) ;
#53097=AXIS2_PLACEMENT_3D('',#93323,#64660,#64661) ;
#53098=AXIS2_PLACEMENT_3D('',#93328,#64665,#64666) ;
#53099=AXIS2_PLACEMENT_3D('',#93330,#64668,#64669) ;
#53100=AXIS2_PLACEMENT_3D('',#93335,#64673,#64674) ;
#53101=AXIS2_PLACEMENT_3D('',#93337,#64676,#64677) ;
#53102=AXIS2_PLACEMENT_3D('',#93340,#64679,#64680) ;
#53103=AXIS2_PLACEMENT_3D('',#93341,#64681,#64682) ;
#53104=AXIS2_PLACEMENT_3D('',#93344,#64683,#64684) ;
#53105=AXIS2_PLACEMENT_3D('',#93348,#64686,#64687) ;
#53106=AXIS2_PLACEMENT_3D('',#93350,#64689,#64690) ;
#53107=AXIS2_PLACEMENT_3D('',#93356,#64694,#64695) ;
#53108=AXIS2_PLACEMENT_3D('',#93358,#64696,#64697) ;
#53109=AXIS2_PLACEMENT_3D('',#93360,#64698,#64699) ;
#53110=AXIS2_PLACEMENT_3D('',#93362,#64701,#64702) ;
#53111=AXIS2_PLACEMENT_3D('',#93365,#64703,#64704) ;
#53112=AXIS2_PLACEMENT_3D('',#93367,#64705,#64706) ;
#53113=AXIS2_PLACEMENT_3D('',#93369,#64707,#64708) ;
#53114=AXIS2_PLACEMENT_3D('',#93370,#64709,#64710) ;
#53115=AXIS2_PLACEMENT_3D('',#93371,#64711,#64712) ;
#53116=AXIS2_PLACEMENT_3D('',#93374,#64713,#64714) ;
#53117=AXIS2_PLACEMENT_3D('',#93376,#64715,#64716) ;
#53118=AXIS2_PLACEMENT_3D('',#93378,#64717,#64718) ;
#53119=AXIS2_PLACEMENT_3D('',#93379,#64719,#64720) ;
#53120=AXIS2_PLACEMENT_3D('',#93380,#64721,#64722) ;
#53121=AXIS2_PLACEMENT_3D('',#93383,#64725,#64726) ;
#53122=AXIS2_PLACEMENT_3D('',#93386,#64727,#64728) ;
#53123=AXIS2_PLACEMENT_3D('',#93390,#64730,#64731) ;
#53124=AXIS2_PLACEMENT_3D('',#93392,#64733,#64734) ;
#53125=AXIS2_PLACEMENT_3D('',#93395,#64735,#64736) ;
#53126=AXIS2_PLACEMENT_3D('',#93396,#64737,#64738) ;
#53127=AXIS2_PLACEMENT_3D('',#93397,#64739,#64740) ;
#53128=AXIS2_PLACEMENT_3D('',#93398,#64741,#64742) ;
#53129=AXIS2_PLACEMENT_3D('',#93401,#64745,#64746) ;
#53130=AXIS2_PLACEMENT_3D('',#93404,#64747,#64748) ;
#53131=AXIS2_PLACEMENT_3D('',#93407,#64751,#64752) ;
#53132=AXIS2_PLACEMENT_3D('',#93410,#64753,#64754) ;
#53133=AXIS2_PLACEMENT_3D('',#93413,#64757,#64758) ;
#53134=AXIS2_PLACEMENT_3D('',#93416,#64759,#64760) ;
#53135=AXIS2_PLACEMENT_3D('',#93419,#64763,#64764) ;
#53136=AXIS2_PLACEMENT_3D('',#93422,#64765,#64766) ;
#53137=AXIS2_PLACEMENT_3D('',#93423,#64767,#64768) ;
#53138=AXIS2_PLACEMENT_3D('',#93424,#64769,#64770) ;
#53139=AXIS2_PLACEMENT_3D('',#93425,#64771,#64772) ;
#53140=AXIS2_PLACEMENT_3D('',#93428,#64773,#64774) ;
#53141=AXIS2_PLACEMENT_3D('',#93431,#64777,#64778) ;
#53142=AXIS2_PLACEMENT_3D('',#93435,#64780,#64781) ;
#53143=AXIS2_PLACEMENT_3D('',#93437,#64783,#64784) ;
#53144=AXIS2_PLACEMENT_3D('',#93443,#64787,#64788) ;
#53145=AXIS2_PLACEMENT_3D('',#93449,#64791,#64792) ;
#53146=AXIS2_PLACEMENT_3D('',#93453,#64794,#64795) ;
#53147=AXIS2_PLACEMENT_3D('',#93457,#64797,#64798) ;
#53148=AXIS2_PLACEMENT_3D('',#93459,#64800,#64801) ;
#53149=AXIS2_PLACEMENT_3D('',#93462,#64803,#64804) ;
#53150=AXIS2_PLACEMENT_3D('',#93463,#64805,#64806) ;
#53151=AXIS2_PLACEMENT_3D('',#93475,#64814,#64815) ;
#53152=AXIS2_PLACEMENT_3D('',#93477,#64816,#64817) ;
#53153=AXIS2_PLACEMENT_3D('',#93480,#64819,#64820) ;
#53154=AXIS2_PLACEMENT_3D('',#93517,#64821,#64822) ;
#53155=AXIS2_PLACEMENT_3D('',#93518,#64823,#64824) ;
#53156=AXIS2_PLACEMENT_3D('',#93519,#64825,#64826) ;
#53157=AXIS2_PLACEMENT_3D('',#93521,#64828,#64829) ;
#53158=AXIS2_PLACEMENT_3D('',#93523,#64830,#64831) ;
#53159=AXIS2_PLACEMENT_3D('',#93524,#64832,#64833) ;
#53160=AXIS2_PLACEMENT_3D('',#93525,#64834,#64835) ;
#53161=AXIS2_PLACEMENT_3D('',#93527,#64836,#64837) ;
#53162=AXIS2_PLACEMENT_3D('',#93529,#64839,#64840) ;
#53163=AXIS2_PLACEMENT_3D('',#93531,#64841,#64842) ;
#53164=AXIS2_PLACEMENT_3D('',#93532,#64843,#64844) ;
#53165=AXIS2_PLACEMENT_3D('',#93533,#64845,#64846) ;
#53166=AXIS2_PLACEMENT_3D('',#93535,#64847,#64848) ;
#53167=AXIS2_PLACEMENT_3D('',#93537,#64850,#64851) ;
#53168=AXIS2_PLACEMENT_3D('',#93539,#64852,#64853) ;
#53169=AXIS2_PLACEMENT_3D('',#93540,#64854,#64855) ;
#53170=AXIS2_PLACEMENT_3D('',#93541,#64856,#64857) ;
#53171=AXIS2_PLACEMENT_3D('',#93543,#64858,#64859) ;
#53172=AXIS2_PLACEMENT_3D('',#93545,#64861,#64862) ;
#53173=AXIS2_PLACEMENT_3D('',#93547,#64863,#64864) ;
#53174=AXIS2_PLACEMENT_3D('',#93548,#64865,#64866) ;
#53175=AXIS2_PLACEMENT_3D('',#93549,#64867,#64868) ;
#53176=AXIS2_PLACEMENT_3D('',#93551,#64869,#64870) ;
#53177=AXIS2_PLACEMENT_3D('',#93553,#64872,#64873) ;
#53178=AXIS2_PLACEMENT_3D('',#93555,#64874,#64875) ;
#53179=AXIS2_PLACEMENT_3D('',#93556,#64876,#64877) ;
#53180=AXIS2_PLACEMENT_3D('',#93557,#64878,#64879) ;
#53181=AXIS2_PLACEMENT_3D('',#93559,#64880,#64881) ;
#53182=AXIS2_PLACEMENT_3D('',#93586,#64883,#64884) ;
#53183=AXIS2_PLACEMENT_3D('',#93587,#64885,#64886) ;
#53184=AXIS2_PLACEMENT_3D('',#93588,#64887,#64888) ;
#53185=AXIS2_PLACEMENT_3D('',#93590,#64889,#64890) ;
#53186=AXIS2_PLACEMENT_3D('',#93621,#64892,#64893) ;
#53187=AXIS2_PLACEMENT_3D('',#93622,#64894,#64895) ;
#53188=AXIS2_PLACEMENT_3D('',#93652,#64896,#64897) ;
#53189=AXIS2_PLACEMENT_3D('',#93653,#64898,#64899) ;
#53190=AXIS2_PLACEMENT_3D('',#93678,#64900,#64901) ;
#53191=AXIS2_PLACEMENT_3D('',#93683,#64902,#64903) ;
#53192=AXIS2_PLACEMENT_3D('',#93684,#64904,#64905) ;
#53193=AXIS2_PLACEMENT_3D('',#93685,#64906,#64907) ;
#53194=AXIS2_PLACEMENT_3D('',#93686,#64908,#64909) ;
#53195=AXIS2_PLACEMENT_3D('',#93687,#64910,#64911) ;
#53196=AXIS2_PLACEMENT_3D('',#93689,#64912,#64913) ;
#53197=AXIS2_PLACEMENT_3D('',#93690,#64914,#64915) ;
#53198=AXIS2_PLACEMENT_3D('',#93691,#64916,#64917) ;
#53199=AXIS2_PLACEMENT_3D('',#93693,#64918,#64919) ;
#53200=AXIS2_PLACEMENT_3D('',#93695,#64921,#64922) ;
#53201=AXIS2_PLACEMENT_3D('',#93697,#64923,#64924) ;
#53202=AXIS2_PLACEMENT_3D('',#93698,#64925,#64926) ;
#53203=AXIS2_PLACEMENT_3D('',#93699,#64927,#64928) ;
#53204=AXIS2_PLACEMENT_3D('',#93701,#64929,#64930) ;
#53205=AXIS2_PLACEMENT_3D('',#93702,#64931,#64932) ;
#53206=AXIS2_PLACEMENT_3D('',#93703,#64933,#64934) ;
#53207=AXIS2_PLACEMENT_3D('',#93704,#64935,#64936) ;
#53208=AXIS2_PLACEMENT_3D('',#93706,#64938,#64939) ;
#53209=AXIS2_PLACEMENT_3D('',#93707,#64940,#64941) ;
#53210=AXIS2_PLACEMENT_3D('',#93708,#64942,#64943) ;
#53211=AXIS2_PLACEMENT_3D('',#93709,#64944,#64945) ;
#53212=AXIS2_PLACEMENT_3D('',#93710,#64946,#64947) ;
#53213=AXIS2_PLACEMENT_3D('',#93711,#64948,#64949) ;
#53214=AXIS2_PLACEMENT_3D('',#93712,#64950,#64951) ;
#53215=AXIS2_PLACEMENT_3D('',#93716,#64954,#64955) ;
#53216=AXIS2_PLACEMENT_3D('',#93717,#64956,#64957) ;
#53217=AXIS2_PLACEMENT_3D('',#93718,#64958,#64959) ;
#53218=AXIS2_PLACEMENT_3D('',#93720,#64961,#64962) ;
#53219=AXIS2_PLACEMENT_3D('',#93722,#64964,#64965) ;
#53220=AXIS2_PLACEMENT_3D('',#93724,#64967,#64968) ;
#53221=AXIS2_PLACEMENT_3D('',#93726,#64970,#64971) ;
#53222=AXIS2_PLACEMENT_3D('',#93727,#64972,#64973) ;
#53223=AXIS2_PLACEMENT_3D('',#93729,#64974,#64975) ;
#53224=AXIS2_PLACEMENT_3D('',#93731,#64977,#64978) ;
#53225=AXIS2_PLACEMENT_3D('',#93732,#64979,#64980) ;
#53226=AXIS2_PLACEMENT_3D('',#93733,#64981,#64982) ;
#53227=AXIS2_PLACEMENT_3D('',#93736,#64984,#64985) ;
#53228=AXIS2_PLACEMENT_3D('',#93737,#64986,#64987) ;
#53229=AXIS2_PLACEMENT_3D('',#93739,#64988,#64989) ;
#53230=AXIS2_PLACEMENT_3D('',#93740,#64990,#64991) ;
#53231=AXIS2_PLACEMENT_3D('',#93741,#64992,#64993) ;
#53232=AXIS2_PLACEMENT_3D('',#93743,#64995,#64996) ;
#53233=AXIS2_PLACEMENT_3D('',#93745,#64997,#64998) ;
#53234=AXIS2_PLACEMENT_3D('',#93746,#64999,#65000) ;
#53235=AXIS2_PLACEMENT_3D('',#93747,#65001,#65002) ;
#53236=AXIS2_PLACEMENT_3D('',#93749,#65003,#65004) ;
#53237=AXIS2_PLACEMENT_3D('',#93751,#65006,#65007) ;
#53238=AXIS2_PLACEMENT_3D('',#93752,#65008,#65009) ;
#53239=AXIS2_PLACEMENT_3D('',#93753,#65010,#65011) ;
#53240=AXIS2_PLACEMENT_3D('',#93754,#65012,#65013) ;
#53241=AXIS2_PLACEMENT_3D('',#93755,#65014,#65015) ;
#53242=AXIS2_PLACEMENT_3D('',#93756,#65016,#65017) ;
#53243=AXIS2_PLACEMENT_3D('',#93757,#65018,#65019) ;
#53244=AXIS2_PLACEMENT_3D('',#93758,#65020,#65021) ;
#53245=AXIS2_PLACEMENT_3D('',#93760,#65022,#65023) ;
#53246=AXIS2_PLACEMENT_3D('',#93762,#65025,#65026) ;
#53247=AXIS2_PLACEMENT_3D('',#93764,#65027,#65028) ;
#53248=AXIS2_PLACEMENT_3D('',#93765,#65029,#65030) ;
#53249=AXIS2_PLACEMENT_3D('',#93766,#65031,#65032) ;
#53250=AXIS2_PLACEMENT_3D('',#93769,#65034,#65035) ;
#53251=AXIS2_PLACEMENT_3D('',#93770,#65036,#65037) ;
#53252=AXIS2_PLACEMENT_3D('',#93773,#65038,#65039) ;
#53253=AXIS2_PLACEMENT_3D('',#93777,#65041,#65042) ;
#53254=AXIS2_PLACEMENT_3D('',#93779,#65044,#65045) ;
#53255=AXIS2_PLACEMENT_3D('',#93781,#65046,#65047) ;
#53256=AXIS2_PLACEMENT_3D('',#93782,#65048,#65049) ;
#53257=AXIS2_PLACEMENT_3D('',#93783,#65050,#65051) ;
#53258=AXIS2_PLACEMENT_3D('',#93784,#65052,#65053) ;
#53259=AXIS2_PLACEMENT_3D('',#93786,#65054,#65055) ;
#53260=AXIS2_PLACEMENT_3D('',#93788,#65057,#65058) ;
#53261=AXIS2_PLACEMENT_3D('',#93790,#65059,#65060) ;
#53262=AXIS2_PLACEMENT_3D('',#93791,#65061,#65062) ;
#53263=AXIS2_PLACEMENT_3D('',#93792,#65063,#65064) ;
#53264=AXIS2_PLACEMENT_3D('',#93794,#65065,#65066) ;
#53265=AXIS2_PLACEMENT_3D('',#93796,#65068,#65069) ;
#53266=AXIS2_PLACEMENT_3D('',#93798,#65070,#65071) ;
#53267=AXIS2_PLACEMENT_3D('',#93799,#65072,#65073) ;
#53268=AXIS2_PLACEMENT_3D('',#93800,#65074,#65075) ;
#53269=AXIS2_PLACEMENT_3D('',#93802,#65077,#65078) ;
#53270=AXIS2_PLACEMENT_3D('',#93803,#65079,#65080) ;
#53271=AXIS2_PLACEMENT_3D('',#93805,#65082,#65083) ;
#53272=AXIS2_PLACEMENT_3D('',#93806,#65084,#65085) ;
#53273=AXIS2_PLACEMENT_3D('',#93810,#65087,#65088) ;
#53274=AXIS2_PLACEMENT_3D('',#93814,#65090,#65091) ;
#53275=AXIS2_PLACEMENT_3D('',#93817,#65093,#65094) ;
#53276=AXIS2_PLACEMENT_3D('',#93903,#65105,#65106) ;
#53277=AXIS2_PLACEMENT_3D('',#93906,#65108,#65109) ;
#53278=AXIS2_PLACEMENT_3D('',#93907,#65110,#65111) ;
#53279=AXIS2_PLACEMENT_3D('',#93912,#65114,#65115) ;
#53280=AXIS2_PLACEMENT_3D('',#93913,#65116,#65117) ;
#53281=AXIS2_PLACEMENT_3D('',#93919,#65121,#65122) ;
#53282=AXIS2_PLACEMENT_3D('',#93921,#65123,#65124) ;
#53283=AXIS2_PLACEMENT_3D('',#93922,#65125,#65126) ;
#53284=AXIS2_PLACEMENT_3D('',#93925,#65128,#65129) ;
#53285=AXIS2_PLACEMENT_3D('',#93926,#65130,#65131) ;
#53286=AXIS2_PLACEMENT_3D('',#93934,#65136,#65137) ;
#53287=AXIS2_PLACEMENT_3D('',#93969,#65140,#65141) ;
#53288=AXIS2_PLACEMENT_3D('',#93971,#65142,#65143) ;
#53289=AXIS2_PLACEMENT_3D('',#93973,#65144,#65145) ;
#53290=AXIS2_PLACEMENT_3D('',#93974,#65146,#65147) ;
#53291=AXIS2_PLACEMENT_3D('',#94007,#65148,#65149) ;
#53292=AXIS2_PLACEMENT_3D('',#94009,#65150,#65151) ;
#53293=AXIS2_PLACEMENT_3D('',#94011,#65152,#65153) ;
#53294=AXIS2_PLACEMENT_3D('',#94012,#65154,#65155) ;
#53295=AXIS2_PLACEMENT_3D('',#94013,#65156,#65157) ;
#53296=AXIS2_PLACEMENT_3D('',#94017,#65159,#65160) ;
#53297=AXIS2_PLACEMENT_3D('',#94046,#65162,#65163) ;
#53298=AXIS2_PLACEMENT_3D('',#94080,#65164,#65165) ;
#53299=AXIS2_PLACEMENT_3D('',#94083,#65166,#65167) ;
#53300=AXIS2_PLACEMENT_3D('',#94084,#65168,#65169) ;
#53301=AXIS2_PLACEMENT_3D('',#94085,#65170,#65171) ;
#53302=AXIS2_PLACEMENT_3D('',#94086,#65172,#65173) ;
#53303=AXIS2_PLACEMENT_3D('',#94089,#65176,#65177) ;
#53304=AXIS2_PLACEMENT_3D('',#94092,#65178,#65179) ;
#53305=AXIS2_PLACEMENT_3D('',#94095,#65182,#65183) ;
#53306=AXIS2_PLACEMENT_3D('',#94098,#65186,#65187) ;
#53307=AXIS2_PLACEMENT_3D('',#94101,#65188,#65189) ;
#53308=AXIS2_PLACEMENT_3D('',#94104,#65192,#65193) ;
#53309=AXIS2_PLACEMENT_3D('',#94106,#65194,#65195) ;
#53310=AXIS2_PLACEMENT_3D('',#94130,#65198,#65199) ;
#53311=AXIS2_PLACEMENT_3D('',#94131,#65200,#65201) ;
#53312=AXIS2_PLACEMENT_3D('',#94156,#65202,#65203) ;
#53313=AXIS2_PLACEMENT_3D('',#94160,#65205,#65206) ;
#53314=AXIS2_PLACEMENT_3D('',#94162,#65208,#65209) ;
#53315=AXIS2_PLACEMENT_3D('',#94164,#65211,#65212) ;
#53316=AXIS2_PLACEMENT_3D('',#94166,#65214,#65215) ;
#53317=AXIS2_PLACEMENT_3D('',#94170,#65217,#65218) ;
#53318=AXIS2_PLACEMENT_3D('',#94172,#65220,#65221) ;
#53319=AXIS2_PLACEMENT_3D('',#94174,#65222,#65223) ;
#53320=AXIS2_PLACEMENT_3D('',#94176,#65224,#65225) ;
#53321=AXIS2_PLACEMENT_3D('',#94192,#65227,#65228) ;
#53322=AXIS2_PLACEMENT_3D('',#94196,#65230,#65231) ;
#53323=AXIS2_PLACEMENT_3D('',#94197,#65232,#65233) ;
#53324=AXIS2_PLACEMENT_3D('',#94198,#65234,#65235) ;
#53325=AXIS2_PLACEMENT_3D('',#94202,#65237,#65238) ;
#53326=AXIS2_PLACEMENT_3D('',#94205,#65240,#65241) ;
#53327=AXIS2_PLACEMENT_3D('',#94206,#65242,#65243) ;
#53328=AXIS2_PLACEMENT_3D('',#94215,#65249,#65250) ;
#53329=AXIS2_PLACEMENT_3D('',#94219,#65253,#65254) ;
#53330=AXIS2_PLACEMENT_3D('',#94247,#65257,#65258) ;
#53331=AXIS2_PLACEMENT_3D('',#94248,#65259,#65260) ;
#53332=AXIS2_PLACEMENT_3D('',#94249,#65261,#65262) ;
#53333=AXIS2_PLACEMENT_3D('',#94250,#65263,#65264) ;
#53334=AXIS2_PLACEMENT_3D('',#94279,#65265,#65266) ;
#53335=AXIS2_PLACEMENT_3D('',#94316,#65267,#65268) ;
#53336=AXIS2_PLACEMENT_3D('',#94374,#65269,#65270) ;
#53337=AXIS2_PLACEMENT_3D('',#94375,#65271,#65272) ;
#53338=AXIS2_PLACEMENT_3D('',#94429,#65273,#65274) ;
#53339=AXIS2_PLACEMENT_3D('',#94431,#65276,#65277) ;
#53340=AXIS2_PLACEMENT_3D('',#94447,#65280,#65281) ;
#53341=AXIS2_PLACEMENT_3D('',#94477,#65283,#65284) ;
#53342=AXIS2_PLACEMENT_3D('',#94479,#65285,#65286) ;
#53343=AXIS2_PLACEMENT_3D('',#94480,#65287,#65288) ;
#53344=AXIS2_PLACEMENT_3D('',#94481,#65289,#65290) ;
#53345=AXIS2_PLACEMENT_3D('',#94484,#65291,#65292) ;
#53346=AXIS2_PLACEMENT_3D('',#94516,#65295,#65296) ;
#53347=AXIS2_PLACEMENT_3D('',#94517,#65297,#65298) ;
#53348=AXIS2_PLACEMENT_3D('',#94518,#65299,#65300) ;
#53349=AXIS2_PLACEMENT_3D('',#94540,#65301,#65302) ;
#53350=AXIS2_PLACEMENT_3D('',#94559,#65303,#65304) ;
#53351=AXIS2_PLACEMENT_3D('',#94563,#65306,#65307) ;
#53352=AXIS2_PLACEMENT_3D('',#94570,#65311,#65312) ;
#53353=AXIS2_PLACEMENT_3D('',#94578,#65316,#65317) ;
#53354=AXIS2_PLACEMENT_3D('',#94586,#65321,#65322) ;
#53355=AXIS2_PLACEMENT_3D('',#94602,#65330,#65331) ;
#53356=AXIS2_PLACEMENT_3D('',#94616,#65338,#65339) ;
#53357=AXIS2_PLACEMENT_3D('',#94626,#65345,#65346) ;
#53358=AXIS2_PLACEMENT_3D('',#94627,#65347,#65348) ;
#53359=AXIS2_PLACEMENT_3D('',#94629,#65350,#65351) ;
#53360=AXIS2_PLACEMENT_3D('',#94631,#65352,#65353) ;
#53361=AXIS2_PLACEMENT_3D('',#94633,#65355,#65356) ;
#53362=AXIS2_PLACEMENT_3D('',#94634,#65357,#65358) ;
#53363=AXIS2_PLACEMENT_3D('',#94668,#65359,#65360) ;
#53364=AXIS2_PLACEMENT_3D('',#94669,#65361,#65362) ;
#53365=AXIS2_PLACEMENT_3D('',#94670,#65363,#65364) ;
#53366=AXIS2_PLACEMENT_3D('',#94683,#65366,#65367) ;
#53367=AXIS2_PLACEMENT_3D('',#94685,#65368,#65369) ;
#53368=AXIS2_PLACEMENT_3D('',#94687,#65371,#65372) ;
#53369=AXIS2_PLACEMENT_3D('',#94735,#65374,#65375) ;
#53370=AXIS2_PLACEMENT_3D('',#94777,#65376,#65377) ;
#53371=AXIS2_PLACEMENT_3D('',#94779,#65379,#65380) ;
#53372=AXIS2_PLACEMENT_3D('',#94781,#65382,#65383) ;
#53373=AXIS2_PLACEMENT_3D('',#94784,#65385,#65386) ;
#53374=AXIS2_PLACEMENT_3D('',#94785,#65387,#65388) ;
#53375=AXIS2_PLACEMENT_3D('',#94789,#65391,#65392) ;
#53376=AXIS2_PLACEMENT_3D('',#94792,#65395,#65396) ;
#53377=AXIS2_PLACEMENT_3D('',#94799,#65398,#65399) ;
#53378=AXIS2_PLACEMENT_3D('',#94807,#65401,#65402) ;
#53379=AXIS2_PLACEMENT_3D('',#94823,#65404,#65405) ;
#53380=AXIS2_PLACEMENT_3D('',#94824,#65406,#65407) ;
#53381=AXIS2_PLACEMENT_3D('',#94825,#65408,#65409) ;
#53382=AXIS2_PLACEMENT_3D('',#94827,#65411,#65412) ;
#53383=AXIS2_PLACEMENT_3D('',#94829,#65414,#65415) ;
#53384=AXIS2_PLACEMENT_3D('',#94830,#65416,#65417) ;
#53385=AXIS2_PLACEMENT_3D('',#94840,#65423,#65424) ;
#53386=AXIS2_PLACEMENT_3D('',#94842,#65425,#65426) ;
#53387=AXIS2_PLACEMENT_3D('',#94844,#65428,#65429) ;
#53388=AXIS2_PLACEMENT_3D('',#94887,#65433,#65434) ;
#53389=AXIS2_PLACEMENT_3D('',#94889,#65435,#65436) ;
#53390=AXIS2_PLACEMENT_3D('',#94892,#65438,#65439) ;
#53391=AXIS2_PLACEMENT_3D('',#94893,#65440,#65441) ;
#53392=AXIS2_PLACEMENT_3D('',#94896,#65443,#65444) ;
#53393=AXIS2_PLACEMENT_3D('',#94897,#65445,#65446) ;
#53394=AXIS2_PLACEMENT_3D('',#94901,#65449,#65450) ;
#53395=AXIS2_PLACEMENT_3D('',#94905,#65453,#65454) ;
#53396=AXIS2_PLACEMENT_3D('',#94907,#65456,#65457) ;
#53397=AXIS2_PLACEMENT_3D('',#94913,#65460,#65461) ;
#53398=AXIS2_PLACEMENT_3D('',#94916,#65463,#65464) ;
#53399=AXIS2_PLACEMENT_3D('',#94920,#65467,#65468) ;
#53400=AXIS2_PLACEMENT_3D('',#94921,#65469,#65470) ;
#53401=AXIS2_PLACEMENT_3D('',#94922,#65471,#65472) ;
#53402=AXIS2_PLACEMENT_3D('',#94923,#65473,#65474) ;
#53403=AXIS2_PLACEMENT_3D('',#94924,#65475,#65476) ;
#53404=AXIS2_PLACEMENT_3D('',#94925,#65477,#65478) ;
#53405=AXIS2_PLACEMENT_3D('',#94926,#65479,#65480) ;
#53406=AXIS2_PLACEMENT_3D('',#94927,#65481,#65482) ;
#53407=AXIS2_PLACEMENT_3D('',#94928,#65483,#65484) ;
#53408=AXIS2_PLACEMENT_3D('',#94930,#65486,#65487) ;
#53409=AXIS2_PLACEMENT_3D('',#94936,#65491,#65492) ;
#53410=AXIS2_PLACEMENT_3D('',#94942,#65496,#65497) ;
#53411=AXIS2_PLACEMENT_3D('',#94945,#65500,#65501) ;
#53412=AXIS2_PLACEMENT_3D('',#94947,#65503,#65504) ;
#53413=AXIS2_PLACEMENT_3D('',#94949,#65506,#65507) ;
#53414=AXIS2_PLACEMENT_3D('',#94951,#65509,#65510) ;
#53415=AXIS2_PLACEMENT_3D('',#94952,#65511,#65512) ;
#53416=AXIS2_PLACEMENT_3D('',#94973,#65515,#65516) ;
#53417=AXIS2_PLACEMENT_3D('',#95156,#65517,#65518) ;
#53418=AXIS2_PLACEMENT_3D('',#95268,#65521,#65522) ;
#53419=AXIS2_PLACEMENT_3D('',#95273,#65525,#65526) ;
#53420=AXIS2_PLACEMENT_3D('',#95274,#65527,#65528) ;
#53421=AXIS2_PLACEMENT_3D('',#95279,#65531,#65532) ;
#53422=AXIS2_PLACEMENT_3D('',#95280,#65533,#65534) ;
#53423=AXIS2_PLACEMENT_3D('',#95283,#65537,#65538) ;
#53424=AXIS2_PLACEMENT_3D('',#95289,#65542,#65543) ;
#53425=AXIS2_PLACEMENT_3D('',#95293,#65546,#65547) ;
#53426=AXIS2_PLACEMENT_3D('',#95297,#65550,#65551) ;
#53427=AXIS2_PLACEMENT_3D('',#95301,#65554,#65555) ;
#53428=AXIS2_PLACEMENT_3D('',#95536,#65556,#65557) ;
#53429=AXIS2_PLACEMENT_3D('',#95540,#65559,#65560) ;
#53430=AXIS2_PLACEMENT_3D('',#95542,#65562,#65563) ;
#53431=AXIS2_PLACEMENT_3D('',#95546,#65565,#65566) ;
#53432=AXIS2_PLACEMENT_3D('',#95548,#65568,#65569) ;
#53433=AXIS2_PLACEMENT_3D('',#95553,#65572,#65573) ;
#53434=AXIS2_PLACEMENT_3D('',#95554,#65574,#65575) ;
#53435=AXIS2_PLACEMENT_3D('',#95782,#65578,#65579) ;
#53436=AXIS2_PLACEMENT_3D('',#95785,#65582,#65583) ;
#53437=AXIS2_PLACEMENT_3D('',#95964,#65588,#65589) ;
#53438=AXIS2_PLACEMENT_3D('',#96075,#65593,#65594) ;
#53439=AXIS2_PLACEMENT_3D('',#96076,#65595,#65596) ;
#53440=AXIS2_PLACEMENT_3D('',#96081,#65598,#65599) ;
#53441=AXIS2_PLACEMENT_3D('',#96084,#65601,#65602) ;
#53442=AXIS2_PLACEMENT_3D('',#96085,#65603,#65604) ;
#53443=AXIS2_PLACEMENT_3D('',#96089,#65606,#65607) ;
#53444=AXIS2_PLACEMENT_3D('',#96091,#65609,#65610) ;
#53445=AXIS2_PLACEMENT_3D('',#96095,#65612,#65613) ;
#53446=AXIS2_PLACEMENT_3D('',#96097,#65615,#65616) ;
#53447=AXIS2_PLACEMENT_3D('',#96102,#65619,#65620) ;
#53448=AXIS2_PLACEMENT_3D('',#96103,#65621,#65622) ;
#53449=AXIS2_PLACEMENT_3D('',#96108,#65625,#65626) ;
#53450=AXIS2_PLACEMENT_3D('',#96109,#65627,#65628) ;
#53451=AXIS2_PLACEMENT_3D('',#96114,#65631,#65632) ;
#53452=AXIS2_PLACEMENT_3D('',#96115,#65633,#65634) ;
#53453=AXIS2_PLACEMENT_3D('',#96118,#65637,#65638) ;
#53454=AXIS2_PLACEMENT_3D('',#96124,#65642,#65643) ;
#53455=AXIS2_PLACEMENT_3D('',#96128,#65646,#65647) ;
#53456=AXIS2_PLACEMENT_3D('',#96132,#65650,#65651) ;
#53457=AXIS2_PLACEMENT_3D('',#96136,#65654,#65655) ;
#53458=AXIS2_PLACEMENT_3D('',#96137,#65656,#65657) ;
#53459=AXIS2_PLACEMENT_3D('',#96142,#65659,#65660) ;
#53460=AXIS2_PLACEMENT_3D('',#96145,#65662,#65663) ;
#53461=AXIS2_PLACEMENT_3D('',#96146,#65664,#65665) ;
#53462=AXIS2_PLACEMENT_3D('',#96151,#65668,#65669) ;
#53463=AXIS2_PLACEMENT_3D('',#96152,#65670,#65671) ;
#53464=AXIS2_PLACEMENT_3D('',#96157,#65674,#65675) ;
#53465=AXIS2_PLACEMENT_3D('',#96158,#65676,#65677) ;
#53466=AXIS2_PLACEMENT_3D('',#96161,#65680,#65681) ;
#53467=AXIS2_PLACEMENT_3D('',#96167,#65685,#65686) ;
#53468=AXIS2_PLACEMENT_3D('',#96171,#65689,#65690) ;
#53469=AXIS2_PLACEMENT_3D('',#96172,#65691,#65692) ;
#53470=AXIS2_PLACEMENT_3D('',#96177,#65694,#65695) ;
#53471=AXIS2_PLACEMENT_3D('',#96180,#65697,#65698) ;
#53472=AXIS2_PLACEMENT_3D('',#96181,#65699,#65700) ;
#53473=AXIS2_PLACEMENT_3D('',#96185,#65702,#65703) ;
#53474=AXIS2_PLACEMENT_3D('',#96187,#65705,#65706) ;
#53475=AXIS2_PLACEMENT_3D('',#96191,#65708,#65709) ;
#53476=AXIS2_PLACEMENT_3D('',#96193,#65711,#65712) ;
#53477=AXIS2_PLACEMENT_3D('',#96198,#65715,#65716) ;
#53478=AXIS2_PLACEMENT_3D('',#96199,#65717,#65718) ;
#53479=AXIS2_PLACEMENT_3D('',#96204,#65721,#65722) ;
#53480=AXIS2_PLACEMENT_3D('',#96205,#65723,#65724) ;
#53481=AXIS2_PLACEMENT_3D('',#96210,#65727,#65728) ;
#53482=AXIS2_PLACEMENT_3D('',#96211,#65729,#65730) ;
#53483=AXIS2_PLACEMENT_3D('',#96214,#65733,#65734) ;
#53484=AXIS2_PLACEMENT_3D('',#96220,#65738,#65739) ;
#53485=AXIS2_PLACEMENT_3D('',#96224,#65742,#65743) ;
#53486=AXIS2_PLACEMENT_3D('',#96228,#65746,#65747) ;
#53487=AXIS2_PLACEMENT_3D('',#96232,#65750,#65751) ;
#53488=AXIS2_PLACEMENT_3D('',#96233,#65752,#65753) ;
#53489=AXIS2_PLACEMENT_3D('',#96238,#65755,#65756) ;
#53490=AXIS2_PLACEMENT_3D('',#96241,#65758,#65759) ;
#53491=AXIS2_PLACEMENT_3D('',#96242,#65760,#65761) ;
#53492=AXIS2_PLACEMENT_3D('',#96247,#65764,#65765) ;
#53493=AXIS2_PLACEMENT_3D('',#96248,#65766,#65767) ;
#53494=AXIS2_PLACEMENT_3D('',#96253,#65770,#65771) ;
#53495=AXIS2_PLACEMENT_3D('',#96254,#65772,#65773) ;
#53496=AXIS2_PLACEMENT_3D('',#96257,#65776,#65777) ;
#53497=AXIS2_PLACEMENT_3D('',#96263,#65781,#65782) ;
#53498=AXIS2_PLACEMENT_3D('',#96267,#65785,#65786) ;
#53499=AXIS2_PLACEMENT_3D('',#96268,#65787,#65788) ;
#53500=AXIS2_PLACEMENT_3D('',#96273,#65790,#65791) ;
#53501=AXIS2_PLACEMENT_3D('',#96276,#65793,#65794) ;
#53502=AXIS2_PLACEMENT_3D('',#96277,#65795,#65796) ;
#53503=AXIS2_PLACEMENT_3D('',#96281,#65798,#65799) ;
#53504=AXIS2_PLACEMENT_3D('',#96283,#65801,#65802) ;
#53505=AXIS2_PLACEMENT_3D('',#96287,#65804,#65805) ;
#53506=AXIS2_PLACEMENT_3D('',#96289,#65807,#65808) ;
#53507=AXIS2_PLACEMENT_3D('',#96292,#65809,#65810) ;
#53508=AXIS2_PLACEMENT_3D('',#96293,#65811,#65812) ;
#53509=AXIS2_PLACEMENT_3D('',#96294,#65813,#65814) ;
#53510=AXIS2_PLACEMENT_3D('',#96295,#65815,#65816) ;
#53511=AXIS2_PLACEMENT_3D('',#96300,#65819,#65820) ;
#53512=AXIS2_PLACEMENT_3D('',#96301,#65821,#65822) ;
#53513=AXIS2_PLACEMENT_3D('',#96306,#65825,#65826) ;
#53514=AXIS2_PLACEMENT_3D('',#96307,#65827,#65828) ;
#53515=AXIS2_PLACEMENT_3D('',#96311,#65830,#65831) ;
#53516=AXIS2_PLACEMENT_3D('',#96313,#65833,#65834) ;
#53517=AXIS2_PLACEMENT_3D('',#96316,#65835,#65836) ;
#53518=AXIS2_PLACEMENT_3D('',#96317,#65837,#65838) ;
#53519=AXIS2_PLACEMENT_3D('',#96318,#65839,#65840) ;
#53520=AXIS2_PLACEMENT_3D('',#96319,#65841,#65842) ;
#53521=AXIS2_PLACEMENT_3D('',#96324,#65845,#65846) ;
#53522=AXIS2_PLACEMENT_3D('',#96325,#65847,#65848) ;
#53523=AXIS2_PLACEMENT_3D('',#96330,#65851,#65852) ;
#53524=AXIS2_PLACEMENT_3D('',#96331,#65853,#65854) ;
#53525=AXIS2_PLACEMENT_3D('',#96334,#65857,#65858) ;
#53526=AXIS2_PLACEMENT_3D('',#96340,#65862,#65863) ;
#53527=AXIS2_PLACEMENT_3D('',#96343,#65865,#65866) ;
#53528=AXIS2_PLACEMENT_3D('',#96344,#65867,#65868) ;
#53529=AXIS2_PLACEMENT_3D('',#96348,#65871,#65872) ;
#53530=AXIS2_PLACEMENT_3D('',#96352,#65875,#65876) ;
#53531=AXIS2_PLACEMENT_3D('',#96356,#65879,#65880) ;
#53532=AXIS2_PLACEMENT_3D('',#96360,#65883,#65884) ;
#53533=AXIS2_PLACEMENT_3D('',#96361,#65885,#65886) ;
#53534=AXIS2_PLACEMENT_3D('',#96366,#65888,#65889) ;
#53535=AXIS2_PLACEMENT_3D('',#96369,#65891,#65892) ;
#53536=AXIS2_PLACEMENT_3D('',#96370,#65893,#65894) ;
#53537=AXIS2_PLACEMENT_3D('',#96374,#65896,#65897) ;
#53538=AXIS2_PLACEMENT_3D('',#96376,#65899,#65900) ;
#53539=AXIS2_PLACEMENT_3D('',#96379,#65901,#65902) ;
#53540=AXIS2_PLACEMENT_3D('',#96380,#65903,#65904) ;
#53541=AXIS2_PLACEMENT_3D('',#96381,#65905,#65906) ;
#53542=AXIS2_PLACEMENT_3D('',#96382,#65907,#65908) ;
#53543=AXIS2_PLACEMENT_3D('',#96387,#65911,#65912) ;
#53544=AXIS2_PLACEMENT_3D('',#96388,#65913,#65914) ;
#53545=AXIS2_PLACEMENT_3D('',#96392,#65916,#65917) ;
#53546=AXIS2_PLACEMENT_3D('',#96394,#65919,#65920) ;
#53547=AXIS2_PLACEMENT_3D('',#96398,#65922,#65923) ;
#53548=AXIS2_PLACEMENT_3D('',#96400,#65925,#65926) ;
#53549=AXIS2_PLACEMENT_3D('',#96403,#65927,#65928) ;
#53550=AXIS2_PLACEMENT_3D('',#96404,#65929,#65930) ;
#53551=AXIS2_PLACEMENT_3D('',#96405,#65931,#65932) ;
#53552=AXIS2_PLACEMENT_3D('',#96406,#65933,#65934) ;
#53553=AXIS2_PLACEMENT_3D('',#96411,#65937,#65938) ;
#53554=AXIS2_PLACEMENT_3D('',#96412,#65939,#65940) ;
#53555=AXIS2_PLACEMENT_3D('',#96417,#65943,#65944) ;
#53556=AXIS2_PLACEMENT_3D('',#96418,#65945,#65946) ;
#53557=AXIS2_PLACEMENT_3D('',#96423,#65949,#65950) ;
#53558=AXIS2_PLACEMENT_3D('',#96424,#65951,#65952) ;
#53559=AXIS2_PLACEMENT_3D('',#96427,#65955,#65956) ;
#53560=AXIS2_PLACEMENT_3D('',#96431,#65958,#65959) ;
#53561=AXIS2_PLACEMENT_3D('',#96433,#65961,#65962) ;
#53562=AXIS2_PLACEMENT_3D('',#96437,#65965,#65966) ;
#53563=AXIS2_PLACEMENT_3D('',#96441,#65969,#65970) ;
#53564=AXIS2_PLACEMENT_3D('',#96445,#65973,#65974) ;
#53565=AXIS2_PLACEMENT_3D('',#96449,#65977,#65978) ;
#53566=AXIS2_PLACEMENT_3D('',#96453,#65981,#65982) ;
#53567=AXIS2_PLACEMENT_3D('',#96757,#65983,#65984) ;
#53568=AXIS2_PLACEMENT_3D('',#96774,#65986,#65987) ;
#53569=AXIS2_PLACEMENT_3D('',#96775,#65988,#65989) ;
#53570=AXIS2_PLACEMENT_3D('',#96776,#65990,#65991) ;
#53571=AXIS2_PLACEMENT_3D('',#96777,#65992,#65993) ;
#53572=AXIS2_PLACEMENT_3D('',#96778,#65994,#65995) ;
#53573=AXIS2_PLACEMENT_3D('',#96779,#65996,#65997) ;
#53574=AXIS2_PLACEMENT_3D('',#96780,#65998,#65999) ;
#53575=AXIS2_PLACEMENT_3D('',#96902,#66001,#66002) ;
#53576=AXIS2_PLACEMENT_3D('',#97048,#66004,#66005) ;
#53577=AXIS2_PLACEMENT_3D('',#97049,#66006,#66007) ;
#53578=AXIS2_PLACEMENT_3D('',#97050,#66008,#66009) ;
#53579=AXIS2_PLACEMENT_3D('',#97052,#66010,#66011) ;
#53580=AXIS2_PLACEMENT_3D('',#97055,#66013,#66014) ;
#53581=AXIS2_PLACEMENT_3D('',#97056,#66015,#66016) ;
#53582=AXIS2_PLACEMENT_3D('',#97072,#66018,#66019) ;
#53583=AXIS2_PLACEMENT_3D('',#97187,#66021,#66022) ;
#53584=AXIS2_PLACEMENT_3D('',#97188,#66023,#66024) ;
#53585=AXIS2_PLACEMENT_3D('',#97190,#66026,#66027) ;
#53586=AXIS2_PLACEMENT_3D('',#97192,#66029,#66030) ;
#53587=AXIS2_PLACEMENT_3D('',#97196,#66032,#66033) ;
#53588=AXIS2_PLACEMENT_3D('',#97199,#66035,#66036) ;
#53589=AXIS2_PLACEMENT_3D('',#97200,#66037,#66038) ;
#53590=AXIS2_PLACEMENT_3D('',#97204,#66040,#66041) ;
#53591=AXIS2_PLACEMENT_3D('',#97206,#66043,#66044) ;
#53592=AXIS2_PLACEMENT_3D('',#97209,#66046,#66047) ;
#53593=AXIS2_PLACEMENT_3D('',#97210,#66048,#66049) ;
#53594=AXIS2_PLACEMENT_3D('',#97213,#66051,#66052) ;
#53595=AXIS2_PLACEMENT_3D('',#97214,#66053,#66054) ;
#53596=AXIS2_PLACEMENT_3D('',#97217,#66056,#66057) ;
#53597=AXIS2_PLACEMENT_3D('',#97218,#66058,#66059) ;
#53598=AXIS2_PLACEMENT_3D('',#97221,#66061,#66062) ;
#53599=AXIS2_PLACEMENT_3D('',#97222,#66063,#66064) ;
#53600=AXIS2_PLACEMENT_3D('',#97225,#66067,#66068) ;
#53601=AXIS2_PLACEMENT_3D('',#97227,#66070,#66071) ;
#53602=AXIS2_PLACEMENT_3D('',#97229,#66073,#66074) ;
#53603=AXIS2_PLACEMENT_3D('',#97230,#66075,#66076) ;
#53604=AXIS2_PLACEMENT_3D('',#97235,#66078,#66079) ;
#53605=AXIS2_PLACEMENT_3D('',#97238,#66081,#66082) ;
#53606=AXIS2_PLACEMENT_3D('',#97240,#66083,#66084) ;
#53607=AXIS2_PLACEMENT_3D('',#97244,#66086,#66087) ;
#53608=AXIS2_PLACEMENT_3D('',#97298,#66090,#66091) ;
#53609=AXIS2_PLACEMENT_3D('',#97321,#66103,#66104) ;
#53610=AXIS2_PLACEMENT_3D('',#97322,#66105,#66106) ;
#53611=AXIS2_PLACEMENT_3D('',#97323,#66107,#66108) ;
#53612=AXIS2_PLACEMENT_3D('',#97324,#66109,#66110) ;
#53613=AXIS2_PLACEMENT_3D('',#97325,#66111,#66112) ;
#53614=AXIS2_PLACEMENT_3D('',#97326,#66113,#66114) ;
#53615=AXIS2_PLACEMENT_3D('',#97329,#66116,#66117) ;
#53616=AXIS2_PLACEMENT_3D('',#97330,#66118,#66119) ;
#53617=AXIS2_PLACEMENT_3D('',#97332,#66121,#66122) ;
#53618=AXIS2_PLACEMENT_3D('',#97334,#66124,#66125) ;
#53619=AXIS2_PLACEMENT_3D('',#97336,#66126,#66127) ;
#53620=AXIS2_PLACEMENT_3D('',#97339,#66129,#66130) ;
#53621=AXIS2_PLACEMENT_3D('',#97340,#66131,#66132) ;
#53622=AXIS2_PLACEMENT_3D('',#97341,#66133,#66134) ;
#53623=AXIS2_PLACEMENT_3D('',#97343,#66136,#66137) ;
#53624=AXIS2_PLACEMENT_3D('',#97344,#66138,#66139) ;
#53625=AXIS2_PLACEMENT_3D('',#97345,#66140,#66141) ;
#53626=AXIS2_PLACEMENT_3D('',#97346,#66142,#66143) ;
#53627=AXIS2_PLACEMENT_3D('',#97347,#66144,#66145) ;
#53628=AXIS2_PLACEMENT_3D('',#97348,#66146,#66147) ;
#53629=AXIS2_PLACEMENT_3D('',#97349,#66148,#66149) ;
#53630=AXIS2_PLACEMENT_3D('',#97350,#66150,#66151) ;
#53631=AXIS2_PLACEMENT_3D('',#97351,#66152,#66153) ;
#53632=AXIS2_PLACEMENT_3D('',#97353,#66155,#66156) ;
#53633=AXIS2_PLACEMENT_3D('',#97355,#66158,#66159) ;
#53634=AXIS2_PLACEMENT_3D('',#97357,#66161,#66162) ;
#53635=AXIS2_PLACEMENT_3D('',#97358,#66163,#66164) ;
#53636=AXIS2_PLACEMENT_3D('',#97359,#66165,#66166) ;
#53637=AXIS2_PLACEMENT_3D('',#97360,#66167,#66168) ;
#53638=AXIS2_PLACEMENT_3D('',#97362,#66169,#66170) ;
#53639=AXIS2_PLACEMENT_3D('',#97364,#66172,#66173) ;
#53640=AXIS2_PLACEMENT_3D('',#97365,#66174,#66175) ;
#53641=AXIS2_PLACEMENT_3D('',#97366,#66176,#66177) ;
#53642=AXIS2_PLACEMENT_3D('',#97368,#66179,#66180) ;
#53643=AXIS2_PLACEMENT_3D('',#97372,#66182,#66183) ;
#53644=AXIS2_PLACEMENT_3D('',#97373,#66184,#66185) ;
#53645=AXIS2_PLACEMENT_3D('',#97374,#66186,#66187) ;
#53646=AXIS2_PLACEMENT_3D('',#97375,#66188,#66189) ;
#53647=AXIS2_PLACEMENT_3D('',#97377,#66191,#66192) ;
#53648=AXIS2_PLACEMENT_3D('',#97378,#66193,#66194) ;
#53649=AXIS2_PLACEMENT_3D('',#97379,#66195,#66196) ;
#53650=AXIS2_PLACEMENT_3D('',#97380,#66197,#66198) ;
#53651=AXIS2_PLACEMENT_3D('',#97381,#66199,#66200) ;
#53652=AXIS2_PLACEMENT_3D('',#97382,#66201,#66202) ;
#53653=AXIS2_PLACEMENT_3D('',#97383,#66203,#66204) ;
#53654=AXIS2_PLACEMENT_3D('',#97384,#66205,#66206) ;
#53655=AXIS2_PLACEMENT_3D('',#97385,#66207,#66208) ;
#53656=AXIS2_PLACEMENT_3D('',#97386,#66209,#66210) ;
#53657=AXIS2_PLACEMENT_3D('',#97387,#66211,#66212) ;
#53658=AXIS2_PLACEMENT_3D('',#97388,#66213,#66214) ;
#53659=AXIS2_PLACEMENT_3D('',#97389,#66215,#66216) ;
#53660=AXIS2_PLACEMENT_3D('',#97391,#66217,#66218) ;
#53661=AXIS2_PLACEMENT_3D('',#97392,#66219,#66220) ;
#53662=AXIS2_PLACEMENT_3D('',#97393,#66221,#66222) ;
#53663=AXIS2_PLACEMENT_3D('',#97395,#66223,#66224) ;
#53664=AXIS2_PLACEMENT_3D('',#97397,#66226,#66227) ;
#53665=AXIS2_PLACEMENT_3D('',#97400,#66230,#66231) ;
#53666=AXIS2_PLACEMENT_3D('',#97402,#66233,#66234) ;
#53667=AXIS2_PLACEMENT_3D('',#97404,#66236,#66237) ;
#53668=AXIS2_PLACEMENT_3D('',#97405,#66238,#66239) ;
#53669=AXIS2_PLACEMENT_3D('',#97407,#66240,#66241) ;
#53670=AXIS2_PLACEMENT_3D('',#97410,#66243,#66244) ;
#53671=AXIS2_PLACEMENT_3D('',#97411,#66245,#66246) ;
#53672=AXIS2_PLACEMENT_3D('',#97414,#66248,#66249) ;
#53673=AXIS2_PLACEMENT_3D('',#97415,#66250,#66251) ;
#53674=AXIS2_PLACEMENT_3D('',#97416,#66252,#66253) ;
#53675=AXIS2_PLACEMENT_3D('',#97417,#66254,#66255) ;
#53676=AXIS2_PLACEMENT_3D('',#97418,#66256,#66257) ;
#53677=AXIS2_PLACEMENT_3D('',#97419,#66258,#66259) ;
#53678=AXIS2_PLACEMENT_3D('',#97420,#66260,#66261) ;
#53679=AXIS2_PLACEMENT_3D('',#97421,#66262,#66263) ;
#53680=AXIS2_PLACEMENT_3D('',#97422,#66264,#66265) ;
#53681=AXIS2_PLACEMENT_3D('',#97423,#66266,#66267) ;
#53682=AXIS2_PLACEMENT_3D('',#97424,#66268,#66269) ;
#53683=AXIS2_PLACEMENT_3D('',#97426,#66270,#66271) ;
#53684=AXIS2_PLACEMENT_3D('',#97427,#66272,#66273) ;
#53685=AXIS2_PLACEMENT_3D('',#97428,#66274,#66275) ;
#53686=AXIS2_PLACEMENT_3D('',#97430,#66277,#66278) ;
#53687=AXIS2_PLACEMENT_3D('',#97432,#66280,#66281) ;
#53688=AXIS2_PLACEMENT_3D('',#97433,#66282,#66283) ;
#53689=AXIS2_PLACEMENT_3D('',#97434,#66284,#66285) ;
#53690=AXIS2_PLACEMENT_3D('',#97435,#66286,#66287) ;
#53691=AXIS2_PLACEMENT_3D('',#97436,#66288,#66289) ;
#53692=AXIS2_PLACEMENT_3D('',#97438,#66291,#66292) ;
#53693=AXIS2_PLACEMENT_3D('',#97440,#66294,#66295) ;
#53694=AXIS2_PLACEMENT_3D('',#97442,#66297,#66298) ;
#53695=AXIS2_PLACEMENT_3D('',#97444,#66300,#66301) ;
#53696=AXIS2_PLACEMENT_3D('',#97445,#66302,#66303) ;
#53697=AXIS2_PLACEMENT_3D('',#97446,#66304,#66305) ;
#53698=AXIS2_PLACEMENT_3D('',#97448,#66307,#66308) ;
#53699=AXIS2_PLACEMENT_3D('',#97449,#66309,#66310) ;
#53700=AXIS2_PLACEMENT_3D('',#97450,#66311,#66312) ;
#53701=AXIS2_PLACEMENT_3D('',#97451,#66313,#66314) ;
#53702=AXIS2_PLACEMENT_3D('',#97452,#66315,#66316) ;
#53703=AXIS2_PLACEMENT_3D('',#97456,#66319,#66320) ;
#53704=AXIS2_PLACEMENT_3D('',#97460,#66322,#66323) ;
#53705=AXIS2_PLACEMENT_3D('',#97464,#66325,#66326) ;
#53706=AXIS2_PLACEMENT_3D('',#97468,#66329,#66330) ;
#53707=AXIS2_PLACEMENT_3D('',#97470,#66332,#66333) ;
#53708=AXIS2_PLACEMENT_3D('',#97473,#66335,#66336) ;
#53709=AXIS2_PLACEMENT_3D('',#97474,#66337,#66338) ;
#53710=AXIS2_PLACEMENT_3D('',#97478,#66341,#66342) ;
#53711=AXIS2_PLACEMENT_3D('',#97481,#66344,#66345) ;
#53712=AXIS2_PLACEMENT_3D('',#97482,#66346,#66347) ;
#53713=AXIS2_PLACEMENT_3D('',#97486,#66350,#66351) ;
#53714=AXIS2_PLACEMENT_3D('',#97490,#66354,#66355) ;
#53715=AXIS2_PLACEMENT_3D('',#97494,#66358,#66359) ;
#53716=AXIS2_PLACEMENT_3D('',#97497,#66361,#66362) ;
#53717=AXIS2_PLACEMENT_3D('',#97498,#66363,#66364) ;
#53718=AXIS2_PLACEMENT_3D('',#97501,#66366,#66367) ;
#53719=AXIS2_PLACEMENT_3D('',#97502,#66368,#66369) ;
#53720=AXIS2_PLACEMENT_3D('',#97506,#66372,#66373) ;
#53721=AXIS2_PLACEMENT_3D('',#97508,#66375,#66376) ;
#53722=AXIS2_PLACEMENT_3D('',#97509,#66377,#66378) ;
#53723=AXIS2_PLACEMENT_3D('',#97515,#66382,#66383) ;
#53724=AXIS2_PLACEMENT_3D('',#97519,#66386,#66387) ;
#53725=AXIS2_PLACEMENT_3D('',#97523,#66390,#66391) ;
#53726=AXIS2_PLACEMENT_3D('',#97525,#66393,#66394) ;
#53727=AXIS2_PLACEMENT_3D('',#97526,#66395,#66396) ;
#53728=AXIS2_PLACEMENT_3D('',#97533,#66401,#66402) ;
#53729=AXIS2_PLACEMENT_3D('',#97537,#66404,#66405) ;
#53730=AXIS2_PLACEMENT_3D('',#97539,#66407,#66408) ;
#53731=AXIS2_PLACEMENT_3D('',#97541,#66410,#66411) ;
#53732=AXIS2_PLACEMENT_3D('',#97543,#66413,#66414) ;
#53733=AXIS2_PLACEMENT_3D('',#97544,#66415,#66416) ;
#53734=AXIS2_PLACEMENT_3D('',#97547,#66418,#66419) ;
#53735=AXIS2_PLACEMENT_3D('',#97548,#66420,#66421) ;
#53736=AXIS2_PLACEMENT_3D('',#97549,#66422,#66423) ;
#53737=AXIS2_PLACEMENT_3D('',#97550,#66424,#66425) ;
#53738=AXIS2_PLACEMENT_3D('',#97552,#66427,#66428) ;
#53739=AXIS2_PLACEMENT_3D('',#97556,#66432,#66433) ;
#53740=AXIS2_PLACEMENT_3D('',#97557,#66434,#66435) ;
#53741=AXIS2_PLACEMENT_3D('',#97560,#66437,#66438) ;
#53742=AXIS2_PLACEMENT_3D('',#97561,#66439,#66440) ;
#53743=AXIS2_PLACEMENT_3D('',#97563,#66442,#66443) ;
#53744=AXIS2_PLACEMENT_3D('',#97565,#66445,#66446) ;
#53745=AXIS2_PLACEMENT_3D('',#97566,#66447,#66448) ;
#53746=AXIS2_PLACEMENT_3D('',#97568,#66450,#66451) ;
#53747=AXIS2_PLACEMENT_3D('',#97569,#66452,#66453) ;
#53748=AXIS2_PLACEMENT_3D('',#97570,#66454,#66455) ;
#53749=AXIS2_PLACEMENT_3D('',#97571,#66456,#66457) ;
#53750=AXIS2_PLACEMENT_3D('',#97591,#66459,#66460) ;
#53751=AXIS2_PLACEMENT_3D('',#97592,#66461,#66462) ;
#53752=AXIS2_PLACEMENT_3D('',#97594,#66463,#66464) ;
#53753=AXIS2_PLACEMENT_3D('',#97596,#66465,#66466) ;
#53754=AXIS2_PLACEMENT_3D('',#97597,#66467,#66468) ;
#53755=AXIS2_PLACEMENT_3D('',#97598,#66469,#66470) ;
#53756=AXIS2_PLACEMENT_3D('',#97616,#66471,#66472) ;
#53757=AXIS2_PLACEMENT_3D('',#97695,#66473,#66474) ;
#53758=AXIS2_PLACEMENT_3D('',#97696,#66475,#66476) ;
#53759=AXIS2_PLACEMENT_3D('',#97724,#66478,#66479) ;
#53760=AXIS2_PLACEMENT_3D('',#97729,#66480,#66481) ;
#53761=AXIS2_PLACEMENT_3D('',#97730,#66482,#66483) ;
#53762=AXIS2_PLACEMENT_3D('',#97732,#66484,#66485) ;
#53763=AXIS2_PLACEMENT_3D('',#97733,#66486,#66487) ;
#53764=AXIS2_PLACEMENT_3D('',#97734,#66488,#66489) ;
#53765=AXIS2_PLACEMENT_3D('',#97736,#66491,#66492) ;
#53766=AXIS2_PLACEMENT_3D('',#97737,#66493,#66494) ;
#53767=AXIS2_PLACEMENT_3D('',#97739,#66495,#66496) ;
#53768=AXIS2_PLACEMENT_3D('',#97740,#66497,#66498) ;
#53769=AXIS2_PLACEMENT_3D('',#97762,#66499,#66500) ;
#53770=AXIS2_PLACEMENT_3D('',#97763,#66501,#66502) ;
#53771=AXIS2_PLACEMENT_3D('',#97764,#66503,#66504) ;
#53772=AXIS2_PLACEMENT_3D('',#97766,#66506,#66507) ;
#53773=AXIS2_PLACEMENT_3D('',#97769,#66508,#66509) ;
#53774=AXIS2_PLACEMENT_3D('',#97770,#66510,#66511) ;
#53775=AXIS2_PLACEMENT_3D('',#97808,#66512,#66513) ;
#53776=AXIS2_PLACEMENT_3D('',#97814,#66514,#66515) ;
#53777=AXIS2_PLACEMENT_3D('',#97815,#66516,#66517) ;
#53778=AXIS2_PLACEMENT_3D('',#97819,#66519,#66520) ;
#53779=AXIS2_PLACEMENT_3D('',#97836,#66521,#66522) ;
#53780=AXIS2_PLACEMENT_3D('',#97837,#66523,#66524) ;
#53781=AXIS2_PLACEMENT_3D('',#97868,#66525,#66526) ;
#53782=AXIS2_PLACEMENT_3D('',#97895,#66527,#66528) ;
#53783=AXIS2_PLACEMENT_3D('',#97896,#66529,#66530) ;
#53784=AXIS2_PLACEMENT_3D('',#97897,#66531,#66532) ;
#53785=AXIS2_PLACEMENT_3D('',#97899,#66533,#66534) ;
#53786=AXIS2_PLACEMENT_3D('',#97900,#66535,#66536) ;
#53787=AXIS2_PLACEMENT_3D('',#97901,#66537,#66538) ;
#53788=AXIS2_PLACEMENT_3D('',#97924,#66540,#66541) ;
#53789=AXIS2_PLACEMENT_3D('',#97930,#66542,#66543) ;
#53790=AXIS2_PLACEMENT_3D('',#97931,#66544,#66545) ;
#53791=AXIS2_PLACEMENT_3D('',#97935,#66547,#66548) ;
#53792=AXIS2_PLACEMENT_3D('',#97952,#66549,#66550) ;
#53793=AXIS2_PLACEMENT_3D('',#97953,#66551,#66552) ;
#53794=AXIS2_PLACEMENT_3D('',#97984,#66553,#66554) ;
#53795=AXIS2_PLACEMENT_3D('',#97985,#66555,#66556) ;
#53796=AXIS2_PLACEMENT_3D('',#97987,#66557,#66558) ;
#53797=AXIS2_PLACEMENT_3D('',#97990,#66560,#66561) ;
#53798=AXIS2_PLACEMENT_3D('',#97991,#66562,#66563) ;
#53799=AXIS2_PLACEMENT_3D('',#97992,#66564,#66565) ;
#53800=AXIS2_PLACEMENT_3D('',#98002,#66566,#66567) ;
#53801=AXIS2_PLACEMENT_3D('',#98003,#66568,#66569) ;
#53802=AXIS2_PLACEMENT_3D('',#98005,#66571,#66572) ;
#53803=AXIS2_PLACEMENT_3D('',#98007,#66573,#66574) ;
#53804=AXIS2_PLACEMENT_3D('',#98010,#66576,#66577) ;
#53805=AXIS2_PLACEMENT_3D('',#98011,#66578,#66579) ;
#53806=AXIS2_PLACEMENT_3D('',#98012,#66580,#66581) ;
#53807=AXIS2_PLACEMENT_3D('',#98013,#66582,#66583) ;
#53808=AXIS2_PLACEMENT_3D('',#98016,#66584,#66585) ;
#53809=AXIS2_PLACEMENT_3D('',#98020,#66587,#66588) ;
#53810=AXIS2_PLACEMENT_3D('',#98042,#66590,#66591) ;
#53811=AXIS2_PLACEMENT_3D('',#98043,#66592,#66593) ;
#53812=AXIS2_PLACEMENT_3D('',#98053,#66594,#66595) ;
#53813=AXIS2_PLACEMENT_3D('',#98076,#66596,#66597) ;
#53814=AXIS2_PLACEMENT_3D('',#98077,#66598,#66599) ;
#53815=AXIS2_PLACEMENT_3D('',#98078,#66600,#66601) ;
#53816=AXIS2_PLACEMENT_3D('',#98079,#66602,#66603) ;
#53817=AXIS2_PLACEMENT_3D('',#98082,#66604,#66605) ;
#53818=AXIS2_PLACEMENT_3D('',#98085,#66608,#66609) ;
#53819=AXIS2_PLACEMENT_3D('',#98089,#66611,#66612) ;
#53820=AXIS2_PLACEMENT_3D('',#98113,#66614,#66615) ;
#53821=AXIS2_PLACEMENT_3D('',#98114,#66616,#66617) ;
#53822=AXIS2_PLACEMENT_3D('',#98115,#66618,#66619) ;
#53823=AXIS2_PLACEMENT_3D('',#98116,#66620,#66621) ;
#53824=AXIS2_PLACEMENT_3D('',#98119,#66624,#66625) ;
#53825=AXIS2_PLACEMENT_3D('',#98122,#66628,#66629) ;
#53826=AXIS2_PLACEMENT_3D('',#98124,#66631,#66632) ;
#53827=AXIS2_PLACEMENT_3D('',#98126,#66634,#66635) ;
#53828=AXIS2_PLACEMENT_3D('',#98128,#66637,#66638) ;
#53829=AXIS2_PLACEMENT_3D('',#98129,#66639,#66640) ;
#53830=AXIS2_PLACEMENT_3D('',#98130,#66641,#66642) ;
#53831=AXIS2_PLACEMENT_3D('',#98131,#66643,#66644) ;
#53832=AXIS2_PLACEMENT_3D('',#98132,#66645,#66646) ;
#53833=AXIS2_PLACEMENT_3D('',#98135,#66649,#66650) ;
#53834=AXIS2_PLACEMENT_3D('',#98138,#66653,#66654) ;
#53835=AXIS2_PLACEMENT_3D('',#98144,#66658,#66659) ;
#53836=AXIS2_PLACEMENT_3D('',#98146,#66660,#66661) ;
#53837=AXIS2_PLACEMENT_3D('',#98148,#66663,#66664) ;
#53838=AXIS2_PLACEMENT_3D('',#98152,#66667,#66668) ;
#53839=AXIS2_PLACEMENT_3D('',#98156,#66671,#66672) ;
#53840=AXIS2_PLACEMENT_3D('',#98158,#66673,#66674) ;
#53841=AXIS2_PLACEMENT_3D('',#98160,#66676,#66677) ;
#53842=AXIS2_PLACEMENT_3D('',#98164,#66680,#66681) ;
#53843=AXIS2_PLACEMENT_3D('',#98166,#66682,#66683) ;
#53844=AXIS2_PLACEMENT_3D('',#98168,#66685,#66686) ;
#53845=AXIS2_PLACEMENT_3D('',#98172,#66689,#66690) ;
#53846=AXIS2_PLACEMENT_3D('',#98196,#66694,#66695) ;
#53847=AXIS2_PLACEMENT_3D('',#98218,#66698,#66699) ;
#53848=AXIS2_PLACEMENT_3D('',#98220,#66701,#66702) ;
#53849=AXIS2_PLACEMENT_3D('',#98223,#66704,#66705) ;
#53850=AXIS2_PLACEMENT_3D('',#98224,#66706,#66707) ;
#53851=AXIS2_PLACEMENT_3D('',#98225,#66708,#66709) ;
#53852=AXIS2_PLACEMENT_3D('',#98228,#66711,#66712) ;
#53853=AXIS2_PLACEMENT_3D('',#98229,#66713,#66714) ;
#53854=AXIS2_PLACEMENT_3D('',#98235,#66718,#66719) ;
#53855=AXIS2_PLACEMENT_3D('',#98237,#66720,#66721) ;
#53856=AXIS2_PLACEMENT_3D('',#98239,#66723,#66724) ;
#53857=AXIS2_PLACEMENT_3D('',#98243,#66727,#66728) ;
#53858=AXIS2_PLACEMENT_3D('',#98245,#66729,#66730) ;
#53859=AXIS2_PLACEMENT_3D('',#98247,#66732,#66733) ;
#53860=AXIS2_PLACEMENT_3D('',#98251,#66736,#66737) ;
#53861=AXIS2_PLACEMENT_3D('',#98254,#66738,#66739) ;
#53862=AXIS2_PLACEMENT_3D('',#98257,#66742,#66743) ;
#53863=AXIS2_PLACEMENT_3D('',#98261,#66746,#66747) ;
#53864=AXIS2_PLACEMENT_3D('',#98263,#66748,#66749) ;
#53865=AXIS2_PLACEMENT_3D('',#98265,#66751,#66752) ;
#53866=AXIS2_PLACEMENT_3D('',#98269,#66755,#66756) ;
#53867=AXIS2_PLACEMENT_3D('',#98273,#66759,#66760) ;
#53868=AXIS2_PLACEMENT_3D('',#98275,#66761,#66762) ;
#53869=AXIS2_PLACEMENT_3D('',#98277,#66764,#66765) ;
#53870=AXIS2_PLACEMENT_3D('',#98281,#66768,#66769) ;
#53871=AXIS2_PLACEMENT_3D('',#98284,#66771,#66772) ;
#53872=AXIS2_PLACEMENT_3D('',#98285,#66773,#66774) ;
#53873=AXIS2_PLACEMENT_3D('',#98291,#66778,#66779) ;
#53874=AXIS2_PLACEMENT_3D('',#98293,#66780,#66781) ;
#53875=AXIS2_PLACEMENT_3D('',#98295,#66783,#66784) ;
#53876=AXIS2_PLACEMENT_3D('',#98299,#66787,#66788) ;
#53877=AXIS2_PLACEMENT_3D('',#98301,#66789,#66790) ;
#53878=AXIS2_PLACEMENT_3D('',#98303,#66792,#66793) ;
#53879=AXIS2_PLACEMENT_3D('',#98327,#66797,#66798) ;
#53880=AXIS2_PLACEMENT_3D('',#98330,#66799,#66800) ;
#53881=AXIS2_PLACEMENT_3D('',#98333,#66803,#66804) ;
#53882=AXIS2_PLACEMENT_3D('',#98337,#66807,#66808) ;
#53883=AXIS2_PLACEMENT_3D('',#98339,#66809,#66810) ;
#53884=AXIS2_PLACEMENT_3D('',#98341,#66812,#66813) ;
#53885=AXIS2_PLACEMENT_3D('',#98345,#66816,#66817) ;
#53886=AXIS2_PLACEMENT_3D('',#98347,#66819,#66820) ;
#53887=AXIS2_PLACEMENT_3D('',#98351,#66823,#66824) ;
#53888=AXIS2_PLACEMENT_3D('',#98354,#66825,#66826) ;
#53889=AXIS2_PLACEMENT_3D('',#98357,#66829,#66830) ;
#53890=AXIS2_PLACEMENT_3D('',#98362,#66834,#66835) ;
#53891=AXIS2_PLACEMENT_3D('',#98364,#66836,#66837) ;
#53892=AXIS2_PLACEMENT_3D('',#98366,#66839,#66840) ;
#53893=AXIS2_PLACEMENT_3D('',#98370,#66843,#66844) ;
#53894=AXIS2_PLACEMENT_3D('',#98371,#66845,#66846) ;
#53895=AXIS2_PLACEMENT_3D('',#98372,#66847,#66848) ;
#53896=AXIS2_PLACEMENT_3D('',#98375,#66849,#66850) ;
#53897=AXIS2_PLACEMENT_3D('',#98378,#66853,#66854) ;
#53898=AXIS2_PLACEMENT_3D('',#98382,#66857,#66858) ;
#53899=AXIS2_PLACEMENT_3D('',#98384,#66859,#66860) ;
#53900=AXIS2_PLACEMENT_3D('',#98386,#66862,#66863) ;
#53901=AXIS2_PLACEMENT_3D('',#98390,#66866,#66867) ;
#53902=AXIS2_PLACEMENT_3D('',#98394,#66870,#66871) ;
#53903=AXIS2_PLACEMENT_3D('',#98396,#66872,#66873) ;
#53904=AXIS2_PLACEMENT_3D('',#98398,#66875,#66876) ;
#53905=AXIS2_PLACEMENT_3D('',#98402,#66879,#66880) ;
#53906=AXIS2_PLACEMENT_3D('',#98404,#66881,#66882) ;
#53907=AXIS2_PLACEMENT_3D('',#98406,#66884,#66885) ;
#53908=AXIS2_PLACEMENT_3D('',#98410,#66888,#66889) ;
#53909=AXIS2_PLACEMENT_3D('',#98414,#66892,#66893) ;
#53910=AXIS2_PLACEMENT_3D('',#98416,#66894,#66895) ;
#53911=AXIS2_PLACEMENT_3D('',#98418,#66897,#66898) ;
#53912=AXIS2_PLACEMENT_3D('',#98422,#66901,#66902) ;
#53913=AXIS2_PLACEMENT_3D('',#98424,#66903,#66904) ;
#53914=AXIS2_PLACEMENT_3D('',#98426,#66906,#66907) ;
#53915=AXIS2_PLACEMENT_3D('',#98428,#66909,#66910) ;
#53916=AXIS2_PLACEMENT_3D('',#98429,#66911,#66912) ;
#53917=AXIS2_PLACEMENT_3D('',#98453,#66916,#66917) ;
#53918=AXIS2_PLACEMENT_3D('',#98457,#66920,#66921) ;
#53919=AXIS2_PLACEMENT_3D('',#98459,#66922,#66923) ;
#53920=AXIS2_PLACEMENT_3D('',#98461,#66925,#66926) ;
#53921=AXIS2_PLACEMENT_3D('',#98465,#66929,#66930) ;
#53922=AXIS2_PLACEMENT_3D('',#98466,#66931,#66932) ;
#53923=AXIS2_PLACEMENT_3D('',#98467,#66933,#66934) ;
#53924=AXIS2_PLACEMENT_3D('',#98488,#66936,#66937) ;
#53925=AXIS2_PLACEMENT_3D('',#98492,#66940,#66941) ;
#53926=AXIS2_PLACEMENT_3D('',#98496,#66944,#66945) ;
#53927=AXIS2_PLACEMENT_3D('',#98498,#66946,#66947) ;
#53928=AXIS2_PLACEMENT_3D('',#98500,#66949,#66950) ;
#53929=AXIS2_PLACEMENT_3D('',#98504,#66953,#66954) ;
#53930=AXIS2_PLACEMENT_3D('',#98506,#66955,#66956) ;
#53931=AXIS2_PLACEMENT_3D('',#98508,#66958,#66959) ;
#53932=AXIS2_PLACEMENT_3D('',#98510,#66961,#66962) ;
#53933=AXIS2_PLACEMENT_3D('',#98511,#66963,#66964) ;
#53934=AXIS2_PLACEMENT_3D('',#98513,#66965,#66966) ;
#53935=AXIS2_PLACEMENT_3D('',#98515,#66968,#66969) ;
#53936=AXIS2_PLACEMENT_3D('',#98519,#66972,#66973) ;
#53937=AXIS2_PLACEMENT_3D('',#98523,#66976,#66977) ;
#53938=AXIS2_PLACEMENT_3D('',#98527,#66980,#66981) ;
#53939=AXIS2_PLACEMENT_3D('',#98531,#66984,#66985) ;
#53940=AXIS2_PLACEMENT_3D('',#98535,#66988,#66989) ;
#53941=AXIS2_PLACEMENT_3D('',#98537,#66990,#66991) ;
#53942=AXIS2_PLACEMENT_3D('',#98539,#66993,#66994) ;
#53943=AXIS2_PLACEMENT_3D('',#98541,#66995,#66996) ;
#53944=AXIS2_PLACEMENT_3D('',#98543,#66998,#66999) ;
#53945=AXIS2_PLACEMENT_3D('',#98545,#67000,#67001) ;
#53946=AXIS2_PLACEMENT_3D('',#98547,#67003,#67004) ;
#53947=AXIS2_PLACEMENT_3D('',#98551,#67007,#67008) ;
#53948=AXIS2_PLACEMENT_3D('',#98555,#67011,#67012) ;
#53949=AXIS2_PLACEMENT_3D('',#98557,#67013,#67014) ;
#53950=AXIS2_PLACEMENT_3D('',#98559,#67016,#67017) ;
#53951=AXIS2_PLACEMENT_3D('',#98563,#67020,#67021) ;
#53952=AXIS2_PLACEMENT_3D('',#98565,#67022,#67023) ;
#53953=AXIS2_PLACEMENT_3D('',#98567,#67025,#67026) ;
#53954=AXIS2_PLACEMENT_3D('',#98569,#67028,#67029) ;
#53955=AXIS2_PLACEMENT_3D('',#98570,#67030,#67031) ;
#53956=AXIS2_PLACEMENT_3D('',#98572,#67032,#67033) ;
#53957=AXIS2_PLACEMENT_3D('',#98574,#67035,#67036) ;
#53958=AXIS2_PLACEMENT_3D('',#98578,#67039,#67040) ;
#53959=AXIS2_PLACEMENT_3D('',#98580,#67041,#67042) ;
#53960=AXIS2_PLACEMENT_3D('',#98582,#67044,#67045) ;
#53961=AXIS2_PLACEMENT_3D('',#98586,#67048,#67049) ;
#53962=AXIS2_PLACEMENT_3D('',#98588,#67050,#67051) ;
#53963=AXIS2_PLACEMENT_3D('',#98590,#67053,#67054) ;
#53964=AXIS2_PLACEMENT_3D('',#98592,#67056,#67057) ;
#53965=AXIS2_PLACEMENT_3D('',#98593,#67058,#67059) ;
#53966=AXIS2_PLACEMENT_3D('',#98594,#67060,#67061) ;
#53967=AXIS2_PLACEMENT_3D('',#98596,#67062,#67063) ;
#53968=AXIS2_PLACEMENT_3D('',#98598,#67065,#67066) ;
#53969=AXIS2_PLACEMENT_3D('',#98602,#67069,#67070) ;
#53970=AXIS2_PLACEMENT_3D('',#98603,#67071,#67072) ;
#53971=AXIS2_PLACEMENT_3D('',#98606,#67075,#67076) ;
#53972=AXIS2_PLACEMENT_3D('',#98609,#67079,#67080) ;
#53973=AXIS2_PLACEMENT_3D('',#98611,#67082,#67083) ;
#53974=AXIS2_PLACEMENT_3D('',#98614,#67086,#67087) ;
#53975=AXIS2_PLACEMENT_3D('',#98615,#67088,#67089) ;
#53976=AXIS2_PLACEMENT_3D('',#98617,#67091,#67092) ;
#53977=AXIS2_PLACEMENT_3D('',#98619,#67094,#67095) ;
#53978=AXIS2_PLACEMENT_3D('',#98621,#67097,#67098) ;
#53979=AXIS2_PLACEMENT_3D('',#98623,#67100,#67101) ;
#53980=AXIS2_PLACEMENT_3D('',#98625,#67103,#67104) ;
#53981=AXIS2_PLACEMENT_3D('',#98626,#67105,#67106) ;
#53982=AXIS2_PLACEMENT_3D('',#98628,#67107,#67108) ;
#53983=AXIS2_PLACEMENT_3D('',#98629,#67109,#67110) ;
#53984=AXIS2_PLACEMENT_3D('',#98630,#67111,#67112) ;
#53985=AXIS2_PLACEMENT_3D('',#98632,#67114,#67115) ;
#53986=AXIS2_PLACEMENT_3D('',#98633,#67116,#67117) ;
#53987=AXIS2_PLACEMENT_3D('',#98635,#67119,#67120) ;
#53988=AXIS2_PLACEMENT_3D('',#98637,#67122,#67123) ;
#53989=AXIS2_PLACEMENT_3D('',#98638,#67124,#67125) ;
#53990=AXIS2_PLACEMENT_3D('',#98640,#67127,#67128) ;
#53991=AXIS2_PLACEMENT_3D('',#98641,#67129,#67130) ;
#53992=AXIS2_PLACEMENT_3D('',#98643,#67132,#67133) ;
#53993=AXIS2_PLACEMENT_3D('',#98644,#67134,#67135) ;
#53994=AXIS2_PLACEMENT_3D('',#98646,#67137,#67138) ;
#53995=AXIS2_PLACEMENT_3D('',#98647,#67139,#67140) ;
#53996=AXIS2_PLACEMENT_3D('',#98648,#67141,#67142) ;
#53997=AXIS2_PLACEMENT_3D('',#98650,#67144,#67145) ;
#53998=AXIS2_PLACEMENT_3D('',#98651,#67146,#67147) ;
#53999=AXIS2_PLACEMENT_3D('',#98653,#67149,#67150) ;
#54000=AXIS2_PLACEMENT_3D('',#98655,#67152,#67153) ;
#54001=AXIS2_PLACEMENT_3D('',#98657,#67155,#67156) ;
#54002=AXIS2_PLACEMENT_3D('',#98659,#67158,#67159) ;
#54003=AXIS2_PLACEMENT_3D('',#98661,#67161,#67162) ;
#54004=AXIS2_PLACEMENT_3D('',#98662,#67163,#67164) ;
#54005=AXIS2_PLACEMENT_3D('',#98664,#67166,#67167) ;
#54006=AXIS2_PLACEMENT_3D('',#98665,#67168,#67169) ;
#54007=AXIS2_PLACEMENT_3D('',#98668,#67172,#67173) ;
#54008=AXIS2_PLACEMENT_3D('',#98669,#67174,#67175) ;
#54009=AXIS2_PLACEMENT_3D('',#98670,#67176,#67177) ;
#54010=AXIS2_PLACEMENT_3D('',#98671,#67178,#67179) ;
#63089=DIRECTION('axis',(0.,0.,1.)) ;
#63090=DIRECTION('refdir',(1.,0.,0.)) ;
#63091=DIRECTION('center_axis',(1.,0.,0.)) ;
#63092=DIRECTION('ref_axis',(0.,0.,-1.)) ;
#63093=DIRECTION('center_axis',(0.245297658020056,0.605609246625242,0.757011558281565)) ;
#63094=DIRECTION('ref_axis',(3.02873619539704E-17,0.780868809443035,-0.624695047554418)) ;
#63095=DIRECTION('center_axis',(0.245297658020056,0.605609246625242,0.757011558281565)) ;
#63096=DIRECTION('ref_axis',(3.02873619539704E-17,0.780868809443035,-0.624695047554418)) ;
#63097=DIRECTION('center_axis',(0.,-1.,0.)) ;
#63098=DIRECTION('ref_axis',(-1.,0.,0.)) ;
#63099=DIRECTION('center_axis',(0.,-1.,0.)) ;
#63100=DIRECTION('ref_axis',(-1.,0.,0.)) ;
#63101=DIRECTION('center_axis',(0.,1.,0.)) ;
#63102=DIRECTION('ref_axis',(-1.,0.,0.)) ;
#63103=DIRECTION('',(-1.,0.,0.)) ;
#63104=DIRECTION('',(0.,0.,1.)) ;
#63105=DIRECTION('',(-1.,0.,0.)) ;
#63106=DIRECTION('',(0.,0.,1.)) ;
#63107=DIRECTION('',(0.,0.,1.)) ;
#63108=DIRECTION('',(0.,0.,1.)) ;
#63109=DIRECTION('',(0.,0.,1.)) ;
#63110=DIRECTION('',(0.,0.,1.)) ;
#63111=DIRECTION('',(0.,0.,1.)) ;
#63112=DIRECTION('center_axis',(0.,-1.,0.)) ;
#63113=DIRECTION('ref_axis',(1.,0.,0.)) ;
#63114=DIRECTION('',(1.,0.,0.)) ;
#63115=DIRECTION('',(0.,0.,1.)) ;
#63116=DIRECTION('',(1.,0.,0.)) ;
#63117=DIRECTION('center_axis',(1.,0.,0.)) ;
#63118=DIRECTION('ref_axis',(0.,1.,0.)) ;
#63119=DIRECTION('',(0.,1.,0.)) ;
#63120=DIRECTION('',(0.,1.,0.)) ;
#63121=DIRECTION('center_axis',(1.,0.,0.)) ;
#63122=DIRECTION('ref_axis',(0.,1.,0.)) ;
#63123=DIRECTION('',(0.,1.,0.)) ;
#63124=DIRECTION('',(0.,0.,1.)) ;
#63125=DIRECTION('',(0.,1.,0.)) ;
#63126=DIRECTION('',(0.,0.,1.)) ;
#63127=DIRECTION('center_axis',(0.,1.,0.)) ;
#63128=DIRECTION('ref_axis',(-1.,0.,0.)) ;
#63129=DIRECTION('',(-1.,0.,0.)) ;
#63130=DIRECTION('',(0.,0.,1.)) ;
#63131=DIRECTION('',(-1.,0.,0.)) ;
#63132=DIRECTION('',(0.,0.,1.)) ;
#63133=DIRECTION('',(0.,0.,1.)) ;
#63134=DIRECTION('',(0.,0.,1.)) ;
#63135=DIRECTION('',(0.,0.,1.)) ;
#63136=DIRECTION('center_axis',(-0.843775502275604,0.536696284465946,0.)) ;
#63137=DIRECTION('ref_axis',(-0.536696284465946,-0.843775502275604,0.)) ;
#63138=DIRECTION('',(-0.536696284465946,-0.843775502275604,0.)) ;
#63139=DIRECTION('',(0.,0.,1.)) ;
#63140=DIRECTION('',(-0.536696284465946,-0.843775502275604,0.)) ;
#63141=DIRECTION('center_axis',(0.,1.,0.)) ;
#63142=DIRECTION('ref_axis',(-1.,0.,0.)) ;
#63143=DIRECTION('',(-1.,0.,0.)) ;
#63144=DIRECTION('',(0.,0.,1.)) ;
#63145=DIRECTION('',(-1.,0.,0.)) ;
#63146=DIRECTION('center_axis',(0.842616363087172,-0.538514312398237,0.)) ;
#63147=DIRECTION('ref_axis',(0.538514312398237,0.842616363087172,0.)) ;
#63148=DIRECTION('',(0.538514312398237,0.842616363087173,0.)) ;
#63149=DIRECTION('',(0.,0.,1.)) ;
#63150=DIRECTION('',(0.538514312398237,0.842616363087172,0.)) ;
#63151=DIRECTION('',(0.,0.,1.)) ;
#63152=DIRECTION('',(0.,0.,1.)) ;
#63153=DIRECTION('',(0.,0.,1.)) ;
#63154=DIRECTION('',(0.,0.,1.)) ;
#63155=DIRECTION('',(0.,0.,1.)) ;
#63156=DIRECTION('',(0.,0.,1.)) ;
#63157=DIRECTION('',(0.,0.,1.)) ;
#63158=DIRECTION('center_axis',(0.,-1.,0.)) ;
#63159=DIRECTION('ref_axis',(1.,0.,0.)) ;
#63160=DIRECTION('',(1.,0.,0.)) ;
#63161=DIRECTION('',(0.,0.,1.)) ;
#63162=DIRECTION('',(1.,0.,0.)) ;
#63163=DIRECTION('center_axis',(-1.,0.,0.)) ;
#63164=DIRECTION('ref_axis',(0.,-1.,0.)) ;
#63165=DIRECTION('',(0.,-1.,0.)) ;
#63166=DIRECTION('',(0.,0.,1.)) ;
#63167=DIRECTION('',(0.,-1.,0.)) ;
#63168=DIRECTION('center_axis',(0.,1.,0.)) ;
#63169=DIRECTION('ref_axis',(-1.,0.,0.)) ;
#63170=DIRECTION('',(-1.,0.,0.)) ;
#63171=DIRECTION('',(-1.,0.,0.)) ;
#63172=DIRECTION('center_axis',(0.,0.,-1.)) ;
#63173=DIRECTION('ref_axis',(1.,0.,0.)) ;
#63174=DIRECTION('center_axis',(0.,0.,-1.)) ;
#63175=DIRECTION('ref_axis',(1.,0.,0.)) ;
#63176=DIRECTION('',(9.79313055424617E-16,-1.,0.)) ;
#63177=DIRECTION('',(-1.,4.33257765707378E-15,0.)) ;
#63178=DIRECTION('center_axis',(0.,0.,1.)) ;
#63179=DIRECTION('ref_axis',(1.,0.,0.)) ;
#63180=DIRECTION('',(-1.,4.33257765707378E-15,0.)) ;
#63181=DIRECTION('center_axis',(0.,0.,-1.)) ;
#63182=DIRECTION('ref_axis',(-0.933145676371942,0.359498465460357,0.)) ;
#63183=DIRECTION('',(0.,1.,0.)) ;
#63184=DIRECTION('center_axis',(0.,0.,1.)) ;
#63185=DIRECTION('ref_axis',(0.923879532511298,-0.382683432365064,0.)) ;
#63186=DIRECTION('',(0.70710678118654,0.707106781186555,0.)) ;
#63187=DIRECTION('center_axis',(0.,0.,-1.)) ;
#63188=DIRECTION('ref_axis',(-0.744997757011426,0.66706696968741,0.)) ;
#63189=DIRECTION('center_axis',(0.,0.,1.)) ;
#63190=DIRECTION('ref_axis',(0.433012701892204,-0.901387818866005,0.)) ;
#63191=DIRECTION('',(1.,-3.55271367880048E-14,0.)) ;
#63192=DIRECTION('center_axis',(0.,0.,-1.)) ;
#63193=DIRECTION('ref_axis',(-0.707106781186519,0.707106781186576,0.)) ;
#63194=DIRECTION('',(3.67742382159233E-14,1.,0.)) ;
#63195=DIRECTION('center_axis',(0.,0.,1.)) ;
#63196=DIRECTION('ref_axis',(0.683460430828417,-0.729987561189802,0.)) ;
#63197=DIRECTION('',(0.997835226140326,-0.0657636789837963,0.)) ;
#63198=DIRECTION('center_axis',(0.,0.,1.)) ;
#63199=DIRECTION('ref_axis',(-0.624947614806638,-0.780666688637023,0.)) ;
#63200=DIRECTION('',(0.573576436351043,-0.819152044288994,0.)) ;
#63201=DIRECTION('center_axis',(0.,0.,1.)) ;
#63202=DIRECTION('ref_axis',(-0.95371695074823,-0.300705799504264,0.)) ;
#63203=DIRECTION('',(1.38777878078145E-15,-1.,0.)) ;
#63204=DIRECTION('center_axis',(0.,0.,1.)) ;
#63205=DIRECTION('ref_axis',(0.,-1.,0.)) ;
#63206=DIRECTION('',(0.,1.,0.)) ;
#63207=DIRECTION('',(-1.,0.,0.)) ;
#63208=DIRECTION('center_axis',(0.,0.,1.)) ;
#63209=DIRECTION('ref_axis',(0.409537713826739,-0.912293188045141,0.)) ;
#63210=DIRECTION('',(0.,0.,1.)) ;
#63211=DIRECTION('center_axis',(0.,0.,1.)) ;
#63212=DIRECTION('ref_axis',(0.409537713799064,-0.912293188057565,0.)) ;
#63213=DIRECTION('',(0.,0.,-1.)) ;
#63214=DIRECTION('',(0.,0.,-1.)) ;
#63215=DIRECTION('center_axis',(-4.3325776570738E-15,-1.,0.)) ;
#63216=DIRECTION('ref_axis',(0.,0.,-1.)) ;
#63217=DIRECTION('center_axis',(1.,0.,0.)) ;
#63218=DIRECTION('ref_axis',(0.,-1.,0.)) ;
#63219=DIRECTION('center_axis',(4.3325776570738E-15,1.,0.)) ;
#63220=DIRECTION('ref_axis',(0.70710678118654,-3.06359504133418E-15,0.707106781186555)) ;
#63221=DIRECTION('center_axis',(-4.3325776570738E-15,-1.,0.)) ;
#63222=DIRECTION('ref_axis',(0.70710678118654,-3.06359504133418E-15,0.707106781186555)) ;
#63223=DIRECTION('center_axis',(-1.,4.3325776570738E-15,0.)) ;
#63224=DIRECTION('ref_axis',(-3.06359504133427E-15,-0.707106781186561,-0.707106781186534)) ;
#63225=DIRECTION('center_axis',(1.,0.,0.)) ;
#63226=DIRECTION('ref_axis',(0.,-1.,0.)) ;
#63227=DIRECTION('',(1.,-4.3325776570738E-15,0.)) ;
#63228=DIRECTION('',(-1.,4.3325776570738E-15,0.)) ;
#63229=DIRECTION('center_axis',(0.,-1.,0.)) ;
#63230=DIRECTION('ref_axis',(-1.,0.,0.)) ;
#63231=DIRECTION('center_axis',(0.,0.,1.)) ;
#63232=DIRECTION('ref_axis',(-0.707106781186558,-0.707106781186537,0.)) ;
#63233=DIRECTION('center_axis',(0.,0.,-1.)) ;
#63234=DIRECTION('ref_axis',(-0.707106781186559,-0.707106781186536,0.)) ;
#63235=DIRECTION('center_axis',(0.,-1.,0.)) ;
#63236=DIRECTION('ref_axis',(-0.707106781186534,0.,-0.707106781186561)) ;
#63237=DIRECTION('center_axis',(0.,-1.,0.)) ;
#63238=DIRECTION('ref_axis',(-1.,0.,0.)) ;
#63239=DIRECTION('',(0.,-1.,0.)) ;
#63240=DIRECTION('',(0.,1.,0.)) ;
#63241=DIRECTION('center_axis',(-1.,-6.18537818639092E-13,1.57759909874306E-11)) ;
#63242=DIRECTION('ref_axis',(1.56498614886827E-11,0.0935501748139615,0.99561456638213)) ;
#63243=DIRECTION('center_axis',(1.,0.,0.)) ;
#63244=DIRECTION('ref_axis',(0.,-1.,0.)) ;
#63245=DIRECTION('',(0.,0.,-1.)) ;
#63246=DIRECTION('',(0.,-1.,0.)) ;
#63247=DIRECTION('',(0.,0.,-1.)) ;
#63248=DIRECTION('',(0.,-1.,0.)) ;
#63249=DIRECTION('',(0.,0.,-1.)) ;
#63250=DIRECTION('center_axis',(0.,0.,1.)) ;
#63251=DIRECTION('ref_axis',(-0.707106781186548,-0.707106781186548,0.)) ;
#63252=DIRECTION('',(0.,0.,1.)) ;
#63253=DIRECTION('center_axis',(0.,0.,-1.)) ;
#63254=DIRECTION('ref_axis',(-0.707106781186548,-0.707106781186548,0.)) ;
#63255=DIRECTION('center_axis',(-4.3325776570738E-15,-1.,0.)) ;
#63256=DIRECTION('ref_axis',(1.,-4.3325776570738E-15,0.)) ;
#63257=DIRECTION('',(0.,0.,1.)) ;
#63258=DIRECTION('',(-1.,4.3325776570738E-15,0.)) ;
#63259=DIRECTION('center_axis',(1.,0.,0.)) ;
#63260=DIRECTION('ref_axis',(0.,1.,0.)) ;
#63261=DIRECTION('center_axis',(0.,1.,2.96059473233375E-13)) ;
#63262=DIRECTION('ref_axis',(1.,0.,0.)) ;
#63263=DIRECTION('center_axis',(-0.938080487976382,0.346417375542847,-6.15360874332621E-14)) ;
#63264=DIRECTION('ref_axis',(0.346417375542847,0.938080487976382,-1.9888398296556E-29)) ;
#63265=DIRECTION('center_axis',(0.,1.,0.)) ;
#63266=DIRECTION('ref_axis',(0.707106781186534,0.,-0.707106781186561)) ;
#63267=DIRECTION('center_axis',(0.,1.,0.)) ;
#63268=DIRECTION('ref_axis',(1.,0.,0.)) ;
#63269=DIRECTION('',(0.,1.,0.)) ;
#63270=DIRECTION('',(0.,-1.,0.)) ;
#63271=DIRECTION('center_axis',(1.,0.,0.)) ;
#63272=DIRECTION('ref_axis',(0.,-1.,0.)) ;
#63273=DIRECTION('center_axis',(0.,0.,1.)) ;
#63274=DIRECTION('ref_axis',(0.707106781186559,-0.707106781186536,0.)) ;
#63275=DIRECTION('center_axis',(0.,0.,-1.)) ;
#63276=DIRECTION('ref_axis',(0.707106781186559,-0.707106781186536,0.)) ;
#63277=DIRECTION('center_axis',(-1.,4.3325776570738E-15,0.)) ;
#63278=DIRECTION('ref_axis',(-3.06359504133427E-15,-0.707106781186561,-0.707106781186534)) ;
#63279=DIRECTION('center_axis',(1.,0.,0.)) ;
#63280=DIRECTION('ref_axis',(0.,-1.,0.)) ;
#63281=DIRECTION('',(1.,-4.3325776570738E-15,0.)) ;
#63282=DIRECTION('',(-1.,4.3325776570738E-15,0.)) ;
#63283=DIRECTION('center_axis',(-4.3325776570738E-15,-1.,0.)) ;
#63284=DIRECTION('ref_axis',(0.,0.,-1.)) ;
#63285=DIRECTION('center_axis',(4.3325776570738E-15,1.,0.)) ;
#63286=DIRECTION('ref_axis',(-0.707106781186536,3.06359504133416E-15,0.707106781186559)) ;
#63287=DIRECTION('center_axis',(-4.3325776570738E-15,-1.,0.)) ;
#63288=DIRECTION('ref_axis',(-0.707106781186536,3.06359504133416E-15,0.707106781186559)) ;
#63289=DIRECTION('center_axis',(-4.3325776570738E-15,-1.,0.)) ;
#63290=DIRECTION('ref_axis',(1.,-4.3325776570738E-15,0.)) ;
#63291=DIRECTION('',(0.,0.,-1.)) ;
#63292=DIRECTION('',(-1.,4.3325776570738E-15,0.)) ;
#63293=DIRECTION('',(0.,0.,-1.)) ;
#63294=DIRECTION('center_axis',(0.,0.,1.)) ;
#63295=DIRECTION('ref_axis',(0.707106781186563,-0.707106781186532,0.)) ;
#63296=DIRECTION('',(0.,0.,1.)) ;
#63297=DIRECTION('center_axis',(0.,0.,-1.)) ;
#63298=DIRECTION('ref_axis',(0.707106781186563,-0.707106781186532,0.)) ;
#63299=DIRECTION('center_axis',(1.,0.,0.)) ;
#63300=DIRECTION('ref_axis',(0.,1.,0.)) ;
#63301=DIRECTION('',(0.,0.,-1.)) ;
#63302=DIRECTION('',(0.,1.,0.)) ;
#63303=DIRECTION('',(-0.693108716251782,-0.720833064901858,0.)) ;
#63304=DIRECTION('center_axis',(0.,1.,0.)) ;
#63305=DIRECTION('ref_axis',(0.99998238013875,0.,0.00593627930944729)) ;
#63306=DIRECTION('center_axis',(0.,0.,-1.)) ;
#63307=DIRECTION('ref_axis',(1.,0.,0.)) ;
#63308=DIRECTION('',(-1.,0.,0.)) ;
#63309=DIRECTION('center_axis',(0.,0.707106781186549,-0.707106781186546)) ;
#63310=DIRECTION('ref_axis',(-1.,0.,0.)) ;
#63311=DIRECTION('center_axis',(0.,0.707106781186549,-0.707106781186546)) ;
#63312=DIRECTION('ref_axis',(0.805613740871385,0.418919145253121,0.418919145253123)) ;
#63313=DIRECTION('',(0.562259334229024,0.584749707598188,0.58474970759819)) ;
#63314=DIRECTION('center_axis',(0.,0.707106781186549,-0.707106781186546)) ;
#63315=DIRECTION('ref_axis',(-0.569728896336401,-0.581123474263131,-0.581123474263133)) ;
#63316=DIRECTION('',(1.,0.,0.)) ;
#63317=DIRECTION('',(6.28036983473509E-16,-0.707106781186546,-0.707106781186549)) ;
#63318=DIRECTION('',(1.,0.,0.)) ;
#63319=DIRECTION('',(8.05175619837834E-16,-0.707106781186546,-0.707106781186549)) ;
#63320=DIRECTION('center_axis',(0.,-0.707106781186549,0.707106781186546)) ;
#63321=DIRECTION('ref_axis',(-8.17756488897798E-17,0.707106781186546,0.707106781186549)) ;
#63322=DIRECTION('',(-1.,0.,0.)) ;
#63323=DIRECTION('center_axis',(0.,0.707106781186549,-0.707106781186546)) ;
#63324=DIRECTION('ref_axis',(0.,-0.707106781186546,-0.707106781186549)) ;
#63325=DIRECTION('',(-1.,0.,0.)) ;
#63326=DIRECTION('center_axis',(0.,1.,0.)) ;
#63327=DIRECTION('ref_axis',(-1.,0.,0.)) ;
#63328=DIRECTION('center_axis',(-0.282166323991552,0.,-0.95936550157127)) ;
#63329=DIRECTION('ref_axis',(0.95936550157127,0.,-0.282166323991552)) ;
#63330=DIRECTION('center_axis',(-0.282166323991552,0.,-0.95936550157127)) ;
#63331=DIRECTION('ref_axis',(0.95936550157127,0.,-0.282166323991552)) ;
#63332=DIRECTION('center_axis',(0.959365501571273,0.,0.282166323991543)) ;
#63333=DIRECTION('ref_axis',(0.282166323991543,0.,-0.959365501571273)) ;
#63334=DIRECTION('center_axis',(0.959365501571273,0.,0.282166323991543)) ;
#63335=DIRECTION('ref_axis',(0.282166323991543,0.,-0.959365501571273)) ;
#63336=DIRECTION('center_axis',(0.,-1.,0.)) ;
#63337=DIRECTION('ref_axis',(-0.707106781186547,0.,0.707106781186547)) ;
#63338=DIRECTION('center_axis',(0.,1.,0.)) ;
#63339=DIRECTION('ref_axis',(-1.,0.,0.)) ;
#63340=DIRECTION('',(0.,-1.,0.)) ;
#63341=DIRECTION('',(0.,1.,0.)) ;
#63342=DIRECTION('center_axis',(-0.613629329650984,0.789594228570653,0.)) ;
#63343=DIRECTION('ref_axis',(-0.672991217643199,-0.523011864576266,0.523011864576303)) ;
#63344=DIRECTION('center_axis',(0.,0.,-1.)) ;
#63345=DIRECTION('ref_axis',(-2.27154580249389E-16,1.,0.)) ;
#63346=DIRECTION('center_axis',(7.1167068359955E-15,-0.274721127897369,
0.961523947640826)) ;
#63347=DIRECTION('ref_axis',(-6.67584762217264E-30,0.961523947640826,0.274721127897369)) ;
#63348=DIRECTION('center_axis',(0.,-0.707106781186546,-0.707106781186549)) ;
#63349=DIRECTION('ref_axis',(0.707106781186519,0.500000000000021,-0.500000000000019)) ;
#63350=DIRECTION('',(0.,-0.707106781186546,-0.707106781186549)) ;
#63351=DIRECTION('center_axis',(0.,0.707106781186529,0.707106781186566)) ;
#63352=DIRECTION('ref_axis',(1.,0.,0.)) ;
#63353=DIRECTION('',(0.,0.707106781186546,0.707106781186549)) ;
#63354=DIRECTION('center_axis',(-1.,0.,0.)) ;
#63355=DIRECTION('ref_axis',(0.,-1.,0.)) ;
#63356=DIRECTION('',(0.,0.,1.)) ;
#63357=DIRECTION('',(0.,-1.,0.)) ;
#63358=DIRECTION('center_axis',(-1.,0.,0.)) ;
#63359=DIRECTION('ref_axis',(0.,0.382683432365097,-0.923879532511284)) ;
#63360=DIRECTION('center_axis',(0.,0.,1.)) ;
#63361=DIRECTION('ref_axis',(0.707106781186359,-0.707106781186736,0.)) ;
#63362=DIRECTION('',(0.,0.,-1.)) ;
#63363=DIRECTION('center_axis',(0.,0.,-1.)) ;
#63364=DIRECTION('ref_axis',(1.,0.,0.)) ;
#63365=DIRECTION('center_axis',(0.,1.,0.)) ;
#63366=DIRECTION('ref_axis',(0.,0.,1.)) ;
#63367=DIRECTION('center_axis',(-0.959365501571273,0.,0.282166323991543)) ;
#63368=DIRECTION('ref_axis',(-0.282166323991543,0.,-0.959365501571273)) ;
#63369=DIRECTION('center_axis',(-0.959365501571273,0.,0.282166323991543)) ;
#63370=DIRECTION('ref_axis',(-0.282166323991543,0.,-0.959365501571273)) ;
#63371=DIRECTION('center_axis',(0.282166323991552,0.,-0.95936550157127)) ;
#63372=DIRECTION('ref_axis',(-0.95936550157127,0.,-0.282166323991552)) ;
#63373=DIRECTION('center_axis',(0.282166323991552,0.,-0.95936550157127)) ;
#63374=DIRECTION('ref_axis',(-0.95936550157127,0.,-0.282166323991552)) ;
#63375=DIRECTION('center_axis',(-8.88178419700125E-16,1.,0.)) ;
#63376=DIRECTION('ref_axis',(0.707106781186561,6.28036983473522E-16,0.707106781186534)) ;
#63377=DIRECTION('center_axis',(0.,1.,0.)) ;
#63378=DIRECTION('ref_axis',(0.,0.,1.)) ;
#63379=DIRECTION('',(8.88178419700125E-16,-1.,0.)) ;
#63380=DIRECTION('',(-8.88178419700125E-16,1.,0.)) ;
#63381=DIRECTION('center_axis',(0.613629329651134,0.789594228570536,0.)) ;
#63382=DIRECTION('ref_axis',(0.,0.,1.)) ;
#63383=DIRECTION('center_axis',(-7.1167068359954E-15,-0.27472112789737,
0.961523947640826)) ;
#63384=DIRECTION('ref_axis',(-1.90123672496938E-31,0.961523947640825,0.27472112789737)) ;
#63385=DIRECTION('center_axis',(0.,0.,-1.)) ;
#63386=DIRECTION('ref_axis',(-4.54309160498778E-16,1.,0.)) ;
#63387=DIRECTION('center_axis',(0.,0.,1.)) ;
#63388=DIRECTION('ref_axis',(1.,0.,0.)) ;
#63389=DIRECTION('',(-1.,0.,0.)) ;
#63390=DIRECTION('',(5.69345140833415E-16,1.,0.)) ;
#63391=DIRECTION('center_axis',(0.,0.,-1.)) ;
#63392=DIRECTION('ref_axis',(-0.70710678118657,-0.707106781186525,0.)) ;
#63393=DIRECTION('',(-1.,0.,0.)) ;
#63394=DIRECTION('center_axis',(0.,0.,-1.)) ;
#63395=DIRECTION('ref_axis',(0.707106781186503,-0.707106781186592,0.)) ;
#63396=DIRECTION('',(1.13869028166683E-15,-1.,0.)) ;
#63397=DIRECTION('',(-1.,0.,0.)) ;
#63398=DIRECTION('',(1.,-8.30329439001789E-15,0.)) ;
#63399=DIRECTION('',(-1.11022302462516E-14,1.,0.)) ;
#63400=DIRECTION('center_axis',(0.,0.,1.)) ;
#63401=DIRECTION('ref_axis',(0.,-1.,0.)) ;
#63402=DIRECTION('',(2.22044604925032E-15,-1.,0.)) ;
#63403=DIRECTION('',(1.,-8.30329439001789E-15,0.)) ;
#63404=DIRECTION('center_axis',(1.,-8.30329439001789E-15,0.)) ;
#63405=DIRECTION('ref_axis',(-5.87131576936922E-15,-0.707106781186469,-0.707106781186626)) ;
#63406=DIRECTION('',(-1.,8.30329439001789E-15,0.)) ;
#63407=DIRECTION('center_axis',(0.70710678118661,0.707106781186485,-6.28036983473565E-14)) ;
#63408=DIRECTION('ref_axis',(-0.707106781186485,0.70710678118661,-6.28036983473666E-14)) ;
#63409=DIRECTION('center_axis',(0.,0.,-1.)) ;
#63410=DIRECTION('ref_axis',(-0.707106781186359,-0.707106781186736,0.)) ;
#63411=DIRECTION('',(0.,0.,-1.)) ;
#63412=DIRECTION('center_axis',(0.,0.,-1.)) ;
#63413=DIRECTION('ref_axis',(-8.88178419700617E-14,-1.,0.)) ;
#63414=DIRECTION('',(0.,0.,1.)) ;
#63415=DIRECTION('center_axis',(-0.50387102552408,0.,0.863778900898437)) ;
#63416=DIRECTION('ref_axis',(0.863778900898437,0.,0.50387102552408)) ;
#63417=DIRECTION('center_axis',(0.86377890089843,0.,-0.503871025524092)) ;
#63418=DIRECTION('ref_axis',(0.503871025524092,0.,0.86377890089843)) ;
#63419=DIRECTION('center_axis',(-7.10542735760115E-13,1.,-3.55271367880042E-13)) ;
#63420=DIRECTION('ref_axis',(7.17464813746296E-42,3.55271367880042E-13,
1.)) ;
#63421=DIRECTION('center_axis',(1.,0.,-7.16300942304673E-47)) ;
#63422=DIRECTION('ref_axis',(5.06501253673939E-47,0.707106781186561,0.707106781186534)) ;
#63423=DIRECTION('',(-1.,0.,7.16300942304673E-47)) ;
#63424=DIRECTION('center_axis',(1.,3.17373410623533E-15,0.)) ;
#63425=DIRECTION('ref_axis',(-2.24416890820207E-15,0.707106781186561,0.707106781186534)) ;
#63426=DIRECTION('',(1.,0.,-7.16300942304673E-47)) ;
#63427=DIRECTION('center_axis',(0.,0.,-1.)) ;
#63428=DIRECTION('ref_axis',(0.707106781186521,0.707106781186574,0.)) ;
#63429=DIRECTION('',(0.,0.,-1.)) ;
#63430=DIRECTION('',(0.,0.,1.)) ;
#63431=DIRECTION('center_axis',(-2.46519032881529E-32,1.65309428213318E-45,
1.)) ;
#63432=DIRECTION('ref_axis',(0.707106781186521,0.707106781186574,1.7431527984206E-32)) ;
#63433=DIRECTION('',(0.,0.,1.)) ;
#63434=DIRECTION('center_axis',(-1.,-3.17373410623533E-15,0.)) ;
#63435=DIRECTION('ref_axis',(-3.17373410623533E-15,1.,0.)) ;
#63436=DIRECTION('',(0.,0.,-1.)) ;
#63437=DIRECTION('',(-3.17373410623533E-15,1.,0.)) ;
#63438=DIRECTION('',(0.,0.,-1.)) ;
#63439=DIRECTION('',(-3.17373410623533E-15,1.,0.)) ;
#63440=DIRECTION('center_axis',(-1.,-3.17373410623533E-15,0.)) ;
#63441=DIRECTION('ref_axis',(-3.17373410623533E-15,1.,6.13317366673399E-17)) ;
#63442=DIRECTION('',(0.,0.,-1.)) ;
#63443=DIRECTION('center_axis',(1.,3.17373410623533E-15,0.)) ;
#63444=DIRECTION('ref_axis',(3.17373410623533E-15,-1.,-6.13317366673399E-17)) ;
#63445=DIRECTION('',(3.17373410623533E-15,-1.,0.)) ;
#63446=DIRECTION('center_axis',(0.,1.,0.)) ;
#63447=DIRECTION('ref_axis',(1.,0.,0.)) ;
#63448=DIRECTION('',(1.,0.,0.)) ;
#63449=DIRECTION('center_axis',(2.46519032881529E-32,-1.65309428213318E-45,
-1.)) ;
#63450=DIRECTION('ref_axis',(1.,3.08616105302236E-93,2.46519032881529E-32)) ;
#63451=DIRECTION('center_axis',(-2.46519032881529E-32,1.65309428213318E-45,
1.)) ;
#63452=DIRECTION('ref_axis',(0.447213595500276,0.894427190999757,1.10246663054185E-32)) ;
#63453=DIRECTION('',(0.800000000000003,0.599999999999996,1.97215226305214E-32)) ;
#63454=DIRECTION('center_axis',(0.,0.,-1.)) ;
#63455=DIRECTION('ref_axis',(0.447213595500276,0.894427190999757,0.)) ;
#63456=DIRECTION('center_axis',(0.,0.,1.)) ;
#63457=DIRECTION('ref_axis',(1.,0.,0.)) ;
#63458=DIRECTION('',(0.,0.,1.)) ;
#63459=DIRECTION('center_axis',(-1.1460366705808E-14,1.,0.)) ;
#63460=DIRECTION('ref_axis',(0.707106781186534,8.10370301256122E-15,0.707106781186561)) ;
#63461=DIRECTION('',(-1.1460366705808E-14,1.,0.)) ;
#63462=DIRECTION('center_axis',(-0.707106781186548,-0.707106781186548,0.)) ;
#63463=DIRECTION('ref_axis',(0.707106781186547,-0.707106781186547,0.)) ;
#63464=DIRECTION('',(1.1460366705808E-14,-1.,0.)) ;
#63465=DIRECTION('center_axis',(0.,0.,-1.)) ;
#63466=DIRECTION('ref_axis',(1.,0.,0.)) ;
#63467=DIRECTION('',(-0.707106781186547,0.707106781186547,0.)) ;
#63468=DIRECTION('center_axis',(0.693108716251755,0.720833064901884,-3.6936252256852E-13)) ;
#63469=DIRECTION('ref_axis',(-0.720833064901884,0.693108716251755,2.48164876568418E-29)) ;
#63470=DIRECTION('center_axis',(0.170786723535891,-0.985308020399649,0.)) ;
#63471=DIRECTION('ref_axis',(-0.985308020399649,-0.170786723535891,0.)) ;
#63472=DIRECTION('center_axis',(2.22044604925026E-13,2.30926389122032E-13,
-1.)) ;
#63473=DIRECTION('ref_axis',(-1.,1.34524652575477E-42,-2.22044604925026E-13)) ;
#63474=DIRECTION('center_axis',(-0.720833064901858,0.693108716251782,0.)) ;
#63475=DIRECTION('ref_axis',(-0.693108716251782,-0.720833064901858,2.25440992778648E-16)) ;
#63476=DIRECTION('center_axis',(5.73018335290399E-15,-1.,0.)) ;
#63477=DIRECTION('ref_axis',(-0.707106781186534,-4.0518515062806E-15,0.707106781186561)) ;
#63478=DIRECTION('',(-5.73018335290399E-15,1.,0.)) ;
#63479=DIRECTION('',(5.73018335290399E-15,-1.,0.)) ;
#63480=DIRECTION('center_axis',(0.720833064901858,-0.693108716251782,0.)) ;
#63481=DIRECTION('ref_axis',(0.,0.,-1.)) ;
#63482=DIRECTION('',(0.,0.,1.)) ;
#63483=DIRECTION('center_axis',(0.720833064901858,-0.693108716251782,0.)) ;
#63484=DIRECTION('ref_axis',(0.693108716251782,0.720833064901858,9.01763971114601E-17)) ;
#63485=DIRECTION('',(-0.562259334229024,-0.584749707598188,-0.58474970759819)) ;
#63486=DIRECTION('',(0.693108716251782,0.720833064901858,0.)) ;
#63487=DIRECTION('center_axis',(0.,0.,1.)) ;
#63488=DIRECTION('ref_axis',(-0.927586401609545,0.373608709145084,0.)) ;
#63489=DIRECTION('',(0.,0.,-1.)) ;
#63490=DIRECTION('center_axis',(0.,0.,-1.)) ;
#63491=DIRECTION('ref_axis',(-1.,0.,0.)) ;
#63492=DIRECTION('center_axis',(-1.,-5.73018335290399E-15,0.)) ;
#63493=DIRECTION('ref_axis',(-5.73018335290399E-15,1.,0.)) ;
#63494=DIRECTION('',(-5.73018335290399E-15,1.,0.)) ;
#63495=DIRECTION('',(0.,0.,1.)) ;
#63496=DIRECTION('',(5.73018335290399E-15,-1.,0.)) ;
#63497=DIRECTION('',(0.,0.,1.)) ;
#63498=DIRECTION('',(5.73018335290399E-15,-1.,1.11561779098947E-30)) ;
#63499=DIRECTION('center_axis',(-1.,5.69345140833415E-16,0.)) ;
#63500=DIRECTION('ref_axis',(0.,0.,1.)) ;
#63501=DIRECTION('center_axis',(0.,1.,0.)) ;
#63502=DIRECTION('ref_axis',(1.,0.,0.)) ;
#63503=DIRECTION('center_axis',(1.,-5.69345140833415E-16,0.)) ;
#63504=DIRECTION('ref_axis',(2.17878952694528E-16,0.382683432365109,-0.923879532511279)) ;
#63505=DIRECTION('center_axis',(4.71027737605141E-14,-0.707106781186581,
-0.707106781186514)) ;
#63506=DIRECTION('ref_axis',(-7.31444512085447E-31,0.707106781186514,-0.707106781186581)) ;
#63507=DIRECTION('center_axis',(-1.,5.69345140833415E-16,0.)) ;
#63508=DIRECTION('ref_axis',(2.17878952694528E-16,0.382683432365109,-0.923879532511279)) ;
#63509=DIRECTION('center_axis',(-1.,0.,0.)) ;
#63510=DIRECTION('ref_axis',(0.,0.382683432365076,-0.923879532511292)) ;
#63511=DIRECTION('',(1.,0.,0.)) ;
#63512=DIRECTION('center_axis',(-4.02587809918917E-16,-0.707106781186546,
-0.707106781186549)) ;
#63513=DIRECTION('ref_axis',(0.707106781186625,0.499999999999946,-0.499999999999944)) ;
#63514=DIRECTION('',(4.02587809918917E-16,0.707106781186546,0.707106781186549)) ;
#63515=DIRECTION('center_axis',(0.,0.70710678118657,0.707106781186525)) ;
#63516=DIRECTION('ref_axis',(1.,0.,0.)) ;
#63517=DIRECTION('',(-4.02587809918917E-16,-0.707106781186546,-0.707106781186549)) ;
#63518=DIRECTION('center_axis',(0.,0.707106781186549,-0.707106781186546)) ;
#63519=DIRECTION('ref_axis',(-1.,0.,0.)) ;
#63520=DIRECTION('',(1.,0.,0.)) ;
#63521=DIRECTION('',(8.82074414990881E-16,-0.707106781186546,-0.707106781186549)) ;
#63522=DIRECTION('',(-1.,0.,0.)) ;
#63523=DIRECTION('center_axis',(0.,-0.707106781186549,0.707106781186546)) ;
#63524=DIRECTION('ref_axis',(8.17756488897798E-17,0.707106781186546,0.707106781186549)) ;
#63525=DIRECTION('center_axis',(-1.,-1.13869028166683E-15,0.)) ;
#63526=DIRECTION('ref_axis',(0.,0.,1.)) ;
#63527=DIRECTION('center_axis',(0.,1.,0.)) ;
#63528=DIRECTION('ref_axis',(0.,0.,-1.)) ;
#63529=DIRECTION('center_axis',(1.,1.13869028166683E-15,0.)) ;
#63530=DIRECTION('ref_axis',(-4.35757905389055E-16,0.382683432365109,-0.923879532511279)) ;
#63531=DIRECTION('center_axis',(-4.7102773760512E-14,-0.707106781186581,
-0.707106781186514)) ;
#63532=DIRECTION('ref_axis',(-1.,-1.7276484112332E-29,6.66133814775108E-14)) ;
#63533=DIRECTION('center_axis',(-1.,-1.13869028166683E-15,0.)) ;
#63534=DIRECTION('ref_axis',(-4.35757905389055E-16,0.382683432365109,-0.923879532511279)) ;
#63535=DIRECTION('center_axis',(-1.,0.,0.)) ;
#63536=DIRECTION('ref_axis',(0.,0.382683432365076,-0.923879532511292)) ;
#63537=DIRECTION('center_axis',(1.13869028166683E-15,-1.,0.)) ;
#63538=DIRECTION('ref_axis',(-0.707106781186532,-8.05175619837817E-16,-0.707106781186563)) ;
#63539=DIRECTION('center_axis',(0.,1.,0.)) ;
#63540=DIRECTION('ref_axis',(0.,0.,-1.)) ;
#63541=DIRECTION('',(-1.13869028166683E-15,1.,0.)) ;
#63542=DIRECTION('center_axis',(-8.30329439001789E-15,-1.,0.)) ;
#63543=DIRECTION('ref_axis',(0.,0.,-1.)) ;
#63544=DIRECTION('center_axis',(8.30329439001789E-15,1.,0.)) ;
#63545=DIRECTION('ref_axis',(0.707106781186555,-5.87131576936993E-15,-0.70710678118654)) ;
#63546=DIRECTION('center_axis',(1.,0.,0.)) ;
#63547=DIRECTION('ref_axis',(0.,-1.,0.)) ;
#63548=DIRECTION('center_axis',(-8.30329439001789E-15,-1.,0.)) ;
#63549=DIRECTION('ref_axis',(0.707106781186555,-5.87131576936993E-15,-0.70710678118654)) ;
#63550=DIRECTION('center_axis',(-1.,0.,0.)) ;
#63551=DIRECTION('ref_axis',(0.,0.,1.)) ;
#63552=DIRECTION('center_axis',(0.,1.,0.)) ;
#63553=DIRECTION('ref_axis',(1.,0.,0.)) ;
#63554=DIRECTION('center_axis',(1.,0.,0.)) ;
#63555=DIRECTION('ref_axis',(0.,0.382683432365097,-0.923879532511284)) ;
#63556=DIRECTION('center_axis',(0.,-1.,0.)) ;
#63557=DIRECTION('ref_axis',(0.707106781186547,0.,-0.707106781186547)) ;
#63558=DIRECTION('',(0.,1.,0.)) ;
#63559=DIRECTION('center_axis',(8.30329439001789E-15,1.,0.)) ;
#63560=DIRECTION('ref_axis',(0.,0.,1.)) ;
#63561=DIRECTION('center_axis',(-8.30329439001789E-15,-1.,0.)) ;
#63562=DIRECTION('ref_axis',(-0.707106781186571,5.87131576937006E-15,-0.707106781186524)) ;
#63563=DIRECTION('center_axis',(-1.,0.,0.)) ;
#63564=DIRECTION('ref_axis',(0.,0.,-1.)) ;
#63565=DIRECTION('center_axis',(8.30329439001789E-15,1.,0.)) ;
#63566=DIRECTION('ref_axis',(-0.707106781186571,5.87131576937006E-15,-0.707106781186524)) ;
#63567=DIRECTION('center_axis',(-8.88178419700125E-16,1.,0.)) ;
#63568=DIRECTION('ref_axis',(-0.707106781186537,-6.28036983473501E-16,-0.707106781186558)) ;
#63569=DIRECTION('center_axis',(0.,-1.,0.)) ;
#63570=DIRECTION('ref_axis',(-1.,0.,0.)) ;
#63571=DIRECTION('',(8.88178419700125E-16,-1.,0.)) ;
#63572=DIRECTION('',(-8.88178419700125E-16,1.,0.)) ;
#63573=DIRECTION('center_axis',(1.,8.88178419700125E-16,0.)) ;
#63574=DIRECTION('ref_axis',(0.,0.,-1.)) ;
#63575=DIRECTION('center_axis',(0.,-0.707106781186536,-0.707106781186559)) ;
#63576=DIRECTION('ref_axis',(-1.,0.,0.)) ;
#63577=DIRECTION('center_axis',(-1.,-8.88178419700125E-16,0.)) ;
#63578=DIRECTION('ref_axis',(-3.39891166203452E-16,0.382683432365097,-0.923879532511284)) ;
#63579=DIRECTION('center_axis',(1.,8.88178419700125E-16,0.)) ;
#63580=DIRECTION('ref_axis',(-3.39891166203451E-16,0.382683432365097,-0.923879532511284)) ;
#63581=DIRECTION('center_axis',(-6.28036983473509E-16,0.707106781186546,
0.707106781186549)) ;
#63582=DIRECTION('ref_axis',(-0.707106781186505,0.500000000000031,-0.500000000000029)) ;
#63583=DIRECTION('',(-6.28036983473509E-16,0.707106781186546,0.707106781186549)) ;
#63584=DIRECTION('center_axis',(-8.30329439001789E-15,-1.,0.)) ;
#63585=DIRECTION('ref_axis',(-1.,8.30329439001789E-15,4.19778536698447E-50)) ;
#63586=DIRECTION('',(-1.,8.30329439001789E-15,0.)) ;
#63587=DIRECTION('',(0.,0.,-1.)) ;
#63588=DIRECTION('',(-1.,8.30329439001789E-15,4.19778536698447E-50)) ;
#63589=DIRECTION('',(0.,0.,-1.)) ;
#63590=DIRECTION('',(1.,-9.87859509815899E-15,0.)) ;
#63591=DIRECTION('',(0.,0.,-1.)) ;
#63592=DIRECTION('center_axis',(-1.,8.30329439001789E-15,0.)) ;
#63593=DIRECTION('ref_axis',(-5.87131576936922E-15,-0.707106781186469,-0.707106781186626)) ;
#63594=DIRECTION('',(1.,-8.30329439001789E-15,0.)) ;
#63595=DIRECTION('center_axis',(1.,0.,0.)) ;
#63596=DIRECTION('ref_axis',(0.,-1.,0.)) ;
#63597=DIRECTION('center_axis',(0.,0.,-1.)) ;
#63598=DIRECTION('ref_axis',(1.,0.,0.)) ;
#63599=DIRECTION('',(-1.,0.,0.)) ;
#63600=DIRECTION('center_axis',(0.,0.,-1.)) ;
#63601=DIRECTION('ref_axis',(0.998370060467465,-0.0570720804088061,0.)) ;
#63602=DIRECTION('',(-5.73018335290399E-15,1.,0.)) ;
#63603=DIRECTION('',(1.,-4.33257765707378E-15,0.)) ;
#63604=DIRECTION('',(9.79313055424617E-16,-1.,0.)) ;
#63605=DIRECTION('center_axis',(0.,0.,-1.)) ;
#63606=DIRECTION('ref_axis',(0.707106781186554,0.707106781186541,0.)) ;
#63607=DIRECTION('center_axis',(-1.,0.,0.)) ;
#63608=DIRECTION('ref_axis',(0.,0.382683432365084,-0.923879532511289)) ;
#63609=DIRECTION('center_axis',(-0.81649658092775,0.408248290463875,0.408248290463804)) ;
#63610=DIRECTION('ref_axis',(0.577350269189602,0.577350269189744,0.577350269189531)) ;
#63611=DIRECTION('center_axis',(0.,0.,1.)) ;
#63612=DIRECTION('ref_axis',(0.,1.,0.)) ;
#63613=DIRECTION('center_axis',(1.,0.,0.)) ;
#63614=DIRECTION('ref_axis',(0.,0.,1.)) ;
#63615=DIRECTION('center_axis',(0.,1.,0.)) ;
#63616=DIRECTION('ref_axis',(1.,0.,0.)) ;
#63617=DIRECTION('center_axis',(1.,0.,2.46519032881572E-32)) ;
#63618=DIRECTION('ref_axis',(-1.74315279842063E-32,0.707106781186736,0.707106781186359)) ;
#63619=DIRECTION('center_axis',(0.70710678118661,0.707106781186485,0.)) ;
#63620=DIRECTION('ref_axis',(-0.707106781186485,0.70710678118661,6.13317366673404E-17)) ;
#63621=DIRECTION('',(1.,0.,2.46519032881572E-32)) ;
#63622=DIRECTION('',(-1.,0.,-2.46519032881572E-32)) ;
#63623=DIRECTION('center_axis',(2.46519032881572E-32,8.55284707229503E-50,
-1.)) ;
#63624=DIRECTION('ref_axis',(-1.,0.,0.)) ;
#63625=DIRECTION('center_axis',(2.46519032881572E-32,8.55284707229503E-50,
-1.)) ;
#63626=DIRECTION('ref_axis',(-0.339202113889148,0.940713519586666,-8.36197770673376E-33)) ;
#63627=DIRECTION('center_axis',(-1.,0.,0.)) ;
#63628=DIRECTION('ref_axis',(0.,-1.,0.)) ;
#63629=DIRECTION('center_axis',(-2.46519032881572E-32,-8.55284707229503E-50,
1.)) ;
#63630=DIRECTION('ref_axis',(-0.339202113889148,0.940713519586666,-8.36197770673376E-33)) ;
#63631=DIRECTION('center_axis',(-1.,3.55271367880048E-14,-2.46519032881572E-32)) ;
#63632=DIRECTION('ref_axis',(-2.51214793389469E-14,-0.707106781186736,0.707106781186359)) ;
#63633=DIRECTION('center_axis',(-1.,0.,0.)) ;
#63634=DIRECTION('ref_axis',(0.,-1.,0.)) ;
#63635=DIRECTION('',(-1.,3.55271367880048E-14,-2.46519032881572E-32)) ;
#63636=DIRECTION('',(1.,-3.55271367880048E-14,2.46519032881572E-32)) ;
#63637=DIRECTION('center_axis',(2.46519032881572E-32,8.55284707229503E-50,
-1.)) ;
#63638=DIRECTION('ref_axis',(-1.,0.,0.)) ;
#63639=DIRECTION('center_axis',(-0.624999999999801,-0.780624749799959,0.)) ;
#63640=DIRECTION('ref_axis',(0.780624749799959,-0.624999999999801,0.)) ;
#63641=DIRECTION('center_axis',(2.46519032881572E-32,8.55284707229503E-50,
-1.)) ;
#63642=DIRECTION('ref_axis',(0.433012701892204,-0.901387818866005,1.06745872495903E-32)) ;
#63643=DIRECTION('center_axis',(-2.46519032881572E-32,-8.55284707229503E-50,
1.)) ;
#63644=DIRECTION('ref_axis',(0.433012701892204,-0.901387818866005,1.06745872495903E-32)) ;
#63645=DIRECTION('center_axis',(2.46519032881572E-32,8.55284707229503E-50,
-1.)) ;
#63646=DIRECTION('ref_axis',(-1.,0.,0.)) ;
#63647=DIRECTION('center_axis',(-0.707106781186459,-0.707106781186636,0.)) ;
#63648=DIRECTION('ref_axis',(0.707106781186636,-0.707106781186459,0.)) ;
#63649=DIRECTION('center_axis',(-2.46519032881572E-32,-8.55284707229503E-50,
1.)) ;
#63650=DIRECTION('ref_axis',(-0.744997757011397,0.667066969687443,-1.8365612655739E-32)) ;
#63651=DIRECTION('center_axis',(2.46519032881572E-32,8.55284707229503E-50,
-1.)) ;
#63652=DIRECTION('ref_axis',(-0.744997757011397,0.667066969687443,-1.8365612655739E-32)) ;
#63653=DIRECTION('center_axis',(0.70710678118654,0.707106781186555,1.74315279842107E-32)) ;
#63654=DIRECTION('ref_axis',(0.499999999999972,-0.499999999999962,0.707106781186594)) ;
#63655=DIRECTION('center_axis',(-0.707106781186548,-0.707106781186548,0.)) ;
#63656=DIRECTION('ref_axis',(0.707106781186547,-0.707106781186547,0.)) ;
#63657=DIRECTION('',(-0.70710678118654,-0.707106781186555,-1.74315279842107E-32)) ;
#63658=DIRECTION('',(0.70710678118654,0.707106781186555,1.74315279842107E-32)) ;
#63659=DIRECTION('center_axis',(2.46519032881572E-32,8.55284707229503E-50,
-1.)) ;
#63660=DIRECTION('ref_axis',(-1.,0.,0.)) ;
#63661=DIRECTION('center_axis',(0.,-1.,0.)) ;
#63662=DIRECTION('ref_axis',(1.,0.,0.)) ;
#63663=DIRECTION('center_axis',(2.46519032881572E-32,8.55284707229503E-50,
-1.)) ;
#63664=DIRECTION('ref_axis',(0.923879532511298,-0.382683432365064,2.27753888853764E-32)) ;
#63665=DIRECTION('center_axis',(-2.46519032881572E-32,-8.55284707229503E-50,
1.)) ;
#63666=DIRECTION('ref_axis',(0.923879532511297,-0.382683432365064,2.27753888853764E-32)) ;
#63667=DIRECTION('center_axis',(0.,1.,8.55284707229503E-50)) ;
#63668=DIRECTION('ref_axis',(0.707106781186485,-6.04777616327186E-50,0.70710678118661)) ;
#63669=DIRECTION('',(0.,-1.,-8.55284707229503E-50)) ;
#63670=DIRECTION('',(0.,1.,8.55284707229503E-50)) ;
#63671=DIRECTION('center_axis',(0.,0.,-1.)) ;
#63672=DIRECTION('ref_axis',(0.707106781186296,0.707106781186799,0.)) ;
#63673=DIRECTION('center_axis',(0.,0.,1.)) ;
#63674=DIRECTION('ref_axis',(1.,0.,0.)) ;
#63675=DIRECTION('',(0.,0.,1.)) ;
#63676=DIRECTION('',(0.,0.,-1.)) ;
#63677=DIRECTION('center_axis',(0.,1.,0.)) ;
#63678=DIRECTION('ref_axis',(0.,0.,1.)) ;
#63679=DIRECTION('center_axis',(0.,1.,0.)) ;
#63680=DIRECTION('ref_axis',(-0.707106781186481,0.,-0.707106781186614)) ;
#63681=DIRECTION('center_axis',(0.,-1.,0.)) ;
#63682=DIRECTION('ref_axis',(-0.707106781186481,0.,-0.707106781186614)) ;
#63683=DIRECTION('center_axis',(2.46519032881572E-32,8.55284707229503E-50,
-1.)) ;
#63684=DIRECTION('ref_axis',(1.,-2.20382687031672E-110,2.46519032881572E-32)) ;
#63685=DIRECTION('',(0.,1.,8.55284707229503E-50)) ;
#63686=DIRECTION('center_axis',(2.46519032881566E-32,0.,-1.)) ;
#63687=DIRECTION('ref_axis',(0.,1.,0.)) ;
#63688=DIRECTION('',(1.77635683939373E-14,1.,-2.46519032880661E-33)) ;
#63689=DIRECTION('center_axis',(2.46519032881572E-32,8.55284707229503E-50,
-1.)) ;
#63690=DIRECTION('ref_axis',(1.,-2.20382687031672E-110,2.46519032881572E-32)) ;
#63691=DIRECTION('',(1.,0.,6.12949496482233E-35)) ;
#63692=DIRECTION('',(0.,1.,0.)) ;
#63693=DIRECTION('',(-1.,3.55271367880048E-14,0.)) ;
#63694=DIRECTION('center_axis',(0.,0.,-1.)) ;
#63695=DIRECTION('ref_axis',(-1.,3.9474596431117E-14,0.)) ;
#63696=DIRECTION('center_axis',(2.46519032881572E-32,8.55284707229503E-50,
-1.)) ;
#63697=DIRECTION('ref_axis',(-1.,2.10843958864616E-81,-2.46519032881572E-32)) ;
#63698=DIRECTION('center_axis',(2.46519032881572E-32,8.55284707229503E-50,
-1.)) ;
#63699=DIRECTION('ref_axis',(-0.498769364572801,-0.86673474659993,-1.22956141385443E-32)) ;
#63700=DIRECTION('center_axis',(0.,1.,8.55284707229503E-50)) ;
#63701=DIRECTION('ref_axis',(-0.707106781186485,-6.04777616327186E-50,0.70710678118661)) ;
#63702=DIRECTION('',(0.,-1.,-8.55284707229503E-50)) ;
#63703=DIRECTION('center_axis',(0.,1.,0.)) ;
#63704=DIRECTION('ref_axis',(-0.707106781186485,0.,0.70710678118661)) ;
#63705=DIRECTION('center_axis',(0.,1.,0.)) ;
#63706=DIRECTION('ref_axis',(1.,0.,1.30736459881558E-32)) ;
#63707=DIRECTION('',(1.,0.,0.)) ;
#63708=DIRECTION('',(0.,0.,-1.)) ;
#63709=DIRECTION('center_axis',(0.,0.,-1.)) ;
#63710=DIRECTION('ref_axis',(0.480391553143902,-0.877054134970008,0.)) ;
#63711=DIRECTION('center_axis',(0.,0.,1.)) ;
#63712=DIRECTION('ref_axis',(0.480391553143902,-0.877054134970008,0.)) ;
#63713=DIRECTION('',(0.,0.,1.)) ;
#63714=DIRECTION('center_axis',(0.,0.,1.)) ;
#63715=DIRECTION('ref_axis',(-0.538447911335745,-0.842658796179197,0.)) ;
#63716=DIRECTION('',(0.,0.,-1.)) ;
#63717=DIRECTION('center_axis',(0.,-0.70710678118661,0.707106781186485)) ;
#63718=DIRECTION('ref_axis',(-6.13317366673295E-17,-0.707106781186485,-0.70710678118661)) ;
#63719=DIRECTION('center_axis',(0.,0.,-1.)) ;
#63720=DIRECTION('ref_axis',(8.28966525053379E-14,1.,0.)) ;
#63721=DIRECTION('center_axis',(0.,0.,-1.)) ;
#63722=DIRECTION('ref_axis',(8.28966525053379E-14,1.,0.)) ;
#63723=DIRECTION('',(0.,0.,-1.)) ;
#63724=DIRECTION('center_axis',(-1.01307418018711E-45,-5.52427741944263E-33,
-1.)) ;
#63725=DIRECTION('ref_axis',(8.28966525053379E-14,1.,-5.52427741944263E-33)) ;
#63726=DIRECTION('center_axis',(0.,1.,0.)) ;
#63727=DIRECTION('ref_axis',(-0.707106781186485,0.,-0.70710678118661)) ;
#63728=DIRECTION('',(0.,-1.,0.)) ;
#63729=DIRECTION('center_axis',(0.,-1.,0.)) ;
#63730=DIRECTION('ref_axis',(-1.,0.,0.)) ;
#63731=DIRECTION('',(0.,1.,0.)) ;
#63732=DIRECTION('center_axis',(1.,0.,0.)) ;
#63733=DIRECTION('ref_axis',(0.,-1.,0.)) ;
#63734=DIRECTION('',(0.,0.,-1.)) ;
#63735=DIRECTION('',(0.,-1.,0.)) ;
#63736=DIRECTION('',(0.,0.,-1.)) ;
#63737=DIRECTION('center_axis',(1.,9.79313055424617E-16,0.)) ;
#63738=DIRECTION('ref_axis',(0.,0.,-1.)) ;
#63739=DIRECTION('center_axis',(-1.,-9.79313055424617E-16,0.)) ;
#63740=DIRECTION('ref_axis',(3.43729761245549E-16,-0.3509906861157,0.936378950137192)) ;
#63741=DIRECTION('center_axis',(0.,1.,0.)) ;
#63742=DIRECTION('ref_axis',(0.,0.,-1.)) ;
#63743=DIRECTION('center_axis',(1.,9.79313055424617E-16,0.)) ;
#63744=DIRECTION('ref_axis',(3.43729761245549E-16,-0.3509906861157,0.936378950137192)) ;
#63745=DIRECTION('center_axis',(0.,-0.753611076520055,-0.65732058034591)) ;
#63746=DIRECTION('ref_axis',(-1.,0.,0.)) ;
#63747=DIRECTION('center_axis',(-9.79313055424617E-16,1.,0.)) ;
#63748=DIRECTION('ref_axis',(-0.707106781186532,-6.92478902395249E-16,-0.707106781186563)) ;
#63749=DIRECTION('center_axis',(0.,-1.,0.)) ;
#63750=DIRECTION('ref_axis',(-1.,0.,0.)) ;
#63751=DIRECTION('',(-9.79313055424617E-16,1.,0.)) ;
#63752=DIRECTION('center_axis',(0.,0.,1.)) ;
#63753=DIRECTION('ref_axis',(1.,0.,0.)) ;
#63754=DIRECTION('center_axis',(0.,0.,1.)) ;
#63755=DIRECTION('ref_axis',(0.707106781186554,0.707106781186541,0.)) ;
#63756=DIRECTION('center_axis',(-1.,4.33257765707378E-15,0.)) ;
#63757=DIRECTION('ref_axis',(-1.52069440450512E-15,-0.350990686115526,0.936378950137257)) ;
#63758=DIRECTION('center_axis',(1.,0.,0.)) ;
#63759=DIRECTION('ref_axis',(0.,0.,1.)) ;
#63760=DIRECTION('',(-1.,4.33257765707378E-15,0.)) ;
#63761=DIRECTION('center_axis',(0.604947702565294,0.517761097730612,0.60494770256425)) ;
#63762=DIRECTION('ref_axis',(-0.707106781185937,-2.45097362971974E-16,0.707106781187158)) ;
#63763=DIRECTION('center_axis',(0.707106781186503,-9.42055475210098E-14,
0.707106781186592)) ;
#63764=DIRECTION('ref_axis',(-0.707106781186592,-8.04690672217442E-31,0.707106781186503)) ;
#63765=DIRECTION('center_axis',(-0.661621637086846,-8.8798640187934E-15,
0.749837855365093)) ;
#63766=DIRECTION('ref_axis',(-0.749837855365093,-5.16196667825131E-32,-0.661621637086846)) ;
#63767=DIRECTION('center_axis',(0.707106781186548,4.05185150628068E-15,
-0.707106781186548)) ;
#63768=DIRECTION('ref_axis',(-0.707106781186548,1.02171457789349E-14,-0.707106781186548)) ;
#63769=DIRECTION('center_axis',(-0.707106781186548,3.06359504133419E-15,
-0.707106781186548)) ;
#63770=DIRECTION('ref_axis',(-0.499999999999867,-0.707106781186738,0.499999999999864)) ;
#63771=DIRECTION('center_axis',(0.707106781186525,0.,0.70710678118657)) ;
#63772=DIRECTION('ref_axis',(-0.70710678118657,0.,0.707106781186525)) ;
#63773=DIRECTION('',(-0.707106781186547,3.06359504133419E-15,-0.707106781186547)) ;
#63774=DIRECTION('',(0.707106781186547,-3.06359504133419E-15,0.707106781186547)) ;
#63775=DIRECTION('center_axis',(-0.89442719099992,0.,0.44721359549995)) ;
#63776=DIRECTION('ref_axis',(0.44721359549995,0.,0.89442719099992)) ;
#63777=DIRECTION('center_axis',(0.707106781186548,4.05185150628068E-15,
-0.707106781186548)) ;
#63778=DIRECTION('ref_axis',(0.707106781186548,3.92523114670944E-15,0.707106781186548)) ;
#63779=DIRECTION('center_axis',(0.,0.,-1.)) ;
#63780=DIRECTION('ref_axis',(-1.,0.,0.)) ;
#63781=DIRECTION('center_axis',(-0.983423055146244,0.181325534454923,0.000381000609942105)) ;
#63782=DIRECTION('ref_axis',(0.181316738273391,0.983349845304303,0.0121376341146972)) ;
#63783=DIRECTION('center_axis',(0.,0.,-1.)) ;
#63784=DIRECTION('ref_axis',(-0.624947614806638,-0.780666688637022,0.)) ;
#63785=DIRECTION('center_axis',(0.573576436350949,-0.81915204428906,0.)) ;
#63786=DIRECTION('ref_axis',(-0.81915204428906,-0.573576436350949,0.)) ;
#63787=DIRECTION('center_axis',(-0.573576436351043,0.819152044288994,0.)) ;
#63788=DIRECTION('ref_axis',(-0.579227965339645,-0.405579787672689,-0.707106781186457)) ;
#63789=DIRECTION('center_axis',(0.573576436351158,-0.819152044288914,0.)) ;
#63790=DIRECTION('ref_axis',(-0.819152044288914,-0.573576436351158,0.)) ;
#63791=DIRECTION('',(-0.573576436351043,0.819152044288994,0.)) ;
#63792=DIRECTION('center_axis',(0.,0.,-1.)) ;
#63793=DIRECTION('ref_axis',(-1.,0.,0.)) ;
#63794=DIRECTION('center_axis',(0.,-1.,0.)) ;
#63795=DIRECTION('ref_axis',(-1.,0.,0.)) ;
#63796=DIRECTION('center_axis',(0.,0.,-1.)) ;
#63797=DIRECTION('ref_axis',(-0.95371695074823,-0.300705799504264,0.)) ;
#63798=DIRECTION('center_axis',(-9.79313055424617E-16,1.,0.)) ;
#63799=DIRECTION('ref_axis',(-0.707106781186532,-6.92478902395249E-16,-0.707106781186563)) ;
#63800=DIRECTION('center_axis',(0.,-1.,0.)) ;
#63801=DIRECTION('ref_axis',(-1.,0.,0.)) ;
#63802=DIRECTION('',(-9.79313055424617E-16,1.,0.)) ;
#63803=DIRECTION('center_axis',(1.,9.79313055424617E-16,0.)) ;
#63804=DIRECTION('ref_axis',(0.,0.,-1.)) ;
#63805=DIRECTION('center_axis',(0.,-0.94868329805046,-0.316227766016998)) ;
#63806=DIRECTION('ref_axis',(-1.,0.,0.)) ;
#63807=DIRECTION('center_axis',(-1.,-9.79313055424617E-16,0.)) ;
#63808=DIRECTION('ref_axis',(-1.56868561823944E-16,0.16018224300699,-0.987087457637493)) ;
#63809=DIRECTION('center_axis',(1.,9.79313055424617E-16,0.)) ;
#63810=DIRECTION('ref_axis',(-1.56868561823944E-16,0.16018224300699,-0.987087457637493)) ;
#63811=DIRECTION('center_axis',(-9.2905793924415E-16,0.948683298050513,
0.316227766016839)) ;
#63812=DIRECTION('ref_axis',(-0.707106781186599,0.223606797749963,-0.670820393249888)) ;
#63813=DIRECTION('center_axis',(0.,-0.948683298050571,-0.316227766016665)) ;
#63814=DIRECTION('ref_axis',(-1.,0.,0.)) ;
#63815=DIRECTION('',(9.29057939244151E-16,-0.948683298050513,-0.316227766016839)) ;
#63816=DIRECTION('',(-9.29057939244151E-16,0.948683298050513,0.316227766016839)) ;
#63817=DIRECTION('center_axis',(1.,9.79313055424617E-16,0.)) ;
#63818=DIRECTION('ref_axis',(0.,0.,-1.)) ;
#63819=DIRECTION('center_axis',(-1.,-9.79313055424617E-16,0.)) ;
#63820=DIRECTION('ref_axis',(-5.0670923265072E-16,0.517412925156009,-0.855735861631089)) ;
#63821=DIRECTION('center_axis',(1.,9.79313055424617E-16,0.)) ;
#63822=DIRECTION('ref_axis',(-5.0670923265072E-16,0.517412925156009,-0.855735861631089)) ;
#63823=DIRECTION('center_axis',(0.,0.,-1.)) ;
#63824=DIRECTION('ref_axis',(0.,1.,0.)) ;
#63825=DIRECTION('',(0.,0.,-1.)) ;
#63826=DIRECTION('center_axis',(-8.57083562089732E-97,-5.13170824337699E-49,
-1.)) ;
#63827=DIRECTION('ref_axis',(0.,1.,-5.13170824337699E-49)) ;
#63828=DIRECTION('center_axis',(-1.,-9.79313055424617E-16,0.)) ;
#63829=DIRECTION('ref_axis',(-9.79313055424617E-16,1.,-5.30037252443606E-33)) ;
#63830=DIRECTION('',(0.,0.,-1.)) ;
#63831=DIRECTION('',(-9.79313055424617E-16,1.,-5.30037252443606E-33)) ;
#63832=DIRECTION('center_axis',(0.,0.,-1.)) ;
#63833=DIRECTION('ref_axis',(-0.819152044288991,-0.573576436351047,0.)) ;
#63834=DIRECTION('',(0.,0.,-1.)) ;
#63835=DIRECTION('center_axis',(-8.11022789614398E-33,1.15826058041052E-32,
-1.)) ;
#63836=DIRECTION('ref_axis',(-0.819152044288991,-0.573576436351047,-1.67157598811966E-45)) ;
#63837=DIRECTION('center_axis',(-0.819152044288994,-0.573576436351043,0.)) ;
#63838=DIRECTION('ref_axis',(-0.573576436351043,0.819152044288994,0.)) ;
#63839=DIRECTION('',(0.,0.,-1.)) ;
#63840=DIRECTION('',(0.573576436351043,-0.819152044288994,4.46962256005402E-32)) ;
#63841=DIRECTION('',(0.,0.,-1.)) ;
#63842=DIRECTION('',(-0.573576436351043,0.819152044288994,0.)) ;
#63843=DIRECTION('center_axis',(0.,0.,-1.)) ;
#63844=DIRECTION('ref_axis',(-0.173648177666935,-0.984807753012207,0.)) ;
#63845=DIRECTION('',(0.,0.,-1.)) ;
#63846=DIRECTION('center_axis',(1.09763027743844E-32,6.22497063709847E-32,
1.)) ;
#63847=DIRECTION('ref_axis',(-0.587740293442623,-0.809049656982796,5.68143190002567E-32)) ;
#63848=DIRECTION('center_axis',(-0.997835226140326,0.0657636789837963,0.)) ;
#63849=DIRECTION('ref_axis',(-0.0465019433652248,-0.705576054910746,-0.707106781186438)) ;
#63850=DIRECTION('center_axis',(0.997835226140338,-0.0657636789836146,0.)) ;
#63851=DIRECTION('ref_axis',(-0.0657636789836146,-0.997835226140338,0.)) ;
#63852=DIRECTION('',(-0.997835226140326,0.0657636789837963,0.)) ;
#63853=DIRECTION('center_axis',(-0.672457840829202,0.309193959537835,0.672457840829181)) ;
#63854=DIRECTION('ref_axis',(1.60829332345463E-16,-0.90856053509436,0.41775322149452)) ;
#63855=DIRECTION('center_axis',(-0.707106781186536,-3.14018491736822E-14,
0.707106781186559)) ;
#63856=DIRECTION('ref_axis',(-4.43693537133302E-29,-1.,-4.44089209850151E-14)) ;
#63857=DIRECTION('center_axis',(-0.70710678118655,-8.10370301256138E-15,
-0.707106781186545)) ;
#63858=DIRECTION('ref_axis',(0.707106781186545,-1.41676311701544E-14,-0.70710678118655)) ;
#63859=DIRECTION('center_axis',(0.447213595499966,1.9860273225975E-14,0.894427190999912)) ;
#63860=DIRECTION('ref_axis',(0.894427190999912,-1.8300617384979E-31,-0.447213595499966)) ;
#63861=DIRECTION('center_axis',(-0.707106781186545,3.06359504133419E-15,
0.70710678118655)) ;
#63862=DIRECTION('ref_axis',(0.500000000000059,-0.707106781186465,0.500000000000058)) ;
#63863=DIRECTION('center_axis',(-0.707106781186525,0.,0.70710678118657)) ;
#63864=DIRECTION('ref_axis',(0.,-1.,0.)) ;
#63865=DIRECTION('',(0.707106781186545,-3.06359504133419E-15,-0.70710678118655)) ;
#63866=DIRECTION('',(-0.707106781186545,3.06359504133419E-15,0.70710678118655)) ;
#63867=DIRECTION('center_axis',(-0.624695047554719,-0.468521285665242,0.624695047554562)) ;
#63868=DIRECTION('ref_axis',(0.599999999999318,-0.800000000000512,-4.45819707740118E-14)) ;
#63869=DIRECTION('center_axis',(-0.70710678118655,-8.10370301256138E-15,
-0.707106781186545)) ;
#63870=DIRECTION('ref_axis',(-0.707106781186545,-8.04672385075432E-15,0.70710678118655)) ;
#63871=DIRECTION('center_axis',(0.780868809443032,1.73387706291061E-14,
0.624695047554423)) ;
#63872=DIRECTION('ref_axis',(-0.624695047554423,-1.75046575158144E-31,0.780868809443031)) ;
#63873=DIRECTION('center_axis',(-0.514495755427105,-0.685994340570717,0.51449575542704)) ;
#63874=DIRECTION('ref_axis',(0.800000000000522,-0.599999999999304,-6.96026688936854E-17)) ;
#63875=DIRECTION('center_axis',(-0.707106781185896,-1.3346564596511E-12,
-0.707106781187199)) ;
#63876=DIRECTION('ref_axis',(0.664495781864865,0.341892836673091,-0.664495781864286)) ;
#63877=DIRECTION('center_axis',(0.781646665849804,-0.00199881414324549,
0.623718281364195)) ;
#63878=DIRECTION('ref_axis',(0.613196036400756,-0.180472748793488,-0.769038495710927)) ;
#63879=DIRECTION('center_axis',(0.780868809443032,1.73387706291061E-14,
0.624695047554423)) ;
#63880=DIRECTION('ref_axis',(-0.624695047554423,-1.75046575158144E-31,0.780868809443031)) ;
#63881=DIRECTION('center_axis',(-0.70710678118655,-8.10370301256138E-15,
-0.707106781186545)) ;
#63882=DIRECTION('ref_axis',(-0.707106781186545,-8.04672385075432E-15,0.70710678118655)) ;
#63883=DIRECTION('center_axis',(0.,0.,-1.)) ;
#63884=DIRECTION('ref_axis',(-0.707106781186548,0.707106781186548,0.)) ;
#63885=DIRECTION('',(0.,0.,-1.)) ;
#63886=DIRECTION('center_axis',(0.,0.242535625036338,-0.970142500145331)) ;
#63887=DIRECTION('ref_axis',(0.,0.970142500145331,0.242535625036338)) ;
#63888=DIRECTION('',(0.,0.,1.)) ;
#63889=DIRECTION('center_axis',(-0.70710678118655,-8.10370301256138E-15,
-0.707106781186545)) ;
#63890=DIRECTION('ref_axis',(-0.707106781186545,-1.02766135666342E-31,0.70710678118655)) ;
#63891=DIRECTION('',(-0.577350269189617,-0.577350269189633,0.577350269189627)) ;
#63892=DIRECTION('',(1.1460366705808E-14,-1.,1.11561779098947E-30)) ;
#63893=DIRECTION('',(0.577350269189627,-0.577350269189627,-0.577350269189624)) ;
#63894=DIRECTION('',(-1.1460366705808E-14,1.,0.)) ;
#63895=DIRECTION('center_axis',(-0.70710678118655,-8.10370301256138E-15,
-0.707106781186545)) ;
#63896=DIRECTION('ref_axis',(-0.707106781186545,1.41902270731371E-14,0.70710678118655)) ;
#63897=DIRECTION('center_axis',(-4.33257765707378E-15,-1.,0.)) ;
#63898=DIRECTION('ref_axis',(-1.,4.33257765707378E-15,0.)) ;
#63899=DIRECTION('',(1.,-4.33257765707378E-15,0.)) ;
#63900=DIRECTION('center_axis',(-1.,4.33257765707378E-15,0.)) ;
#63901=DIRECTION('ref_axis',(3.44001377016025E-15,0.793987792588958,-0.607933701335692)) ;
#63902=DIRECTION('',(-1.,4.33257765707378E-15,0.)) ;
#63903=DIRECTION('center_axis',(-1.,0.,0.)) ;
#63904=DIRECTION('ref_axis',(0.,1.,0.)) ;
#63905=DIRECTION('center_axis',(-1.38777878078145E-15,1.,0.)) ;
#63906=DIRECTION('ref_axis',(-0.707106781186532,-9.81307786677341E-16,-0.707106781186563)) ;
#63907=DIRECTION('center_axis',(0.70710678118661,0.707106781186485,0.)) ;
#63908=DIRECTION('ref_axis',(0.707106781186485,-0.70710678118661,0.)) ;
#63909=DIRECTION('',(-1.38777878078145E-15,1.,0.)) ;
#63910=DIRECTION('center_axis',(0.,0.,-1.)) ;
#63911=DIRECTION('ref_axis',(-1.,0.,0.)) ;
#63912=DIRECTION('center_axis',(0.,0.,-1.)) ;
#63913=DIRECTION('ref_axis',(0.,-1.,0.)) ;
#63914=DIRECTION('center_axis',(0.,-1.,0.)) ;
#63915=DIRECTION('ref_axis',(0.707106781186532,0.,-0.707106781186563)) ;
#63916=DIRECTION('',(0.,-1.,0.)) ;
#63917=DIRECTION('center_axis',(-0.70710678118661,0.707106781186485,0.)) ;
#63918=DIRECTION('ref_axis',(0.707106781186485,0.70710678118661,0.)) ;
#63919=DIRECTION('center_axis',(1.,0.,0.)) ;
#63920=DIRECTION('ref_axis',(0.,0.707106781186469,-0.707106781186626)) ;
#63921=DIRECTION('',(1.,0.,0.)) ;
#63922=DIRECTION('center_axis',(0.,0.,-1.)) ;
#63923=DIRECTION('ref_axis',(1.,0.,0.)) ;
#63924=DIRECTION('',(0.,0.,-1.)) ;
#63925=DIRECTION('center_axis',(1.09763027743844E-32,6.22497063709847E-32,
1.)) ;
#63926=DIRECTION('ref_axis',(1.,-6.83271624744454E-64,-1.09763027743844E-32)) ;
#63927=DIRECTION('',(0.,0.,-1.)) ;
#63928=DIRECTION('center_axis',(1.,1.38777878078145E-15,0.)) ;
#63929=DIRECTION('ref_axis',(1.38777878078145E-15,-1.,0.)) ;
#63930=DIRECTION('',(0.,0.,1.)) ;
#63931=DIRECTION('',(1.38777878078145E-15,-1.,6.22497063709847E-32)) ;
#63932=DIRECTION('center_axis',(0.,0.,-1.)) ;
#63933=DIRECTION('ref_axis',(1.,0.,0.)) ;
#63934=DIRECTION('center_axis',(-1.,8.88178419700302E-14,-8.88178419700105E-14)) ;
#63935=DIRECTION('ref_axis',(8.88178419700302E-14,1.,-3.58732406902838E-43)) ;
#63936=DIRECTION('center_axis',(-3.97205464519572E-14,0.447213595499958,
0.894427190999916)) ;
#63937=DIRECTION('ref_axis',(-3.97205464519572E-14,-0.894427190999916,0.447213595499958)) ;
#63938=DIRECTION('center_axis',(3.97205464519622E-14,-0.894427190999888,
-0.447213595500014)) ;
#63939=DIRECTION('ref_axis',(-3.97205464519551E-14,-0.447213595500014,0.894427190999888)) ;
#63940=DIRECTION('center_axis',(1.09763027743844E-32,6.22497063709847E-32,
1.)) ;
#63941=DIRECTION('ref_axis',(1.,0.,0.)) ;
#63942=DIRECTION('center_axis',(-0.707106781186459,0.707106781186636,0.)) ;
#63943=DIRECTION('ref_axis',(0.707106781186636,0.707106781186459,0.)) ;
#63944=DIRECTION('center_axis',(1.09763027743844E-32,6.22497063709847E-32,
1.)) ;
#63945=DIRECTION('ref_axis',(-0.38268343236507,-0.923879532511295,6.17116788413704E-32)) ;
#63946=DIRECTION('center_axis',(-1.09763027743844E-32,-6.22497063709847E-32,
-1.)) ;
#63947=DIRECTION('ref_axis',(-0.38268343236507,-0.923879532511295,6.17116788413704E-32)) ;
#63948=DIRECTION('center_axis',(0.707106781186472,-0.707106781186624,3.62557713776763E-32)) ;
#63949=DIRECTION('ref_axis',(0.500000000000021,0.499999999999913,-0.707106781186594)) ;
#63950=DIRECTION('',(0.707106781186472,-0.707106781186624,3.62557713776763E-32)) ;
#63951=DIRECTION('',(-0.707106781186472,0.707106781186624,-3.62557713776763E-32)) ;
#63952=DIRECTION('center_axis',(-0.707106781186624,-0.707106781186472,0.)) ;
#63953=DIRECTION('ref_axis',(-0.707106781186472,0.707106781186624,0.)) ;
#63954=DIRECTION('',(0.,0.,-1.)) ;
#63955=DIRECTION('',(-0.707106781186471,0.707106781186624,0.)) ;
#63956=DIRECTION('',(0.,0.,-1.)) ;
#63957=DIRECTION('',(-0.707106781186471,0.707106781186624,0.)) ;
#63958=DIRECTION('',(0.,0.,-1.)) ;
#63959=DIRECTION('center_axis',(0.,0.,-1.)) ;
#63960=DIRECTION('ref_axis',(0.382683432365038,-0.923879532511308,0.)) ;
#63961=DIRECTION('',(0.,0.,1.)) ;
#63962=DIRECTION('center_axis',(2.46519032881572E-32,8.55284707229503E-50,
-1.)) ;
#63963=DIRECTION('ref_axis',(0.382683432365038,-0.923879532511308,9.43387496464296E-33)) ;
#63964=DIRECTION('center_axis',(3.67742382159233E-14,1.,-6.22497063709851E-32)) ;
#63965=DIRECTION('ref_axis',(0.707106781186548,-2.60033132154489E-14,0.707106781186548)) ;
#63966=DIRECTION('',(-3.67742382159233E-14,-1.,6.22497063709851E-32)) ;
#63967=DIRECTION('center_axis',(0.,-1.,0.)) ;
#63968=DIRECTION('ref_axis',(1.,0.,0.)) ;
#63969=DIRECTION('',(3.67742382159233E-14,1.,-6.22497063709851E-32)) ;
#63970=DIRECTION('center_axis',(-0.439732612032359,-0.182143211721388,-0.879465224064611)) ;
#63971=DIRECTION('ref_axis',(0.812519920068743,0.336556770590752,-0.475963149477991)) ;
#63972=DIRECTION('center_axis',(0.,0.,1.)) ;
#63973=DIRECTION('ref_axis',(0.707106781186547,0.707106781186547,0.)) ;
#63974=DIRECTION('center_axis',(-0.707106781186548,0.707106781186548,0.)) ;
#63975=DIRECTION('ref_axis',(0.,0.,-1.)) ;
#63976=DIRECTION('center_axis',(0.,-1.,0.)) ;
#63977=DIRECTION('ref_axis',(1.,0.,0.)) ;
#63978=DIRECTION('center_axis',(-0.707106781186607,0.707106781186488,0.)) ;
#63979=DIRECTION('ref_axis',(0.499999999999925,0.500000000000009,-0.707106781186594)) ;
#63980=DIRECTION('',(0.707106781186607,-0.707106781186488,0.)) ;
#63981=DIRECTION('',(-0.707106781186607,0.707106781186488,0.)) ;
#63982=DIRECTION('center_axis',(1.08152878803189E-14,1.,0.)) ;
#63983=DIRECTION('ref_axis',(0.707106781186485,-7.6475634006575E-15,-0.70710678118661)) ;
#63984=DIRECTION('',(1.08152878803189E-14,1.,0.)) ;
#63985=DIRECTION('',(-1.08152878803189E-14,-1.,0.)) ;
#63986=DIRECTION('center_axis',(0.,0.,-1.)) ;
#63987=DIRECTION('ref_axis',(-1.,0.,0.)) ;
#63988=DIRECTION('center_axis',(0.,0.,-1.)) ;
#63989=DIRECTION('ref_axis',(1.,0.,0.)) ;
#63990=DIRECTION('center_axis',(0.,-1.,0.)) ;
#63991=DIRECTION('ref_axis',(0.,0.,1.)) ;
#63992=DIRECTION('center_axis',(7.16300942304673E-47,-7.6997105554314E-34,
1.)) ;
#63993=DIRECTION('ref_axis',(0.923879532511283,0.382683432365099,2.94655166356961E-34)) ;
#63994=DIRECTION('center_axis',(-0.707106781186548,0.707106781186548,0.)) ;
#63995=DIRECTION('ref_axis',(-0.707106781186547,-0.707106781186547,0.)) ;
#63996=DIRECTION('center_axis',(-1.08152878803189E-14,-1.,-7.6997105554314E-34)) ;
#63997=DIRECTION('ref_axis',(-0.70710678118661,7.64756340065885E-15,0.707106781186485)) ;
#63998=DIRECTION('',(1.08152878803189E-14,1.,7.6997105554314E-34)) ;
#63999=DIRECTION('',(-1.08152878803189E-14,-1.,-7.6997105554314E-34)) ;
#64000=DIRECTION('center_axis',(0.707106781186607,-0.707106781186488,-5.44451754691923E-34)) ;
#64001=DIRECTION('ref_axis',(-0.499999999999925,-0.500000000000009,0.707106781186594)) ;
#64002=DIRECTION('',(0.707106781186607,-0.707106781186488,-5.44451754691923E-34)) ;
#64003=DIRECTION('',(-0.707106781186607,0.707106781186488,5.44451754691923E-34)) ;
#64004=DIRECTION('center_axis',(0.,0.,-1.)) ;
#64005=DIRECTION('ref_axis',(0.923879532511283,0.382683432365099,0.)) ;
#64006=DIRECTION('',(0.,0.,1.)) ;
#64007=DIRECTION('',(0.,0.,-1.)) ;
#64008=DIRECTION('center_axis',(0.,0.,-1.)) ;
#64009=DIRECTION('ref_axis',(1.,0.,0.)) ;
#64010=DIRECTION('',(0.800000000000003,0.599999999999996,0.)) ;
#64011=DIRECTION('center_axis',(0.,0.,-1.)) ;
#64012=DIRECTION('ref_axis',(-0.894427190999906,0.447213595499978,0.)) ;
#64013=DIRECTION('',(0.,1.,0.)) ;
#64014=DIRECTION('center_axis',(2.46519032881566E-32,2.3408381773461E-97,
-1.)) ;
#64015=DIRECTION('ref_axis',(1.,1.99159183953863E-159,2.46519032881566E-32)) ;
#64016=DIRECTION('',(0.,-1.,0.)) ;
#64017=DIRECTION('center_axis',(0.,0.,-1.)) ;
#64018=DIRECTION('ref_axis',(1.,0.,0.)) ;
#64019=DIRECTION('',(-1.,0.,2.76147456380442E-35)) ;
#64020=DIRECTION('center_axis',(0.,5.60383084497445E-34,1.)) ;
#64021=DIRECTION('ref_axis',(0.,1.,-5.60383084497445E-34)) ;
#64022=DIRECTION('',(1.77635683940243E-14,1.,0.)) ;
#64023=DIRECTION('',(1.,0.,0.)) ;
#64024=DIRECTION('',(-6.34413156929222E-15,1.,0.)) ;
#64025=DIRECTION('',(-1.,0.,0.)) ;
#64026=DIRECTION('',(0.,1.,0.)) ;
#64027=DIRECTION('center_axis',(0.,0.,1.)) ;
#64028=DIRECTION('ref_axis',(1.,0.,0.)) ;
#64029=DIRECTION('',(1.,-1.75071816546432E-14,-2.18941313571177E-49)) ;
#64030=DIRECTION('center_axis',(-2.46519032881566E-32,4.44295269748681E-48,
1.)) ;
#64031=DIRECTION('ref_axis',(0.,-1.,4.44295269748681E-48)) ;
#64032=DIRECTION('',(0.707106781186581,-0.707106781186514,0.)) ;
#64033=DIRECTION('center_axis',(0.,0.,1.)) ;
#64034=DIRECTION('ref_axis',(-0.707106781186481,-0.707106781186614,0.)) ;
#64035=DIRECTION('',(-5.35505761538791E-15,-1.,1.48632706569949E-33)) ;
#64036=DIRECTION('center_axis',(0.,0.,-1.)) ;
#64037=DIRECTION('ref_axis',(1.,0.,0.)) ;
#64038=DIRECTION('',(0.,1.,0.)) ;
#64039=DIRECTION('center_axis',(2.46519032881566E-32,2.3408381773461E-97,
-1.)) ;
#64040=DIRECTION('ref_axis',(1.,1.99159183953863E-159,2.46519032881566E-32)) ;
#64041=DIRECTION('',(2.61228946970624E-14,1.,0.)) ;
#64042=DIRECTION('center_axis',(0.,0.,-1.)) ;
#64043=DIRECTION('ref_axis',(0.948683298050522,0.316227766016813,0.)) ;
#64044=DIRECTION('',(0.599999999999982,-0.800000000000014,0.)) ;
#64045=DIRECTION('',(1.,0.,3.20175569450239E-16)) ;
#64046=DIRECTION('',(0.800000000000002,0.599999999999998,0.)) ;
#64047=DIRECTION('center_axis',(0.,0.,-1.)) ;
#64048=DIRECTION('ref_axis',(-0.89442719099992,0.44721359549995,0.)) ;
#64049=DIRECTION('',(0.,1.,0.)) ;
#64050=DIRECTION('center_axis',(2.46519032881566E-32,2.3408381773461E-97,
-1.)) ;
#64051=DIRECTION('ref_axis',(1.,1.99159183953863E-159,2.46519032881566E-32)) ;
#64052=DIRECTION('',(0.,-1.,0.)) ;
#64053=DIRECTION('center_axis',(0.,0.,-1.)) ;
#64054=DIRECTION('ref_axis',(1.,0.,0.)) ;
#64055=DIRECTION('',(0.,1.,0.)) ;
#64056=DIRECTION('center_axis',(2.46519032881566E-32,2.3408381773461E-97,
-1.)) ;
#64057=DIRECTION('ref_axis',(1.,1.99159183953863E-159,2.46519032881566E-32)) ;
#64058=DIRECTION('',(0.,1.,0.)) ;
#64059=DIRECTION('center_axis',(0.,0.,-1.)) ;
#64060=DIRECTION('ref_axis',(0.948683298050519,0.316227766016821,0.)) ;
#64061=DIRECTION('',(0.600000000000002,-0.799999999999998,0.)) ;
#64062=DIRECTION('',(-1.,0.,0.)) ;
#64063=DIRECTION('',(0.,-1.,0.)) ;
#64064=DIRECTION('',(1.,0.,0.)) ;
#64065=DIRECTION('',(-1.30614473485314E-15,1.,0.)) ;
#64066=DIRECTION('',(1.,0.,0.)) ;
#64067=DIRECTION('',(-1.,0.,0.)) ;
#64068=DIRECTION('',(1.,0.,0.)) ;
#64069=DIRECTION('',(0.,-1.,0.)) ;
#64070=DIRECTION('',(1.,-4.35522519302374E-15,0.)) ;
#64071=DIRECTION('center_axis',(0.,0.,-1.)) ;
#64072=DIRECTION('ref_axis',(0.,1.,0.)) ;
#64073=DIRECTION('',(-1.46896958313692E-15,-1.,0.)) ;
#64074=DIRECTION('center_axis',(0.,0.,1.)) ;
#64075=DIRECTION('ref_axis',(-0.819152044288993,-0.573576436351044,0.)) ;
#64076=DIRECTION('',(0.573576436351043,-0.819152044288994,0.)) ;
#64077=DIRECTION('',(0.,1.,0.)) ;
#64078=DIRECTION('center_axis',(0.,0.,-1.)) ;
#64079=DIRECTION('ref_axis',(-1.,0.,0.)) ;
#64080=DIRECTION('',(0.529919264233188,0.848048096156437,0.)) ;
#64081=DIRECTION('',(-0.707106781186471,0.707106781186624,0.)) ;
#64082=DIRECTION('center_axis',(0.,0.,-1.)) ;
#64083=DIRECTION('ref_axis',(-1.,0.,0.)) ;
#64084=DIRECTION('',(0.801695394071906,-0.597732795757345,0.)) ;
#64085=DIRECTION('',(3.67742382159233E-14,1.,0.)) ;
#64086=DIRECTION('',(1.,0.,0.)) ;
#64087=DIRECTION('',(-3.67742382159233E-14,-1.,0.)) ;
#64088=DIRECTION('center_axis',(0.,0.,1.)) ;
#64089=DIRECTION('ref_axis',(-0.918360381793699,0.395745131557839,0.)) ;
#64090=DIRECTION('center_axis',(0.,0.,1.)) ;
#64091=DIRECTION('ref_axis',(-0.977748097404052,0.209782406370878,0.)) ;
#64092=DIRECTION('center_axis',(2.52374105052742E-18,5.60383084497445E-34,
-1.)) ;
#64093=DIRECTION('ref_axis',(-1.,3.9474596431117E-14,-2.52374105052742E-18)) ;
#64094=DIRECTION('center_axis',(2.46519032881566E-32,-1.7915701050753E-48,
-1.)) ;
#64095=DIRECTION('ref_axis',(0.,-1.,1.7915701050753E-48)) ;
#64096=DIRECTION('',(-3.17206578464333E-15,-1.,1.76085023486835E-33)) ;
#64097=DIRECTION('center_axis',(2.46519032881571E-32,4.87512283120816E-48,
-1.)) ;
#64098=DIRECTION('ref_axis',(-1.,-3.7453410837561E-96,-2.46519032881571E-32)) ;
#64099=DIRECTION('',(-1.,-3.55271367880026E-13,3.80009837042949E-30)) ;
#64100=DIRECTION('',(0.,-1.,1.41044871512355E-33)) ;
#64101=DIRECTION('center_axis',(2.46519032881571E-32,4.87512283120816E-48,
-1.)) ;
#64102=DIRECTION('ref_axis',(-1.,-3.7453410837561E-96,-2.46519032881571E-32)) ;
#64103=DIRECTION('',(-1.,0.,-1.40067632319071E-31)) ;
#64104=DIRECTION('center_axis',(2.46519032881566E-32,-1.7915701050753E-48,
-1.)) ;
#64105=DIRECTION('ref_axis',(0.,1.,-1.7915701050753E-48)) ;
#64106=DIRECTION('',(1.53134210293125E-15,1.,-6.60793205056998E-32)) ;
#64107=DIRECTION('',(-1.,0.,3.83260058933034E-30)) ;
#64108=DIRECTION('center_axis',(2.46519032881566E-32,0.,-1.)) ;
#64109=DIRECTION('ref_axis',(0.,1.,0.)) ;
#64110=DIRECTION('',(3.17206578464333E-15,1.,-1.76085023486835E-33)) ;
#64111=DIRECTION('center_axis',(0.,0.,-1.)) ;
#64112=DIRECTION('ref_axis',(-1.,3.9474596431117E-14,0.)) ;
#64113=DIRECTION('',(1.,-3.55271367880048E-14,0.)) ;
#64114=DIRECTION('',(0.,1.,0.)) ;
#64115=DIRECTION('',(1.,0.,6.12949496482233E-35)) ;
#64116=DIRECTION('center_axis',(2.46519032881566E-32,-2.48770373612753E-33,
1.)) ;
#64117=DIRECTION('ref_axis',(0.,-1.,-2.48770373612753E-33)) ;
#64118=DIRECTION('',(0.707106781186586,-0.707106781186509,-7.3914897815741E-47)) ;
#64119=DIRECTION('center_axis',(8.71576399210415E-33,-8.71576399210634E-33,
1.)) ;
#64120=DIRECTION('ref_axis',(-0.707106781186681,-0.707106781186414,7.78326232344021E-46)) ;
#64121=DIRECTION('',(-5.35505761538786E-15,-1.,7.43163532849736E-34)) ;
#64122=DIRECTION('center_axis',(-2.46519032881571E-32,-5.98699295060652E-49,
1.)) ;
#64123=DIRECTION('ref_axis',(-1.,7.31836847501401E-110,-2.46519032881571E-32)) ;
#64124=DIRECTION('',(-0.707106781186539,-0.707106781186556,1.17554800907501E-33)) ;
#64125=DIRECTION('center_axis',(3.18850138855159E-46,1.74315279842113E-32,
1.)) ;
#64126=DIRECTION('ref_axis',(-0.707106781186636,0.707106781186459,-1.23259516440771E-32)) ;
#64127=DIRECTION('',(-1.,0.,0.)) ;
#64128=DIRECTION('',(0.,1.,0.)) ;
#64129=DIRECTION('center_axis',(0.,0.,1.)) ;
#64130=DIRECTION('ref_axis',(-0.73407014073105,0.679073654684893,0.)) ;
#64131=DIRECTION('center_axis',(0.,0.,-1.)) ;
#64132=DIRECTION('ref_axis',(0.457543425680166,-0.889187277021471,0.)) ;
#64133=DIRECTION('',(-0.642787609686516,-0.766044443118998,0.)) ;
#64134=DIRECTION('center_axis',(0.,0.,-1.)) ;
#64135=DIRECTION('ref_axis',(0.939692620785897,-0.3420201433257,0.)) ;
#64136=DIRECTION('',(-1.20119700805775E-14,-1.,0.)) ;
#64137=DIRECTION('',(0.642787609686599,-0.766044443118928,0.)) ;
#64138=DIRECTION('center_axis',(0.,0.,-1.)) ;
#64139=DIRECTION('ref_axis',(0.422618261740741,0.906307787036631,0.)) ;
#64140=DIRECTION('',(1.,-1.28403006865249E-14,0.)) ;
#64141=DIRECTION('center_axis',(0.,0.,1.)) ;
#64142=DIRECTION('ref_axis',(0.,1.,0.)) ;
#64143=DIRECTION('center_axis',(0.,0.,1.)) ;
#64144=DIRECTION('ref_axis',(1.,0.,0.)) ;
#64145=DIRECTION('',(0.,1.,0.)) ;
#64146=DIRECTION('',(1.,0.,0.)) ;
#64147=DIRECTION('center_axis',(0.,0.,1.)) ;
#64148=DIRECTION('ref_axis',(1.,0.,0.)) ;
#64149=DIRECTION('',(1.,0.,-1.93235546378459E-35)) ;
#64150=DIRECTION('center_axis',(0.,5.60383084497445E-34,1.)) ;
#64151=DIRECTION('ref_axis',(0.,-1.,5.60383084497445E-34)) ;
#64152=DIRECTION('',(-5.69345140833415E-16,-1.,3.47655046371441E-32)) ;
#64153=DIRECTION('center_axis',(-1.35585468084861E-30,4.50611349139124E-93,
1.)) ;
#64154=DIRECTION('ref_axis',(-1.,4.98510362034913E-139,-1.35585468084861E-30)) ;
#64155=DIRECTION('',(-1.,-6.125368411725E-15,1.93235546378459E-35)) ;
#64156=DIRECTION('center_axis',(0.,5.60383084497445E-34,1.)) ;
#64157=DIRECTION('ref_axis',(0.,1.,-5.60383084497445E-34)) ;
#64158=DIRECTION('',(-1.13869028166683E-15,1.,0.)) ;
#64159=DIRECTION('center_axis',(0.,0.,1.)) ;
#64160=DIRECTION('ref_axis',(1.,0.,0.)) ;
#64161=DIRECTION('center_axis',(-2.46519032881571E-32,-4.87512283120816E-48,
1.)) ;
#64162=DIRECTION('ref_axis',(-1.,-3.7453410837561E-96,-2.46519032881571E-32)) ;
#64163=DIRECTION('',(-1.,0.,1.62870009552296E-49)) ;
#64164=DIRECTION('center_axis',(-2.46519032881566E-32,1.7915701050753E-48,
1.)) ;
#64165=DIRECTION('ref_axis',(0.,1.,-1.7915701050753E-48)) ;
#64166=DIRECTION('',(1.53134210293126E-15,1.,0.)) ;
#64167=DIRECTION('',(-1.,3.55271367880026E-13,9.05696233641872E-48)) ;
#64168=DIRECTION('center_axis',(-2.46519032881566E-32,4.52848116820976E-48,
1.)) ;
#64169=DIRECTION('ref_axis',(0.,1.,-4.52848116820976E-48)) ;
#64170=DIRECTION('',(0.,1.,-1.76085023486835E-33)) ;
#64171=DIRECTION('center_axis',(-2.46519032881572E-32,-8.55284707229503E-50,
1.)) ;
#64172=DIRECTION('ref_axis',(1.,-2.20382687031672E-110,2.46519032881572E-32)) ;
#64173=DIRECTION('',(1.,-1.26882631385732E-14,-1.27969293219661E-49)) ;
#64174=DIRECTION('center_axis',(-2.46519032881566E-32,1.7915701050753E-48,
1.)) ;
#64175=DIRECTION('ref_axis',(0.,-1.,1.7915701050753E-48)) ;
#64176=DIRECTION('',(0.,-1.,1.76085023486835E-33)) ;
#64177=DIRECTION('center_axis',(-2.46519032881571E-32,-4.87512283120816E-48,
1.)) ;
#64178=DIRECTION('ref_axis',(-1.,-3.7453410837561E-96,-2.46519032881571E-32)) ;
#64179=DIRECTION('',(-1.,-3.55271367880026E-13,5.47382212626845E-48)) ;
#64180=DIRECTION('',(0.,-1.,8.50065630626093E-34)) ;
#64181=DIRECTION('center_axis',(0.,0.,1.)) ;
#64182=DIRECTION('ref_axis',(1.,0.,0.)) ;
#64183=DIRECTION('',(0.,-1.,0.)) ;
#64184=DIRECTION('',(-1.,8.7535908273216E-15,2.56873619635494E-49)) ;
#64185=DIRECTION('center_axis',(-2.46519032881566E-32,5.21270893399338E-48,
1.)) ;
#64186=DIRECTION('ref_axis',(0.,1.,-5.21270893399338E-48)) ;
#64187=DIRECTION('',(-0.707106781186556,0.707106781186539,0.)) ;
#64188=DIRECTION('center_axis',(0.,0.,1.)) ;
#64189=DIRECTION('ref_axis',(0.707106781186636,0.707106781186459,0.)) ;
#64190=DIRECTION('',(0.,1.,-1.48632706569949E-33)) ;
#64191=DIRECTION('center_axis',(-2.46519032881571E-32,-3.84878118253276E-49,
1.)) ;
#64192=DIRECTION('ref_axis',(1.,7.31836847501401E-110,2.46519032881571E-32)) ;
#64193=DIRECTION('',(0.707106781186522,0.707106781186573,-4.31889331967372E-49)) ;
#64194=DIRECTION('center_axis',(-8.71576399210634E-33,-8.71576399210415E-33,
1.)) ;
#64195=DIRECTION('ref_axis',(0.707106781186459,-0.707106781186636,6.33174217877954E-48)) ;
#64196=DIRECTION('',(1.,0.,0.)) ;
#64197=DIRECTION('',(-1.,0.,0.)) ;
#64198=DIRECTION('',(0.,1.,0.)) ;
#64199=DIRECTION('',(-1.,3.55271367880026E-13,2.00046065889556E-47)) ;
#64200=DIRECTION('center_axis',(-2.46519032881566E-32,1.00023032944787E-47,
1.)) ;
#64201=DIRECTION('ref_axis',(0.,1.,-1.00023032944787E-47)) ;
#64202=DIRECTION('',(0.,1.,-1.76085023486835E-33)) ;
#64203=DIRECTION('center_axis',(-2.46519032881571E-32,0.,1.)) ;
#64204=DIRECTION('ref_axis',(1.,0.,2.46519032881571E-32)) ;
#64205=DIRECTION('',(1.,0.,-4.0027363178395E-35)) ;
#64206=DIRECTION('center_axis',(0.,5.60383084497445E-34,1.)) ;
#64207=DIRECTION('ref_axis',(0.,-1.,5.60383084497445E-34)) ;
#64208=DIRECTION('',(0.,-1.,1.76085023486835E-33)) ;
#64209=DIRECTION('center_axis',(-2.46519032881571E-32,-4.6816763546922E-97,
1.)) ;
#64210=DIRECTION('ref_axis',(-1.,1.001486182168E-157,-2.46519032881571E-32)) ;
#64211=DIRECTION('',(-1.,0.,0.)) ;
#64212=DIRECTION('',(0.,-1.,0.)) ;
#64213=DIRECTION('center_axis',(-2.46519032881571E-32,-4.87512283120816E-48,
1.)) ;
#64214=DIRECTION('ref_axis',(-1.,-3.7453410837561E-96,-2.46519032881571E-32)) ;
#64215=DIRECTION('',(-1.,0.,1.62870009552296E-49)) ;
#64216=DIRECTION('center_axis',(-2.46519032881566E-32,1.7915701050753E-48,
1.)) ;
#64217=DIRECTION('ref_axis',(0.,1.,-1.7915701050753E-48)) ;
#64218=DIRECTION('',(1.53134210293126E-15,1.,0.)) ;
#64219=DIRECTION('',(-1.,3.55271367880026E-13,9.05696233641872E-48)) ;
#64220=DIRECTION('center_axis',(-2.46519032881566E-32,4.52848116820976E-48,
1.)) ;
#64221=DIRECTION('ref_axis',(0.,1.,-4.52848116820976E-48)) ;
#64222=DIRECTION('',(0.,1.,-1.76085023486835E-33)) ;
#64223=DIRECTION('center_axis',(-2.46519032881571E-32,-5.98699295060652E-49,
1.)) ;
#64224=DIRECTION('ref_axis',(1.,-7.31836847501401E-110,2.46519032881571E-32)) ;
#64225=DIRECTION('',(1.,-1.26882631385732E-14,-1.27969293219661E-49)) ;
#64226=DIRECTION('center_axis',(-2.46519032881566E-32,1.7915701050753E-48,
1.)) ;
#64227=DIRECTION('ref_axis',(0.,-1.,1.7915701050753E-48)) ;
#64228=DIRECTION('',(0.,-1.,1.76085023486835E-33)) ;
#64229=DIRECTION('center_axis',(-2.46519032881571E-32,-4.87512283120816E-48,
1.)) ;
#64230=DIRECTION('ref_axis',(-1.,-3.7453410837561E-96,-2.46519032881571E-32)) ;
#64231=DIRECTION('',(-1.,-3.55271367880026E-13,5.47382212626845E-48)) ;
#64232=DIRECTION('',(0.,-1.,8.50065630626093E-34)) ;
#64233=DIRECTION('center_axis',(-0.707106781186488,-0.707106781186607,0.)) ;
#64234=DIRECTION('ref_axis',(-0.707106781186607,0.707106781186488,3.7126864764714E-32)) ;
#64235=DIRECTION('center_axis',(0.,0.,1.)) ;
#64236=DIRECTION('ref_axis',(-0.986303541071623,0.164940367616834,0.)) ;
#64237=DIRECTION('center_axis',(-0.720370089059342,-0.693589889479825,1.27963433459996E-13)) ;
#64238=DIRECTION('ref_axis',(0.693589889479825,-0.720370089059342,3.63922431499158E-30)) ;
#64239=DIRECTION('center_axis',(0.,0.,-1.)) ;
#64240=DIRECTION('ref_axis',(-0.498769364572801,-0.86673474659993,0.)) ;
#64241=DIRECTION('',(0.,0.,-1.)) ;
#64242=DIRECTION('',(0.,0.,1.)) ;
#64243=DIRECTION('center_axis',(0.,0.,1.)) ;
#64244=DIRECTION('ref_axis',(1.,0.,0.)) ;
#64245=DIRECTION('center_axis',(0.,0.,-1.)) ;
#64246=DIRECTION('ref_axis',(-0.977748097404052,0.209782406370878,0.)) ;
#64247=DIRECTION('center_axis',(0.,0.,1.)) ;
#64248=DIRECTION('ref_axis',(1.,0.,0.)) ;
#64249=DIRECTION('center_axis',(0.,1.,0.)) ;
#64250=DIRECTION('ref_axis',(0.,0.,1.)) ;
#64251=DIRECTION('center_axis',(0.,0.,-1.)) ;
#64252=DIRECTION('ref_axis',(-0.918360381793699,0.395745131557839,0.)) ;
#64253=DIRECTION('center_axis',(3.67742382159233E-14,1.,0.)) ;
#64254=DIRECTION('ref_axis',(0.707106781186548,-2.60033132154489E-14,0.707106781186548)) ;
#64255=DIRECTION('center_axis',(0.,-1.,0.)) ;
#64256=DIRECTION('ref_axis',(0.707106781186548,0.,0.707106781186548)) ;
#64257=DIRECTION('',(3.67742382159233E-14,1.,0.)) ;
#64258=DIRECTION('center_axis',(0.,0.,-1.)) ;
#64259=DIRECTION('ref_axis',(-1.,0.,0.)) ;
#64260=DIRECTION('',(0.,0.,1.)) ;
#64261=DIRECTION('center_axis',(0.,0.,-1.)) ;
#64262=DIRECTION('ref_axis',(-1.,3.55271367880053E-14,0.)) ;
#64263=DIRECTION('',(0.,0.,-1.)) ;
#64264=DIRECTION('center_axis',(0.,0.,1.)) ;
#64265=DIRECTION('ref_axis',(-0.707106781186519,0.707106781186576,0.)) ;
#64266=DIRECTION('',(0.,0.,-1.)) ;
#64267=DIRECTION('center_axis',(1.,-3.67742382159233E-14,0.)) ;
#64268=DIRECTION('ref_axis',(-3.67742382159233E-14,-1.,0.)) ;
#64269=DIRECTION('',(0.,0.,-1.)) ;
#64270=DIRECTION('',(-3.67742382159233E-14,-1.,0.)) ;
#64271=DIRECTION('',(0.,0.,-1.)) ;
#64272=DIRECTION('',(-3.67742382159233E-14,-1.,0.)) ;
#64273=DIRECTION('center_axis',(0.,-1.,0.)) ;
#64274=DIRECTION('ref_axis',(-1.,0.,0.)) ;
#64275=DIRECTION('',(0.,0.,-1.)) ;
#64276=DIRECTION('',(0.,0.,-1.)) ;
#64277=DIRECTION('',(1.,0.,-3.18850138855159E-46)) ;
#64278=DIRECTION('',(0.,0.,-1.)) ;
#64279=DIRECTION('center_axis',(-0.120859073829245,-0.847660295597975,-0.516589883311598)) ;
#64280=DIRECTION('ref_axis',(0.193100538836725,-0.530539370138308,0.825372739211936)) ;
#64281=DIRECTION('center_axis',(0.,0.,1.)) ;
#64282=DIRECTION('ref_axis',(1.,0.,0.)) ;
#64283=DIRECTION('center_axis',(0.,-1.,0.)) ;
#64284=DIRECTION('ref_axis',(0.,0.,1.)) ;
#64285=DIRECTION('center_axis',(0.642787609686577,-0.766044443118946,-1.14182016674851E-13)) ;
#64286=DIRECTION('ref_axis',(-0.766044443118946,-0.642787609686577,1.64598929132938E-30)) ;
#64287=DIRECTION('center_axis',(0.,-1.,-7.6997105554314E-34)) ;
#64288=DIRECTION('ref_axis',(0.707106781186548,-5.44451754691918E-34,0.707106781186548)) ;
#64289=DIRECTION('',(0.,-1.,-7.6997105554314E-34)) ;
#64290=DIRECTION('center_axis',(0.,1.,0.)) ;
#64291=DIRECTION('ref_axis',(0.,0.,1.)) ;
#64292=DIRECTION('',(0.,1.,7.6997105554314E-34)) ;
#64293=DIRECTION('center_axis',(-7.16300942304673E-47,7.6997105554314E-34,
-1.)) ;
#64294=DIRECTION('ref_axis',(-1.,0.,0.)) ;
#64295=DIRECTION('center_axis',(-0.707106781186725,0.70710678118637,0.)) ;
#64296=DIRECTION('ref_axis',(0.,0.,1.)) ;
#64297=DIRECTION('center_axis',(-7.16300942304673E-47,7.6997105554314E-34,
-1.)) ;
#64298=DIRECTION('ref_axis',(-0.923879532511266,-0.382683432365139,-2.94655166356992E-34)) ;
#64299=DIRECTION('center_axis',(7.16300942304673E-47,-7.6997105554314E-34,
1.)) ;
#64300=DIRECTION('ref_axis',(-0.923879532511267,-0.382683432365139,-2.94655166356992E-34)) ;
#64301=DIRECTION('center_axis',(-0.70710678118661,0.707106781186485,5.4445175469192E-34)) ;
#64302=DIRECTION('ref_axis',(0.499999999999923,0.500000000000011,0.707106781186594)) ;
#64303=DIRECTION('center_axis',(-0.707106781186548,0.707106781186548,0.)) ;
#64304=DIRECTION('ref_axis',(0.,0.,1.)) ;
#64305=DIRECTION('',(-0.70710678118661,0.707106781186485,5.4445175469192E-34)) ;
#64306=DIRECTION('',(0.70710678118661,-0.707106781186485,-5.4445175469192E-34)) ;
#64307=DIRECTION('center_axis',(-7.16300942304673E-47,7.6997105554314E-34,
-1.)) ;
#64308=DIRECTION('ref_axis',(-1.,0.,0.)) ;
#64309=DIRECTION('center_axis',(0.,1.,0.)) ;
#64310=DIRECTION('ref_axis',(0.,0.,1.)) ;
#64311=DIRECTION('center_axis',(7.16300942304673E-47,-7.6997105554314E-34,
1.)) ;
#64312=DIRECTION('ref_axis',(0.923879532511283,0.382683432365099,2.94655166356961E-34)) ;
#64313=DIRECTION('center_axis',(-7.16300942304673E-47,7.6997105554314E-34,
-1.)) ;
#64314=DIRECTION('ref_axis',(0.923879532511283,0.382683432365099,2.94655166356961E-34)) ;
#64315=DIRECTION('center_axis',(-1.20119700805775E-14,-1.,-7.6997105554314E-34)) ;
#64316=DIRECTION('ref_axis',(0.70710678118661,-8.49374549938702E-15,0.707106781186485)) ;
#64317=DIRECTION('',(1.20119700805775E-14,1.,7.6997105554314E-34)) ;
#64318=DIRECTION('',(-1.20119700805775E-14,-1.,-7.6997105554314E-34)) ;
#64319=DIRECTION('center_axis',(1.,-1.28403006865249E-14,-8.15167541035622E-47)) ;
#64320=DIRECTION('ref_axis',(-9.07946368791524E-15,-0.707106781186485,0.70710678118661)) ;
#64321=DIRECTION('',(1.,-1.28403006865249E-14,-8.15167541035622E-47)) ;
#64322=DIRECTION('center_axis',(-1.,0.,0.)) ;
#64323=DIRECTION('ref_axis',(0.,-1.,0.)) ;
#64324=DIRECTION('',(-1.,1.28403006865249E-14,8.15167541035622E-47)) ;
#64325=DIRECTION('center_axis',(-7.16300942304673E-47,7.6997105554314E-34,
-1.)) ;
#64326=DIRECTION('ref_axis',(-1.,0.,0.)) ;
#64327=DIRECTION('center_axis',(-0.64278760968649,0.76604444311902,0.)) ;
#64328=DIRECTION('ref_axis',(-0.76604444311902,-0.64278760968649,0.)) ;
#64329=DIRECTION('center_axis',(7.16300942304673E-47,-7.6997105554314E-34,
1.)) ;
#64330=DIRECTION('ref_axis',(0.42261826174077,0.906307787036617,6.97830763431521E-34)) ;
#64331=DIRECTION('center_axis',(-7.16300942304673E-47,7.6997105554314E-34,
-1.)) ;
#64332=DIRECTION('ref_axis',(0.42261826174077,0.906307787036617,6.97830763431521E-34)) ;
#64333=DIRECTION('center_axis',(0.642787609686599,-0.766044443118928,-5.89832048461284E-34)) ;
#64334=DIRECTION('ref_axis',(-0.541675220419631,-0.454519477672056,0.707106781186594)) ;
#64335=DIRECTION('',(-0.642787609686599,0.766044443118928,5.89832048461284E-34)) ;
#64336=DIRECTION('',(0.642787609686599,-0.766044443118928,-5.89832048461284E-34)) ;
#64337=DIRECTION('center_axis',(-0.95507414978076,-0.296366948934188,0.)) ;
#64338=DIRECTION('ref_axis',(-0.296366948934188,0.955074149780759,0.)) ;
#64339=DIRECTION('center_axis',(0.,-1.,0.)) ;
#64340=DIRECTION('ref_axis',(1.,0.,0.)) ;
#64341=DIRECTION('center_axis',(1.,-1.20119700805775E-14,0.)) ;
#64342=DIRECTION('ref_axis',(1.20119700805775E-14,1.,-5.57529378295193E-17)) ;
#64343=DIRECTION('center_axis',(0.,0.,1.)) ;
#64344=DIRECTION('ref_axis',(-0.76604444311902,-0.64278760968649,0.)) ;
#64345=DIRECTION('center_axis',(0.,0.,-1.)) ;
#64346=DIRECTION('ref_axis',(-1.,0.,0.)) ;
#64347=DIRECTION('center_axis',(0.,0.,-1.)) ;
#64348=DIRECTION('ref_axis',(-0.73407014073105,0.679073654684893,0.)) ;
#64349=DIRECTION('center_axis',(-0.996975386522573,-0.0777179430258286,
0.)) ;
#64350=DIRECTION('ref_axis',(0.0777179430258286,-0.996975386522573,0.)) ;
#64351=DIRECTION('center_axis',(-0.642787609686786,-0.766044443118771,0.)) ;
#64352=DIRECTION('ref_axis',(0.766044443118771,-0.642787609686786,0.)) ;
#64353=DIRECTION('center_axis',(0.,0.,1.)) ;
#64354=DIRECTION('ref_axis',(0.457543425680166,-0.889187277021471,0.)) ;
#64355=DIRECTION('center_axis',(0.642787609686516,0.766044443118998,0.)) ;
#64356=DIRECTION('ref_axis',(0.54167522041968,-0.454519477671997,0.707106781186594)) ;
#64357=DIRECTION('center_axis',(-0.642787609686577,-0.766044443118946,0.)) ;
#64358=DIRECTION('ref_axis',(0.766044443118946,-0.642787609686577,0.)) ;
#64359=DIRECTION('',(0.642787609686516,0.766044443118998,0.)) ;
#64360=DIRECTION('center_axis',(0.,0.,-1.)) ;
#64361=DIRECTION('ref_axis',(-1.,0.,0.)) ;
#64362=DIRECTION('center_axis',(3.55271367880058E-13,-1.,0.)) ;
#64363=DIRECTION('ref_axis',(1.,3.55271367880058E-13,0.)) ;
#64364=DIRECTION('center_axis',(0.,0.,1.)) ;
#64365=DIRECTION('ref_axis',(0.939692620785897,-0.3420201433257,0.)) ;
#64366=DIRECTION('center_axis',(-1.20119700805775E-14,-1.,0.)) ;
#64367=DIRECTION('ref_axis',(0.70710678118661,-8.49374549938702E-15,0.707106781186485)) ;
#64368=DIRECTION('',(1.20119700805775E-14,1.,0.)) ;
#64369=DIRECTION('center_axis',(0.,0.,-1.)) ;
#64370=DIRECTION('ref_axis',(0.342020143325632,-0.939692620785922,0.)) ;
#64371=DIRECTION('',(0.,0.,1.)) ;
#64372=DIRECTION('',(0.,0.,-1.)) ;
#64373=DIRECTION('center_axis',(-0.642787609686599,0.766044443118928,0.)) ;
#64374=DIRECTION('ref_axis',(0.541675220419631,0.454519477672056,-0.707106781186594)) ;
#64375=DIRECTION('center_axis',(-0.642787609686503,0.766044443119009,0.)) ;
#64376=DIRECTION('ref_axis',(0.766044443119009,0.642787609686503,0.)) ;
#64377=DIRECTION('',(-0.642787609686599,0.766044443118928,0.)) ;
#64378=DIRECTION('center_axis',(0.,0.,1.)) ;
#64379=DIRECTION('ref_axis',(1.,0.,0.)) ;
#64380=DIRECTION('center_axis',(-1.,1.7763568394006E-13,0.)) ;
#64381=DIRECTION('ref_axis',(1.7763568394006E-13,1.,0.)) ;
#64382=DIRECTION('center_axis',(0.,0.,1.)) ;
#64383=DIRECTION('ref_axis',(0.422618261740741,0.906307787036631,0.)) ;
#64384=DIRECTION('center_axis',(-1.,1.28403006865249E-14,0.)) ;
#64385=DIRECTION('ref_axis',(9.07946368791846E-15,0.707106781186736,-0.707106781186359)) ;
#64386=DIRECTION('center_axis',(-1.,0.,0.)) ;
#64387=DIRECTION('ref_axis',(0.,1.,0.)) ;
#64388=DIRECTION('',(-1.,1.28403006865249E-14,0.)) ;
#64389=DIRECTION('center_axis',(-7.16300942304673E-47,7.6997105554314E-34,
-1.)) ;
#64390=DIRECTION('ref_axis',(1.,7.82584617141943E-97,-7.16300942304673E-47)) ;
#64391=DIRECTION('',(-1.,0.,2.99489585516063E-33)) ;
#64392=DIRECTION('',(0.,-1.,2.39087358882206E-65)) ;
#64393=DIRECTION('center_axis',(-7.16300942304673E-47,7.6997105554314E-34,
-1.)) ;
#64394=DIRECTION('ref_axis',(1.,7.82584617141943E-97,-7.16300942304673E-47)) ;
#64395=DIRECTION('center_axis',(1.,0.,0.)) ;
#64396=DIRECTION('ref_axis',(0.,-1.,0.)) ;
#64397=DIRECTION('',(0.,0.,-1.)) ;
#64398=DIRECTION('',(0.,-1.,0.)) ;
#64399=DIRECTION('',(0.,-0.624695047554423,-0.780868809443031)) ;
#64400=DIRECTION('center_axis',(-1.,0.,0.)) ;
#64401=DIRECTION('ref_axis',(0.,0.624695047554423,0.780868809443031)) ;
#64402=DIRECTION('center_axis',(0.,0.,-1.)) ;
#64403=DIRECTION('ref_axis',(-0.707106781186437,-0.707106781186659,0.)) ;
#64404=DIRECTION('',(0.,0.,-1.)) ;
#64405=DIRECTION('center_axis',(0.,0.,1.)) ;
#64406=DIRECTION('ref_axis',(-0.923879532511266,-0.382683432365139,0.)) ;
#64407=DIRECTION('center_axis',(0.707106781186485,0.70710678118661,0.)) ;
#64408=DIRECTION('ref_axis',(0.70710678118661,-0.707106781186485,-2.64349870476783E-32)) ;
#64409=DIRECTION('',(0.,0.,1.)) ;
#64410=DIRECTION('',(0.70710678118661,-0.707106781186485,0.)) ;
#64411=DIRECTION('center_axis',(0.,0.,-1.)) ;
#64412=DIRECTION('ref_axis',(0.923879532511278,0.38268343236511,0.)) ;
#64413=DIRECTION('',(0.,0.,-1.)) ;
#64414=DIRECTION('center_axis',(0.,0.,-1.)) ;
#64415=DIRECTION('ref_axis',(0.923879532511283,0.382683432365099,0.)) ;
#64416=DIRECTION('center_axis',(1.,-1.20119700805775E-14,0.)) ;
#64417=DIRECTION('ref_axis',(-1.20119700805775E-14,-1.,2.16979082419566E-32)) ;
#64418=DIRECTION('',(0.,0.,-1.)) ;
#64419=DIRECTION('',(-1.13955553921264E-14,-0.948683298050513,-0.316227766016839)) ;
#64420=DIRECTION('center_axis',(1.,-1.20119700805775E-14,0.)) ;
#64421=DIRECTION('ref_axis',(-1.92410431043973E-15,-0.160182243006988,0.987087457637493)) ;
#64422=DIRECTION('',(-1.20119700805775E-14,-1.,0.)) ;
#64423=DIRECTION('center_axis',(-1.,1.20119700805775E-14,0.)) ;
#64424=DIRECTION('ref_axis',(4.59678193990225E-15,0.382683432365097,-0.923879532511284)) ;
#64425=DIRECTION('',(-8.49374549938626E-15,-0.707106781186546,-0.707106781186549)) ;
#64426=DIRECTION('center_axis',(1.,-1.20119700805775E-14,0.)) ;
#64427=DIRECTION('ref_axis',(-4.59678193990225E-15,-0.382683432365097,0.923879532511284)) ;
#64428=DIRECTION('',(-1.20119700805775E-14,-1.,0.)) ;
#64429=DIRECTION('center_axis',(0.,0.,-1.)) ;
#64430=DIRECTION('ref_axis',(1.,7.10542735760242E-14,0.)) ;
#64431=DIRECTION('',(0.,0.,-1.)) ;
#64432=DIRECTION('center_axis',(-1.14425202895153E-15,0.257662650560322,
-0.966234939601249)) ;
#64433=DIRECTION('ref_axis',(1.02982682605711E-13,-0.966234939601249,-0.257662650560322)) ;
#64434=DIRECTION('center_axis',(0.766044443118998,-0.642787609686516,0.)) ;
#64435=DIRECTION('ref_axis',(-0.642787609686516,-0.766044443118998,0.)) ;
#64436=DIRECTION('',(0.,0.,-1.)) ;
#64437=DIRECTION('',(-0.622803969959022,-0.742228868680647,-0.247409622893551)) ;
#64438=DIRECTION('center_axis',(0.,0.,-1.)) ;
#64439=DIRECTION('ref_axis',(0.766044443118867,-0.642787609686671,0.)) ;
#64440=DIRECTION('',(0.,0.,1.)) ;
#64441=DIRECTION('center_axis',(0.,0.16439898730545,-0.986393923832128)) ;
#64442=DIRECTION('ref_axis',(0.,-0.986393923832128,-0.16439898730545)) ;
#64443=DIRECTION('center_axis',(0.,0.,-1.)) ;
#64444=DIRECTION('ref_axis',(1.,0.,0.)) ;
#64445=DIRECTION('center_axis',(0.,0.,1.)) ;
#64446=DIRECTION('ref_axis',(-0.933145676371942,0.359498465460357,0.)) ;
#64447=DIRECTION('center_axis',(-2.08472420634511E-15,-0.344254649158429,
0.938876315886606)) ;
#64448=DIRECTION('ref_axis',(-7.36069948638338E-33,0.938876315886606,0.344254649158429)) ;
#64449=DIRECTION('center_axis',(0.,0.983937861384704,0.178511301977483)) ;
#64450=DIRECTION('ref_axis',(1.,0.,0.)) ;
#64451=DIRECTION('center_axis',(1.,0.,0.)) ;
#64452=DIRECTION('ref_axis',(0.,0.511844635310909,-0.85907803446686)) ;
#64453=DIRECTION('center_axis',(0.,0.,-1.)) ;
#64454=DIRECTION('ref_axis',(-0.707106781186359,-0.707106781186736,0.)) ;
#64455=DIRECTION('center_axis',(0.,0.,-1.)) ;
#64456=DIRECTION('ref_axis',(-0.707106781186359,-0.707106781186736,0.)) ;
#64457=DIRECTION('',(0.,0.,-1.)) ;
#64458=DIRECTION('',(0.,0.,1.)) ;
#64459=DIRECTION('center_axis',(0.,0.,1.)) ;
#64460=DIRECTION('ref_axis',(1.,0.,0.)) ;
#64461=DIRECTION('center_axis',(0.,0.,1.)) ;
#64462=DIRECTION('ref_axis',(-1.,0.,0.)) ;
#64463=DIRECTION('center_axis',(0.,-1.,0.)) ;
#64464=DIRECTION('ref_axis',(0.,0.,-1.)) ;
#64465=DIRECTION('center_axis',(0.,0.,-1.)) ;
#64466=DIRECTION('ref_axis',(-0.707106781186485,0.70710678118661,0.)) ;
#64467=DIRECTION('center_axis',(1.,0.,0.)) ;
#64468=DIRECTION('ref_axis',(0.,-1.,0.)) ;
#64469=DIRECTION('center_axis',(0.,-1.,0.)) ;
#64470=DIRECTION('ref_axis',(0.707106781186548,0.,-0.707106781186548)) ;
#64471=DIRECTION('center_axis',(0.,1.,0.)) ;
#64472=DIRECTION('ref_axis',(1.,0.,0.)) ;
#64473=DIRECTION('',(0.,1.,0.)) ;
#64474=DIRECTION('',(0.,-1.,0.)) ;
#64475=DIRECTION('center_axis',(-1.,0.,0.)) ;
#64476=DIRECTION('ref_axis',(0.,0.,1.)) ;
#64477=DIRECTION('center_axis',(1.,0.,0.)) ;
#64478=DIRECTION('ref_axis',(0.,-0.211920125136302,0.977286989866443)) ;
#64479=DIRECTION('center_axis',(-1.,0.,0.)) ;
#64480=DIRECTION('ref_axis',(0.,-0.211920125136302,0.977286989866444)) ;
#64481=DIRECTION('center_axis',(0.,0.,-1.)) ;
#64482=DIRECTION('ref_axis',(-1.,0.,0.)) ;
#64483=DIRECTION('center_axis',(0.,0.,-1.)) ;
#64484=DIRECTION('ref_axis',(0.707106781186485,0.70710678118661,0.)) ;
#64485=DIRECTION('center_axis',(0.,-1.,0.)) ;
#64486=DIRECTION('ref_axis',(-1.,0.,0.)) ;
#64487=DIRECTION('center_axis',(0.,0.,1.)) ;
#64488=DIRECTION('ref_axis',(0.,1.,0.)) ;
#64489=DIRECTION('center_axis',(-1.,0.,0.)) ;
#64490=DIRECTION('ref_axis',(0.,0.,-1.)) ;
#64491=DIRECTION('center_axis',(3.495649499231E-13,0.983937861384641,0.178511301977827)) ;
#64492=DIRECTION('ref_axis',(-1.96833879041829E-30,0.178511301977827,-0.983937861384641)) ;
#64493=DIRECTION('center_axis',(-1.,0.,0.)) ;
#64494=DIRECTION('ref_axis',(0.,1.,0.)) ;
#64495=DIRECTION('center_axis',(-1.,0.,0.)) ;
#64496=DIRECTION('ref_axis',(0.,0.,1.)) ;
#64497=DIRECTION('center_axis',(0.,-1.,0.)) ;
#64498=DIRECTION('ref_axis',(-1.,0.,0.)) ;
#64499=DIRECTION('center_axis',(1.,0.,0.)) ;
#64500=DIRECTION('ref_axis',(0.,-0.211920125136302,0.977286989866444)) ;
#64501=DIRECTION('center_axis',(-1.,0.,0.)) ;
#64502=DIRECTION('ref_axis',(0.,-0.211920125136302,0.977286989866443)) ;
#64503=DIRECTION('center_axis',(0.,1.,0.)) ;
#64504=DIRECTION('ref_axis',(-0.707106781186548,0.,-0.707106781186548)) ;
#64505=DIRECTION('',(0.,-1.,0.)) ;
#64506=DIRECTION('',(0.,1.,0.)) ;
#64507=DIRECTION('center_axis',(-1.,0.,0.)) ;
#64508=DIRECTION('ref_axis',(0.,0.869437932031723,-0.49404218680635)) ;
#64509=DIRECTION('center_axis',(1.,0.,0.)) ;
#64510=DIRECTION('ref_axis',(0.,0.511844635310909,-0.85907803446686)) ;
#64511=DIRECTION('',(1.,0.,0.)) ;
#64512=DIRECTION('',(-1.,0.,0.)) ;
#64513=DIRECTION('center_axis',(0.477592250328493,0.621251013257736,0.62125101283813)) ;
#64514=DIRECTION('ref_axis',(5.81314738453177E-17,0.70710678094775,-0.707106781425345)) ;
#64515=DIRECTION('center_axis',(0.,0.70710678118657,0.707106781186525)) ;
#64516=DIRECTION('ref_axis',(0.,0.707106781186525,-0.70710678118657)) ;
#64517=DIRECTION('center_axis',(0.,0.600000000000011,-0.799999999999992)) ;
#64518=DIRECTION('ref_axis',(0.,0.799999999999991,0.600000000000011)) ;
#64519=DIRECTION('center_axis',(-8.05175619837835E-16,0.707106781186546,
0.707106781186549)) ;
#64520=DIRECTION('ref_axis',(-0.707106781186594,0.499999999999968,-0.499999999999966)) ;
#64521=DIRECTION('',(-8.05175619837834E-16,0.707106781186546,0.707106781186549)) ;
#64522=DIRECTION('center_axis',(0.,0.,1.)) ;
#64523=DIRECTION('ref_axis',(0.707106781186359,-0.707106781186736,0.)) ;
#64524=DIRECTION('center_axis',(0.,0.,-1.)) ;
#64525=DIRECTION('ref_axis',(0.707106781186359,-0.707106781186736,0.)) ;
#64526=DIRECTION('',(0.,0.,-1.)) ;
#64527=DIRECTION('',(0.,0.,1.)) ;
#64528=DIRECTION('center_axis',(0.,0.,-1.)) ;
#64529=DIRECTION('ref_axis',(-1.,0.,0.)) ;
#64530=DIRECTION('center_axis',(1.,0.,0.)) ;
#64531=DIRECTION('ref_axis',(0.,0.,-1.)) ;
#64532=DIRECTION('center_axis',(0.,0.,1.)) ;
#64533=DIRECTION('ref_axis',(0.707106781186503,-0.707106781186592,0.)) ;
#64534=DIRECTION('center_axis',(-1.,0.,0.)) ;
#64535=DIRECTION('ref_axis',(0.,0.707106781186469,-0.707106781186626)) ;
#64536=DIRECTION('center_axis',(1.,0.,0.)) ;
#64537=DIRECTION('ref_axis',(0.,0.,-1.)) ;
#64538=DIRECTION('',(1.,0.,0.)) ;
#64539=DIRECTION('center_axis',(0.,0.,-1.)) ;
#64540=DIRECTION('ref_axis',(-1.,0.,0.)) ;
#64541=DIRECTION('center_axis',(0.,-1.,0.)) ;
#64542=DIRECTION('ref_axis',(0.,0.,-1.)) ;
#64543=DIRECTION('center_axis',(0.,0.,1.)) ;
#64544=DIRECTION('ref_axis',(-0.70710678118657,-0.707106781186525,0.)) ;
#64545=DIRECTION('center_axis',(5.69345140833415E-16,1.,0.)) ;
#64546=DIRECTION('ref_axis',(0.707106781186532,-4.02587809918909E-16,-0.707106781186563)) ;
#64547=DIRECTION('',(-5.69345140833415E-16,-1.,0.)) ;
#64548=DIRECTION('center_axis',(0.,0.,1.)) ;
#64549=DIRECTION('ref_axis',(0.707106781186359,0.707106781186736,0.)) ;
#64550=DIRECTION('center_axis',(0.,0.,-1.)) ;
#64551=DIRECTION('ref_axis',(0.707106781186359,0.707106781186736,0.)) ;
#64552=DIRECTION('',(0.,0.,-1.)) ;
#64553=DIRECTION('',(0.,0.,1.)) ;
#64554=DIRECTION('center_axis',(-1.,0.,0.)) ;
#64555=DIRECTION('ref_axis',(0.,-0.707106781186736,-0.707106781186359)) ;
#64556=DIRECTION('center_axis',(1.,0.,0.)) ;
#64557=DIRECTION('ref_axis',(0.,-1.,0.)) ;
#64558=DIRECTION('',(1.,0.,0.)) ;
#64559=DIRECTION('',(-1.,0.,0.)) ;
#64560=DIRECTION('center_axis',(0.,0.,1.)) ;
#64561=DIRECTION('ref_axis',(1.,0.,0.)) ;
#64562=DIRECTION('center_axis',(0.,-1.,0.)) ;
#64563=DIRECTION('ref_axis',(-1.,0.,0.)) ;
#64564=DIRECTION('center_axis',(0.,0.,1.)) ;
#64565=DIRECTION('ref_axis',(-0.707106781186559,-0.707106781186536,0.)) ;
#64566=DIRECTION('center_axis',(0.,0.,-1.)) ;
#64567=DIRECTION('ref_axis',(-0.707106781186559,-0.707106781186536,0.)) ;
#64568=DIRECTION('center_axis',(-1.13869028166683E-15,1.,0.)) ;
#64569=DIRECTION('ref_axis',(-0.707106781186548,-8.05175619837835E-16,-0.707106781186548)) ;
#64570=DIRECTION('center_axis',(0.,-1.,0.)) ;
#64571=DIRECTION('ref_axis',(-1.,0.,0.)) ;
#64572=DIRECTION('',(1.13869028166683E-15,-1.,0.)) ;
#64573=DIRECTION('',(-1.13869028166683E-15,1.,0.)) ;
#64574=DIRECTION('center_axis',(0.,0.,1.)) ;
#64575=DIRECTION('ref_axis',(1.,0.,0.)) ;
#64576=DIRECTION('center_axis',(1.,0.,0.)) ;
#64577=DIRECTION('ref_axis',(0.,-1.,0.)) ;
#64578=DIRECTION('center_axis',(0.,0.,-1.)) ;
#64579=DIRECTION('ref_axis',(0.70710678118657,0.707106781186525,0.)) ;
#64580=DIRECTION('center_axis',(0.,0.,1.)) ;
#64581=DIRECTION('ref_axis',(0.70710678118657,0.707106781186525,0.)) ;
#64582=DIRECTION('center_axis',(-1.,-6.125368411725E-15,0.)) ;
#64583=DIRECTION('ref_axis',(4.33128954119624E-15,-0.707106781186485,-0.70710678118661)) ;
#64584=DIRECTION('center_axis',(1.,0.,0.)) ;
#64585=DIRECTION('ref_axis',(0.,-1.,0.)) ;
#64586=DIRECTION('',(1.,6.125368411725E-15,0.)) ;
#64587=DIRECTION('',(-1.,-6.125368411725E-15,0.)) ;
#64588=DIRECTION('center_axis',(0.,0.,1.)) ;
#64589=DIRECTION('ref_axis',(1.,0.,0.)) ;
#64590=DIRECTION('center_axis',(0.,1.,0.)) ;
#64591=DIRECTION('ref_axis',(1.,0.,0.)) ;
#64592=DIRECTION('center_axis',(0.,0.,-1.)) ;
#64593=DIRECTION('ref_axis',(-0.707106781186514,0.707106781186581,0.)) ;
#64594=DIRECTION('center_axis',(0.,0.,1.)) ;
#64595=DIRECTION('ref_axis',(-0.707106781186514,0.707106781186581,0.)) ;
#64596=DIRECTION('center_axis',(-5.69345140833415E-16,-1.,0.)) ;
#64597=DIRECTION('ref_axis',(0.707106781186548,-4.02587809918918E-16,-0.707106781186548)) ;
#64598=DIRECTION('center_axis',(0.,1.,0.)) ;
#64599=DIRECTION('ref_axis',(1.,0.,0.)) ;
#64600=DIRECTION('',(5.69345140833415E-16,1.,0.)) ;
#64601=DIRECTION('',(-5.69345140833415E-16,-1.,0.)) ;
#64602=DIRECTION('center_axis',(0.,0.,1.)) ;
#64603=DIRECTION('ref_axis',(1.,0.,0.)) ;
#64604=DIRECTION('center_axis',(1.,0.,0.)) ;
#64605=DIRECTION('ref_axis',(0.,-1.,0.)) ;
#64606=DIRECTION('center_axis',(0.,0.,1.)) ;
#64607=DIRECTION('ref_axis',(0.707106781186553,-0.707106781186542,0.)) ;
#64608=DIRECTION('center_axis',(0.,0.,-1.)) ;
#64609=DIRECTION('ref_axis',(0.707106781186553,-0.707106781186542,0.)) ;
#64610=DIRECTION('center_axis',(-1.,0.,0.)) ;
#64611=DIRECTION('ref_axis',(0.,-0.707106781186736,-0.707106781186359)) ;
#64612=DIRECTION('',(1.,0.,0.)) ;
#64613=DIRECTION('',(-1.,0.,0.)) ;
#64614=DIRECTION('center_axis',(1.,0.,0.)) ;
#64615=DIRECTION('ref_axis',(0.,0.869437932031723,-0.49404218680635)) ;
#64616=DIRECTION('center_axis',(-1.,0.,0.)) ;
#64617=DIRECTION('ref_axis',(0.,1.,0.)) ;
#64618=DIRECTION('',(-1.,0.,0.)) ;
#64619=DIRECTION('',(1.,0.,0.)) ;
#64620=DIRECTION('center_axis',(-0.477592250328042,0.621251013257686,0.621251012838527)) ;
#64621=DIRECTION('ref_axis',(0.792804743230373,0.60947570838502,-1.22539280089609E-16)) ;
#64622=DIRECTION('center_axis',(0.,0.600000000000011,-0.799999999999992)) ;
#64623=DIRECTION('ref_axis',(0.,0.799999999999991,0.600000000000011)) ;
#64624=DIRECTION('center_axis',(0.,0.,1.)) ;
#64625=DIRECTION('ref_axis',(-0.707106781186359,0.707106781186736,0.)) ;
#64626=DIRECTION('center_axis',(0.,0.,-1.)) ;
#64627=DIRECTION('ref_axis',(-0.707106781186359,0.707106781186736,0.)) ;
#64628=DIRECTION('',(0.,0.,-1.)) ;
#64629=DIRECTION('',(0.,0.,1.)) ;
#64630=DIRECTION('center_axis',(-1.,0.,0.)) ;
#64631=DIRECTION('ref_axis',(0.,-0.382683432365103,0.923879532511281)) ;
#64632=DIRECTION('center_axis',(1.,1.24744160070242E-15,0.)) ;
#64633=DIRECTION('ref_axis',(4.77375233431813E-16,-0.382683432365097,0.923879532511284)) ;
#64634=DIRECTION('',(1.,0.,0.)) ;
#64635=DIRECTION('center_axis',(-1.,0.,0.)) ;
#64636=DIRECTION('ref_axis',(0.,-0.382683432365103,0.923879532511281)) ;
#64637=DIRECTION('',(1.,0.,0.)) ;
#64638=DIRECTION('center_axis',(0.,0.,-1.)) ;
#64639=DIRECTION('ref_axis',(-0.707106781186548,0.707106781186548,0.)) ;
#64640=DIRECTION('',(0.,0.,1.)) ;
#64641=DIRECTION('center_axis',(0.,0.,1.)) ;
#64642=DIRECTION('ref_axis',(-0.707106781186548,0.707106781186548,0.)) ;
#64643=DIRECTION('',(0.,0.,-1.)) ;
#64644=DIRECTION('center_axis',(0.,0.,-1.)) ;
#64645=DIRECTION('ref_axis',(1.,0.,0.)) ;
#64646=DIRECTION('',(0.,0.,-1.)) ;
#64647=DIRECTION('',(0.,0.,-1.)) ;
#64648=DIRECTION('center_axis',(0.,1.,0.)) ;
#64649=DIRECTION('ref_axis',(1.,0.,-1.93235546378459E-35)) ;
#64650=DIRECTION('',(0.,0.,-1.)) ;
#64651=DIRECTION('center_axis',(0.,0.,-1.)) ;
#64652=DIRECTION('ref_axis',(0.,-1.,0.)) ;
#64653=DIRECTION('',(0.,0.,-1.)) ;
#64654=DIRECTION('center_axis',(0.,0.,1.)) ;
#64655=DIRECTION('ref_axis',(0.707106781186548,0.707106781186548,0.)) ;
#64656=DIRECTION('',(0.,0.,1.)) ;
#64657=DIRECTION('center_axis',(0.,0.,1.)) ;
#64658=DIRECTION('ref_axis',(0.707106781186548,0.707106781186548,0.)) ;
#64659=DIRECTION('',(0.,0.,-1.)) ;
#64660=DIRECTION('center_axis',(-1.,-1.13869028166683E-15,0.)) ;
#64661=DIRECTION('ref_axis',(-1.13869028166683E-15,1.,0.)) ;
#64662=DIRECTION('',(0.,0.,-1.)) ;
#64663=DIRECTION('',(0.,0.,-1.)) ;
#64664=DIRECTION('',(1.13869028166683E-15,-1.,0.)) ;
#64665=DIRECTION('center_axis',(0.,-1.,0.)) ;
#64666=DIRECTION('ref_axis',(1.,0.,0.)) ;
#64667=DIRECTION('',(1.,0.,0.)) ;
#64668=DIRECTION('center_axis',(1.,-5.69345140833415E-16,0.)) ;
#64669=DIRECTION('ref_axis',(-5.69345140833415E-16,-1.,3.47655046371441E-32)) ;
#64670=DIRECTION('',(5.69345140833415E-16,1.,0.)) ;
#64671=DIRECTION('',(0.,0.,1.)) ;
#64672=DIRECTION('',(0.,0.,-1.)) ;
#64673=DIRECTION('center_axis',(-1.,0.,0.)) ;
#64674=DIRECTION('ref_axis',(0.,-1.,0.)) ;
#64675=DIRECTION('',(0.,-1.,0.)) ;
#64676=DIRECTION('center_axis',(0.,0.,1.)) ;
#64677=DIRECTION('ref_axis',(1.,0.,0.)) ;
#64678=DIRECTION('',(-1.,0.,0.)) ;
#64679=DIRECTION('center_axis',(0.,0.,1.)) ;
#64680=DIRECTION('ref_axis',(0.707106781186555,-0.70710678118654,0.)) ;
#64681=DIRECTION('center_axis',(0.,0.,1.)) ;
#64682=DIRECTION('ref_axis',(-0.70710678118661,0.707106781186485,0.)) ;
#64683=DIRECTION('center_axis',(0.,0.,-1.)) ;
#64684=DIRECTION('ref_axis',(-0.70710678118661,0.707106781186485,0.)) ;
#64685=DIRECTION('',(0.,0.,1.)) ;
#64686=DIRECTION('center_axis',(0.,0.,1.)) ;
#64687=DIRECTION('ref_axis',(-0.70710678118661,0.707106781186485,0.)) ;
#64688=DIRECTION('',(0.,0.,-1.)) ;
#64689=DIRECTION('center_axis',(-1.,0.,0.)) ;
#64690=DIRECTION('ref_axis',(0.,-1.,0.)) ;
#64691=DIRECTION('',(0.,1.,0.)) ;
#64692=DIRECTION('',(0.,0.,-1.)) ;
#64693=DIRECTION('',(0.,-1.,0.)) ;
#64694=DIRECTION('center_axis',(0.,0.,-1.)) ;
#64695=DIRECTION('ref_axis',(-0.707106781186359,-0.707106781186736,0.)) ;
#64696=DIRECTION('center_axis',(0.,0.,1.)) ;
#64697=DIRECTION('ref_axis',(-0.707106781186359,-0.707106781186736,0.)) ;
#64698=DIRECTION('center_axis',(0.,0.,-1.)) ;
#64699=DIRECTION('ref_axis',(-0.707106781186359,-0.707106781186736,0.)) ;
#64700=DIRECTION('',(0.,0.,1.)) ;
#64701=DIRECTION('center_axis',(-1.,0.,0.)) ;
#64702=DIRECTION('ref_axis',(0.,0.,1.)) ;
#64703=DIRECTION('center_axis',(-1.,-1.24744160070242E-15,0.)) ;
#64704=DIRECTION('ref_axis',(-8.8207441499096E-16,0.70710678118661,0.707106781186485)) ;
#64705=DIRECTION('center_axis',(0.,0.,-1.)) ;
#64706=DIRECTION('ref_axis',(0.,-1.,0.)) ;
#64707=DIRECTION('center_axis',(1.,0.,0.)) ;
#64708=DIRECTION('ref_axis',(0.,0.,1.)) ;
#64709=DIRECTION('center_axis',(0.,-1.,0.)) ;
#64710=DIRECTION('ref_axis',(-1.,0.,0.)) ;
#64711=DIRECTION('center_axis',(1.,0.,0.)) ;
#64712=DIRECTION('ref_axis',(0.,0.,-1.)) ;
#64713=DIRECTION('center_axis',(1.,0.,0.)) ;
#64714=DIRECTION('ref_axis',(0.,1.,0.)) ;
#64715=DIRECTION('center_axis',(0.,0.,1.)) ;
#64716=DIRECTION('ref_axis',(-1.,0.,0.)) ;
#64717=DIRECTION('center_axis',(-1.,-1.24744160070242E-15,0.)) ;
#64718=DIRECTION('ref_axis',(-8.82074414991118E-16,0.707106781186736,-0.707106781186359)) ;
#64719=DIRECTION('center_axis',(0.,-1.,0.)) ;
#64720=DIRECTION('ref_axis',(0.,0.,1.)) ;
#64721=DIRECTION('center_axis',(0.,0.,1.)) ;
#64722=DIRECTION('ref_axis',(-0.70710678118661,-0.707106781186485,0.)) ;
#64723=DIRECTION('',(0.,0.,-1.)) ;
#64724=DIRECTION('',(0.,0.,1.)) ;
#64725=DIRECTION('center_axis',(-1.,8.30329439001789E-15,0.)) ;
#64726=DIRECTION('ref_axis',(-5.87131576937143E-15,-0.707106781186736,0.707106781186359)) ;
#64727=DIRECTION('center_axis',(1.,0.,0.)) ;
#64728=DIRECTION('ref_axis',(0.,0.,1.)) ;
#64729=DIRECTION('',(1.,-8.30329439001789E-15,0.)) ;
#64730=DIRECTION('center_axis',(1.,0.,0.)) ;
#64731=DIRECTION('ref_axis',(0.,-0.707106781186736,0.707106781186359)) ;
#64732=DIRECTION('',(-1.,8.30329439001789E-15,0.)) ;
#64733=DIRECTION('center_axis',(0.,0.,-1.)) ;
#64734=DIRECTION('ref_axis',(-1.,0.,0.)) ;
#64735=DIRECTION('center_axis',(0.,-1.,0.)) ;
#64736=DIRECTION('ref_axis',(0.,0.,1.)) ;
#64737=DIRECTION('center_axis',(0.,0.,1.)) ;
#64738=DIRECTION('ref_axis',(-0.707106781186548,-0.707106781186548,0.)) ;
#64739=DIRECTION('center_axis',(0.,0.,-1.)) ;
#64740=DIRECTION('ref_axis',(-0.707106781186547,-0.707106781186547,0.)) ;
#64741=DIRECTION('center_axis',(-1.24744160070242E-15,1.,0.)) ;
#64742=DIRECTION('ref_axis',(-0.707106781186548,-8.82074414990883E-16,0.707106781186548)) ;
#64743=DIRECTION('',(1.24744160070242E-15,-1.,0.)) ;
#64744=DIRECTION('',(-1.24744160070242E-15,1.,0.)) ;
#64745=DIRECTION('center_axis',(1.,0.,0.)) ;
#64746=DIRECTION('ref_axis',(0.,0.707106781186736,-0.707106781186359)) ;
#64747=DIRECTION('center_axis',(-1.,0.,0.)) ;
#64748=DIRECTION('ref_axis',(0.,0.707106781186736,-0.707106781186359)) ;
#64749=DIRECTION('',(-1.,0.,0.)) ;
#64750=DIRECTION('',(1.,0.,0.)) ;
#64751=DIRECTION('center_axis',(1.,0.,0.)) ;
#64752=DIRECTION('ref_axis',(0.,0.707106781186485,0.70710678118661)) ;
#64753=DIRECTION('center_axis',(-1.,0.,0.)) ;
#64754=DIRECTION('ref_axis',(0.,0.707106781186485,0.70710678118661)) ;
#64755=DIRECTION('',(-1.,0.,0.)) ;
#64756=DIRECTION('',(1.,0.,0.)) ;
#64757=DIRECTION('center_axis',(1.24744160070242E-15,-1.,0.)) ;
#64758=DIRECTION('ref_axis',(-0.707106781186548,-8.82074414990883E-16,-0.707106781186548)) ;
#64759=DIRECTION('center_axis',(0.,1.,0.)) ;
#64760=DIRECTION('ref_axis',(0.,0.,-1.)) ;
#64761=DIRECTION('',(-1.24744160070242E-15,1.,0.)) ;
#64762=DIRECTION('',(1.24744160070242E-15,-1.,0.)) ;
#64763=DIRECTION('center_axis',(0.,0.,1.)) ;
#64764=DIRECTION('ref_axis',(1.,0.,0.)) ;
#64765=DIRECTION('center_axis',(-1.,4.44089209850151E-14,0.)) ;
#64766=DIRECTION('ref_axis',(0.,0.,-1.)) ;
#64767=DIRECTION('center_axis',(0.,0.,-1.)) ;
#64768=DIRECTION('ref_axis',(-0.707106781186539,-0.707106781186556,0.)) ;
#64769=DIRECTION('center_axis',(0.,0.,1.)) ;
#64770=DIRECTION('ref_axis',(-0.707106781186539,-0.707106781186556,0.)) ;
#64771=DIRECTION('center_axis',(1.,-8.30329439001789E-15,0.)) ;
#64772=DIRECTION('ref_axis',(-5.87131576937143E-15,-0.707106781186736,-0.707106781186359)) ;
#64773=DIRECTION('center_axis',(1.,0.,0.)) ;
#64774=DIRECTION('ref_axis',(0.,-0.707106781186736,-0.707106781186359)) ;
#64775=DIRECTION('',(-1.,8.30329439001789E-15,0.)) ;
#64776=DIRECTION('',(1.,-8.30329439001789E-15,0.)) ;
#64777=DIRECTION('center_axis',(0.,0.,-1.)) ;
#64778=DIRECTION('ref_axis',(-4.44089209850056E-14,-1.,0.)) ;
#64779=DIRECTION('',(0.,0.,-1.)) ;
#64780=DIRECTION('center_axis',(0.,0.,-1.)) ;
#64781=DIRECTION('ref_axis',(-0.707106781186548,-0.707106781186548,0.)) ;
#64782=DIRECTION('',(0.,0.,-1.)) ;
#64783=DIRECTION('center_axis',(-1.,-1.24744160070242E-15,0.)) ;
#64784=DIRECTION('ref_axis',(-1.24744160070242E-15,1.,-3.26886029821929E-63)) ;
#64785=DIRECTION('',(0.,0.,-1.)) ;
#64786=DIRECTION('',(1.24744160070242E-15,-1.,-1.96585022416868E-45)) ;
#64787=DIRECTION('center_axis',(1.,1.24744160070242E-15,0.)) ;
#64788=DIRECTION('ref_axis',(-8.82074414990876E-16,0.707106781186542,0.707106781186553)) ;
#64789=DIRECTION('',(0.,0.,1.)) ;
#64790=DIRECTION('',(-7.79270590072164E-16,0.624695047554423,0.780868809443031)) ;
#64791=DIRECTION('center_axis',(1.,1.24744160070242E-15,0.)) ;
#64792=DIRECTION('ref_axis',(-5.40377643367589E-16,0.433188730489114,-0.901303236306866)) ;
#64793=DIRECTION('',(-1.24744160070242E-15,1.,0.)) ;
#64794=DIRECTION('center_axis',(-1.,-1.24744160070242E-15,0.)) ;
#64795=DIRECTION('ref_axis',(4.77375233431813E-16,-0.382683432365097,0.923879532511284)) ;
#64796=DIRECTION('',(-8.82074414990881E-16,0.707106781186546,0.707106781186549)) ;
#64797=DIRECTION('center_axis',(1.,1.24744160070242E-15,0.)) ;
#64798=DIRECTION('ref_axis',(-4.77375233431814E-16,0.382683432365098,-0.923879532511283)) ;
#64799=DIRECTION('',(-1.24744160070242E-15,1.,0.)) ;
#64800=DIRECTION('center_axis',(0.,0.,-1.)) ;
#64801=DIRECTION('ref_axis',(-4.44089209850056E-14,-1.,0.)) ;
#64802=DIRECTION('',(0.,0.,-1.)) ;
#64803=DIRECTION('center_axis',(-1.95689141014107E-45,-1.96585022416868E-45,
1.)) ;
#64804=DIRECTION('ref_axis',(-0.707106781186548,-0.707106781186548,-2.77379721046322E-45)) ;
#64805=DIRECTION('center_axis',(-8.30329439001789E-15,-1.,0.)) ;
#64806=DIRECTION('ref_axis',(-1.,8.30329439001789E-15,4.19778536698447E-50)) ;
#64807=DIRECTION('',(-1.,8.30329439001789E-15,0.)) ;
#64808=DIRECTION('',(0.,0.,1.)) ;
#64809=DIRECTION('',(1.,-9.87859509815899E-15,0.)) ;
#64810=DIRECTION('',(0.,0.,-1.)) ;
#64811=DIRECTION('',(1.,-8.30329439001789E-15,1.95689141014106E-45)) ;
#64812=DIRECTION('',(0.,0.,-1.)) ;
#64813=DIRECTION('',(-1.,8.30329439001789E-15,0.)) ;
#64814=DIRECTION('center_axis',(0.,-1.,0.)) ;
#64815=DIRECTION('ref_axis',(0.707106781186548,0.,-0.707106781186548)) ;
#64816=DIRECTION('center_axis',(0.,1.,0.)) ;
#64817=DIRECTION('ref_axis',(1.,0.,0.)) ;
#64818=DIRECTION('',(0.,1.,0.)) ;
#64819=DIRECTION('center_axis',(-1.92374441038943E-14,-0.901303236306783,
-0.433188730489285)) ;
#64820=DIRECTION('ref_axis',(-4.00259042046792E-14,0.433188730489285,-0.901303236306783)) ;
#64821=DIRECTION('center_axis',(0.,0.624695047554251,0.780868809443169)) ;
#64822=DIRECTION('ref_axis',(1.,0.,0.)) ;
#64823=DIRECTION('center_axis',(0.993839018553024,0.0692369708135714,0.0865462135169529)) ;
#64824=DIRECTION('ref_axis',(-0.110833231485694,0.620846312956424,0.77605789119553)) ;
#64825=DIRECTION('center_axis',(0.,-0.624695047554423,-0.780868809443031)) ;
#64826=DIRECTION('ref_axis',(0.707106781186373,0.55215763037437,-0.441726104299494)) ;
#64827=DIRECTION('',(0.,0.624695047554423,0.780868809443031)) ;
#64828=DIRECTION('center_axis',(0.,0.,1.)) ;
#64829=DIRECTION('ref_axis',(1.,0.,0.)) ;
#64830=DIRECTION('center_axis',(-0.707106781186725,0.70710678118637,0.)) ;
#64831=DIRECTION('ref_axis',(0.70710678118637,0.707106781186725,0.)) ;
#64832=DIRECTION('center_axis',(0.,0.,-1.)) ;
#64833=DIRECTION('ref_axis',(-0.923879532511267,-0.382683432365139,0.)) ;
#64834=DIRECTION('center_axis',(0.70710678118661,-0.707106781186485,0.)) ;
#64835=DIRECTION('ref_axis',(0.499999999999892,0.49999999999998,-0.707106781186638)) ;
#64836=DIRECTION('center_axis',(-0.707106781186548,0.707106781186548,0.)) ;
#64837=DIRECTION('ref_axis',(0.707106781186547,0.707106781186547,0.)) ;
#64838=DIRECTION('',(-0.70710678118661,0.707106781186485,0.)) ;
#64839=DIRECTION('center_axis',(0.,0.,1.)) ;
#64840=DIRECTION('ref_axis',(1.,0.,0.)) ;
#64841=DIRECTION('center_axis',(0.,1.,0.)) ;
#64842=DIRECTION('ref_axis',(1.,0.,0.)) ;
#64843=DIRECTION('center_axis',(0.,0.,1.)) ;
#64844=DIRECTION('ref_axis',(0.923879532511283,0.382683432365099,0.)) ;
#64845=DIRECTION('center_axis',(-1.20119700805775E-14,-1.,0.)) ;
#64846=DIRECTION('ref_axis',(0.70710678118661,-8.49374549938702E-15,-0.707106781186485)) ;
#64847=DIRECTION('center_axis',(0.,1.,0.)) ;
#64848=DIRECTION('ref_axis',(1.,0.,0.)) ;
#64849=DIRECTION('',(1.20119700805775E-14,1.,0.)) ;
#64850=DIRECTION('center_axis',(1.,-1.20119700805775E-14,0.)) ;
#64851=DIRECTION('ref_axis',(0.,0.,-1.)) ;
#64852=DIRECTION('center_axis',(0.,0.707106781186548,0.707106781186548)) ;
#64853=DIRECTION('ref_axis',(1.,0.,0.)) ;
#64854=DIRECTION('center_axis',(-1.,1.20119700805775E-14,0.)) ;
#64855=DIRECTION('ref_axis',(-4.59678193990225E-15,-0.382683432365097,0.923879532511284)) ;
#64856=DIRECTION('center_axis',(-8.49374549938626E-15,-0.707106781186546,
-0.707106781186549)) ;
#64857=DIRECTION('ref_axis',(0.707106781186531,0.500000000000009,-0.500000000000015)) ;
#64858=DIRECTION('center_axis',(0.,0.707106781186503,0.707106781186592)) ;
#64859=DIRECTION('ref_axis',(1.,0.,0.)) ;
#64860=DIRECTION('',(8.49374549938626E-15,0.707106781186546,0.707106781186549)) ;
#64861=DIRECTION('center_axis',(-1.,1.20119700805775E-14,0.)) ;
#64862=DIRECTION('ref_axis',(0.,0.,1.)) ;
#64863=DIRECTION('center_axis',(0.,1.,0.)) ;
#64864=DIRECTION('ref_axis',(1.,0.,0.)) ;
#64865=DIRECTION('center_axis',(1.,-1.20119700805775E-14,0.)) ;
#64866=DIRECTION('ref_axis',(4.59678193990225E-15,0.382683432365097,-0.923879532511284)) ;
#64867=DIRECTION('center_axis',(-1.20119700805775E-14,-1.,0.)) ;
#64868=DIRECTION('ref_axis',(0.707106781186469,-8.49374549938533E-15,-0.707106781186626)) ;
#64869=DIRECTION('center_axis',(0.,1.,0.)) ;
#64870=DIRECTION('ref_axis',(1.,0.,0.)) ;
#64871=DIRECTION('',(1.20119700805775E-14,1.,0.)) ;
#64872=DIRECTION('center_axis',(1.,-1.20119700805775E-14,0.)) ;
#64873=DIRECTION('ref_axis',(0.,0.,-1.)) ;
#64874=DIRECTION('center_axis',(0.,0.948683298050458,0.316227766017004)) ;
#64875=DIRECTION('ref_axis',(1.,0.,0.)) ;
#64876=DIRECTION('center_axis',(-1.,1.20119700805775E-14,0.)) ;
#64877=DIRECTION('ref_axis',(-1.92410431043973E-15,-0.160182243006988,0.987087457637493)) ;
#64878=DIRECTION('center_axis',(-1.13955553921264E-14,-0.948683298050513,
-0.316227766016839)) ;
#64879=DIRECTION('ref_axis',(0.707106781186476,0.223606797749995,-0.670820393250007)) ;
#64880=DIRECTION('center_axis',(0.,0.948683298050465,0.316227766016985)) ;
#64881=DIRECTION('ref_axis',(1.,0.,0.)) ;
#64882=DIRECTION('',(1.13955553921264E-14,0.948683298050513,0.316227766016839)) ;
#64883=DIRECTION('center_axis',(0.622803969958969,0.742228868680653,0.247409622893667)) ;
#64884=DIRECTION('ref_axis',(0.76604444311902,-0.64278760968649,4.44819739379099E-14)) ;
#64885=DIRECTION('center_axis',(-1.37008135359091E-15,-0.316227766016839,
0.948683298050513)) ;
#64886=DIRECTION('ref_axis',(6.7408002596686E-14,-0.948683298050513,-0.316227766016839)) ;
#64887=DIRECTION('center_axis',(-0.622803969959022,-0.742228868680647,-0.247409622893551)) ;
#64888=DIRECTION('ref_axis',(0.606851800616499,-0.258697038951143,-0.751536249376186)) ;
#64889=DIRECTION('center_axis',(0.622803969958982,0.742228868680643,0.247409622893663)) ;
#64890=DIRECTION('ref_axis',(0.76604444311902,-0.642787609686489,-2.20979765740922E-14)) ;
#64891=DIRECTION('',(0.622803969959022,0.742228868680647,0.247409622893551)) ;
#64892=DIRECTION('center_axis',(0.996641009831356,0.0776918771178938,0.025897292372644)) ;
#64893=DIRECTION('ref_axis',(0.0777179430258286,-0.996975386522573,-4.44097402191553E-14)) ;
#64894=DIRECTION('center_axis',(-1.37008135359091E-15,-0.316227766016839,
0.948683298050513)) ;
#64895=DIRECTION('ref_axis',(-3.86740249272492E-15,-0.948683298050513,-0.316227766016839)) ;
#64896=DIRECTION('center_axis',(0.781110574983513,0.592350945541578,0.197450315180618)) ;
#64897=DIRECTION('ref_axis',(0.604246815762238,-0.796797204840226,-2.22012953032117E-14)) ;
#64898=DIRECTION('center_axis',(1.37008135359091E-15,0.316227766016839,
-0.948683298050513)) ;
#64899=DIRECTION('ref_axis',(6.51683787482125E-33,0.948683298050513,0.316227766016839)) ;
#64900=DIRECTION('center_axis',(0.609935343346627,0.792451182683597,-8.98660408355326E-10)) ;
#64901=DIRECTION('ref_axis',(0.792451182683597,-0.609935343346627,1.791498019765E-26)) ;
#64902=DIRECTION('center_axis',(0.,0.,-1.)) ;
#64903=DIRECTION('ref_axis',(-1.,0.,0.)) ;
#64904=DIRECTION('center_axis',(0.,1.,0.)) ;
#64905=DIRECTION('ref_axis',(1.,0.,0.)) ;
#64906=DIRECTION('center_axis',(0.,-1.,0.)) ;
#64907=DIRECTION('ref_axis',(0.707106781186469,0.,-0.707106781186626)) ;
#64908=DIRECTION('center_axis',(0.,1.,0.)) ;
#64909=DIRECTION('ref_axis',(1.,0.,0.)) ;
#64910=DIRECTION('center_axis',(0.,0.,-1.)) ;
#64911=DIRECTION('ref_axis',(-1.,0.,0.)) ;
#64912=DIRECTION('center_axis',(0.707106781186459,0.707106781186636,0.)) ;
#64913=DIRECTION('ref_axis',(0.707106781186636,-0.707106781186459,0.)) ;
#64914=DIRECTION('center_axis',(0.,0.,-1.)) ;
#64915=DIRECTION('ref_axis',(0.923879532511297,-0.382683432365064,0.)) ;
#64916=DIRECTION('center_axis',(-0.70710678118654,-0.707106781186555,0.)) ;
#64917=DIRECTION('ref_axis',(0.499999999999993,-0.499999999999982,-0.707106781186565)) ;
#64918=DIRECTION('center_axis',(0.707106781186459,0.707106781186636,0.)) ;
#64919=DIRECTION('ref_axis',(0.707106781186636,-0.707106781186459,0.)) ;
#64920=DIRECTION('',(-0.70710678118654,-0.707106781186555,0.)) ;
#64921=DIRECTION('center_axis',(0.,0.,1.)) ;
#64922=DIRECTION('ref_axis',(1.,0.,0.)) ;
#64923=DIRECTION('center_axis',(0.625000000000018,0.780624749799786,0.)) ;
#64924=DIRECTION('ref_axis',(0.780624749799786,-0.625000000000018,0.)) ;
#64925=DIRECTION('center_axis',(0.,0.,1.)) ;
#64926=DIRECTION('ref_axis',(-0.744997757011426,0.66706696968741,0.)) ;
#64927=DIRECTION('center_axis',(0.,0.,1.)) ;
#64928=DIRECTION('ref_axis',(1.,0.,0.)) ;
#64929=DIRECTION('center_axis',(1.,0.,0.)) ;
#64930=DIRECTION('ref_axis',(0.,-1.,0.)) ;
#64931=DIRECTION('center_axis',(0.,0.,-1.)) ;
#64932=DIRECTION('ref_axis',(0.433012701892204,-0.901387818866005,0.)) ;
#64933=DIRECTION('center_axis',(-1.,3.55271367880048E-14,0.)) ;
#64934=DIRECTION('ref_axis',(-2.51214793389375E-14,-0.707106781186469,-0.707106781186626)) ;
#64935=DIRECTION('center_axis',(1.,0.,0.)) ;
#64936=DIRECTION('ref_axis',(0.,-1.,0.)) ;
#64937=DIRECTION('',(-1.,3.55271367880048E-14,0.)) ;
#64938=DIRECTION('center_axis',(0.,0.,1.)) ;
#64939=DIRECTION('ref_axis',(1.,0.,0.)) ;
#64940=DIRECTION('center_axis',(0.,1.,0.)) ;
#64941=DIRECTION('ref_axis',(1.,0.,0.)) ;
#64942=DIRECTION('center_axis',(-3.67742382159233E-14,-1.,0.)) ;
#64943=DIRECTION('ref_axis',(0.707106781186532,-2.60033132154483E-14,-0.707106781186563)) ;
#64944=DIRECTION('center_axis',(0.,1.,0.)) ;
#64945=DIRECTION('ref_axis',(1.,0.,0.)) ;
#64946=DIRECTION('center_axis',(0.,0.,-1.)) ;
#64947=DIRECTION('ref_axis',(-1.,0.,0.)) ;
#64948=DIRECTION('center_axis',(0.,0.,-1.)) ;
#64949=DIRECTION('ref_axis',(0.683460430828417,-0.729987561189802,0.)) ;
#64950=DIRECTION('center_axis',(-0.0657636789837963,-0.997835226140326,
0.)) ;
#64951=DIRECTION('ref_axis',(-0.997835226140326,0.0657636789837963,0.)) ;
#64952=DIRECTION('',(0.,0.,-1.)) ;
#64953=DIRECTION('',(0.997835226140326,-0.0657636789837963,-6.85877185444556E-33)) ;
#64954=DIRECTION('center_axis',(0.,0.,-1.)) ;
#64955=DIRECTION('ref_axis',(1.,-2.36847578586694E-14,0.)) ;
#64956=DIRECTION('center_axis',(1.09763027743844E-32,6.22497063709847E-32,
1.)) ;
#64957=DIRECTION('ref_axis',(0.683460430828417,-0.729987561189802,3.79396427154525E-32)) ;
#64958=DIRECTION('center_axis',(-3.55271367880048E-14,-1.,0.)) ;
#64959=DIRECTION('ref_axis',(-1.,3.55271367880048E-14,0.)) ;
#64960=DIRECTION('',(0.,0.,-1.)) ;
#64961=DIRECTION('center_axis',(0.,0.,-1.)) ;
#64962=DIRECTION('ref_axis',(0.433012701892208,-0.901387818866003,0.)) ;
#64963=DIRECTION('',(0.,0.,1.)) ;
#64964=DIRECTION('center_axis',(0.,0.,-1.)) ;
#64965=DIRECTION('ref_axis',(-1.,5.92118946466623E-14,0.)) ;
#64966=DIRECTION('',(0.,0.,-1.)) ;
#64967=DIRECTION('center_axis',(0.707106781186555,-0.70710678118654,0.)) ;
#64968=DIRECTION('ref_axis',(-0.70710678118654,-0.707106781186555,-1.79753461476134E-31)) ;
#64969=DIRECTION('',(0.,0.,-1.)) ;
#64970=DIRECTION('center_axis',(0.,0.,-1.)) ;
#64971=DIRECTION('ref_axis',(1.,-5.92118946466623E-14,0.)) ;
#64972=DIRECTION('center_axis',(-1.,8.30329439001789E-15,0.)) ;
#64973=DIRECTION('ref_axis',(-5.87131576936922E-15,-0.707106781186469,-0.707106781186626)) ;
#64974=DIRECTION('center_axis',(1.,0.,0.)) ;
#64975=DIRECTION('ref_axis',(0.,-1.,0.)) ;
#64976=DIRECTION('',(1.,-8.30329439001789E-15,0.)) ;
#64977=DIRECTION('center_axis',(1.,-8.30329439001789E-15,0.)) ;
#64978=DIRECTION('ref_axis',(-5.87131576936922E-15,-0.707106781186469,-0.707106781186626)) ;
#64979=DIRECTION('center_axis',(-0.707106781186626,0.707106781186469,0.)) ;
#64980=DIRECTION('ref_axis',(-0.707106781186469,-0.707106781186626,0.)) ;
#64981=DIRECTION('center_axis',(1.11022302462516E-14,-1.,0.)) ;
#64982=DIRECTION('ref_axis',(0.707106781186548,7.8504622934189E-15,-0.707106781186548)) ;
#64983=DIRECTION('',(1.11022302462516E-14,-1.,0.)) ;
#64984=DIRECTION('center_axis',(0.,1.,0.)) ;
#64985=DIRECTION('ref_axis',(1.,0.,0.)) ;
#64986=DIRECTION('center_axis',(0.,0.,-1.)) ;
#64987=DIRECTION('ref_axis',(-1.,0.,0.)) ;
#64988=DIRECTION('center_axis',(0.,-1.,0.)) ;
#64989=DIRECTION('ref_axis',(-1.,0.,0.)) ;
#64990=DIRECTION('center_axis',(0.,0.,-1.)) ;
#64991=DIRECTION('ref_axis',(0.,-1.,0.)) ;
#64992=DIRECTION('center_axis',(-2.22044604925032E-15,1.,0.)) ;
#64993=DIRECTION('ref_axis',(-0.707106781186548,-1.57009245868378E-15,-0.707106781186548)) ;
#64994=DIRECTION('',(-2.22044604925032E-15,1.,0.)) ;
#64995=DIRECTION('center_axis',(0.,0.,-1.)) ;
#64996=DIRECTION('ref_axis',(-1.,0.,0.)) ;
#64997=DIRECTION('center_axis',(0.,-1.,0.)) ;
#64998=DIRECTION('ref_axis',(-1.,0.,0.)) ;
#64999=DIRECTION('center_axis',(0.,0.,1.)) ;
#65000=DIRECTION('ref_axis',(-0.707106781186547,-0.707106781186547,0.)) ;
#65001=DIRECTION('center_axis',(-1.24744160070242E-15,1.,0.)) ;
#65002=DIRECTION('ref_axis',(-0.707106781186532,-8.82074414990863E-16,-0.707106781186563)) ;
#65003=DIRECTION('center_axis',(0.,-1.,0.)) ;
#65004=DIRECTION('ref_axis',(-1.,0.,0.)) ;
#65005=DIRECTION('',(1.24744160070242E-15,-1.,0.)) ;
#65006=DIRECTION('center_axis',(1.,1.24744160070242E-15,0.)) ;
#65007=DIRECTION('ref_axis',(0.,0.,-1.)) ;
#65008=DIRECTION('center_axis',(0.,-0.707106781186581,-0.707106781186514)) ;
#65009=DIRECTION('ref_axis',(-1.,0.,0.)) ;
#65010=DIRECTION('center_axis',(-1.,-1.24744160070242E-15,0.)) ;
#65011=DIRECTION('ref_axis',(-4.77375233431814E-16,0.382683432365098,-0.923879532511283)) ;
#65012=DIRECTION('center_axis',(-8.82074414990881E-16,0.707106781186546,
0.707106781186549)) ;
#65013=DIRECTION('ref_axis',(-0.707106781186616,0.499999999999952,-0.499999999999951)) ;
#65014=DIRECTION('center_axis',(0.,-0.707106781186414,-0.707106781186681)) ;
#65015=DIRECTION('ref_axis',(-1.,0.,0.)) ;
#65016=DIRECTION('center_axis',(-1.,-1.24744160070242E-15,0.)) ;
#65017=DIRECTION('ref_axis',(0.,0.,1.)) ;
#65018=DIRECTION('center_axis',(0.,-1.,0.)) ;
#65019=DIRECTION('ref_axis',(-1.,0.,0.)) ;
#65020=DIRECTION('center_axis',(-1.24744160070242E-15,1.,0.)) ;
#65021=DIRECTION('ref_axis',(-0.707106781186548,-8.82074414990883E-16,-0.707106781186548)) ;
#65022=DIRECTION('center_axis',(0.,-1.,0.)) ;
#65023=DIRECTION('ref_axis',(-1.,0.,0.)) ;
#65024=DIRECTION('',(1.24744160070242E-15,-1.,0.)) ;
#65025=DIRECTION('center_axis',(1.,1.24744160070242E-15,0.)) ;
#65026=DIRECTION('ref_axis',(0.,0.,-1.)) ;
#65027=DIRECTION('center_axis',(0.,-0.624695047554359,-0.780868809443082)) ;
#65028=DIRECTION('ref_axis',(-1.,0.,0.)) ;
#65029=DIRECTION('center_axis',(-1.,-1.24744160070242E-15,0.)) ;
#65030=DIRECTION('ref_axis',(-5.4037764336759E-16,0.433188730489114,-0.901303236306866)) ;
#65031=DIRECTION('center_axis',(-7.79270590072164E-16,0.624695047554423,
0.780868809443031)) ;
#65032=DIRECTION('ref_axis',(-0.707106781186341,0.552157630374394,-0.441726104299515)) ;
#65033=DIRECTION('',(7.79270590072164E-16,-0.624695047554423,-0.780868809443031)) ;
#65034=DIRECTION('center_axis',(0.,-0.331006941435217,-0.943628319160517)) ;
#65035=DIRECTION('ref_axis',(2.3542424418412E-15,-0.943628319160517,0.331006941435217)) ;
#65036=DIRECTION('center_axis',(1.34572487833352E-15,-1.,-1.96585022416868E-45)) ;
#65037=DIRECTION('ref_axis',(0.707106781186516,9.51571187081031E-16,0.707106781186579)) ;
#65038=DIRECTION('center_axis',(0.,-1.,0.)) ;
#65039=DIRECTION('ref_axis',(0.707106781186516,0.,0.707106781186579)) ;
#65040=DIRECTION('',(1.34572487833352E-15,-1.,-1.96585022416868E-45)) ;
#65041=DIRECTION('center_axis',(0.,1.,0.)) ;
#65042=DIRECTION('ref_axis',(0.,0.,1.)) ;
#65043=DIRECTION('',(-1.34572487833352E-15,1.,1.96585022416868E-45)) ;
#65044=DIRECTION('center_axis',(1.95689141014107E-45,1.96585022416868E-45,
-1.)) ;
#65045=DIRECTION('ref_axis',(-1.,0.,0.)) ;
#65046=DIRECTION('center_axis',(1.,8.88178419700302E-14,0.)) ;
#65047=DIRECTION('ref_axis',(0.,0.,1.)) ;
#65048=DIRECTION('center_axis',(-1.95689141014107E-45,-1.96585022416868E-45,
1.)) ;
#65049=DIRECTION('ref_axis',(0.707106781186525,-0.70710678118657,-6.3348381504005E-48)) ;
#65050=DIRECTION('center_axis',(1.95689141014107E-45,1.96585022416868E-45,
-1.)) ;
#65051=DIRECTION('ref_axis',(0.707106781186525,-0.70710678118657,-6.3348381504005E-48)) ;
#65052=DIRECTION('center_axis',(-1.,8.30329439001789E-15,-1.95689141014106E-45)) ;
#65053=DIRECTION('ref_axis',(-5.87131576937143E-15,-0.707106781186736,0.707106781186359)) ;
#65054=DIRECTION('center_axis',(1.,0.,0.)) ;
#65055=DIRECTION('ref_axis',(0.,0.,1.)) ;
#65056=DIRECTION('',(-1.,8.30329439001789E-15,-1.95689141014106E-45)) ;
#65057=DIRECTION('center_axis',(1.95689141014107E-45,1.96585022416868E-45,
-1.)) ;
#65058=DIRECTION('ref_axis',(-1.,0.,0.)) ;
#65059=DIRECTION('center_axis',(0.,-1.,0.)) ;
#65060=DIRECTION('ref_axis',(0.,0.,1.)) ;
#65061=DIRECTION('center_axis',(1.95689141014107E-45,1.96585022416868E-45,
-1.)) ;
#65062=DIRECTION('ref_axis',(-0.707106781186547,-0.707106781186547,-2.77379721046322E-45)) ;
#65063=DIRECTION('center_axis',(-1.24744160070242E-15,1.,1.96585022416868E-45)) ;
#65064=DIRECTION('ref_axis',(-0.707106781186548,-8.82074414990883E-16,0.707106781186548)) ;
#65065=DIRECTION('center_axis',(0.,-1.,0.)) ;
#65066=DIRECTION('ref_axis',(0.,0.,1.)) ;
#65067=DIRECTION('',(-1.24744160070242E-15,1.,1.96585022416868E-45)) ;
#65068=DIRECTION('center_axis',(1.,1.24744160070242E-15,0.)) ;
#65069=DIRECTION('ref_axis',(0.,0.,-1.)) ;
#65070=DIRECTION('center_axis',(0.,0.,1.)) ;
#65071=DIRECTION('ref_axis',(0.,1.,0.)) ;
#65072=DIRECTION('center_axis',(-1.,-1.24744160070242E-15,0.)) ;
#65073=DIRECTION('ref_axis',(-8.82074414990876E-16,0.707106781186542,0.707106781186553)) ;
#65074=DIRECTION('center_axis',(0.,0.,-1.)) ;
#65075=DIRECTION('ref_axis',(-0.707106781186359,0.707106781186736,0.)) ;
#65076=DIRECTION('',(0.,0.,-1.)) ;
#65077=DIRECTION('center_axis',(1.,8.88178419700125E-16,0.)) ;
#65078=DIRECTION('ref_axis',(-8.88178419700125E-16,1.,0.)) ;
#65079=DIRECTION('center_axis',(0.,0.,-1.)) ;
#65080=DIRECTION('ref_axis',(1.,0.,0.)) ;
#65081=DIRECTION('',(-1.,0.,0.)) ;
#65082=DIRECTION('center_axis',(-1.,0.,0.)) ;
#65083=DIRECTION('ref_axis',(0.,0.382683432365084,-0.923879532511289)) ;
#65084=DIRECTION('center_axis',(0.,0.,-1.)) ;
#65085=DIRECTION('ref_axis',(1.,0.,0.)) ;
#65086=DIRECTION('',(-1.,0.,0.)) ;
#65087=DIRECTION('center_axis',(0.,0.,1.)) ;
#65088=DIRECTION('ref_axis',(0.985598559653495,0.169101978725727,0.)) ;
#65089=DIRECTION('',(0.,1.,0.)) ;
#65090=DIRECTION('center_axis',(0.,0.,-1.)) ;
#65091=DIRECTION('ref_axis',(-0.999082519440321,-0.0428266196282222,0.)) ;
#65092=DIRECTION('',(0.,1.,0.)) ;
#65093=DIRECTION('center_axis',(0.,0.,-1.)) ;
#65094=DIRECTION('ref_axis',(-0.945182639171645,-0.326542154412755,0.)) ;
#65095=DIRECTION('',(0.0419797672693987,0.999118461014512,0.)) ;
#65096=DIRECTION('',(-0.906307787036666,0.422618261740665,0.)) ;
#65097=DIRECTION('',(-0.0501684275789832,-0.998740771609056,0.)) ;
#65098=DIRECTION('',(0.732832174562208,0.680409438446018,0.)) ;
#65099=DIRECTION('',(-0.906307787036666,0.422618261740665,0.)) ;
#65100=DIRECTION('',(0.0501684275790028,0.998740771609055,0.)) ;
#65101=DIRECTION('',(-0.732832174562234,-0.68040943844599,0.)) ;
#65102=DIRECTION('',(0.906307787036654,-0.42261826174069,0.)) ;
#65103=DIRECTION('',(0.1631941084961,-0.986593980800695,0.)) ;
#65104=DIRECTION('',(0.906307787036654,-0.42261826174069,0.)) ;
#65105=DIRECTION('center_axis',(-1.,0.,0.)) ;
#65106=DIRECTION('ref_axis',(0.,0.433188730489175,-0.901303236306837)) ;
#65107=DIRECTION('',(1.,0.,0.)) ;
#65108=DIRECTION('center_axis',(1.,0.,0.)) ;
#65109=DIRECTION('ref_axis',(0.,0.780868809443035,-0.624695047554418)) ;
#65110=DIRECTION('center_axis',(0.,0.780868809443031,-0.624695047554423)) ;
#65111=DIRECTION('ref_axis',(-1.,0.,0.)) ;
#65112=DIRECTION('',(1.,0.,0.)) ;
#65113=DIRECTION('',(-0.42426406871193,0.565685424949236,0.707106781186548)) ;
#65114=DIRECTION('center_axis',(0.,-0.780868809443031,0.624695047554423)) ;
#65115=DIRECTION('ref_axis',(0.,0.624695047554423,0.780868809443031)) ;
#65116=DIRECTION('center_axis',(0.,1.,0.)) ;
#65117=DIRECTION('ref_axis',(1.,0.,0.)) ;
#65118=DIRECTION('',(-1.,0.,-1.95689141014107E-45)) ;
#65119=DIRECTION('',(0.,0.,-1.)) ;
#65120=DIRECTION('',(0.,0.,1.)) ;
#65121=DIRECTION('center_axis',(0.,-1.,0.)) ;
#65122=DIRECTION('ref_axis',(0.514495755427527,0.,-0.857492925712544)) ;
#65123=DIRECTION('center_axis',(0.,-1.,0.)) ;
#65124=DIRECTION('ref_axis',(-1.,0.,0.)) ;
#65125=DIRECTION('center_axis',(-1.,0.,-1.95689141014107E-45)) ;
#65126=DIRECTION('ref_axis',(-1.38373118615647E-45,0.70710678118654,0.707106781186555)) ;
#65127=DIRECTION('',(1.,0.,1.95689141014107E-45)) ;
#65128=DIRECTION('center_axis',(-1.,0.,0.)) ;
#65129=DIRECTION('ref_axis',(0.,0.70710678118654,0.707106781186555)) ;
#65130=DIRECTION('center_axis',(1.95689141014107E-45,1.96585022416868E-45,
-1.)) ;
#65131=DIRECTION('ref_axis',(1.,1.86628956086257E-106,1.95689141014107E-45)) ;
#65132=DIRECTION('',(-1.,0.,0.)) ;
#65133=DIRECTION('',(1.30614473485314E-15,-1.,0.)) ;
#65134=DIRECTION('',(1.,0.,0.)) ;
#65135=DIRECTION('',(0.,-1.,0.)) ;
#65136=DIRECTION('center_axis',(0.,1.,0.)) ;
#65137=DIRECTION('ref_axis',(1.,0.,0.)) ;
#65138=DIRECTION('',(0.,0.,-1.)) ;
#65139=DIRECTION('',(0.,0.,-1.)) ;
#65140=DIRECTION('center_axis',(1.37008135359091E-15,0.316227766016839,
-0.948683298050513)) ;
#65141=DIRECTION('ref_axis',(-4.03197281156824E-15,-0.948683298050513,-0.316227766016839)) ;
#65142=DIRECTION('center_axis',(-1.,0.,0.)) ;
#65143=DIRECTION('ref_axis',(0.,1.,0.)) ;
#65144=DIRECTION('center_axis',(0.,-0.554700196225204,0.832050294337861)) ;
#65145=DIRECTION('ref_axis',(0.,-0.832050294337861,-0.554700196225204)) ;
#65146=DIRECTION('center_axis',(0.,0.94868329805046,0.316227766016998)) ;
#65147=DIRECTION('ref_axis',(0.,0.316227766016998,-0.94868329805046)) ;
#65148=DIRECTION('center_axis',(1.37008135359091E-15,0.316227766016839,
-0.948683298050513)) ;
#65149=DIRECTION('ref_axis',(-4.0319728115686E-15,-0.948683298050513,-0.316227766016839)) ;
#65150=DIRECTION('center_axis',(0.,0.948683298050465,0.316227766016985)) ;
#65151=DIRECTION('ref_axis',(1.,0.,0.)) ;
#65152=DIRECTION('center_axis',(0.,-0.554700196225165,0.832050294337886)) ;
#65153=DIRECTION('ref_axis',(0.,-0.832050294337886,-0.554700196225165)) ;
#65154=DIRECTION('center_axis',(1.,0.,0.)) ;
#65155=DIRECTION('ref_axis',(0.,0.316227766016984,-0.948683298050465)) ;
#65156=DIRECTION('center_axis',(0.,0.,1.)) ;
#65157=DIRECTION('ref_axis',(0.496136371636827,0.868244608816573,0.)) ;
#65158=DIRECTION('',(0.,0.,-1.)) ;
#65159=DIRECTION('center_axis',(0.,0.,1.)) ;
#65160=DIRECTION('ref_axis',(0.861535459822987,0.507697401478079,0.)) ;
#65161=DIRECTION('',(0.,0.,1.)) ;
#65162=DIRECTION('center_axis',(0.,0.643223921263855,0.765678122394751)) ;
#65163=DIRECTION('ref_axis',(1.,0.,0.)) ;
#65164=DIRECTION('center_axis',(-1.,0.,0.)) ;
#65165=DIRECTION('ref_axis',(0.,0.,1.)) ;
#65166=DIRECTION('center_axis',(0.,0.948683298050574,0.316227766016658)) ;
#65167=DIRECTION('ref_axis',(1.,0.,0.)) ;
#65168=DIRECTION('center_axis',(1.,0.,0.)) ;
#65169=DIRECTION('ref_axis',(0.,0.500068151122686,-0.865986053139852)) ;
#65170=DIRECTION('center_axis',(-1.,0.,0.)) ;
#65171=DIRECTION('ref_axis',(0.,0.500068151122686,-0.865986053139852)) ;
#65172=DIRECTION('center_axis',(0.,-0.948683298050513,-0.316227766016839)) ;
#65173=DIRECTION('ref_axis',(0.707106781186539,0.223606797749982,-0.670820393249945)) ;
#65174=DIRECTION('',(0.,0.948683298050513,0.316227766016839)) ;
#65175=DIRECTION('',(0.,-0.948683298050513,-0.316227766016839)) ;
#65176=DIRECTION('center_axis',(0.,0.,-1.)) ;
#65177=DIRECTION('ref_axis',(-0.707106781186359,-0.707106781186736,0.)) ;
#65178=DIRECTION('center_axis',(0.,0.,-1.)) ;
#65179=DIRECTION('ref_axis',(-0.707106781186359,-0.707106781186736,0.)) ;
#65180=DIRECTION('',(0.,0.,-1.)) ;
#65181=DIRECTION('',(0.,0.,1.)) ;
#65182=DIRECTION('center_axis',(1.,0.,1.44419255235793E-15)) ;
#65183=DIRECTION('ref_axis',(8.44434238398369E-16,0.811242185175624,-0.584710284663678)) ;
#65184=DIRECTION('',(-1.,0.,-1.44419255235793E-15)) ;
#65185=DIRECTION('',(1.,0.,1.44419255235793E-15)) ;
#65186=DIRECTION('center_axis',(0.,0.,-1.)) ;
#65187=DIRECTION('ref_axis',(0.707106781186359,-0.707106781186736,0.)) ;
#65188=DIRECTION('center_axis',(0.,0.,-1.)) ;
#65189=DIRECTION('ref_axis',(0.707106781186359,-0.707106781186736,0.)) ;
#65190=DIRECTION('',(0.,0.,-1.)) ;
#65191=DIRECTION('',(0.,0.,1.)) ;
#65192=DIRECTION('center_axis',(0.,0.948683298050513,0.316227766016839)) ;
#65193=DIRECTION('ref_axis',(-0.707106781186474,0.223606797750003,-0.670820393250006)) ;
#65194=DIRECTION('center_axis',(0.,-0.94868329805046,-0.316227766016998)) ;
#65195=DIRECTION('ref_axis',(-1.,0.,0.)) ;
#65196=DIRECTION('',(0.,-0.948683298050513,-0.316227766016839)) ;
#65197=DIRECTION('',(0.,0.948683298050513,0.316227766016839)) ;
#65198=DIRECTION('center_axis',(-0.829818692458,-0.529396679138204,-0.176465559712756)) ;
#65199=DIRECTION('ref_axis',(-0.537837055500907,0.843048813373291,-5.64517599036335E-17)) ;
#65200=DIRECTION('center_axis',(-1.37008135359091E-15,-0.316227766016839,
0.948683298050513)) ;
#65201=DIRECTION('ref_axis',(4.05940119804181E-15,0.948683298050513,0.316227766016839)) ;
#65202=DIRECTION('center_axis',(0.,0.,-1.)) ;
#65203=DIRECTION('ref_axis',(0.891721613427202,0.452584317168402,0.)) ;
#65204=DIRECTION('',(0.,0.,-1.)) ;
#65205=DIRECTION('center_axis',(0.,0.,1.)) ;
#65206=DIRECTION('ref_axis',(0.891721613427202,0.452584317168402,0.)) ;
#65207=DIRECTION('',(0.,0.,-1.)) ;
#65208=DIRECTION('center_axis',(-4.33257765707378E-15,-1.,0.)) ;
#65209=DIRECTION('ref_axis',(-1.,4.33257765707378E-15,0.)) ;
#65210=DIRECTION('',(1.,-4.33257765707378E-15,0.)) ;
#65211=DIRECTION('center_axis',(1.,-4.33257765707378E-15,0.)) ;
#65212=DIRECTION('ref_axis',(3.51476976596738E-15,0.811242185175568,-0.584710284663755)) ;
#65213=DIRECTION('',(-1.,4.33257765707378E-15,-1.87094791317046E-31)) ;
#65214=DIRECTION('center_axis',(1.37008135359091E-15,0.316227766016839,
-0.948683298050513)) ;
#65215=DIRECTION('ref_axis',(-1.,2.21856832751295E-31,-1.44419255235793E-15)) ;
#65216=DIRECTION('',(-1.,4.33257765707378E-15,0.)) ;
#65217=DIRECTION('center_axis',(-1.37008135359091E-15,-0.316227766016839,
0.948683298050513)) ;
#65218=DIRECTION('ref_axis',(6.51683787482125E-33,0.948683298050513,0.316227766016839)) ;
#65219=DIRECTION('',(1.,-4.33257765707378E-15,0.)) ;
#65220=DIRECTION('center_axis',(-1.,4.33257765707378E-15,0.)) ;
#65221=DIRECTION('ref_axis',(-6.94002007111956E-16,-0.160182243006969,0.987087457637497)) ;
#65222=DIRECTION('center_axis',(-0.619644288569963,3.43140279610413E-12,
-0.784882765540577)) ;
#65223=DIRECTION('ref_axis',(-0.758435045527754,-0.257405018879986,0.59876450961184)) ;
#65224=DIRECTION('center_axis',(0.619644288579022,1.3942318686827E-14,0.784882765533426)) ;
#65225=DIRECTION('ref_axis',(-0.784882765533426,2.93522498670039E-14,0.619644288579022)) ;
#65226=DIRECTION('',(1.,-4.33257765707378E-15,0.)) ;
#65227=DIRECTION('center_axis',(-1.1460366705808E-14,1.,0.)) ;
#65228=DIRECTION('ref_axis',(-0.923879532511294,-1.05879982345699E-14,-0.382683432365072)) ;
#65229=DIRECTION('',(-1.1460366705808E-14,1.,0.)) ;
#65230=DIRECTION('center_axis',(0.707106781186548,0.707106781186548,0.)) ;
#65231=DIRECTION('ref_axis',(-0.707106781186548,0.707106781186548,-6.13317366673343E-17)) ;
#65232=DIRECTION('center_axis',(0.325057583671787,0.888073833977182,-0.325057583671767)) ;
#65233=DIRECTION('ref_axis',(0.627963030199634,-0.459700843380854,-0.627963030199569)) ;
#65234=DIRECTION('center_axis',(-0.577350269189617,-0.577350269189633,0.577350269189627)) ;
#65235=DIRECTION('ref_axis',(-0.816496580927732,0.408248290463818,-0.408248290463895)) ;
#65236=DIRECTION('',(-0.577350269189617,-0.577350269189633,0.577350269189627)) ;
#65237=DIRECTION('center_axis',(1.,0.,0.)) ;
#65238=DIRECTION('ref_axis',(0.,0.707106781186527,-0.707106781186567)) ;
#65239=DIRECTION('',(0.577350269189617,0.577350269189633,-0.577350269189627)) ;
#65240=DIRECTION('center_axis',(-1.,-1.1460366705808E-14,0.)) ;
#65241=DIRECTION('ref_axis',(-8.10370301256115E-15,0.707106781186528,-0.707106781186567)) ;
#65242=DIRECTION('center_axis',(1.,1.1460366705808E-14,0.)) ;
#65243=DIRECTION('ref_axis',(1.1460366705808E-14,-1.,0.)) ;
#65244=DIRECTION('',(0.,0.,-1.)) ;
#65245=DIRECTION('',(0.,0.,-1.)) ;
#65246=DIRECTION('',(-1.1460366705808E-14,1.,0.)) ;
#65247=DIRECTION('',(0.,0.,-1.)) ;
#65248=DIRECTION('',(1.1460366705808E-14,-1.,0.)) ;
#65249=DIRECTION('center_axis',(-0.707106781186557,0.707106781186538,0.)) ;
#65250=DIRECTION('ref_axis',(0.,0.,1.)) ;
#65251=DIRECTION('',(0.,0.,1.)) ;
#65252=DIRECTION('',(-0.707106781186538,-0.707106781186557,0.)) ;
#65253=DIRECTION('center_axis',(1.,0.,0.)) ;
#65254=DIRECTION('ref_axis',(0.,-1.,0.)) ;
#65255=DIRECTION('',(0.,-1.,0.)) ;
#65256=DIRECTION('',(0.,1.,-1.1460366705808E-14)) ;
#65257=DIRECTION('center_axis',(-0.775298772960297,-0.446604865986822,-0.446604865986871)) ;
#65258=DIRECTION('ref_axis',(2.37792745215863E-16,0.707106781186586,-0.707106781186509)) ;
#65259=DIRECTION('center_axis',(0.562259334229024,0.584749707598188,0.58474970759819)) ;
#65260=DIRECTION('ref_axis',(0.713802383285103,0.0138615341031294,-0.700209979569568)) ;
#65261=DIRECTION('center_axis',(0.562259334229093,0.584749707598142,0.58474970759817)) ;
#65262=DIRECTION('ref_axis',(0.720833064901749,-0.693108716251896,7.79318925176357E-14)) ;
#65263=DIRECTION('center_axis',(-0.562259334229085,-0.584749707598146,-0.584749707598173)) ;
#65264=DIRECTION('ref_axis',(-1.18627502215973E-16,0.707106781186564,-0.707106781186531)) ;
#65265=DIRECTION('center_axis',(0.19685783251961,-0.583304900665865,0.78803704648631)) ;
#65266=DIRECTION('ref_axis',(0.78119171350986,0.579006600237654,0.233432781812587)) ;
#65267=DIRECTION('center_axis',(0.565722293792106,0.583077304611728,0.583077304611765)) ;
#65268=DIRECTION('ref_axis',(0.789377540093176,-0.587385910954562,-0.178496192700365)) ;
#65269=DIRECTION('center_axis',(0.564625956820454,0.583608399907212,0.583608399907276)) ;
#65270=DIRECTION('ref_axis',(0.77036467547575,-0.626421912814156,-0.118885886148851)) ;
#65271=DIRECTION('center_axis',(0.00458966530060586,-0.702402377604852,
0.711765294818088)) ;
#65272=DIRECTION('ref_axis',(-0.569710409149352,-0.58680098182834,-0.575408252836344)) ;
#65273=DIRECTION('center_axis',(-0.693108716251782,-0.720833064901858,0.)) ;
#65274=DIRECTION('ref_axis',(-0.509705948295558,0.49010187336111,0.707106781186587)) ;
#65275=DIRECTION('',(-0.693108716251782,-0.720833064901858,0.)) ;
#65276=DIRECTION('center_axis',(-1.,0.,0.)) ;
#65277=DIRECTION('ref_axis',(0.,-0.382683432365103,0.923879532511281)) ;
#65278=DIRECTION('',(1.,0.,0.)) ;
#65279=DIRECTION('',(-1.,0.,0.)) ;
#65280=DIRECTION('center_axis',(0.5812381937191,0.813733471206732,0.)) ;
#65281=DIRECTION('ref_axis',(0.813733471206732,-0.5812381937191,0.)) ;
#65282=DIRECTION('',(1.,0.,0.)) ;
#65283=DIRECTION('center_axis',(0.,1.,0.)) ;
#65284=DIRECTION('ref_axis',(0.999543602081496,0.,-0.0302090638376767)) ;
#65285=DIRECTION('center_axis',(-0.57735026918968,0.577350269189644,0.577350269189553)) ;
#65286=DIRECTION('ref_axis',(4.44309531493773E-14,0.707106781186514,-0.707106781186581)) ;
#65287=DIRECTION('center_axis',(-0.707106781186548,-0.707106781186548,0.)) ;
#65288=DIRECTION('ref_axis',(0.707106781186548,-0.707106781186548,1.05140120001146E-16)) ;
#65289=DIRECTION('center_axis',(0.577350269189625,-0.577350269189625,-0.577350269189627)) ;
#65290=DIRECTION('ref_axis',(-0.707106781186519,5.9788700148313E-14,-0.707106781186576)) ;
#65291=DIRECTION('center_axis',(-0.577350269189553,0.577350269189626,0.577350269189698)) ;
#65292=DIRECTION('ref_axis',(2.33165764110149E-16,0.707106781186592,-0.707106781186503)) ;
#65293=DIRECTION('',(-0.577350269189625,0.577350269189625,0.577350269189627)) ;
#65294=DIRECTION('',(0.577350269189625,-0.577350269189625,-0.577350269189627)) ;
#65295=DIRECTION('center_axis',(-0.685916369319234,0.685916369319179,0.242976271680828)) ;
#65296=DIRECTION('ref_axis',(1.06456572474764E-16,0.33390521253534,-0.942606656586791)) ;
#65297=DIRECTION('center_axis',(0.707106781186548,0.707106781186548,0.)) ;
#65298=DIRECTION('ref_axis',(-0.707106781186547,0.707106781186547,4.46048993944254E-17)) ;
#65299=DIRECTION('center_axis',(-0.806404995855704,-0.591363663627519,0.)) ;
#65300=DIRECTION('ref_axis',(-0.591363663627519,0.806404995855704,0.)) ;
#65301=DIRECTION('center_axis',(-0.806404995855704,-0.591363663627519,0.)) ;
#65302=DIRECTION('ref_axis',(-0.591363663627519,0.806404995855704,0.)) ;
#65303=DIRECTION('center_axis',(0.,0.,-1.)) ;
#65304=DIRECTION('ref_axis',(1.,0.,0.)) ;
#65305=DIRECTION('',(1.,-4.33257765707378E-15,0.)) ;
#65306=DIRECTION('center_axis',(0.,0.,1.)) ;
#65307=DIRECTION('ref_axis',(1.,0.,0.)) ;
#65308=DIRECTION('',(0.,1.,0.)) ;
#65309=DIRECTION('',(-1.,1.97372982155583E-14,0.)) ;
#65310=DIRECTION('',(7.40148683083432E-15,-1.,0.)) ;
#65311=DIRECTION('center_axis',(0.,0.,1.)) ;
#65312=DIRECTION('ref_axis',(1.,0.,0.)) ;
#65313=DIRECTION('',(1.1460366705808E-14,-1.,0.)) ;
#65314=DIRECTION('',(-1.,0.,0.)) ;
#65315=DIRECTION('',(1.32407757812447E-14,1.,0.)) ;
#65316=DIRECTION('center_axis',(0.,0.,-1.)) ;
#65317=DIRECTION('ref_axis',(-0.483396168210882,-0.875401704681363,0.)) ;
#65318=DIRECTION('',(-0.846331659376489,-0.532656289118076,0.)) ;
#65319=DIRECTION('',(0.532656289118094,-0.846331659376477,0.)) ;
#65320=DIRECTION('',(0.846331659376502,0.532656289118055,0.)) ;
#65321=DIRECTION('center_axis',(0.,0.,1.)) ;
#65322=DIRECTION('ref_axis',(-0.483396168210815,-0.8754017046814,0.)) ;
#65323=DIRECTION('',(-8.82718385416297E-15,-1.,0.)) ;
#65324=DIRECTION('',(-1.,-2.61228946970635E-14,0.)) ;
#65325=DIRECTION('',(0.376618052248766,-0.926368632197974,0.)) ;
#65326=DIRECTION('',(0.376618052248709,0.926368632197997,0.)) ;
#65327=DIRECTION('',(-1.,-2.61228946970635E-14,0.)) ;
#65328=DIRECTION('',(0.532656289118094,-0.846331659376477,0.)) ;
#65329=DIRECTION('',(-0.846331659376499,-0.532656289118059,0.)) ;
#65330=DIRECTION('center_axis',(0.,0.,1.)) ;
#65331=DIRECTION('ref_axis',(0.483396168210815,0.8754017046814,0.)) ;
#65332=DIRECTION('',(8.82718385416297E-15,1.,0.)) ;
#65333=DIRECTION('',(1.,2.61228946970635E-14,0.)) ;
#65334=DIRECTION('',(-0.376618052248766,0.926368632197974,0.)) ;
#65335=DIRECTION('',(-0.376618052248709,-0.926368632197997,0.)) ;
#65336=DIRECTION('',(1.,2.61228946970635E-14,0.)) ;
#65337=DIRECTION('',(-1.32407757812447E-14,-1.,0.)) ;
#65338=DIRECTION('center_axis',(0.,0.,-1.)) ;
#65339=DIRECTION('ref_axis',(0.483396168210882,0.875401704681363,0.)) ;
#65340=DIRECTION('',(0.846331659376486,0.532656289118079,0.)) ;
#65341=DIRECTION('',(1.,0.,0.)) ;
#65342=DIRECTION('',(0.,1.,0.)) ;
#65343=DIRECTION('',(-1.,0.,0.)) ;
#65344=DIRECTION('',(0.,-1.,0.)) ;
#65345=DIRECTION('center_axis',(-1.,0.,0.)) ;
#65346=DIRECTION('ref_axis',(0.,0.382683432365084,-0.923879532511289)) ;
#65347=DIRECTION('center_axis',(-0.887969814182011,-0.45887534031808,0.0307088122455258)) ;
#65348=DIRECTION('ref_axis',(0.459384428746892,-0.888157645910459,0.011913968091454)) ;
#65349=DIRECTION('',(1.,0.,0.)) ;
#65350=DIRECTION('center_axis',(0.,0.707106781186549,-0.707106781186546)) ;
#65351=DIRECTION('ref_axis',(-1.,0.,0.)) ;
#65352=DIRECTION('center_axis',(0.,0.707106781186549,-0.707106781186546)) ;
#65353=DIRECTION('ref_axis',(0.,-0.707106781186546,-0.707106781186549)) ;
#65354=DIRECTION('',(-1.,0.,0.)) ;
#65355=DIRECTION('center_axis',(1.1460366705808E-14,-1.,0.)) ;
#65356=DIRECTION('ref_axis',(-0.382683432365084,-4.38569246714114E-15,-0.923879532511289)) ;
#65357=DIRECTION('center_axis',(0.,1.,0.)) ;
#65358=DIRECTION('ref_axis',(0.,0.,-1.)) ;
#65359=DIRECTION('center_axis',(-0.901252424525186,0.433294434867879,0.)) ;
#65360=DIRECTION('ref_axis',(0.433294434867879,0.901252424525186,0.)) ;
#65361=DIRECTION('center_axis',(0.569654939187224,0.592441136754725,0.569654939187197)) ;
#65362=DIRECTION('ref_axis',(-0.720833064901863,0.693108716251777,1.10346919822314E-16)) ;
#65363=DIRECTION('center_axis',(-0.569654939187217,-0.592441136754709,-0.569654939187221)) ;
#65364=DIRECTION('ref_axis',(-0.821767065280649,0.398878088061543,0.406933853696639)) ;
#65365=DIRECTION('',(-0.569654939187217,-0.592441136754709,-0.56965493918722)) ;
#65366=DIRECTION('center_axis',(5.73018335290399E-15,-1.,1.11561779098947E-30)) ;
#65367=DIRECTION('ref_axis',(0.923879532511287,5.2939991172849E-15,-0.382683432365089)) ;
#65368=DIRECTION('center_axis',(-0.707106781186548,-0.707106781186548,0.)) ;
#65369=DIRECTION('ref_axis',(0.707106781186548,-0.707106781186548,3.06658683336673E-17)) ;
#65370=DIRECTION('',(-5.73018335290399E-15,1.,-1.11561779098947E-30)) ;
#65371=DIRECTION('center_axis',(0.,0.,-1.)) ;
#65372=DIRECTION('ref_axis',(1.,0.,0.)) ;
#65373=DIRECTION('',(0.707106781186547,-3.06359504133421E-15,0.707106781186547)) ;
#65374=DIRECTION('center_axis',(0.576796645215489,0.816887770791164,-7.08636583986139E-13)) ;
#65375=DIRECTION('ref_axis',(0.632637288397505,-0.446699141098588,-0.632637288397417)) ;
#65376=DIRECTION('center_axis',(4.3325776570738E-15,1.,0.)) ;
#65377=DIRECTION('ref_axis',(0.382683432365084,-1.65800568879728E-15,-0.923879532511289)) ;
#65378=DIRECTION('',(-0.707106781186547,3.06359504133421E-15,-0.707106781186547)) ;
#65379=DIRECTION('center_axis',(-5.73018335290399E-15,1.,0.)) ;
#65380=DIRECTION('ref_axis',(0.382683432365084,2.19284623357057E-15,-0.923879532511289)) ;
#65381=DIRECTION('',(5.73018335290399E-15,-1.,0.)) ;
#65382=DIRECTION('center_axis',(0.707106781186548,4.05185150628068E-15,
-0.707106781186548)) ;
#65383=DIRECTION('ref_axis',(-0.707106781186548,-8.49416976177182E-32,-0.707106781186548)) ;
#65384=DIRECTION('',(-0.577350269189627,0.577350269189627,-0.577350269189624)) ;
#65385=DIRECTION('center_axis',(0.707106781186548,4.05185150628068E-15,
-0.707106781186548)) ;
#65386=DIRECTION('ref_axis',(-0.707106781186548,-4.04789462004418E-15,-0.707106781186548)) ;
#65387=DIRECTION('center_axis',(0.,1.,0.)) ;
#65388=DIRECTION('ref_axis',(1.,0.,0.)) ;
#65389=DIRECTION('',(-1.,0.,0.)) ;
#65390=DIRECTION('',(0.,0.,1.)) ;
#65391=DIRECTION('center_axis',(-0.707106781186548,-0.707106781186548,0.)) ;
#65392=DIRECTION('ref_axis',(0.,0.,1.)) ;
#65393=DIRECTION('',(0.707106781186547,-0.707106781186547,0.)) ;
#65394=DIRECTION('',(0.707106781186547,-0.707106781186547,0.)) ;
#65395=DIRECTION('center_axis',(-1.,4.33257765707378E-15,0.)) ;
#65396=DIRECTION('ref_axis',(6.94002007111956E-16,0.160182243006969,-0.987087457637497)) ;
#65397=DIRECTION('',(1.,-4.33257765707378E-15,0.)) ;
#65398=DIRECTION('center_axis',(0.,0.,1.)) ;
#65399=DIRECTION('ref_axis',(8.05483811725849E-15,-1.,0.)) ;
#65400=DIRECTION('',(0.,0.,1.)) ;
#65401=DIRECTION('center_axis',(0.,0.,1.)) ;
#65402=DIRECTION('ref_axis',(1.,0.,0.)) ;
#65403=DIRECTION('',(0.,0.,1.)) ;
#65404=DIRECTION('center_axis',(-1.37008135359091E-15,-0.316227766016839,
0.948683298050513)) ;
#65405=DIRECTION('ref_axis',(6.51683787482125E-33,0.948683298050513,0.316227766016839)) ;
#65406=DIRECTION('center_axis',(-0.707106781186548,-0.707106781186548,0.)) ;
#65407=DIRECTION('ref_axis',(0.,0.,1.)) ;
#65408=DIRECTION('center_axis',(-1.,4.33257765707378E-15,0.)) ;
#65409=DIRECTION('ref_axis',(-6.94002007111956E-16,-0.160182243006969,0.987087457637497)) ;
#65410=DIRECTION('',(-1.,4.33257765707378E-15,0.)) ;
#65411=DIRECTION('center_axis',(-1.,0.,0.)) ;
#65412=DIRECTION('ref_axis',(0.,1.,0.)) ;
#65413=DIRECTION('',(0.,1.,0.)) ;
#65414=DIRECTION('center_axis',(-1.,4.33257765707378E-15,0.)) ;
#65415=DIRECTION('ref_axis',(6.94002007111956E-16,0.160182243006969,-0.987087457637497)) ;
#65416=DIRECTION('center_axis',(-1.,0.,0.)) ;
#65417=DIRECTION('ref_axis',(0.,-1.,0.)) ;
#65418=DIRECTION('',(0.,1.,1.15826058041052E-32)) ;
#65419=DIRECTION('',(0.,0.,1.)) ;
#65420=DIRECTION('',(0.,-1.,0.)) ;
#65421=DIRECTION('',(0.,0.,1.)) ;
#65422=DIRECTION('',(0.,0.,-1.)) ;
#65423=DIRECTION('center_axis',(0.,0.,1.)) ;
#65424=DIRECTION('ref_axis',(-1.,0.,0.)) ;
#65425=DIRECTION('center_axis',(-1.09763027743844E-32,-3.07546720254364E-67,
1.)) ;
#65426=DIRECTION('ref_axis',(-1.,1.74482680966927E-115,-1.09763027743844E-32)) ;
#65427=DIRECTION('',(0.,0.,-1.)) ;
#65428=DIRECTION('center_axis',(0.597732795757345,0.801695394071906,0.)) ;
#65429=DIRECTION('ref_axis',(-0.801695394071906,0.597732795757345,-4.49124931094878E-33)) ;
#65430=DIRECTION('',(0.,0.,1.)) ;
#65431=DIRECTION('',(0.801695394071906,-0.597732795757345,4.49124931094878E-33)) ;
#65432=DIRECTION('',(0.,0.,1.)) ;
#65433=DIRECTION('center_axis',(0.,0.,1.)) ;
#65434=DIRECTION('ref_axis',(-1.,0.,0.)) ;
#65435=DIRECTION('center_axis',(-8.11022789614398E-33,1.15826058041052E-32,
-1.)) ;
#65436=DIRECTION('ref_axis',(-1.,-9.39375727024932E-65,8.11022789614398E-33)) ;
#65437=DIRECTION('',(0.,0.,1.)) ;
#65438=DIRECTION('center_axis',(-1.09763027743844E-32,-3.07546720254364E-67,
1.)) ;
#65439=DIRECTION('ref_axis',(-1.,1.74482680966927E-115,-1.09763027743844E-32)) ;
#65440=DIRECTION('center_axis',(0.,0.,1.)) ;
#65441=DIRECTION('ref_axis',(-1.,0.,0.)) ;
#65442=DIRECTION('',(0.,0.,1.)) ;
#65443=DIRECTION('center_axis',(-1.09763027743844E-32,-3.07546720254364E-67,
1.)) ;
#65444=DIRECTION('ref_axis',(-1.,1.74482680966927E-115,-1.09763027743844E-32)) ;
#65445=DIRECTION('center_axis',(0.819152044288994,0.573576436351043,0.)) ;
#65446=DIRECTION('ref_axis',(0.573576436351043,-0.819152044288994,-1.49215481678704E-49)) ;
#65447=DIRECTION('',(0.,0.,-1.)) ;
#65448=DIRECTION('',(0.573576436351043,-0.819152044288994,-1.49215481678704E-49)) ;
#65449=DIRECTION('center_axis',(-0.707106781186624,-0.707106781186472,0.)) ;
#65450=DIRECTION('ref_axis',(-0.707106781186472,0.707106781186624,0.)) ;
#65451=DIRECTION('',(0.,0.,-1.)) ;
#65452=DIRECTION('',(-0.707106781186472,0.707106781186624,-3.62557713776763E-32)) ;
#65453=DIRECTION('center_axis',(0.848048096156437,-0.529919264233188,0.)) ;
#65454=DIRECTION('ref_axis',(-0.529919264233188,-0.848048096156437,0.)) ;
#65455=DIRECTION('',(-0.529919264233188,-0.848048096156437,5.86072992644132E-32)) ;
#65456=DIRECTION('center_axis',(-1.09763027743844E-32,-6.22497063709847E-32,
-1.)) ;
#65457=DIRECTION('ref_axis',(1.,6.87414502838482E-81,-1.09763027743844E-32)) ;
#65458=DIRECTION('',(-0.529919264233188,-0.848048096156437,5.86072992644132E-32)) ;
#65459=DIRECTION('',(-0.573576436351043,0.819152044288994,-4.46962256005402E-32)) ;
#65460=DIRECTION('center_axis',(-1.09763027743844E-32,-6.22497063709847E-32,
-1.)) ;
#65461=DIRECTION('ref_axis',(-0.587740293442623,-0.809049656982796,5.68143190002567E-32)) ;
#65462=DIRECTION('',(-0.997835226140326,0.0657636789837963,6.85877185444556E-33)) ;
#65463=DIRECTION('center_axis',(-1.09763027743844E-32,-6.22497063709847E-32,
-1.)) ;
#65464=DIRECTION('ref_axis',(0.683460430828417,-0.729987561189802,3.79396427154525E-32)) ;
#65465=DIRECTION('',(-1.,0.,1.09763027743844E-32)) ;
#65466=DIRECTION('',(0.,1.,-6.22497063709847E-32)) ;
#65467=DIRECTION('center_axis',(1.09763027743844E-32,6.22497063709847E-32,
1.)) ;
#65468=DIRECTION('ref_axis',(1.,0.,0.)) ;
#65469=DIRECTION('center_axis',(0.573576436350949,-0.81915204428906,0.)) ;
#65470=DIRECTION('ref_axis',(0.,0.,1.)) ;
#65471=DIRECTION('center_axis',(-0.98342301872822,0.181325731544663,-0.000381202396841977)) ;
#65472=DIRECTION('ref_axis',(0.181316930497745,0.983349760701326,-0.0121416161824282)) ;
#65473=DIRECTION('center_axis',(0.997835226140326,-0.0657636789837963,-6.85877185444556E-33)) ;
#65474=DIRECTION('ref_axis',(-0.0465019433652248,-0.705576054910746,0.707106781186438)) ;
#65475=DIRECTION('center_axis',(-0.997835226140325,0.0657636789838148,0.)) ;
#65476=DIRECTION('ref_axis',(-0.0657636789838148,-0.997835226140325,0.)) ;
#65477=DIRECTION('center_axis',(1.09763027743844E-32,6.22497063709847E-32,
1.)) ;
#65478=DIRECTION('ref_axis',(1.,0.,0.)) ;
#65479=DIRECTION('center_axis',(-0.573576436351043,0.819152044288994,-4.46962256005402E-32)) ;
#65480=DIRECTION('ref_axis',(-0.579227965339615,-0.405579787672668,0.707106781186493)) ;
#65481=DIRECTION('center_axis',(-0.848048096156437,0.529919264233188,0.)) ;
#65482=DIRECTION('ref_axis',(-0.529919264233188,-0.848048096156437,7.98410689517261E-17)) ;
#65483=DIRECTION('center_axis',(0.848048096156437,-0.529919264233188,0.)) ;
#65484=DIRECTION('ref_axis',(-0.529919264233188,-0.848048096156437,0.)) ;
#65485=DIRECTION('',(0.529919264233188,0.848048096156437,0.)) ;
#65486=DIRECTION('center_axis',(0.,1.,0.)) ;
#65487=DIRECTION('ref_axis',(0.,0.,1.)) ;
#65488=DIRECTION('',(-1.,0.,0.)) ;
#65489=DIRECTION('',(0.,0.,1.)) ;
#65490=DIRECTION('',(1.,0.,0.)) ;
#65491=DIRECTION('center_axis',(0.,-1.,0.)) ;
#65492=DIRECTION('ref_axis',(0.,0.,-1.)) ;
#65493=DIRECTION('',(-1.,0.,0.)) ;
#65494=DIRECTION('',(0.,0.,-1.)) ;
#65495=DIRECTION('',(1.,0.,0.)) ;
#65496=DIRECTION('center_axis',(1.,0.,0.)) ;
#65497=DIRECTION('ref_axis',(0.,0.,-1.)) ;
#65498=DIRECTION('',(0.,1.,0.)) ;
#65499=DIRECTION('',(0.,-1.,0.)) ;
#65500=DIRECTION('center_axis',(0.,0.,1.)) ;
#65501=DIRECTION('ref_axis',(0.,-1.,0.)) ;
#65502=DIRECTION('',(0.,-1.,0.)) ;
#65503=DIRECTION('center_axis',(0.,1.,0.)) ;
#65504=DIRECTION('ref_axis',(0.,0.,1.)) ;
#65505=DIRECTION('',(0.,0.,1.)) ;
#65506=DIRECTION('center_axis',(0.,0.,-1.)) ;
#65507=DIRECTION('ref_axis',(0.,1.,0.)) ;
#65508=DIRECTION('',(0.,1.,0.)) ;
#65509=DIRECTION('center_axis',(1.,0.,0.)) ;
#65510=DIRECTION('ref_axis',(0.,0.,-1.)) ;
#65511=DIRECTION('center_axis',(0.906307787036666,-0.422618261740665,0.)) ;
#65512=DIRECTION('ref_axis',(-0.298836238730083,-0.640856382055773,0.707106781186577)) ;
#65513=DIRECTION('',(0.906307787036666,-0.422618261740665,0.)) ;
#65514=DIRECTION('',(-0.906307787036666,0.422618261740665,0.)) ;
#65515=DIRECTION('center_axis',(0.155362542872172,-0.987857520228647,6.89948289044009E-15)) ;
#65516=DIRECTION('ref_axis',(0.987857520228647,0.155362542872172,4.6428742654117E-15)) ;
#65517=DIRECTION('center_axis',(-0.0419797672693987,-0.999118461014512,
0.)) ;
#65518=DIRECTION('ref_axis',(-0.706483438992048,0.0296841781088257,0.707106781186528)) ;
#65519=DIRECTION('',(-0.0419797672693987,-0.999118461014512,0.)) ;
#65520=DIRECTION('',(0.0419797672693987,0.999118461014512,0.)) ;
#65521=DIRECTION('center_axis',(0.906307787036666,-0.422618261740665,0.)) ;
#65522=DIRECTION('ref_axis',(-0.298836238730185,-0.640856382055991,0.707106781186336)) ;
#65523=DIRECTION('',(-0.906307787036666,0.422618261740665,0.)) ;
#65524=DIRECTION('',(0.906307787036666,-0.422618261740665,0.)) ;
#65525=DIRECTION('center_axis',(0.856607881531938,0.51596796150281,0.)) ;
#65526=DIRECTION('ref_axis',(-0.51596796150281,0.856607881531938,0.)) ;
#65527=DIRECTION('center_axis',(0.0501684275789832,0.998740771609056,0.)) ;
#65528=DIRECTION('ref_axis',(0.706216372252235,-0.0354744353425645,0.707106781186561)) ;
#65529=DIRECTION('',(-0.0501684275789832,-0.998740771609056,0.)) ;
#65530=DIRECTION('',(0.0501684275789832,0.998740771609056,0.)) ;
#65531=DIRECTION('center_axis',(-0.906307787036635,0.422618261740731,-8.04963018052133E-14)) ;
#65532=DIRECTION('ref_axis',(-0.422618261740731,-0.906307787036635,-3.27260221745424E-14)) ;
#65533=DIRECTION('center_axis',(-0.732832174562208,-0.680409438446018,0.)) ;
#65534=DIRECTION('ref_axis',(-0.48112212790844,0.518190600104545,0.707106781186651)) ;
#65535=DIRECTION('',(0.732832174562208,0.680409438446018,0.)) ;
#65536=DIRECTION('',(-0.732832174562208,-0.680409438446018,0.)) ;
#65537=DIRECTION('center_axis',(-0.422618261740665,-0.906307787036666,0.)) ;
#65538=DIRECTION('ref_axis',(0.906307787036666,-0.422618261740665,0.)) ;
#65539=DIRECTION('',(0.,0.,1.)) ;
#65540=DIRECTION('',(0.906307787036666,-0.422618261740665,0.)) ;
#65541=DIRECTION('',(0.,0.,1.)) ;
#65542=DIRECTION('center_axis',(0.998740771609056,-0.0501684275789832,0.)) ;
#65543=DIRECTION('ref_axis',(0.0501684275789832,0.998740771609056,0.)) ;
#65544=DIRECTION('',(0.,0.,1.)) ;
#65545=DIRECTION('',(0.0501684275789832,0.998740771609056,0.)) ;
#65546=DIRECTION('center_axis',(-0.680409438446018,0.732832174562208,0.)) ;
#65547=DIRECTION('ref_axis',(-0.732832174562208,-0.680409438446018,0.)) ;
#65548=DIRECTION('',(0.,0.,1.)) ;
#65549=DIRECTION('',(-0.732832174562208,-0.680409438446018,0.)) ;
#65550=DIRECTION('center_axis',(-0.422618261740665,-0.906307787036666,0.)) ;
#65551=DIRECTION('ref_axis',(0.906307787036666,-0.422618261740665,0.)) ;
#65552=DIRECTION('',(0.,0.,1.)) ;
#65553=DIRECTION('',(0.906307787036666,-0.422618261740665,0.)) ;
#65554=DIRECTION('center_axis',(0.,0.,-1.)) ;
#65555=DIRECTION('ref_axis',(1.,0.,0.)) ;
#65556=DIRECTION('center_axis',(-0.906307787036654,0.42261826174069,0.)) ;
#65557=DIRECTION('ref_axis',(0.298836238730101,0.640856382055765,0.707106781186577)) ;
#65558=DIRECTION('',(-0.906307787036654,0.42261826174069,0.)) ;
#65559=DIRECTION('center_axis',(-0.856607881531938,-0.51596796150281,0.)) ;
#65560=DIRECTION('ref_axis',(0.51596796150281,-0.856607881531938,0.)) ;
#65561=DIRECTION('',(0.906307787036654,-0.42261826174069,0.)) ;
#65562=DIRECTION('center_axis',(-0.0501684275790028,-0.998740771609055,
0.)) ;
#65563=DIRECTION('ref_axis',(-0.706216372252234,0.0354744353425784,0.707106781186561)) ;
#65564=DIRECTION('',(-0.0501684275790028,-0.998740771609055,0.)) ;
#65565=DIRECTION('center_axis',(0.906307787036677,-0.422618261740641,0.)) ;
#65566=DIRECTION('ref_axis',(0.422618261740641,0.906307787036677,0.)) ;
#65567=DIRECTION('',(0.0501684275790028,0.998740771609055,0.)) ;
#65568=DIRECTION('center_axis',(0.732832174562234,0.68040943844599,0.)) ;
#65569=DIRECTION('ref_axis',(0.481122127908406,-0.518190600104549,0.707106781186672)) ;
#65570=DIRECTION('',(-0.732832174562234,-0.68040943844599,0.)) ;
#65571=DIRECTION('',(0.732832174562234,0.68040943844599,0.)) ;
#65572=DIRECTION('center_axis',(-0.155362542872191,0.987857520228644,-6.89948289044093E-15)) ;
#65573=DIRECTION('ref_axis',(-0.987857520228644,-0.155362542872191,-4.64287426541169E-15)) ;
#65574=DIRECTION('center_axis',(-0.906307787036654,0.42261826174069,0.)) ;
#65575=DIRECTION('ref_axis',(0.298836238730106,0.640856382055777,0.707106781186564)) ;
#65576=DIRECTION('',(0.906307787036654,-0.42261826174069,0.)) ;
#65577=DIRECTION('',(-0.906307787036654,0.42261826174069,0.)) ;
#65578=DIRECTION('center_axis',(-0.1631941084961,0.986593980800695,0.)) ;
#65579=DIRECTION('ref_axis',(0.69762729410203,0.11539566076729,0.707106781186519)) ;
#65580=DIRECTION('',(0.1631941084961,-0.986593980800695,0.)) ;
#65581=DIRECTION('',(-0.1631941084961,0.986593980800695,0.)) ;
#65582=DIRECTION('center_axis',(0.42261826174069,0.906307787036654,0.)) ;
#65583=DIRECTION('ref_axis',(-0.906307787036654,0.42261826174069,0.)) ;
#65584=DIRECTION('',(0.,0.,1.)) ;
#65585=DIRECTION('',(-0.906307787036654,0.42261826174069,0.)) ;
#65586=DIRECTION('',(0.,0.,1.)) ;
#65587=DIRECTION('',(0.,0.,1.)) ;
#65588=DIRECTION('center_axis',(0.986593980800695,0.1631941084961,0.)) ;
#65589=DIRECTION('ref_axis',(-0.1631941084961,0.986593980800696,0.)) ;
#65590=DIRECTION('',(0.,0.,1.)) ;
#65591=DIRECTION('',(-0.1631941084961,0.986593980800695,0.)) ;
#65592=DIRECTION('',(0.,0.,1.)) ;
#65593=DIRECTION('center_axis',(0.,0.,-1.)) ;
#65594=DIRECTION('ref_axis',(1.,0.,0.)) ;
#65595=DIRECTION('center_axis',(6.53072367426566E-15,-1.,0.)) ;
#65596=DIRECTION('ref_axis',(-0.707106781186485,-4.61791899612837E-15,0.70710678118661)) ;
#65597=DIRECTION('',(6.53072367426566E-15,-1.,0.)) ;
#65598=DIRECTION('center_axis',(0.829643915257841,-0.558292910465143,0.)) ;
#65599=DIRECTION('ref_axis',(0.558292910465143,0.829643915257841,0.)) ;
#65600=DIRECTION('',(-6.53072367426566E-15,1.,0.)) ;
#65601=DIRECTION('center_axis',(0.707106781186642,-0.707106781186453,0.)) ;
#65602=DIRECTION('ref_axis',(-0.707106781186453,-0.707106781186642,0.)) ;
#65603=DIRECTION('center_axis',(0.926368632197979,0.376618052248755,0.)) ;
#65604=DIRECTION('ref_axis',(0.266309178662358,-0.655041541705682,0.707106781186564)) ;
#65605=DIRECTION('',(0.926368632197979,0.376618052248755,0.)) ;
#65606=DIRECTION('center_axis',(-1.33801610590714E-13,1.,1.18839703047794E-26)) ;
#65607=DIRECTION('ref_axis',(-1.,-1.33801610590714E-13,4.83146513558743E-27)) ;
#65608=DIRECTION('',(-0.926368632197979,-0.376618052248755,0.)) ;
#65609=DIRECTION('center_axis',(-0.926368632197992,0.376618052248722,0.)) ;
#65610=DIRECTION('ref_axis',(0.266309178662343,0.655041541705713,0.707106781186541)) ;
#65611=DIRECTION('',(-0.926368632197992,0.376618052248721,0.)) ;
#65612=DIRECTION('center_axis',(-0.829643915257841,-0.558292910465143,0.)) ;
#65613=DIRECTION('ref_axis',(0.558292910465143,-0.829643915257841,0.)) ;
#65614=DIRECTION('',(0.926368632197992,-0.376618052248721,0.)) ;
#65615=DIRECTION('center_axis',(6.53072367426566E-15,-1.,0.)) ;
#65616=DIRECTION('ref_axis',(-0.707106781186548,-4.61791899612877E-15,0.707106781186548)) ;
#65617=DIRECTION('',(-6.53072367426566E-15,1.,0.)) ;
#65618=DIRECTION('',(6.53072367426566E-15,-1.,0.)) ;
#65619=DIRECTION('center_axis',(-0.707106781186485,-0.70710678118661,0.)) ;
#65620=DIRECTION('ref_axis',(-0.70710678118661,0.707106781186485,0.)) ;
#65621=DIRECTION('center_axis',(-1.,-1.77635683940026E-14,0.)) ;
#65622=DIRECTION('ref_axis',(-1.25607396694692E-14,0.707106781186485,0.70710678118661)) ;
#65623=DIRECTION('',(1.,1.77635683940026E-14,0.)) ;
#65624=DIRECTION('',(-1.,-1.77635683940026E-14,0.)) ;
#65625=DIRECTION('center_axis',(-0.707106781186485,-0.70710678118661,0.)) ;
#65626=DIRECTION('ref_axis',(0.70710678118661,-0.707106781186485,0.)) ;
#65627=DIRECTION('center_axis',(0.,-1.,0.)) ;
#65628=DIRECTION('ref_axis',(-0.707106781186548,0.,0.707106781186548)) ;
#65629=DIRECTION('',(0.,1.,0.)) ;
#65630=DIRECTION('',(0.,-1.,0.)) ;
#65631=DIRECTION('center_axis',(0.70710678118661,-0.707106781186485,0.)) ;
#65632=DIRECTION('ref_axis',(0.707106781186485,0.70710678118661,0.)) ;
#65633=DIRECTION('center_axis',(1.,0.,0.)) ;
#65634=DIRECTION('ref_axis',(0.,-0.707106781186736,0.707106781186359)) ;
#65635=DIRECTION('',(-1.,0.,0.)) ;
#65636=DIRECTION('',(1.,0.,0.)) ;
#65637=DIRECTION('center_axis',(-1.77635683940026E-14,1.,0.)) ;
#65638=DIRECTION('ref_axis',(-1.,-1.77635683940026E-14,0.)) ;
#65639=DIRECTION('',(0.,0.,1.)) ;
#65640=DIRECTION('',(-1.,-1.77635683940026E-14,0.)) ;
#65641=DIRECTION('',(0.,0.,1.)) ;
#65642=DIRECTION('center_axis',(-1.,0.,0.)) ;
#65643=DIRECTION('ref_axis',(0.,-1.,0.)) ;
#65644=DIRECTION('',(0.,0.,1.)) ;
#65645=DIRECTION('',(0.,-1.,0.)) ;
#65646=DIRECTION('center_axis',(0.,-1.,0.)) ;
#65647=DIRECTION('ref_axis',(1.,0.,0.)) ;
#65648=DIRECTION('',(0.,0.,1.)) ;
#65649=DIRECTION('',(1.,0.,0.)) ;
#65650=DIRECTION('center_axis',(-1.,-6.53072367426566E-15,0.)) ;
#65651=DIRECTION('ref_axis',(6.53072367426566E-15,-1.,0.)) ;
#65652=DIRECTION('',(0.,0.,1.)) ;
#65653=DIRECTION('',(6.53072367426566E-15,-1.,0.)) ;
#65654=DIRECTION('center_axis',(0.,0.,1.)) ;
#65655=DIRECTION('ref_axis',(1.,0.,0.)) ;
#65656=DIRECTION('center_axis',(1.,8.88178419700144E-14,0.)) ;
#65657=DIRECTION('ref_axis',(6.28036983473691E-14,-0.707106781186736,0.707106781186359)) ;
#65658=DIRECTION('',(1.,8.88178419700144E-14,0.)) ;
#65659=DIRECTION('center_axis',(0.70710678118661,0.707106781186485,0.)) ;
#65660=DIRECTION('ref_axis',(-0.707106781186485,0.70710678118661,0.)) ;
#65661=DIRECTION('',(-1.,-8.88178419700144E-14,0.)) ;
#65662=DIRECTION('center_axis',(0.707106781186736,-0.707106781186359,0.)) ;
#65663=DIRECTION('ref_axis',(0.707106781186359,0.707106781186736,0.)) ;
#65664=DIRECTION('center_axis',(0.,1.,0.)) ;
#65665=DIRECTION('ref_axis',(0.707106781186548,0.,0.707106781186548)) ;
#65666=DIRECTION('',(0.,-1.,0.)) ;
#65667=DIRECTION('',(0.,1.,0.)) ;
#65668=DIRECTION('center_axis',(-0.70710678118661,0.707106781186485,0.)) ;
#65669=DIRECTION('ref_axis',(-0.707106781186485,-0.70710678118661,0.)) ;
#65670=DIRECTION('center_axis',(-1.,0.,0.)) ;
#65671=DIRECTION('ref_axis',(0.,0.707106781186736,0.707106781186359)) ;
#65672=DIRECTION('',(1.,0.,0.)) ;
#65673=DIRECTION('',(-1.,0.,0.)) ;
#65674=DIRECTION('center_axis',(-0.70710678118661,-0.707106781186485,0.)) ;
#65675=DIRECTION('ref_axis',(0.707106781186485,-0.70710678118661,0.)) ;
#65676=DIRECTION('center_axis',(0.,-1.,0.)) ;
#65677=DIRECTION('ref_axis',(-0.707106781186548,0.,0.707106781186548)) ;
#65678=DIRECTION('',(0.,1.,0.)) ;
#65679=DIRECTION('',(0.,-1.,0.)) ;
#65680=DIRECTION('center_axis',(-1.,0.,0.)) ;
#65681=DIRECTION('ref_axis',(0.,-1.,0.)) ;
#65682=DIRECTION('',(0.,0.,1.)) ;
#65683=DIRECTION('',(0.,-1.,0.)) ;
#65684=DIRECTION('',(0.,0.,1.)) ;
#65685=DIRECTION('center_axis',(8.88178419700144E-14,-1.,0.)) ;
#65686=DIRECTION('ref_axis',(1.,8.88178419700144E-14,0.)) ;
#65687=DIRECTION('',(0.,0.,1.)) ;
#65688=DIRECTION('',(1.,8.88178419700144E-14,0.)) ;
#65689=DIRECTION('center_axis',(0.,0.,1.)) ;
#65690=DIRECTION('ref_axis',(1.,0.,0.)) ;
#65691=DIRECTION('center_axis',(6.53072367426566E-15,1.,0.)) ;
#65692=DIRECTION('ref_axis',(0.707106781186548,-4.61791899612877E-15,0.707106781186548)) ;
#65693=DIRECTION('',(6.53072367426566E-15,1.,0.)) ;
#65694=DIRECTION('center_axis',(0.70710678118661,0.707106781186485,0.)) ;
#65695=DIRECTION('ref_axis',(0.707106781186485,-0.70710678118661,0.)) ;
#65696=DIRECTION('',(-6.53072367426566E-15,-1.,0.)) ;
#65697=DIRECTION('center_axis',(0.82964391525788,0.558292910465086,0.)) ;
#65698=DIRECTION('ref_axis',(-0.558292910465086,0.82964391525788,0.)) ;
#65699=DIRECTION('center_axis',(1.,0.,0.)) ;
#65700=DIRECTION('ref_axis',(0.,-0.707106781186736,0.707106781186359)) ;
#65701=DIRECTION('',(1.,0.,0.)) ;
#65702=DIRECTION('center_axis',(0.70710678118661,0.707106781186485,0.)) ;
#65703=DIRECTION('ref_axis',(-0.707106781186485,0.70710678118661,0.)) ;
#65704=DIRECTION('',(-1.,0.,0.)) ;
#65705=DIRECTION('center_axis',(-2.22044604925036E-14,1.,0.)) ;
#65706=DIRECTION('ref_axis',(0.707106781186548,1.57009245868381E-14,0.707106781186548)) ;
#65707=DIRECTION('',(-2.22044604925036E-14,1.,0.)) ;
#65708=DIRECTION('center_axis',(-0.707106781186642,0.707106781186453,0.)) ;
#65709=DIRECTION('ref_axis',(-0.707106781186453,-0.707106781186642,0.)) ;
#65710=DIRECTION('',(2.22044604925036E-14,-1.,0.)) ;
#65711=DIRECTION('center_axis',(-1.,1.77635683940026E-14,0.)) ;
#65712=DIRECTION('ref_axis',(1.25607396694736E-14,0.707106781186736,0.707106781186359)) ;
#65713=DIRECTION('',(1.,-1.77635683940026E-14,0.)) ;
#65714=DIRECTION('',(-1.,1.77635683940026E-14,0.)) ;
#65715=DIRECTION('center_axis',(-0.707106781186736,0.707106781186359,0.)) ;
#65716=DIRECTION('ref_axis',(0.707106781186359,0.707106781186736,0.)) ;
#65717=DIRECTION('center_axis',(6.53072367426566E-15,1.,0.)) ;
#65718=DIRECTION('ref_axis',(0.707106781186548,-4.61791899612877E-15,0.707106781186548)) ;
#65719=DIRECTION('',(-6.53072367426566E-15,-1.,0.)) ;
#65720=DIRECTION('',(6.53072367426566E-15,1.,0.)) ;
#65721=DIRECTION('center_axis',(-0.829643915257779,0.558292910465235,0.)) ;
#65722=DIRECTION('ref_axis',(-0.558292910465235,-0.829643915257779,0.)) ;
#65723=DIRECTION('center_axis',(-0.926368632197986,-0.376618052248738,0.)) ;
#65724=DIRECTION('ref_axis',(-0.266309178662346,0.655041541705687,0.707106781186564)) ;
#65725=DIRECTION('',(0.926368632197986,0.376618052248738,0.)) ;
#65726=DIRECTION('',(-0.926368632197986,-0.376618052248738,0.)) ;
#65727=DIRECTION('center_axis',(0.,-1.,0.)) ;
#65728=DIRECTION('ref_axis',(1.,0.,0.)) ;
#65729=DIRECTION('center_axis',(0.926368632197979,-0.376618052248755,0.)) ;
#65730=DIRECTION('ref_axis',(-0.266309178662367,-0.655041541705704,0.707106781186541)) ;
#65731=DIRECTION('',(-0.926368632197979,0.376618052248755,0.)) ;
#65732=DIRECTION('',(0.926368632197979,-0.376618052248755,0.)) ;
#65733=DIRECTION('center_axis',(1.,-6.53072367426566E-15,0.)) ;
#65734=DIRECTION('ref_axis',(6.53072367426566E-15,1.,0.)) ;
#65735=DIRECTION('',(0.,0.,1.)) ;
#65736=DIRECTION('',(6.53072367426566E-15,1.,0.)) ;
#65737=DIRECTION('',(0.,0.,1.)) ;
#65738=DIRECTION('center_axis',(-0.376618052248738,0.926368632197986,0.)) ;
#65739=DIRECTION('ref_axis',(-0.926368632197986,-0.376618052248738,0.)) ;
#65740=DIRECTION('',(0.,0.,1.)) ;
#65741=DIRECTION('',(-0.926368632197986,-0.376618052248738,0.)) ;
#65742=DIRECTION('center_axis',(-0.376618052248755,-0.926368632197979,0.)) ;
#65743=DIRECTION('ref_axis',(0.926368632197979,-0.376618052248755,0.)) ;
#65744=DIRECTION('',(0.,0.,1.)) ;
#65745=DIRECTION('',(0.926368632197979,-0.376618052248755,0.)) ;
#65746=DIRECTION('center_axis',(1.,-6.53072367426566E-15,0.)) ;
#65747=DIRECTION('ref_axis',(6.53072367426566E-15,1.,0.)) ;
#65748=DIRECTION('',(0.,0.,1.)) ;
#65749=DIRECTION('',(6.53072367426566E-15,1.,0.)) ;
#65750=DIRECTION('center_axis',(0.,0.,1.)) ;
#65751=DIRECTION('ref_axis',(1.,0.,0.)) ;
#65752=DIRECTION('center_axis',(0.,-1.,0.)) ;
#65753=DIRECTION('ref_axis',(-0.707106781186532,0.,0.707106781186563)) ;
#65754=DIRECTION('',(0.,-1.,0.)) ;
#65755=DIRECTION('center_axis',(0.70710678118661,-0.707106781186485,0.)) ;
#65756=DIRECTION('ref_axis',(0.707106781186485,0.70710678118661,0.)) ;
#65757=DIRECTION('',(0.,1.,0.)) ;
#65758=DIRECTION('center_axis',(-0.70710678118661,-0.707106781186485,0.)) ;
#65759=DIRECTION('ref_axis',(0.707106781186485,-0.70710678118661,0.)) ;
#65760=DIRECTION('center_axis',(1.,0.,0.)) ;
#65761=DIRECTION('ref_axis',(0.,-0.70710678118672,0.707106781186375)) ;
#65762=DIRECTION('',(-1.,0.,0.)) ;
#65763=DIRECTION('',(1.,0.,0.)) ;
#65764=DIRECTION('center_axis',(0.70710678118661,0.707106781186485,0.)) ;
#65765=DIRECTION('ref_axis',(-0.707106781186485,0.70710678118661,0.)) ;
#65766=DIRECTION('center_axis',(0.,1.,0.)) ;
#65767=DIRECTION('ref_axis',(0.707106781186532,0.,0.707106781186563)) ;
#65768=DIRECTION('',(0.,-1.,0.)) ;
#65769=DIRECTION('',(0.,1.,0.)) ;
#65770=DIRECTION('center_axis',(-0.70710678118661,0.707106781186485,0.)) ;
#65771=DIRECTION('ref_axis',(-0.707106781186485,-0.70710678118661,0.)) ;
#65772=DIRECTION('center_axis',(-1.,0.,0.)) ;
#65773=DIRECTION('ref_axis',(0.,0.70710678118672,0.707106781186375)) ;
#65774=DIRECTION('',(1.,0.,0.)) ;
#65775=DIRECTION('',(-1.,0.,0.)) ;
#65776=DIRECTION('center_axis',(0.,1.,0.)) ;
#65777=DIRECTION('ref_axis',(-1.,0.,0.)) ;
#65778=DIRECTION('',(0.,0.,1.)) ;
#65779=DIRECTION('',(-1.,0.,0.)) ;
#65780=DIRECTION('',(0.,0.,1.)) ;
#65781=DIRECTION('center_axis',(-1.,0.,0.)) ;
#65782=DIRECTION('ref_axis',(0.,-1.,0.)) ;
#65783=DIRECTION('',(0.,0.,1.)) ;
#65784=DIRECTION('',(0.,-1.,0.)) ;
#65785=DIRECTION('center_axis',(0.,0.,1.)) ;
#65786=DIRECTION('ref_axis',(1.,0.,0.)) ;
#65787=DIRECTION('center_axis',(0.376618052248709,0.926368632197998,0.)) ;
#65788=DIRECTION('ref_axis',(0.655041541705691,-0.266309178662323,0.707106781186569)) ;
#65789=DIRECTION('',(0.376618052248709,0.926368632197997,0.)) ;
#65790=DIRECTION('center_axis',(-0.558292910465349,0.829643915257702,0.)) ;
#65791=DIRECTION('ref_axis',(-0.829643915257702,-0.558292910465349,0.)) ;
#65792=DIRECTION('',(-0.376618052248709,-0.926368632197997,0.)) ;
#65793=DIRECTION('center_axis',(1.,1.67252013238358E-13,0.)) ;
#65794=DIRECTION('ref_axis',(-1.67252013238358E-13,1.,0.)) ;
#65795=DIRECTION('center_axis',(-1.,-2.61228946970635E-14,0.)) ;
#65796=DIRECTION('ref_axis',(-1.84716759845137E-14,0.707106781186469,0.707106781186626)) ;
#65797=DIRECTION('',(-1.,-2.61228946970635E-14,0.)) ;
#65798=DIRECTION('center_axis',(-0.70710678118661,0.707106781186485,0.)) ;
#65799=DIRECTION('ref_axis',(0.707106781186485,0.70710678118661,0.)) ;
#65800=DIRECTION('',(1.,2.61228946970635E-14,0.)) ;
#65801=DIRECTION('center_axis',(1.32407757812447E-14,1.,0.)) ;
#65802=DIRECTION('ref_axis',(0.707106781186532,-9.36264234308853E-15,0.707106781186563)) ;
#65803=DIRECTION('',(1.32407757812447E-14,1.,0.)) ;
#65804=DIRECTION('center_axis',(0.,1.,0.)) ;
#65805=DIRECTION('ref_axis',(0.,0.,1.)) ;
#65806=DIRECTION('',(-1.32407757812447E-14,-1.,0.)) ;
#65807=DIRECTION('center_axis',(0.,0.,1.)) ;
#65808=DIRECTION('ref_axis',(1.,0.,0.)) ;
#65809=DIRECTION('center_axis',(-0.846331659376392,-0.53265628911823,0.)) ;
#65810=DIRECTION('ref_axis',(0.,0.,1.)) ;
#65811=DIRECTION('center_axis',(0.,0.,-1.)) ;
#65812=DIRECTION('ref_axis',(0.483396168210882,0.875401704681363,0.)) ;
#65813=DIRECTION('center_axis',(0.,0.,1.)) ;
#65814=DIRECTION('ref_axis',(0.483396168210882,0.875401704681363,0.)) ;
#65815=DIRECTION('center_axis',(-0.846331659376486,-0.532656289118079,0.)) ;
#65816=DIRECTION('ref_axis',(-0.376644874077004,0.598446855477894,0.707106781186646)) ;
#65817=DIRECTION('',(0.846331659376486,0.532656289118079,0.)) ;
#65818=DIRECTION('',(-0.846331659376486,-0.532656289118079,0.)) ;
#65819=DIRECTION('center_axis',(-0.221801981400905,-0.975091729555037,0.)) ;
#65820=DIRECTION('ref_axis',(0.975091729555037,-0.221801981400905,0.)) ;
#65821=DIRECTION('center_axis',(0.532656289118094,-0.846331659376477,0.)) ;
#65822=DIRECTION('ref_axis',(-0.598446855477921,-0.376644874077035,0.707106781186606)) ;
#65823=DIRECTION('',(-0.532656289118094,0.846331659376477,0.)) ;
#65824=DIRECTION('',(0.532656289118094,-0.846331659376477,0.)) ;
#65825=DIRECTION('center_axis',(0.975091729555031,-0.221801981400932,0.)) ;
#65826=DIRECTION('ref_axis',(0.221801981400932,0.97509172955503,0.)) ;
#65827=DIRECTION('center_axis',(0.846331659376499,0.532656289118059,0.)) ;
#65828=DIRECTION('ref_axis',(0.376644874077103,-0.598446855478083,0.707106781186433)) ;
#65829=DIRECTION('',(0.846331659376499,0.532656289118059,0.)) ;
#65830=DIRECTION('center_axis',(0.846331659376493,0.53265628911807,0.)) ;
#65831=DIRECTION('ref_axis',(0.,0.,1.)) ;
#65832=DIRECTION('',(-0.846331659376499,-0.532656289118059,0.)) ;
#65833=DIRECTION('center_axis',(0.,0.,-1.)) ;
#65834=DIRECTION('ref_axis',(-1.,0.,0.)) ;
#65835=DIRECTION('center_axis',(0.,-1.,0.)) ;
#65836=DIRECTION('ref_axis',(0.,0.,1.)) ;
#65837=DIRECTION('center_axis',(0.,0.,1.)) ;
#65838=DIRECTION('ref_axis',(0.483396168210815,0.8754017046814,0.)) ;
#65839=DIRECTION('center_axis',(0.,0.,-1.)) ;
#65840=DIRECTION('ref_axis',(0.483396168210815,0.8754017046814,0.)) ;
#65841=DIRECTION('center_axis',(-8.82718385416297E-15,-1.,0.)) ;
#65842=DIRECTION('ref_axis',(-0.707106781186469,6.24176156205835E-15,0.707106781186626)) ;
#65843=DIRECTION('',(8.82718385416297E-15,1.,0.)) ;
#65844=DIRECTION('',(-8.82718385416297E-15,-1.,0.)) ;
#65845=DIRECTION('center_axis',(-0.707106781186642,-0.707106781186453,0.)) ;
#65846=DIRECTION('ref_axis',(-0.707106781186453,0.707106781186642,0.)) ;
#65847=DIRECTION('center_axis',(-1.,-2.61228946970635E-14,0.)) ;
#65848=DIRECTION('ref_axis',(-1.84716759845202E-14,0.70710678118672,0.707106781186375)) ;
#65849=DIRECTION('',(1.,2.61228946970635E-14,0.)) ;
#65850=DIRECTION('',(-1.,-2.61228946970635E-14,0.)) ;
#65851=DIRECTION('center_axis',(-0.558292910465166,-0.829643915257826,0.)) ;
#65852=DIRECTION('ref_axis',(0.829643915257826,-0.558292910465166,0.)) ;
#65853=DIRECTION('center_axis',(0.376618052248766,-0.926368632197974,0.)) ;
#65854=DIRECTION('ref_axis',(-0.65504154170562,-0.266309178662342,0.707106781186627)) ;
#65855=DIRECTION('',(-0.376618052248766,0.926368632197974,0.)) ;
#65856=DIRECTION('',(0.376618052248766,-0.926368632197974,0.)) ;
#65857=DIRECTION('center_axis',(0.532656289118059,-0.846331659376499,0.)) ;
#65858=DIRECTION('ref_axis',(0.846331659376499,0.532656289118059,0.)) ;
#65859=DIRECTION('',(0.,0.,1.)) ;
#65860=DIRECTION('',(0.846331659376499,0.532656289118059,0.)) ;
#65861=DIRECTION('',(0.,0.,1.)) ;
#65862=DIRECTION('center_axis',(0.,0.,1.)) ;
#65863=DIRECTION('ref_axis',(-0.532656289118219,0.846331659376399,0.)) ;
#65864=DIRECTION('',(0.,0.,1.)) ;
#65865=DIRECTION('center_axis',(0.,0.,-1.)) ;
#65866=DIRECTION('ref_axis',(0.483396168210815,0.8754017046814,0.)) ;
#65867=DIRECTION('center_axis',(-1.,8.82718385416297E-15,0.)) ;
#65868=DIRECTION('ref_axis',(-8.82718385416297E-15,-1.,0.)) ;
#65869=DIRECTION('',(0.,0.,1.)) ;
#65870=DIRECTION('',(-8.82718385416297E-15,-1.,0.)) ;
#65871=DIRECTION('center_axis',(-2.61228946970635E-14,1.,0.)) ;
#65872=DIRECTION('ref_axis',(-1.,-2.61228946970635E-14,0.)) ;
#65873=DIRECTION('',(0.,0.,1.)) ;
#65874=DIRECTION('',(-1.,-2.61228946970635E-14,0.)) ;
#65875=DIRECTION('center_axis',(-0.926368632197974,-0.376618052248766,0.)) ;
#65876=DIRECTION('ref_axis',(0.376618052248766,-0.926368632197974,0.)) ;
#65877=DIRECTION('',(0.,0.,1.)) ;
#65878=DIRECTION('',(0.376618052248766,-0.926368632197974,0.)) ;
#65879=DIRECTION('center_axis',(0.926368632197998,-0.376618052248709,0.)) ;
#65880=DIRECTION('ref_axis',(0.376618052248709,0.926368632197998,0.)) ;
#65881=DIRECTION('',(0.,0.,1.)) ;
#65882=DIRECTION('',(0.376618052248709,0.926368632197997,0.)) ;
#65883=DIRECTION('center_axis',(0.,0.,-1.)) ;
#65884=DIRECTION('ref_axis',(1.,0.,0.)) ;
#65885=DIRECTION('center_axis',(1.,2.61228946970635E-14,0.)) ;
#65886=DIRECTION('ref_axis',(1.84716759845137E-14,-0.707106781186469,0.707106781186626)) ;
#65887=DIRECTION('',(1.,2.61228946970635E-14,0.)) ;
#65888=DIRECTION('center_axis',(0.70710678118661,-0.707106781186485,0.)) ;
#65889=DIRECTION('ref_axis',(-0.707106781186485,-0.70710678118661,0.)) ;
#65890=DIRECTION('',(-1.,-2.61228946970635E-14,0.)) ;
#65891=DIRECTION('center_axis',(0.558292910465349,-0.829643915257702,0.)) ;
#65892=DIRECTION('ref_axis',(0.829643915257702,0.558292910465349,0.)) ;
#65893=DIRECTION('center_axis',(-1.32407757812447E-14,-1.,0.)) ;
#65894=DIRECTION('ref_axis',(-0.707106781186532,9.36264234308853E-15,0.707106781186563)) ;
#65895=DIRECTION('',(-1.32407757812447E-14,-1.,0.)) ;
#65896=DIRECTION('center_axis',(0.,-1.,0.)) ;
#65897=DIRECTION('ref_axis',(0.,0.,1.)) ;
#65898=DIRECTION('',(1.32407757812447E-14,1.,0.)) ;
#65899=DIRECTION('center_axis',(0.,0.,1.)) ;
#65900=DIRECTION('ref_axis',(1.,0.,0.)) ;
#65901=DIRECTION('center_axis',(0.846331659376392,0.53265628911823,0.)) ;
#65902=DIRECTION('ref_axis',(0.,0.,1.)) ;
#65903=DIRECTION('center_axis',(0.,0.,-1.)) ;
#65904=DIRECTION('ref_axis',(-0.483396168210882,-0.875401704681363,0.)) ;
#65905=DIRECTION('center_axis',(0.,0.,1.)) ;
#65906=DIRECTION('ref_axis',(-0.483396168210882,-0.875401704681363,0.)) ;
#65907=DIRECTION('center_axis',(0.846331659376489,0.532656289118076,0.)) ;
#65908=DIRECTION('ref_axis',(0.376644874077132,-0.598446855478104,0.7071067811864)) ;
#65909=DIRECTION('',(-0.846331659376489,-0.532656289118076,0.)) ;
#65910=DIRECTION('',(0.846331659376489,0.532656289118076,0.)) ;
#65911=DIRECTION('center_axis',(0.221801981400905,0.975091729555037,0.)) ;
#65912=DIRECTION('ref_axis',(-0.975091729555037,0.221801981400905,0.)) ;
#65913=DIRECTION('center_axis',(-0.532656289118094,0.846331659376477,0.)) ;
#65914=DIRECTION('ref_axis',(0.598446855477966,0.376644874077064,0.707106781186553)) ;
#65915=DIRECTION('',(-0.532656289118094,0.846331659376477,0.)) ;
#65916=DIRECTION('center_axis',(-0.975091729555031,0.221801981400932,0.)) ;
#65917=DIRECTION('ref_axis',(-0.221801981400932,-0.97509172955503,0.)) ;
#65918=DIRECTION('',(0.532656289118094,-0.846331659376477,0.)) ;
#65919=DIRECTION('center_axis',(-0.846331659376502,-0.532656289118055,0.)) ;
#65920=DIRECTION('ref_axis',(-0.3766448740771,0.598446855478085,0.707106781186433)) ;
#65921=DIRECTION('',(-0.846331659376502,-0.532656289118055,0.)) ;
#65922=DIRECTION('center_axis',(-0.846331659376493,-0.53265628911807,0.)) ;
#65923=DIRECTION('ref_axis',(0.,0.,1.)) ;
#65924=DIRECTION('',(0.846331659376502,0.532656289118055,0.)) ;
#65925=DIRECTION('center_axis',(0.,0.,-1.)) ;
#65926=DIRECTION('ref_axis',(-1.,0.,0.)) ;
#65927=DIRECTION('center_axis',(0.,1.,0.)) ;
#65928=DIRECTION('ref_axis',(0.,0.,1.)) ;
#65929=DIRECTION('center_axis',(0.,0.,1.)) ;
#65930=DIRECTION('ref_axis',(-0.483396168210815,-0.8754017046814,0.)) ;
#65931=DIRECTION('center_axis',(0.,0.,-1.)) ;
#65932=DIRECTION('ref_axis',(-0.483396168210815,-0.8754017046814,0.)) ;
#65933=DIRECTION('center_axis',(8.82718385416297E-15,1.,0.)) ;
#65934=DIRECTION('ref_axis',(0.707106781186469,-6.24176156205835E-15,0.707106781186626)) ;
#65935=DIRECTION('',(-8.82718385416297E-15,-1.,0.)) ;
#65936=DIRECTION('',(8.82718385416297E-15,1.,0.)) ;
#65937=DIRECTION('center_axis',(0.707106781186642,0.707106781186453,0.)) ;
#65938=DIRECTION('ref_axis',(0.707106781186453,-0.707106781186642,0.)) ;
#65939=DIRECTION('center_axis',(1.,2.61228946970635E-14,0.)) ;
#65940=DIRECTION('ref_axis',(1.84716759845202E-14,-0.70710678118672,0.707106781186375)) ;
#65941=DIRECTION('',(-1.,-2.61228946970635E-14,0.)) ;
#65942=DIRECTION('',(1.,2.61228946970635E-14,0.)) ;
#65943=DIRECTION('center_axis',(0.558292910465166,0.829643915257826,0.)) ;
#65944=DIRECTION('ref_axis',(-0.829643915257826,0.558292910465166,0.)) ;
#65945=DIRECTION('center_axis',(-0.376618052248766,0.926368632197974,0.)) ;
#65946=DIRECTION('ref_axis',(0.65504154170562,0.266309178662342,0.707106781186627)) ;
#65947=DIRECTION('',(0.376618052248766,-0.926368632197974,0.)) ;
#65948=DIRECTION('',(-0.376618052248766,0.926368632197974,0.)) ;
#65949=DIRECTION('center_axis',(-1.,-1.67252013238358E-13,0.)) ;
#65950=DIRECTION('ref_axis',(1.67252013238358E-13,-1.,0.)) ;
#65951=DIRECTION('center_axis',(-0.376618052248709,-0.926368632197998,0.)) ;
#65952=DIRECTION('ref_axis',(-0.655041541705691,0.266309178662323,0.707106781186569)) ;
#65953=DIRECTION('',(0.376618052248709,0.926368632197997,0.)) ;
#65954=DIRECTION('',(-0.376618052248709,-0.926368632197997,0.)) ;
#65955=DIRECTION('center_axis',(0.,0.,1.)) ;
#65956=DIRECTION('ref_axis',(0.532656289118219,-0.846331659376399,0.)) ;
#65957=DIRECTION('',(0.,0.,1.)) ;
#65958=DIRECTION('center_axis',(0.,0.,-1.)) ;
#65959=DIRECTION('ref_axis',(-0.483396168210815,-0.8754017046814,0.)) ;
#65960=DIRECTION('',(0.,0.,1.)) ;
#65961=DIRECTION('center_axis',(1.,-8.82718385416297E-15,0.)) ;
#65962=DIRECTION('ref_axis',(8.82718385416297E-15,1.,0.)) ;
#65963=DIRECTION('',(0.,0.,1.)) ;
#65964=DIRECTION('',(8.82718385416297E-15,1.,0.)) ;
#65965=DIRECTION('center_axis',(2.61228946970635E-14,-1.,0.)) ;
#65966=DIRECTION('ref_axis',(1.,2.61228946970635E-14,0.)) ;
#65967=DIRECTION('',(0.,0.,1.)) ;
#65968=DIRECTION('',(1.,2.61228946970635E-14,0.)) ;
#65969=DIRECTION('center_axis',(0.926368632197974,0.376618052248766,0.)) ;
#65970=DIRECTION('ref_axis',(-0.376618052248766,0.926368632197974,0.)) ;
#65971=DIRECTION('',(0.,0.,1.)) ;
#65972=DIRECTION('',(-0.376618052248766,0.926368632197974,0.)) ;
#65973=DIRECTION('center_axis',(-0.926368632197998,0.376618052248709,0.)) ;
#65974=DIRECTION('ref_axis',(-0.376618052248709,-0.926368632197998,0.)) ;
#65975=DIRECTION('',(0.,0.,1.)) ;
#65976=DIRECTION('',(-0.376618052248709,-0.926368632197997,0.)) ;
#65977=DIRECTION('center_axis',(2.61228946970635E-14,-1.,0.)) ;
#65978=DIRECTION('ref_axis',(1.,2.61228946970635E-14,0.)) ;
#65979=DIRECTION('',(0.,0.,1.)) ;
#65980=DIRECTION('',(1.,2.61228946970635E-14,0.)) ;
#65981=DIRECTION('center_axis',(0.,0.,-1.)) ;
#65982=DIRECTION('ref_axis',(1.,0.,0.)) ;
#65983=DIRECTION('center_axis',(-0.0419797672693987,-0.999118461014512,
0.)) ;
#65984=DIRECTION('ref_axis',(0.706483438992037,-0.0296841781088253,-0.707106781186539)) ;
#65985=DIRECTION('',(-0.0419797672693987,-0.999118461014512,0.)) ;
#65986=DIRECTION('center_axis',(0.906307787036666,-0.422618261740665,0.)) ;
#65987=DIRECTION('ref_axis',(0.298836238730083,0.640856382055773,-0.707106781186577)) ;
#65988=DIRECTION('center_axis',(0.155362542871686,-0.987857520228724,6.8994828904185E-15)) ;
#65989=DIRECTION('ref_axis',(-0.987857520228724,-0.155362542871686,4.64287426539732E-15)) ;
#65990=DIRECTION('center_axis',(-0.732832174562208,-0.680409438446018,0.)) ;
#65991=DIRECTION('ref_axis',(0.48112212790844,-0.518190600104545,-0.707106781186651)) ;
#65992=DIRECTION('center_axis',(-0.906307787036715,0.422618261740561,0.)) ;
#65993=DIRECTION('ref_axis',(0.422618261740561,0.906307787036715,0.)) ;
#65994=DIRECTION('center_axis',(0.0501684275789832,0.998740771609056,0.)) ;
#65995=DIRECTION('ref_axis',(-0.706216372252266,0.0354744353425661,-0.70710678118653)) ;
#65996=DIRECTION('center_axis',(0.856607881531863,0.515967961502934,0.)) ;
#65997=DIRECTION('ref_axis',(0.515967961502934,-0.856607881531863,0.)) ;
#65998=DIRECTION('center_axis',(0.906307787036666,-0.422618261740665,0.)) ;
#65999=DIRECTION('ref_axis',(0.298836238730072,0.64085638205575,-0.707106781186603)) ;
#66000=DIRECTION('',(0.,0.,1.)) ;
#66001=DIRECTION('center_axis',(-0.999118461014512,0.0419797672693987,0.)) ;
#66002=DIRECTION('ref_axis',(-0.0419797672693987,-0.999118461014512,0.)) ;
#66003=DIRECTION('',(0.,0.,1.)) ;
#66004=DIRECTION('center_axis',(-0.906307787036654,0.42261826174069,0.)) ;
#66005=DIRECTION('ref_axis',(-0.298836238730101,-0.640856382055765,-0.707106781186577)) ;
#66006=DIRECTION('center_axis',(-0.15536254287169,0.987857520228723,-6.89948289041867E-15)) ;
#66007=DIRECTION('ref_axis',(0.987857520228723,0.15536254287169,-4.64287426539775E-15)) ;
#66008=DIRECTION('center_axis',(-0.0501684275790028,-0.998740771609055,
0.)) ;
#66009=DIRECTION('ref_axis',(0.706216372252234,-0.0354744353425784,-0.707106781186561)) ;
#66010=DIRECTION('center_axis',(-0.856607881531885,-0.515967961502898,0.)) ;
#66011=DIRECTION('ref_axis',(-0.515967961502898,0.856607881531885,0.)) ;
#66012=DIRECTION('',(-0.0501684275790028,-0.998740771609055,0.)) ;
#66013=DIRECTION('center_axis',(-0.906307787036588,0.422618261740832,-4.02481509026046E-14)) ;
#66014=DIRECTION('ref_axis',(0.422618261740832,0.906307787036588,1.63630110872747E-14)) ;
#66015=DIRECTION('center_axis',(-0.906307787036654,0.42261826174069,0.)) ;
#66016=DIRECTION('ref_axis',(-0.298836238730101,-0.640856382055765,-0.707106781186577)) ;
#66017=DIRECTION('',(-0.906307787036654,0.42261826174069,0.)) ;
#66018=DIRECTION('center_axis',(0.732832174562234,0.68040943844599,0.)) ;
#66019=DIRECTION('ref_axis',(-0.481122127908406,0.518190600104549,-0.707106781186672)) ;
#66020=DIRECTION('',(0.732832174562234,0.68040943844599,0.)) ;
#66021=DIRECTION('center_axis',(-0.1631941084961,0.986593980800695,0.)) ;
#66022=DIRECTION('ref_axis',(-0.69762729410203,-0.11539566076729,-0.707106781186519)) ;
#66023=DIRECTION('center_axis',(0.68040943844599,-0.732832174562234,0.)) ;
#66024=DIRECTION('ref_axis',(0.732832174562234,0.68040943844599,0.)) ;
#66025=DIRECTION('',(0.,0.,1.)) ;
#66026=DIRECTION('center_axis',(-0.998740771609055,0.0501684275790028,0.)) ;
#66027=DIRECTION('ref_axis',(-0.0501684275790028,-0.998740771609055,0.)) ;
#66028=DIRECTION('',(0.,0.,1.)) ;
#66029=DIRECTION('center_axis',(0.926368632197979,0.376618052248755,0.)) ;
#66030=DIRECTION('ref_axis',(-0.266309178662367,0.655041541705704,-0.707106781186541)) ;
#66031=DIRECTION('',(-0.926368632197979,-0.376618052248755,0.)) ;
#66032=DIRECTION('center_axis',(0.829643915257887,-0.558292910465075,0.)) ;
#66033=DIRECTION('ref_axis',(-0.558292910465075,-0.829643915257887,0.)) ;
#66034=DIRECTION('',(0.926368632197979,0.376618052248755,0.)) ;
#66035=DIRECTION('center_axis',(1.33801610590758E-13,1.,0.)) ;
#66036=DIRECTION('ref_axis',(1.,-1.33801610590758E-13,0.)) ;
#66037=DIRECTION('center_axis',(-0.926368632197992,0.376618052248722,0.)) ;
#66038=DIRECTION('ref_axis',(-0.266309178662335,-0.655041541705692,-0.707106781186564)) ;
#66039=DIRECTION('',(-0.926368632197992,0.376618052248721,0.)) ;
#66040=DIRECTION('center_axis',(0.829643915257841,0.558292910465143,0.)) ;
#66041=DIRECTION('ref_axis',(0.558292910465143,-0.829643915257841,0.)) ;
#66042=DIRECTION('',(0.926368632197992,-0.376618052248721,0.)) ;
#66043=DIRECTION('center_axis',(6.53072367426566E-15,-1.,0.)) ;
#66044=DIRECTION('ref_axis',(0.707106781186548,4.61791899612877E-15,-0.707106781186548)) ;
#66045=DIRECTION('',(-6.53072367426566E-15,1.,0.)) ;
#66046=DIRECTION('center_axis',(0.707106781186642,-0.707106781186453,0.)) ;
#66047=DIRECTION('ref_axis',(0.707106781186453,0.707106781186642,0.)) ;
#66048=DIRECTION('center_axis',(1.,0.,0.)) ;
#66049=DIRECTION('ref_axis',(0.,0.707106781186736,-0.707106781186359)) ;
#66050=DIRECTION('',(-1.,0.,0.)) ;
#66051=DIRECTION('center_axis',(0.70710678118661,-0.707106781186485,0.)) ;
#66052=DIRECTION('ref_axis',(-0.707106781186485,-0.70710678118661,0.)) ;
#66053=DIRECTION('center_axis',(0.,-1.,0.)) ;
#66054=DIRECTION('ref_axis',(0.707106781186548,0.,-0.707106781186548)) ;
#66055=DIRECTION('',(0.,1.,0.)) ;
#66056=DIRECTION('center_axis',(-0.707106781186736,-0.707106781186359,0.)) ;
#66057=DIRECTION('ref_axis',(-0.707106781186359,0.707106781186736,0.)) ;
#66058=DIRECTION('center_axis',(-1.,-1.77635683940026E-14,0.)) ;
#66059=DIRECTION('ref_axis',(1.25607396694692E-14,-0.707106781186485,-0.70710678118661)) ;
#66060=DIRECTION('',(1.,1.77635683940026E-14,0.)) ;
#66061=DIRECTION('center_axis',(-0.70710678118661,-0.707106781186485,0.)) ;
#66062=DIRECTION('ref_axis',(0.707106781186485,-0.70710678118661,0.)) ;
#66063=DIRECTION('center_axis',(6.53072367426566E-15,-1.,0.)) ;
#66064=DIRECTION('ref_axis',(0.707106781186548,4.61791899612877E-15,-0.707106781186548)) ;
#66065=DIRECTION('',(6.53072367426566E-15,-1.,0.)) ;
#66066=DIRECTION('',(-6.53072367426566E-15,1.,0.)) ;
#66067=DIRECTION('center_axis',(-1.,-6.53072367426566E-15,0.)) ;
#66068=DIRECTION('ref_axis',(6.53072367426566E-15,-1.,0.)) ;
#66069=DIRECTION('',(0.,0.,1.)) ;
#66070=DIRECTION('center_axis',(0.376618052248722,0.926368632197992,0.)) ;
#66071=DIRECTION('ref_axis',(-0.926368632197992,0.376618052248722,0.)) ;
#66072=DIRECTION('',(0.,0.,1.)) ;
#66073=DIRECTION('center_axis',(0.376618052248755,-0.926368632197979,0.)) ;
#66074=DIRECTION('ref_axis',(0.926368632197979,0.376618052248755,0.)) ;
#66075=DIRECTION('center_axis',(0.,0.,-1.)) ;
#66076=DIRECTION('ref_axis',(1.,0.,0.)) ;
#66077=DIRECTION('',(2.61228946970624E-14,1.,0.)) ;
#66078=DIRECTION('center_axis',(0.,0.,-1.)) ;
#66079=DIRECTION('ref_axis',(-0.999082519440321,-0.0428266196282222,0.)) ;
#66080=DIRECTION('',(0.,1.,0.)) ;
#66081=DIRECTION('center_axis',(0.,0.,-1.)) ;
#66082=DIRECTION('ref_axis',(-0.945182639171645,-0.326542154412755,0.)) ;
#66083=DIRECTION('center_axis',(0.,0.,-1.)) ;
#66084=DIRECTION('ref_axis',(0.945182639171645,-0.326542154412755,0.)) ;
#66085=DIRECTION('',(0.,-1.,0.)) ;
#66086=DIRECTION('center_axis',(0.,0.,-1.)) ;
#66087=DIRECTION('ref_axis',(0.999082519440321,-0.0428266196282222,0.)) ;
#66088=DIRECTION('',(0.,-1.,0.)) ;
#66089=DIRECTION('',(-1.,0.,0.)) ;
#66090=DIRECTION('center_axis',(0.,0.,1.)) ;
#66091=DIRECTION('ref_axis',(0.985598559653489,0.169101978725763,0.)) ;
#66092=DIRECTION('',(-1.,-8.88178419700144E-14,0.)) ;
#66093=DIRECTION('',(0.,-1.,0.)) ;
#66094=DIRECTION('',(1.,0.,0.)) ;
#66095=DIRECTION('',(0.,1.,0.)) ;
#66096=DIRECTION('',(2.22044604925036E-14,-1.,0.)) ;
#66097=DIRECTION('',(1.,-1.77635683940026E-14,0.)) ;
#66098=DIRECTION('',(-6.53072367426566E-15,-1.,0.)) ;
#66099=DIRECTION('',(0.926368632197986,0.376618052248738,0.)) ;
#66100=DIRECTION('',(-0.926368632197979,0.376618052248755,0.)) ;
#66101=DIRECTION('',(-6.53072367426566E-15,-1.,0.)) ;
#66102=DIRECTION('',(-1.,0.,0.)) ;
#66103=DIRECTION('center_axis',(1.,8.88178419700144E-14,0.)) ;
#66104=DIRECTION('ref_axis',(-6.28036983473468E-14,0.707106781186485,-0.70710678118661)) ;
#66105=DIRECTION('center_axis',(0.70710678118661,-0.707106781186485,0.)) ;
#66106=DIRECTION('ref_axis',(-0.707106781186485,-0.70710678118661,0.)) ;
#66107=DIRECTION('center_axis',(-0.70710678118661,-0.707106781186485,0.)) ;
#66108=DIRECTION('ref_axis',(-0.707106781186485,0.70710678118661,0.)) ;
#66109=DIRECTION('center_axis',(0.,-1.,0.)) ;
#66110=DIRECTION('ref_axis',(0.707106781186548,0.,-0.707106781186548)) ;
#66111=DIRECTION('center_axis',(-0.70710678118661,-0.707106781186485,0.)) ;
#66112=DIRECTION('ref_axis',(-0.707106781186485,0.70710678118661,0.)) ;
#66113=DIRECTION('center_axis',(-1.,0.,0.)) ;
#66114=DIRECTION('ref_axis',(0.,-0.707106781186736,-0.707106781186359)) ;
#66115=DIRECTION('',(-1.,0.,0.)) ;
#66116=DIRECTION('center_axis',(-0.70710678118661,0.707106781186485,0.)) ;
#66117=DIRECTION('ref_axis',(0.707106781186485,0.70710678118661,0.)) ;
#66118=DIRECTION('center_axis',(0.,1.,0.)) ;
#66119=DIRECTION('ref_axis',(-0.707106781186548,0.,-0.707106781186548)) ;
#66120=DIRECTION('',(0.,1.,0.)) ;
#66121=DIRECTION('center_axis',(1.,0.,0.)) ;
#66122=DIRECTION('ref_axis',(0.,1.,0.)) ;
#66123=DIRECTION('',(0.,0.,1.)) ;
#66124=DIRECTION('center_axis',(-2.22044604925036E-14,1.,0.)) ;
#66125=DIRECTION('ref_axis',(-0.707106781186548,-1.57009245868381E-14,-0.707106781186548)) ;
#66126=DIRECTION('center_axis',(0.70710678118661,0.707106781186485,0.)) ;
#66127=DIRECTION('ref_axis',(0.707106781186485,-0.70710678118661,0.)) ;
#66128=DIRECTION('',(-2.22044604925036E-14,1.,0.)) ;
#66129=DIRECTION('center_axis',(0.70710678118661,-0.707106781186485,0.)) ;
#66130=DIRECTION('ref_axis',(-0.707106781186485,-0.70710678118661,0.)) ;
#66131=DIRECTION('center_axis',(1.,0.,0.)) ;
#66132=DIRECTION('ref_axis',(0.,0.707106781186736,-0.707106781186359)) ;
#66133=DIRECTION('center_axis',(0.707106781186579,0.707106781186516,0.)) ;
#66134=DIRECTION('ref_axis',(-0.707106781186516,0.707106781186579,0.)) ;
#66135=DIRECTION('',(1.,0.,0.)) ;
#66136=DIRECTION('center_axis',(6.53072367426566E-15,1.,0.)) ;
#66137=DIRECTION('ref_axis',(-0.707106781186548,4.61791899612877E-15,-0.707106781186548)) ;
#66138=DIRECTION('center_axis',(0.829643915257864,0.558292910465109,0.)) ;
#66139=DIRECTION('ref_axis',(0.558292910465109,-0.829643915257864,0.)) ;
#66140=DIRECTION('center_axis',(0.926368632197979,-0.376618052248755,0.)) ;
#66141=DIRECTION('ref_axis',(0.266309178662367,0.655041541705704,-0.707106781186541)) ;
#66142=DIRECTION('center_axis',(1.33801610590799E-13,-1.,0.)) ;
#66143=DIRECTION('ref_axis',(-1.,-1.33801610590799E-13,0.)) ;
#66144=DIRECTION('center_axis',(-0.926368632197986,-0.376618052248738,0.)) ;
#66145=DIRECTION('ref_axis',(0.266309178662354,-0.655041541705708,-0.707106781186541)) ;
#66146=DIRECTION('center_axis',(-0.829643915257841,0.558292910465143,0.)) ;
#66147=DIRECTION('ref_axis',(0.558292910465143,0.829643915257841,0.)) ;
#66148=DIRECTION('center_axis',(6.53072367426566E-15,1.,0.)) ;
#66149=DIRECTION('ref_axis',(-0.707106781186548,4.61791899612877E-15,-0.707106781186548)) ;
#66150=DIRECTION('center_axis',(-0.70710678118661,0.707106781186485,0.)) ;
#66151=DIRECTION('ref_axis',(-0.707106781186485,-0.70710678118661,0.)) ;
#66152=DIRECTION('center_axis',(-1.,1.77635683940026E-14,0.)) ;
#66153=DIRECTION('ref_axis',(-1.25607396694736E-14,-0.707106781186736,-0.707106781186359)) ;
#66154=DIRECTION('',(-1.,1.77635683940026E-14,0.)) ;
#66155=DIRECTION('center_axis',(1.77635683940026E-14,1.,0.)) ;
#66156=DIRECTION('ref_axis',(-1.,1.77635683940026E-14,0.)) ;
#66157=DIRECTION('',(0.,0.,1.)) ;
#66158=DIRECTION('center_axis',(1.,2.22044604925036E-14,0.)) ;
#66159=DIRECTION('ref_axis',(-2.22044604925036E-14,1.,0.)) ;
#66160=DIRECTION('',(0.,0.,1.)) ;
#66161=DIRECTION('center_axis',(-1.,0.,0.)) ;
#66162=DIRECTION('ref_axis',(0.,-0.707106781186736,-0.707106781186359)) ;
#66163=DIRECTION('center_axis',(-0.70710678118661,0.707106781186485,0.)) ;
#66164=DIRECTION('ref_axis',(0.707106781186485,0.70710678118661,0.)) ;
#66165=DIRECTION('center_axis',(-0.70710678118661,-0.707106781186485,0.)) ;
#66166=DIRECTION('ref_axis',(-0.707106781186485,0.70710678118661,0.)) ;
#66167=DIRECTION('center_axis',(0.,1.,0.)) ;
#66168=DIRECTION('ref_axis',(-0.707106781186548,0.,-0.707106781186548)) ;
#66169=DIRECTION('center_axis',(0.70710678118661,0.707106781186485,0.)) ;
#66170=DIRECTION('ref_axis',(0.707106781186485,-0.70710678118661,0.)) ;
#66171=DIRECTION('',(0.,1.,0.)) ;
#66172=DIRECTION('center_axis',(0.,-1.,0.)) ;
#66173=DIRECTION('ref_axis',(0.707106781186548,0.,-0.707106781186548)) ;
#66174=DIRECTION('center_axis',(-0.70710678118661,0.707106781186485,0.)) ;
#66175=DIRECTION('ref_axis',(0.707106781186485,0.70710678118661,0.)) ;
#66176=DIRECTION('center_axis',(1.,0.,0.)) ;
#66177=DIRECTION('ref_axis',(0.,0.707106781186736,-0.707106781186359)) ;
#66178=DIRECTION('',(1.,0.,0.)) ;
#66179=DIRECTION('center_axis',(1.32407757812447E-14,1.,0.)) ;
#66180=DIRECTION('ref_axis',(-0.707106781186485,9.36264234308791E-15,-0.70710678118661)) ;
#66181=DIRECTION('',(1.32407757812447E-14,1.,0.)) ;
#66182=DIRECTION('center_axis',(0.,-1.,0.)) ;
#66183=DIRECTION('ref_axis',(-1.,0.,0.)) ;
#66184=DIRECTION('center_axis',(-0.70710678118661,0.707106781186485,0.)) ;
#66185=DIRECTION('ref_axis',(-0.707106781186485,-0.70710678118661,0.)) ;
#66186=DIRECTION('center_axis',(-1.,-2.61228946970635E-14,0.)) ;
#66187=DIRECTION('ref_axis',(1.84716759845141E-14,-0.707106781186485,-0.70710678118661)) ;
#66188=DIRECTION('center_axis',(-0.558292910464982,0.82964391525795,4.95863714946571E-14)) ;
#66189=DIRECTION('ref_axis',(0.82964391525795,0.558292910464982,3.3368194657995E-14)) ;
#66190=DIRECTION('',(-1.,-2.61228946970635E-14,0.)) ;
#66191=DIRECTION('center_axis',(0.376618052248709,0.926368632197998,0.)) ;
#66192=DIRECTION('ref_axis',(-0.655041541705793,0.266309178662365,-0.707106781186459)) ;
#66193=DIRECTION('center_axis',(1.,-6.69008052953881E-14,0.)) ;
#66194=DIRECTION('ref_axis',(-6.69008052953881E-14,-1.,0.)) ;
#66195=DIRECTION('center_axis',(0.376618052248766,-0.926368632197974,0.)) ;
#66196=DIRECTION('ref_axis',(0.655041541705581,0.266309178662326,-0.70710678118667)) ;
#66197=DIRECTION('center_axis',(-0.558292910465075,-0.829643915257887,0.)) ;
#66198=DIRECTION('ref_axis',(-0.829643915257887,0.558292910465075,0.)) ;
#66199=DIRECTION('center_axis',(-1.,-2.61228946970635E-14,0.)) ;
#66200=DIRECTION('ref_axis',(1.84716759845206E-14,-0.707106781186736,-0.707106781186359)) ;
#66201=DIRECTION('center_axis',(-0.70710678118661,-0.707106781186485,0.)) ;
#66202=DIRECTION('ref_axis',(0.707106781186485,-0.70710678118661,0.)) ;
#66203=DIRECTION('center_axis',(0.846331659376499,0.532656289118059,0.)) ;
#66204=DIRECTION('ref_axis',(-0.376644874076998,0.598446855477916,-0.70710678118663)) ;
#66205=DIRECTION('center_axis',(-0.846331659376493,-0.53265628911807,0.)) ;
#66206=DIRECTION('ref_axis',(-0.53265628911807,0.846331659376493,0.)) ;
#66207=DIRECTION('center_axis',(-0.846331659376477,-0.532656289118094,0.)) ;
#66208=DIRECTION('ref_axis',(-0.376644874077023,0.598446855477901,-0.70710678118663)) ;
#66209=DIRECTION('center_axis',(0.,0.,-1.)) ;
#66210=DIRECTION('ref_axis',(-1.,0.,0.)) ;
#66211=DIRECTION('center_axis',(0.,1.,0.)) ;
#66212=DIRECTION('ref_axis',(1.,0.,0.)) ;
#66213=DIRECTION('center_axis',(-8.82718385416297E-15,-1.,0.)) ;
#66214=DIRECTION('ref_axis',(0.707106781186548,-6.24176156205904E-15,-0.707106781186548)) ;
#66215=DIRECTION('center_axis',(0.,0.,1.)) ;
#66216=DIRECTION('ref_axis',(1.,0.,0.)) ;
#66217=DIRECTION('center_axis',(0.846331659376392,0.53265628911823,0.)) ;
#66218=DIRECTION('ref_axis',(0.53265628911823,-0.846331659376392,0.)) ;
#66219=DIRECTION('center_axis',(0.,0.,1.)) ;
#66220=DIRECTION('ref_axis',(0.483396168210882,0.875401704681363,0.)) ;
#66221=DIRECTION('center_axis',(-0.846331659376486,-0.532656289118079,0.)) ;
#66222=DIRECTION('ref_axis',(0.376644874077126,-0.598446855478087,-0.707106781186417)) ;
#66223=DIRECTION('center_axis',(-0.846331659376477,-0.532656289118094,0.)) ;
#66224=DIRECTION('ref_axis',(0.376644874077136,-0.598446855478081,-0.707106781186417)) ;
#66225=DIRECTION('',(-0.846331659376486,-0.532656289118079,0.)) ;
#66226=DIRECTION('center_axis',(-0.532656289118079,0.846331659376486,0.)) ;
#66227=DIRECTION('ref_axis',(-0.846331659376486,-0.532656289118079,0.)) ;
#66228=DIRECTION('',(0.,0.,1.)) ;
#66229=DIRECTION('',(0.,0.,1.)) ;
#66230=DIRECTION('center_axis',(0.,0.,1.)) ;
#66231=DIRECTION('ref_axis',(-0.532656289118115,0.846331659376464,0.)) ;
#66232=DIRECTION('',(0.,0.,1.)) ;
#66233=DIRECTION('center_axis',(1.,-1.32407757812447E-14,0.)) ;
#66234=DIRECTION('ref_axis',(1.32407757812447E-14,1.,0.)) ;
#66235=DIRECTION('',(0.,0.,1.)) ;
#66236=DIRECTION('center_axis',(-2.61228946970635E-14,1.,0.)) ;
#66237=DIRECTION('ref_axis',(-1.,-2.61228946970635E-14,0.)) ;
#66238=DIRECTION('center_axis',(-0.532656289118094,0.846331659376477,0.)) ;
#66239=DIRECTION('ref_axis',(-0.598446855478002,-0.376644874077087,-0.70710678118651)) ;
#66240=DIRECTION('center_axis',(0.221801981400932,0.975091729555031,1.96999733327036E-14)) ;
#66241=DIRECTION('ref_axis',(0.97509172955503,-0.221801981400932,1.96999733327025E-14)) ;
#66242=DIRECTION('',(-0.532656289118094,0.846331659376477,0.)) ;
#66243=DIRECTION('center_axis',(0.975091729555058,-0.221801981400812,0.)) ;
#66244=DIRECTION('ref_axis',(-0.221801981400812,-0.975091729555058,0.)) ;
#66245=DIRECTION('center_axis',(-1.32407757812447E-14,-1.,0.)) ;
#66246=DIRECTION('ref_axis',(0.707106781186548,-9.36264234308873E-15,-0.707106781186548)) ;
#66247=DIRECTION('',(-1.32407757812447E-14,-1.,0.)) ;
#66248=DIRECTION('center_axis',(0.,1.,0.)) ;
#66249=DIRECTION('ref_axis',(1.,0.,0.)) ;
#66250=DIRECTION('center_axis',(0.70710678118661,-0.707106781186485,0.)) ;
#66251=DIRECTION('ref_axis',(0.707106781186485,0.70710678118661,0.)) ;
#66252=DIRECTION('center_axis',(1.,2.61228946970635E-14,0.)) ;
#66253=DIRECTION('ref_axis',(-1.84716759845141E-14,0.707106781186485,-0.70710678118661)) ;
#66254=DIRECTION('center_axis',(0.558292910464982,-0.82964391525795,0.)) ;
#66255=DIRECTION('ref_axis',(-0.82964391525795,-0.558292910464982,0.)) ;
#66256=DIRECTION('center_axis',(-0.376618052248709,-0.926368632197998,0.)) ;
#66257=DIRECTION('ref_axis',(0.655041541705652,-0.266309178662307,-0.707106781186612)) ;
#66258=DIRECTION('center_axis',(-1.,3.3450402647694E-14,-8.88178419700124E-14)) ;
#66259=DIRECTION('ref_axis',(3.34504026476972E-14,1.,-3.61091702428531E-14)) ;
#66260=DIRECTION('center_axis',(-0.376618052248766,0.926368632197974,0.)) ;
#66261=DIRECTION('ref_axis',(-0.655041541705635,-0.266309178662348,-0.707106781186612)) ;
#66262=DIRECTION('center_axis',(0.558292910465098,0.829643915257871,0.)) ;
#66263=DIRECTION('ref_axis',(0.829643915257871,-0.558292910465098,0.)) ;
#66264=DIRECTION('center_axis',(1.,2.61228946970635E-14,0.)) ;
#66265=DIRECTION('ref_axis',(-1.84716759845206E-14,0.707106781186736,-0.707106781186359)) ;
#66266=DIRECTION('center_axis',(0.70710678118661,0.707106781186485,0.)) ;
#66267=DIRECTION('ref_axis',(-0.707106781186485,0.70710678118661,0.)) ;
#66268=DIRECTION('center_axis',(0.,0.,1.)) ;
#66269=DIRECTION('ref_axis',(1.,0.,0.)) ;
#66270=DIRECTION('center_axis',(-0.846331659376392,-0.53265628911823,0.)) ;
#66271=DIRECTION('ref_axis',(-0.53265628911823,0.846331659376392,0.)) ;
#66272=DIRECTION('center_axis',(0.,0.,1.)) ;
#66273=DIRECTION('ref_axis',(-0.483396168210882,-0.875401704681363,0.)) ;
#66274=DIRECTION('center_axis',(0.846331659376489,0.532656289118076,0.)) ;
#66275=DIRECTION('ref_axis',(-0.376644874077123,0.598446855478089,-0.707106781186417)) ;
#66276=DIRECTION('',(0.846331659376489,0.532656289118076,0.)) ;
#66277=DIRECTION('center_axis',(-0.846331659376502,-0.532656289118055,0.)) ;
#66278=DIRECTION('ref_axis',(0.376644874076995,-0.598446855477918,-0.70710678118663)) ;
#66279=DIRECTION('',(-0.846331659376502,-0.532656289118055,0.)) ;
#66280=DIRECTION('center_axis',(0.846331659376493,0.53265628911807,0.)) ;
#66281=DIRECTION('ref_axis',(0.53265628911807,-0.846331659376493,0.)) ;
#66282=DIRECTION('center_axis',(0.,0.,-1.)) ;
#66283=DIRECTION('ref_axis',(-1.,0.,0.)) ;
#66284=DIRECTION('center_axis',(0.,-1.,0.)) ;
#66285=DIRECTION('ref_axis',(-1.,0.,0.)) ;
#66286=DIRECTION('center_axis',(8.82718385416297E-15,1.,0.)) ;
#66287=DIRECTION('ref_axis',(-0.707106781186548,6.24176156205904E-15,-0.707106781186548)) ;
#66288=DIRECTION('center_axis',(-0.532656289118055,0.846331659376502,0.)) ;
#66289=DIRECTION('ref_axis',(-0.846331659376502,-0.532656289118055,0.)) ;
#66290=DIRECTION('',(0.,0.,1.)) ;
#66291=DIRECTION('center_axis',(0.846331659376477,0.532656289118094,0.)) ;
#66292=DIRECTION('ref_axis',(-0.532656289118094,0.846331659376477,0.)) ;
#66293=DIRECTION('',(0.,0.,1.)) ;
#66294=DIRECTION('center_axis',(0.532656289118076,-0.846331659376489,0.)) ;
#66295=DIRECTION('ref_axis',(0.846331659376489,0.532656289118076,0.)) ;
#66296=DIRECTION('',(0.,0.,1.)) ;
#66297=DIRECTION('center_axis',(0.,0.,1.)) ;
#66298=DIRECTION('ref_axis',(0.532656289118115,-0.846331659376464,0.)) ;
#66299=DIRECTION('',(0.,0.,1.)) ;
#66300=DIRECTION('center_axis',(-1.,1.32407757812447E-14,0.)) ;
#66301=DIRECTION('ref_axis',(-1.32407757812447E-14,-1.,0.)) ;
#66302=DIRECTION('center_axis',(-0.846331659376477,-0.532656289118094,0.)) ;
#66303=DIRECTION('ref_axis',(0.532656289118094,-0.846331659376477,0.)) ;
#66304=DIRECTION('center_axis',(1.,0.,0.)) ;
#66305=DIRECTION('ref_axis',(0.,1.,0.)) ;
#66306=DIRECTION('',(0.,0.,1.)) ;
#66307=DIRECTION('center_axis',(0.,-1.,0.)) ;
#66308=DIRECTION('ref_axis',(1.,0.,0.)) ;
#66309=DIRECTION('center_axis',(0.,1.,0.)) ;
#66310=DIRECTION('ref_axis',(-1.,0.,0.)) ;
#66311=DIRECTION('center_axis',(0.42261826174069,0.906307787036654,0.)) ;
#66312=DIRECTION('ref_axis',(-0.906307787036654,0.42261826174069,0.)) ;
#66313=DIRECTION('center_axis',(0.,-1.,0.)) ;
#66314=DIRECTION('ref_axis',(1.,0.,0.)) ;
#66315=DIRECTION('center_axis',(2.46519032881572E-32,8.55284707229503E-50,
-1.)) ;
#66316=DIRECTION('ref_axis',(1.,-2.20382687031672E-110,2.46519032881572E-32)) ;
#66317=DIRECTION('',(1.,0.,2.46519032881572E-32)) ;
#66318=DIRECTION('',(-3.67742382159233E-14,-1.,0.)) ;
#66319=DIRECTION('center_axis',(0.,0.,-1.)) ;
#66320=DIRECTION('ref_axis',(1.,0.,0.)) ;
#66321=DIRECTION('',(1.,0.,0.)) ;
#66322=DIRECTION('center_axis',(0.,0.,-1.)) ;
#66323=DIRECTION('ref_axis',(0.945182639171645,-0.326542154412755,0.)) ;
#66324=DIRECTION('',(0.,-1.,0.)) ;
#66325=DIRECTION('center_axis',(0.,0.,-1.)) ;
#66326=DIRECTION('ref_axis',(0.99891280361996,0.0466177086965058,0.)) ;
#66327=DIRECTION('',(0.,-1.,0.)) ;
#66328=DIRECTION('',(-1.,0.,0.)) ;
#66329=DIRECTION('center_axis',(1.,0.,0.)) ;
#66330=DIRECTION('ref_axis',(0.,-1.,0.)) ;
#66331=DIRECTION('',(0.,0.,-1.)) ;
#66332=DIRECTION('center_axis',(0.,0.,-1.)) ;
#66333=DIRECTION('ref_axis',(-0.819152044288993,-0.573576436351044,0.)) ;
#66334=DIRECTION('',(0.,0.,-1.)) ;
#66335=DIRECTION('center_axis',(-3.21481891221798E-49,-2.25104043631415E-49,
-1.)) ;
#66336=DIRECTION('ref_axis',(-0.819152044288993,-0.573576436351044,3.92456923550545E-49)) ;
#66337=DIRECTION('center_axis',(1.,-1.46896958313692E-15,0.)) ;
#66338=DIRECTION('ref_axis',(-1.46896958313692E-15,-1.,9.70774749479708E-52)) ;
#66339=DIRECTION('',(0.,0.,-1.)) ;
#66340=DIRECTION('',(-1.46896958313692E-15,-1.,9.70774749479708E-52)) ;
#66341=DIRECTION('center_axis',(0.,0.,-1.)) ;
#66342=DIRECTION('ref_axis',(0.,1.,0.)) ;
#66343=DIRECTION('',(0.,0.,-1.)) ;
#66344=DIRECTION('center_axis',(0.,0.,-1.)) ;
#66345=DIRECTION('ref_axis',(0.,1.,0.)) ;
#66346=DIRECTION('center_axis',(4.35522519302374E-15,1.,0.)) ;
#66347=DIRECTION('ref_axis',(1.,-4.35522519302374E-15,-1.99220223446153E-34)) ;
#66348=DIRECTION('',(0.,0.,-1.)) ;
#66349=DIRECTION('',(1.,-4.35522519302374E-15,-1.99220223446153E-34)) ;
#66350=DIRECTION('center_axis',(1.,0.,0.)) ;
#66351=DIRECTION('ref_axis',(0.,-1.,5.60383084497476E-34)) ;
#66352=DIRECTION('',(0.,0.,-1.)) ;
#66353=DIRECTION('',(0.,-1.,5.60383084497476E-34)) ;
#66354=DIRECTION('center_axis',(0.,1.,0.)) ;
#66355=DIRECTION('ref_axis',(1.,0.,0.)) ;
#66356=DIRECTION('',(0.,0.,-1.)) ;
#66357=DIRECTION('',(-1.,0.,0.)) ;
#66358=DIRECTION('center_axis',(-8.11022789614398E-33,1.15826058041052E-32,
-1.)) ;
#66359=DIRECTION('ref_axis',(1.,-2.17980433592234E-81,-8.11022789614398E-33)) ;
#66360=DIRECTION('',(8.07434927000127E-15,1.,9.03922915636472E-64)) ;
#66361=DIRECTION('center_axis',(-6.80308557388104E-64,1.462910905831E-62,
-1.)) ;
#66362=DIRECTION('ref_axis',(-1.06581410364006E-13,-1.,-1.46291090583099E-62)) ;
#66363=DIRECTION('center_axis',(0.,0.,-1.)) ;
#66364=DIRECTION('ref_axis',(-1.06581410364006E-13,-1.,0.)) ;
#66365=DIRECTION('',(0.,0.,-1.)) ;
#66366=DIRECTION('center_axis',(-6.80308557388104E-64,1.462910905831E-62,
-1.)) ;
#66367=DIRECTION('ref_axis',(-1.06581410364006E-13,-1.,-1.46291090583099E-62)) ;
#66368=DIRECTION('center_axis',(-1.,8.07434927000127E-15,0.)) ;
#66369=DIRECTION('ref_axis',(8.07434927000127E-15,1.,9.03922915636472E-64)) ;
#66370=DIRECTION('',(0.,0.,-1.)) ;
#66371=DIRECTION('',(8.07434927000127E-15,1.,9.03922915636472E-64)) ;
#66372=DIRECTION('center_axis',(-1.,-1.30614473485314E-15,0.)) ;
#66373=DIRECTION('ref_axis',(-1.30614473485314E-15,1.,0.)) ;
#66374=DIRECTION('',(0.,0.,-1.)) ;
#66375=DIRECTION('center_axis',(0.,1.,0.)) ;
#66376=DIRECTION('ref_axis',(1.,0.,0.)) ;
#66377=DIRECTION('center_axis',(1.,1.34572487833352E-15,0.)) ;
#66378=DIRECTION('ref_axis',(1.34572487833352E-15,-1.,0.)) ;
#66379=DIRECTION('',(0.,0.,-1.)) ;
#66380=DIRECTION('',(1.34572487833352E-15,-1.,0.)) ;
#66381=DIRECTION('',(0.,0.,-1.)) ;
#66382=DIRECTION('center_axis',(1.,0.,0.)) ;
#66383=DIRECTION('ref_axis',(0.,1.,0.)) ;
#66384=DIRECTION('',(0.,1.,0.)) ;
#66385=DIRECTION('',(0.,0.,1.)) ;
#66386=DIRECTION('center_axis',(1.97372982155583E-14,1.,0.)) ;
#66387=DIRECTION('ref_axis',(-1.,1.97372982155583E-14,0.)) ;
#66388=DIRECTION('',(-1.,1.97372982155583E-14,0.)) ;
#66389=DIRECTION('',(0.,0.,1.)) ;
#66390=DIRECTION('center_axis',(-1.,-7.40148683083432E-15,0.)) ;
#66391=DIRECTION('ref_axis',(7.40148683083432E-15,-1.,0.)) ;
#66392=DIRECTION('',(7.40148683083432E-15,-1.,0.)) ;
#66393=DIRECTION('center_axis',(0.,0.,-1.)) ;
#66394=DIRECTION('ref_axis',(1.,0.,0.)) ;
#66395=DIRECTION('center_axis',(6.22031196910783E-15,1.,0.)) ;
#66396=DIRECTION('ref_axis',(-1.,6.22031196910783E-15,0.)) ;
#66397=DIRECTION('',(1.,-9.87859509815899E-15,0.)) ;
#66398=DIRECTION('',(0.,0.,1.)) ;
#66399=DIRECTION('',(-1.,6.22031196910783E-15,0.)) ;
#66400=DIRECTION('',(0.,0.,1.)) ;
#66401=DIRECTION('center_axis',(0.,0.,1.)) ;
#66402=DIRECTION('ref_axis',(1.,0.,0.)) ;
#66403=DIRECTION('',(0.,0.,1.)) ;
#66404=DIRECTION('center_axis',(0.,0.,1.)) ;
#66405=DIRECTION('ref_axis',(1.,0.,0.)) ;
#66406=DIRECTION('',(0.,0.,1.)) ;
#66407=DIRECTION('center_axis',(-1.,-2.22044604925032E-15,0.)) ;
#66408=DIRECTION('ref_axis',(2.22044604925032E-15,-1.,0.)) ;
#66409=DIRECTION('',(2.22044604925032E-15,-1.,0.)) ;
#66410=DIRECTION('center_axis',(1.,1.11022302462516E-14,0.)) ;
#66411=DIRECTION('ref_axis',(-1.11022302462516E-14,1.,0.)) ;
#66412=DIRECTION('',(-1.11022302462516E-14,1.,0.)) ;
#66413=DIRECTION('center_axis',(0.,0.,-1.)) ;
#66414=DIRECTION('ref_axis',(1.,0.,0.)) ;
#66415=DIRECTION('center_axis',(0.,0.,-1.)) ;
#66416=DIRECTION('ref_axis',(-0.180669743412801,-0.983543818960372,0.)) ;
#66417=DIRECTION('',(0.,0.,1.)) ;
#66418=DIRECTION('center_axis',(0.,0.,-1.)) ;
#66419=DIRECTION('ref_axis',(-0.180669743412801,-0.983543818960372,0.)) ;
#66420=DIRECTION('center_axis',(1.37008135359091E-15,0.316227766016839,
-0.948683298050513)) ;
#66421=DIRECTION('ref_axis',(-1.,2.21856832751295E-31,-1.44419255235793E-15)) ;
#66422=DIRECTION('center_axis',(0.,0.,1.)) ;
#66423=DIRECTION('ref_axis',(1.,0.,0.)) ;
#66424=DIRECTION('center_axis',(0.,0.,1.)) ;
#66425=DIRECTION('ref_axis',(1.,0.,0.)) ;
#66426=DIRECTION('',(0.693108716251782,0.720833064901858,0.)) ;
#66427=DIRECTION('center_axis',(0.,0.,-1.)) ;
#66428=DIRECTION('ref_axis',(1.,0.,0.)) ;
#66429=DIRECTION('',(-0.707106781186547,0.707106781186547,0.)) ;
#66430=DIRECTION('',(0.693108716251782,0.720833064901858,0.)) ;
#66431=DIRECTION('',(-1.,0.,0.)) ;
#66432=DIRECTION('center_axis',(0.707106781186548,0.707106781186548,0.)) ;
#66433=DIRECTION('ref_axis',(0.,0.,-1.)) ;
#66434=DIRECTION('center_axis',(0.,0.,1.)) ;
#66435=DIRECTION('ref_axis',(-0.707106781186563,-0.707106781186532,0.)) ;
#66436=DIRECTION('',(0.,0.,1.)) ;
#66437=DIRECTION('center_axis',(0.,0.,1.)) ;
#66438=DIRECTION('ref_axis',(-0.707106781186563,-0.707106781186532,0.)) ;
#66439=DIRECTION('center_axis',(0.,1.,0.)) ;
#66440=DIRECTION('ref_axis',(-1.,0.,0.)) ;
#66441=DIRECTION('',(-1.,0.,0.)) ;
#66442=DIRECTION('center_axis',(0.,0.,-1.)) ;
#66443=DIRECTION('ref_axis',(0.707106781186555,-0.70710678118654,0.)) ;
#66444=DIRECTION('',(0.,0.,-1.)) ;
#66445=DIRECTION('center_axis',(0.720833064901858,-0.693108716251782,0.)) ;
#66446=DIRECTION('ref_axis',(0.,0.,-1.)) ;
#66447=DIRECTION('center_axis',(-1.,0.,0.)) ;
#66448=DIRECTION('ref_axis',(0.,1.,0.)) ;
#66449=DIRECTION('',(0.,0.,-1.)) ;
#66450=DIRECTION('center_axis',(0.,-1.,0.)) ;
#66451=DIRECTION('ref_axis',(-1.,0.,0.)) ;
#66452=DIRECTION('center_axis',(0.,-1.,0.)) ;
#66453=DIRECTION('ref_axis',(-1.,0.,0.)) ;
#66454=DIRECTION('center_axis',(-0.70710678118655,-8.10370301256138E-15,
-0.707106781186545)) ;
#66455=DIRECTION('ref_axis',(-0.707106781186545,-1.02766135666342E-31,0.70710678118655)) ;
#66456=DIRECTION('center_axis',(0.,1.,0.)) ;
#66457=DIRECTION('ref_axis',(-0.707106781186554,0.,-0.707106781186541)) ;
#66458=DIRECTION('',(0.,1.,0.)) ;
#66459=DIRECTION('center_axis',(0.,-0.901303236306861,-0.433188730489123)) ;
#66460=DIRECTION('ref_axis',(0.,-0.433188730489123,0.901303236306861)) ;
#66461=DIRECTION('center_axis',(0.234832610329562,-0.891105237687952,-0.388310572211089)) ;
#66462=DIRECTION('ref_axis',(0.461132845926743,0.453796711496567,-0.762512323206913)) ;
#66463=DIRECTION('center_axis',(-0.186041819180148,0.98254182685326,0.)) ;
#66464=DIRECTION('ref_axis',(0.,0.,-1.)) ;
#66465=DIRECTION('center_axis',(1.,0.,0.)) ;
#66466=DIRECTION('ref_axis',(0.,0.780868809443035,-0.624695047554418)) ;
#66467=DIRECTION('center_axis',(0.117465545166938,-0.620370257876694,-0.77546282234588)) ;
#66468=DIRECTION('ref_axis',(0.98254182685326,0.186041819180148,-2.37800624313497E-16)) ;
#66469=DIRECTION('center_axis',(0.,0.,1.)) ;
#66470=DIRECTION('ref_axis',(1.,0.,0.)) ;
#66471=DIRECTION('center_axis',(0.,0.,1.)) ;
#66472=DIRECTION('ref_axis',(0.998912803619959,0.0466177086965058,0.)) ;
#66473=DIRECTION('center_axis',(1.,0.,0.)) ;
#66474=DIRECTION('ref_axis',(0.,0.,-1.)) ;
#66475=DIRECTION('center_axis',(-1.,0.,0.)) ;
#66476=DIRECTION('ref_axis',(0.,0.433188730489175,-0.901303236306837)) ;
#66477=DIRECTION('',(1.,0.,0.)) ;
#66478=DIRECTION('center_axis',(0.503932575563369,0.863742993769599,0.)) ;
#66479=DIRECTION('ref_axis',(0.,0.,-1.)) ;
#66480=DIRECTION('center_axis',(-0.527005614249989,-0.600943043286542,-0.60094304328655)) ;
#66481=DIRECTION('ref_axis',(-0.751844328927355,0.65934065934066,8.09346471661972E-17)) ;
#66482=DIRECTION('center_axis',(0.,0.,1.)) ;
#66483=DIRECTION('ref_axis',(1.,0.,0.)) ;
#66484=DIRECTION('center_axis',(0.,-1.,0.)) ;
#66485=DIRECTION('ref_axis',(-1.,0.,0.)) ;
#66486=DIRECTION('center_axis',(0.,0.,1.)) ;
#66487=DIRECTION('ref_axis',(0.945182639171645,-0.326542154412755,0.)) ;
#66488=DIRECTION('center_axis',(0.,1.,0.)) ;
#66489=DIRECTION('ref_axis',(-0.707106781186554,0.,-0.707106781186541)) ;
#66490=DIRECTION('',(0.,1.,0.)) ;
#66491=DIRECTION('center_axis',(-1.,0.,0.)) ;
#66492=DIRECTION('ref_axis',(0.,-0.382683432365103,0.923879532511281)) ;
#66493=DIRECTION('center_axis',(0.234832610329551,-0.891105237687967,-0.388310572211061)) ;
#66494=DIRECTION('ref_axis',(0.461132845926749,0.453796711496559,-0.762512323206914)) ;
#66495=DIRECTION('center_axis',(-0.186041819180008,0.982541826853286,0.)) ;
#66496=DIRECTION('ref_axis',(0.,0.,-1.)) ;
#66497=DIRECTION('center_axis',(0.117465545166847,-0.620370257876695,-0.775462822345893)) ;
#66498=DIRECTION('ref_axis',(0.982541826853286,0.186041819180008,1.81771110290286E-17)) ;
#66499=DIRECTION('center_axis',(0.424264068711907,-0.565685424949239,-0.70710678118656)) ;
#66500=DIRECTION('ref_axis',(6.96661453349048E-17,0.780868809443035,-0.624695047554418)) ;
#66501=DIRECTION('center_axis',(0.,0.529998940003177,-0.84799830400509)) ;
#66502=DIRECTION('ref_axis',(0.,0.84799830400509,0.529998940003177)) ;
#66503=DIRECTION('center_axis',(-0.42426406871193,0.565685424949236,0.707106781186548)) ;
#66504=DIRECTION('ref_axis',(0.466804319685465,0.805744406458676,-0.364512933355658)) ;
#66505=DIRECTION('',(0.42426406871193,-0.565685424949236,-0.707106781186548)) ;
#66506=DIRECTION('center_axis',(0.,0.,1.)) ;
#66507=DIRECTION('ref_axis',(1.,0.,0.)) ;
#66508=DIRECTION('center_axis',(0.,0.,1.)) ;
#66509=DIRECTION('ref_axis',(0.999082519440321,-0.0428266196282222,0.)) ;
#66510=DIRECTION('center_axis',(0.,-1.,0.)) ;
#66511=DIRECTION('ref_axis',(-1.,0.,0.)) ;
#66512=DIRECTION('center_axis',(-0.503932575563422,0.863742993769568,6.1372630978665E-14)) ;
#66513=DIRECTION('ref_axis',(0.863742993769568,0.503932575563422,6.75875089903394E-31)) ;
#66514=DIRECTION('center_axis',(0.527005614249974,-0.600943043286547,-0.600943043286559)) ;
#66515=DIRECTION('ref_axis',(-3.7754359406558E-16,0.707106781186554,-0.707106781186541)) ;
#66516=DIRECTION('center_axis',(0.,-1.,0.)) ;
#66517=DIRECTION('ref_axis',(0.707106781186554,0.,-0.707106781186541)) ;
#66518=DIRECTION('',(0.,-1.,0.)) ;
#66519=DIRECTION('center_axis',(0.,1.,0.)) ;
#66520=DIRECTION('ref_axis',(1.,0.,0.)) ;
#66521=DIRECTION('center_axis',(0.,0.,1.)) ;
#66522=DIRECTION('ref_axis',(1.,0.,0.)) ;
#66523=DIRECTION('center_axis',(0.,0.,1.)) ;
#66524=DIRECTION('ref_axis',(-0.945182639171645,-0.326542154412755,0.)) ;
#66525=DIRECTION('center_axis',(0.,-0.74695627272243,0.664873165829855)) ;
#66526=DIRECTION('ref_axis',(0.,-0.664873165829855,-0.74695627272243)) ;
#66527=DIRECTION('center_axis',(0.503932575563377,0.863742993769594,0.)) ;
#66528=DIRECTION('ref_axis',(0.,0.,-1.)) ;
#66529=DIRECTION('center_axis',(-0.527005614249989,-0.600943043286542,-0.60094304328655)) ;
#66530=DIRECTION('ref_axis',(-0.751844328927355,0.65934065934066,8.09346471661972E-17)) ;
#66531=DIRECTION('center_axis',(0.,0.,1.)) ;
#66532=DIRECTION('ref_axis',(1.,0.,0.)) ;
#66533=DIRECTION('center_axis',(0.,-1.,0.)) ;
#66534=DIRECTION('ref_axis',(-1.,0.,0.)) ;
#66535=DIRECTION('center_axis',(0.,0.,1.)) ;
#66536=DIRECTION('ref_axis',(0.945182639171645,-0.326542154412755,0.)) ;
#66537=DIRECTION('center_axis',(0.,1.,0.)) ;
#66538=DIRECTION('ref_axis',(-0.707106781186541,0.,-0.707106781186554)) ;
#66539=DIRECTION('',(0.,1.,0.)) ;
#66540=DIRECTION('center_axis',(-0.50393257556343,0.863742993769564,6.13726309786647E-14)) ;
#66541=DIRECTION('ref_axis',(0.863742993769564,0.50393257556343,-3.71214407864697E-30)) ;
#66542=DIRECTION('center_axis',(0.527005614249974,-0.600943043286547,-0.600943043286559)) ;
#66543=DIRECTION('ref_axis',(-3.7754359406558E-16,0.707106781186554,-0.707106781186541)) ;
#66544=DIRECTION('center_axis',(0.,-1.,0.)) ;
#66545=DIRECTION('ref_axis',(0.707106781186541,0.,-0.707106781186554)) ;
#66546=DIRECTION('',(0.,-1.,0.)) ;
#66547=DIRECTION('center_axis',(0.,1.,0.)) ;
#66548=DIRECTION('ref_axis',(1.,0.,0.)) ;
#66549=DIRECTION('center_axis',(0.,0.,1.)) ;
#66550=DIRECTION('ref_axis',(1.,0.,0.)) ;
#66551=DIRECTION('center_axis',(0.,0.,1.)) ;
#66552=DIRECTION('ref_axis',(-0.945182639171645,-0.326542154412755,0.)) ;
#66553=DIRECTION('center_axis',(0.,-0.74695627272243,0.664873165829855)) ;
#66554=DIRECTION('ref_axis',(0.,-0.664873165829855,-0.74695627272243)) ;
#66555=DIRECTION('center_axis',(0.,-1.,0.)) ;
#66556=DIRECTION('ref_axis',(0.707106781186541,0.,-0.707106781186554)) ;
#66557=DIRECTION('center_axis',(0.,-1.,0.)) ;
#66558=DIRECTION('ref_axis',(0.,0.,-1.)) ;
#66559=DIRECTION('',(0.,-1.,0.)) ;
#66560=DIRECTION('center_axis',(0.,1.,0.)) ;
#66561=DIRECTION('ref_axis',(1.,0.,0.)) ;
#66562=DIRECTION('center_axis',(0.,0.,1.)) ;
#66563=DIRECTION('ref_axis',(1.,0.,0.)) ;
#66564=DIRECTION('center_axis',(0.,0.,1.)) ;
#66565=DIRECTION('ref_axis',(-0.999082519440321,-0.0428266196282222,0.)) ;
#66566=DIRECTION('center_axis',(0.,0.,-1.)) ;
#66567=DIRECTION('ref_axis',(0.985598559653495,0.169101978725727,0.)) ;
#66568=DIRECTION('center_axis',(0.,1.,0.)) ;
#66569=DIRECTION('ref_axis',(-0.707106781186548,0.,-0.707106781186548)) ;
#66570=DIRECTION('',(0.,1.,0.)) ;
#66571=DIRECTION('center_axis',(-2.61228946970624E-14,-1.,0.)) ;
#66572=DIRECTION('ref_axis',(0.707106781186554,-1.84716759845151E-14,-0.707106781186541)) ;
#66573=DIRECTION('center_axis',(0.,-1.,0.)) ;
#66574=DIRECTION('ref_axis',(0.,0.,-1.)) ;
#66575=DIRECTION('',(-2.61228946970624E-14,-1.,0.)) ;
#66576=DIRECTION('center_axis',(0.,1.,0.)) ;
#66577=DIRECTION('ref_axis',(1.,0.,0.)) ;
#66578=DIRECTION('center_axis',(0.,0.,1.)) ;
#66579=DIRECTION('ref_axis',(1.,0.,0.)) ;
#66580=DIRECTION('center_axis',(0.,0.,1.)) ;
#66581=DIRECTION('ref_axis',(-0.999082519440321,-0.0428266196282222,0.)) ;
#66582=DIRECTION('center_axis',(-0.640000000000002,-0.479999999999999,-0.599999999999999)) ;
#66583=DIRECTION('ref_axis',(-0.332851351149329,0.876990532021574,-0.346550984391306)) ;
#66584=DIRECTION('center_axis',(0.,-1.,0.)) ;
#66585=DIRECTION('ref_axis',(-0.729537204140087,0.,-0.683941128881328)) ;
#66586=DIRECTION('',(-0.640000000000002,-0.479999999999999,-0.599999999999999)) ;
#66587=DIRECTION('center_axis',(0.640000000000011,0.479999999999994,0.599999999999994)) ;
#66588=DIRECTION('ref_axis',(-1.29788565499151E-16,0.780868809443031,-0.624695047554423)) ;
#66589=DIRECTION('',(0.640000000000002,0.479999999999998,0.599999999999999)) ;
#66590=DIRECTION('center_axis',(0.,0.529998940003175,-0.847998304005091)) ;
#66591=DIRECTION('ref_axis',(0.,0.847998304005091,0.529998940003175)) ;
#66592=DIRECTION('center_axis',(0.,-0.780868809443031,0.624695047554424)) ;
#66593=DIRECTION('ref_axis',(8.66938531455285E-17,0.624695047554424,0.780868809443031)) ;
#66594=DIRECTION('center_axis',(0.,0.,-1.)) ;
#66595=DIRECTION('ref_axis',(0.985598559653489,0.169101978725763,0.)) ;
#66596=DIRECTION('center_axis',(0.42426406871193,-0.565685424949232,-0.707106781186552)) ;
#66597=DIRECTION('ref_axis',(-1.36184273839256E-16,0.780868809443035,-0.624695047554418)) ;
#66598=DIRECTION('center_axis',(0.,0.529998940003175,-0.847998304005091)) ;
#66599=DIRECTION('ref_axis',(0.,0.847998304005091,0.529998940003175)) ;
#66600=DIRECTION('center_axis',(0.,-0.780868809443031,0.624695047554424)) ;
#66601=DIRECTION('ref_axis',(0.,0.624695047554424,0.780868809443031)) ;
#66602=DIRECTION('center_axis',(-0.424264068711912,0.565685424949242,0.707106781186554)) ;
#66603=DIRECTION('ref_axis',(0.466804319685494,0.805744406458664,-0.364512933355647)) ;
#66604=DIRECTION('center_axis',(0.,-1.,0.)) ;
#66605=DIRECTION('ref_axis',(0.514495755427508,0.,-0.857492925712555)) ;
#66606=DIRECTION('',(0.424264068711912,-0.565685424949242,-0.707106781186554)) ;
#66607=DIRECTION('',(-0.424264068711912,0.565685424949242,0.707106781186554)) ;
#66608=DIRECTION('center_axis',(-0.640000000000003,-0.479999999999997,-0.599999999999999)) ;
#66609=DIRECTION('ref_axis',(-0.332851351149322,0.876990532021575,-0.346550984391311)) ;
#66610=DIRECTION('',(-0.640000000000003,-0.479999999999997,-0.599999999999999)) ;
#66611=DIRECTION('center_axis',(0.639999999999996,0.479999999999997,0.600000000000007)) ;
#66612=DIRECTION('ref_axis',(4.28317217346062E-16,0.780868809443036,-0.624695047554418)) ;
#66613=DIRECTION('',(0.640000000000003,0.479999999999997,0.599999999999999)) ;
#66614=DIRECTION('center_axis',(0.,0.624695047554418,0.780868809443036)) ;
#66615=DIRECTION('ref_axis',(0.,0.780868809443036,-0.624695047554418)) ;
#66616=DIRECTION('center_axis',(0.,0.529998940003177,-0.84799830400509)) ;
#66617=DIRECTION('ref_axis',(0.,0.84799830400509,0.529998940003177)) ;
#66618=DIRECTION('center_axis',(0.,-0.780868809443031,0.624695047554423)) ;
#66619=DIRECTION('ref_axis',(8.66938531455284E-17,0.624695047554423,0.780868809443031)) ;
#66620=DIRECTION('center_axis',(0.,-0.624695047554423,-0.780868809443031)) ;
#66621=DIRECTION('ref_axis',(-0.707106781186523,0.552157630374252,-0.441726104299401)) ;
#66622=DIRECTION('',(0.,0.624695047554423,0.780868809443031)) ;
#66623=DIRECTION('',(0.,-0.624695047554423,-0.780868809443031)) ;
#66624=DIRECTION('center_axis',(-1.,0.,0.)) ;
#66625=DIRECTION('ref_axis',(0.,1.,0.)) ;
#66626=DIRECTION('',(0.,0.,-1.)) ;
#66627=DIRECTION('',(0.,0.,-1.)) ;
#66628=DIRECTION('center_axis',(0.,0.,-1.)) ;
#66629=DIRECTION('ref_axis',(1.,0.,0.)) ;
#66630=DIRECTION('',(0.,0.,-1.)) ;
#66631=DIRECTION('center_axis',(1.,0.,0.)) ;
#66632=DIRECTION('ref_axis',(0.,-1.,0.)) ;
#66633=DIRECTION('',(0.,0.,-1.)) ;
#66634=DIRECTION('center_axis',(0.,0.,-1.)) ;
#66635=DIRECTION('ref_axis',(0.948683298050519,0.316227766016821,0.)) ;
#66636=DIRECTION('',(0.,0.,1.)) ;
#66637=DIRECTION('center_axis',(0.799999999999998,0.600000000000002,0.)) ;
#66638=DIRECTION('ref_axis',(0.,0.,-1.)) ;
#66639=DIRECTION('center_axis',(0.,0.780868809443031,-0.624695047554423)) ;
#66640=DIRECTION('ref_axis',(-1.,0.,0.)) ;
#66641=DIRECTION('center_axis',(0.,0.,-1.)) ;
#66642=DIRECTION('ref_axis',(1.,-7.1054273576004E-14,0.)) ;
#66643=DIRECTION('center_axis',(1.95689141014107E-45,1.96585022416868E-45,
-1.)) ;
#66644=DIRECTION('ref_axis',(1.,-7.1054273576004E-14,1.95689141014093E-45)) ;
#66645=DIRECTION('center_axis',(0.,0.,-1.)) ;
#66646=DIRECTION('ref_axis',(1.,0.,0.)) ;
#66647=DIRECTION('',(0.,0.,1.)) ;
#66648=DIRECTION('',(0.,0.,-1.)) ;
#66649=DIRECTION('center_axis',(0.,0.,-1.)) ;
#66650=DIRECTION('ref_axis',(1.,0.,0.)) ;
#66651=DIRECTION('',(0.,0.,-1.)) ;
#66652=DIRECTION('',(0.,0.,-1.)) ;
#66653=DIRECTION('center_axis',(-1.,3.17206578464333E-15,0.)) ;
#66654=DIRECTION('ref_axis',(3.17206578464333E-15,1.,-1.76085023486835E-33)) ;
#66655=DIRECTION('',(0.,0.,1.)) ;
#66656=DIRECTION('',(0.,0.,-1.)) ;
#66657=DIRECTION('',(-3.17206578464333E-15,-1.,6.60793205057061E-32)) ;
#66658=DIRECTION('center_axis',(0.,0.,-1.)) ;
#66659=DIRECTION('ref_axis',(0.,1.,0.)) ;
#66660=DIRECTION('center_axis',(-3.83260058933034E-30,-6.60793205056939E-32,
-1.)) ;
#66661=DIRECTION('ref_axis',(-2.53255642712671E-61,1.,-6.60793205056939E-32)) ;
#66662=DIRECTION('',(0.,0.,-1.)) ;
#66663=DIRECTION('center_axis',(0.,-1.,0.)) ;
#66664=DIRECTION('ref_axis',(-1.,0.,3.83260058933034E-30)) ;
#66665=DIRECTION('',(1.,0.,-3.83260058933034E-30)) ;
#66666=DIRECTION('',(0.,0.,-1.)) ;
#66667=DIRECTION('center_axis',(-1.,1.53134210293125E-15,0.)) ;
#66668=DIRECTION('ref_axis',(1.53134210293125E-15,1.,-6.60793205056998E-32)) ;
#66669=DIRECTION('',(-1.53134210293125E-15,-1.,6.60793205056998E-32)) ;
#66670=DIRECTION('',(0.,0.,-1.)) ;
#66671=DIRECTION('center_axis',(0.,0.,-1.)) ;
#66672=DIRECTION('ref_axis',(0.,1.,0.)) ;
#66673=DIRECTION('center_axis',(-3.83260058933034E-30,-6.60793205056939E-32,
-1.)) ;
#66674=DIRECTION('ref_axis',(-2.53255642712671E-61,1.,-6.60793205056939E-32)) ;
#66675=DIRECTION('',(0.,0.,-1.)) ;
#66676=DIRECTION('center_axis',(0.,-1.,0.)) ;
#66677=DIRECTION('ref_axis',(-1.,0.,-1.40067632319071E-31)) ;
#66678=DIRECTION('',(1.,0.,-3.83260058933034E-30)) ;
#66679=DIRECTION('',(0.,0.,-1.)) ;
#66680=DIRECTION('center_axis',(0.,0.,-1.)) ;
#66681=DIRECTION('ref_axis',(-1.,0.,0.)) ;
#66682=DIRECTION('center_axis',(-3.83260058933034E-30,-6.60793205056939E-32,
-1.)) ;
#66683=DIRECTION('ref_axis',(-1.,2.53255642712671E-61,3.83260058933034E-30)) ;
#66684=DIRECTION('',(0.,0.,-1.)) ;
#66685=DIRECTION('center_axis',(1.,0.,0.)) ;
#66686=DIRECTION('ref_axis',(0.,-1.,1.41044871512355E-33)) ;
#66687=DIRECTION('',(0.,1.,-6.60793205056939E-32)) ;
#66688=DIRECTION('',(0.,0.,-1.)) ;
#66689=DIRECTION('center_axis',(3.55271367880026E-13,-1.,0.)) ;
#66690=DIRECTION('ref_axis',(-1.,-3.55271367880026E-13,3.80009837042949E-30)) ;
#66691=DIRECTION('',(1.,3.55271367880026E-13,-3.83260058933036E-30)) ;
#66692=DIRECTION('',(0.,0.,-1.)) ;
#66693=DIRECTION('',(0.,0.,-1.)) ;
#66694=DIRECTION('center_axis',(0.,-1.,0.)) ;
#66695=DIRECTION('ref_axis',(-1.,0.,0.)) ;
#66696=DIRECTION('',(0.,0.,-1.)) ;
#66697=DIRECTION('',(-1.,0.,0.)) ;
#66698=DIRECTION('center_axis',(0.,0.,-1.)) ;
#66699=DIRECTION('ref_axis',(0.,1.,0.)) ;
#66700=DIRECTION('',(0.,0.,-1.)) ;
#66701=DIRECTION('center_axis',(6.125368411725E-15,-1.,0.)) ;
#66702=DIRECTION('ref_axis',(-1.,-6.125368411725E-15,1.93235546378459E-35)) ;
#66703=DIRECTION('',(0.,0.,-1.)) ;
#66704=DIRECTION('center_axis',(-6.125368411725E-15,1.,0.)) ;
#66705=DIRECTION('ref_axis',(-1.,-6.125368411725E-15,0.)) ;
#66706=DIRECTION('center_axis',(0.,0.,-1.)) ;
#66707=DIRECTION('ref_axis',(-1.,0.,0.)) ;
#66708=DIRECTION('center_axis',(0.,0.,-1.)) ;
#66709=DIRECTION('ref_axis',(1.,0.,0.)) ;
#66710=DIRECTION('',(0.,0.,-1.)) ;
#66711=DIRECTION('center_axis',(0.,0.,-1.)) ;
#66712=DIRECTION('ref_axis',(1.,0.,0.)) ;
#66713=DIRECTION('center_axis',(1.,-5.35505761538791E-15,0.)) ;
#66714=DIRECTION('ref_axis',(-5.35505761538791E-15,-1.,1.48632706569949E-33)) ;
#66715=DIRECTION('',(0.,0.,1.)) ;
#66716=DIRECTION('',(0.,0.,-1.)) ;
#66717=DIRECTION('',(5.35505761538791E-15,1.,0.)) ;
#66718=DIRECTION('center_axis',(0.,0.,-1.)) ;
#66719=DIRECTION('ref_axis',(-0.707106781186481,-0.707106781186614,0.)) ;
#66720=DIRECTION('center_axis',(0.,0.,-1.)) ;
#66721=DIRECTION('ref_axis',(-0.707106781186481,-0.707106781186614,0.)) ;
#66722=DIRECTION('',(0.,0.,-1.)) ;
#66723=DIRECTION('center_axis',(0.707106781186514,0.707106781186581,0.)) ;
#66724=DIRECTION('ref_axis',(0.707106781186581,-0.707106781186514,0.)) ;
#66725=DIRECTION('',(-0.707106781186581,0.707106781186514,0.)) ;
#66726=DIRECTION('',(0.,0.,-1.)) ;
#66727=DIRECTION('center_axis',(0.,0.,-1.)) ;
#66728=DIRECTION('ref_axis',(0.,-1.,0.)) ;
#66729=DIRECTION('center_axis',(0.,0.,-1.)) ;
#66730=DIRECTION('ref_axis',(0.,-1.,0.)) ;
#66731=DIRECTION('',(0.,0.,-1.)) ;
#66732=DIRECTION('center_axis',(1.75071816546432E-14,1.,0.)) ;
#66733=DIRECTION('ref_axis',(1.,-1.75071816546432E-14,-2.18941313571177E-49)) ;
#66734=DIRECTION('',(-1.,1.75071816546432E-14,0.)) ;
#66735=DIRECTION('',(0.,0.,-1.)) ;
#66736=DIRECTION('center_axis',(0.,0.,-1.)) ;
#66737=DIRECTION('ref_axis',(1.,0.,0.)) ;
#66738=DIRECTION('center_axis',(2.46519032881571E-32,4.87512283120816E-48,
-1.)) ;
#66739=DIRECTION('ref_axis',(1.,-1.2018105655283E-79,2.46519032881571E-32)) ;
#66740=DIRECTION('',(0.,0.,-1.)) ;
#66741=DIRECTION('',(0.,0.,-1.)) ;
#66742=DIRECTION('center_axis',(-1.,0.,0.)) ;
#66743=DIRECTION('ref_axis',(0.,1.,-1.76085023486835E-33)) ;
#66744=DIRECTION('',(0.,-1.,-4.87512283120816E-48)) ;
#66745=DIRECTION('',(0.,0.,-1.)) ;
#66746=DIRECTION('center_axis',(0.,0.,-1.)) ;
#66747=DIRECTION('ref_axis',(0.,1.,0.)) ;
#66748=DIRECTION('center_axis',(2.46519032881571E-32,4.87512283120816E-48,
-1.)) ;
#66749=DIRECTION('ref_axis',(-1.2018105655283E-79,1.,4.87512283120816E-48)) ;
#66750=DIRECTION('',(0.,0.,-1.)) ;
#66751=DIRECTION('center_axis',(-3.55271367880026E-13,-1.,0.)) ;
#66752=DIRECTION('ref_axis',(-1.,3.55271367880026E-13,9.05696233641872E-48)) ;
#66753=DIRECTION('',(1.,-3.55271367880026E-13,2.46519032881571E-32)) ;
#66754=DIRECTION('',(0.,0.,-1.)) ;
#66755=DIRECTION('center_axis',(-1.,1.53134210293125E-15,0.)) ;
#66756=DIRECTION('ref_axis',(1.53134210293125E-15,1.,0.)) ;
#66757=DIRECTION('',(-1.53134210293126E-15,-1.,-4.26256202537526E-47)) ;
#66758=DIRECTION('',(0.,0.,-1.)) ;
#66759=DIRECTION('center_axis',(0.,0.,-1.)) ;
#66760=DIRECTION('ref_axis',(0.,1.,0.)) ;
#66761=DIRECTION('center_axis',(2.46519032881571E-32,4.87512283120816E-48,
-1.)) ;
#66762=DIRECTION('ref_axis',(-1.2018105655283E-79,1.,4.87512283120816E-48)) ;
#66763=DIRECTION('',(0.,0.,-1.)) ;
#66764=DIRECTION('center_axis',(0.,-1.,0.)) ;
#66765=DIRECTION('ref_axis',(-1.,0.,1.62870009552296E-49)) ;
#66766=DIRECTION('',(1.,0.,2.46519032881571E-32)) ;
#66767=DIRECTION('',(0.,0.,-1.)) ;
#66768=DIRECTION('center_axis',(0.,0.,-1.)) ;
#66769=DIRECTION('ref_axis',(1.,0.,0.)) ;
#66770=DIRECTION('',(0.,0.,-1.)) ;
#66771=DIRECTION('center_axis',(0.,0.,-1.)) ;
#66772=DIRECTION('ref_axis',(1.,0.,0.)) ;
#66773=DIRECTION('center_axis',(-1.,0.,0.)) ;
#66774=DIRECTION('ref_axis',(0.,1.,-1.48632706569949E-33)) ;
#66775=DIRECTION('',(0.,-1.,0.)) ;
#66776=DIRECTION('',(0.,0.,-1.)) ;
#66777=DIRECTION('',(0.,0.,-1.)) ;
#66778=DIRECTION('center_axis',(0.,0.,-1.)) ;
#66779=DIRECTION('ref_axis',(0.707106781186636,0.707106781186459,0.)) ;
#66780=DIRECTION('center_axis',(0.,0.,-1.)) ;
#66781=DIRECTION('ref_axis',(0.707106781186636,0.707106781186459,0.)) ;
#66782=DIRECTION('',(0.,0.,-1.)) ;
#66783=DIRECTION('center_axis',(-0.707106781186539,-0.707106781186556,0.)) ;
#66784=DIRECTION('ref_axis',(-0.707106781186556,0.707106781186539,0.)) ;
#66785=DIRECTION('',(0.707106781186556,-0.707106781186539,0.)) ;
#66786=DIRECTION('',(0.,0.,-1.)) ;
#66787=DIRECTION('center_axis',(0.,0.,-1.)) ;
#66788=DIRECTION('ref_axis',(0.,1.,0.)) ;
#66789=DIRECTION('center_axis',(0.,0.,-1.)) ;
#66790=DIRECTION('ref_axis',(0.,1.,0.)) ;
#66791=DIRECTION('',(0.,0.,-1.)) ;
#66792=DIRECTION('center_axis',(-8.7535908273216E-15,-1.,0.)) ;
#66793=DIRECTION('ref_axis',(-1.,8.7535908273216E-15,2.56873619635494E-49)) ;
#66794=DIRECTION('',(1.,-8.7535908273216E-15,0.)) ;
#66795=DIRECTION('',(0.,0.,-1.)) ;
#66796=DIRECTION('',(0.,0.,-1.)) ;
#66797=DIRECTION('center_axis',(0.,0.,-1.)) ;
#66798=DIRECTION('ref_axis',(1.,0.,0.)) ;
#66799=DIRECTION('center_axis',(0.,0.,-1.)) ;
#66800=DIRECTION('ref_axis',(1.,0.,0.)) ;
#66801=DIRECTION('',(0.,0.,-1.)) ;
#66802=DIRECTION('',(0.,0.,-1.)) ;
#66803=DIRECTION('center_axis',(-1.,0.,0.)) ;
#66804=DIRECTION('ref_axis',(0.,1.,-1.76085023486835E-33)) ;
#66805=DIRECTION('',(0.,-1.,0.)) ;
#66806=DIRECTION('',(0.,0.,-1.)) ;
#66807=DIRECTION('center_axis',(0.,0.,-1.)) ;
#66808=DIRECTION('ref_axis',(0.,1.,0.)) ;
#66809=DIRECTION('center_axis',(0.,0.,-1.)) ;
#66810=DIRECTION('ref_axis',(0.,1.,0.)) ;
#66811=DIRECTION('',(0.,0.,-1.)) ;
#66812=DIRECTION('center_axis',(-3.55271367880026E-13,-1.,0.)) ;
#66813=DIRECTION('ref_axis',(-1.,3.55271367880026E-13,2.00046065889556E-47)) ;
#66814=DIRECTION('',(1.,-3.55271367880026E-13,0.)) ;
#66815=DIRECTION('',(0.,0.,-1.)) ;
#66816=DIRECTION('center_axis',(-1.,0.,0.)) ;
#66817=DIRECTION('ref_axis',(0.,1.,0.)) ;
#66818=DIRECTION('',(0.,-1.,0.)) ;
#66819=DIRECTION('center_axis',(0.,-1.,0.)) ;
#66820=DIRECTION('ref_axis',(-1.,0.,0.)) ;
#66821=DIRECTION('',(1.,0.,0.)) ;
#66822=DIRECTION('',(0.,0.,-1.)) ;
#66823=DIRECTION('center_axis',(0.,0.,-1.)) ;
#66824=DIRECTION('ref_axis',(0.,-1.,0.)) ;
#66825=DIRECTION('center_axis',(-3.18850138855159E-46,-1.74315279842113E-32,
-1.)) ;
#66826=DIRECTION('ref_axis',(5.55804511822336E-78,-1.,1.74315279842113E-32)) ;
#66827=DIRECTION('',(0.,0.,-1.)) ;
#66828=DIRECTION('',(0.,0.,-1.)) ;
#66829=DIRECTION('center_axis',(0.,1.,0.)) ;
#66830=DIRECTION('ref_axis',(1.,0.,6.12949496482233E-35)) ;
#66831=DIRECTION('',(-1.,0.,3.18850138855159E-46)) ;
#66832=DIRECTION('',(0.,0.,-1.)) ;
#66833=DIRECTION('',(0.,0.,-1.)) ;
#66834=DIRECTION('center_axis',(0.,0.,-1.)) ;
#66835=DIRECTION('ref_axis',(1.,0.,0.)) ;
#66836=DIRECTION('center_axis',(-3.18850138855159E-46,-1.74315279842113E-32,
-1.)) ;
#66837=DIRECTION('ref_axis',(1.,-5.55804511822336E-78,-3.18850138855159E-46)) ;
#66838=DIRECTION('',(0.,0.,-1.)) ;
#66839=DIRECTION('center_axis',(-1.,1.7763568394025E-14,0.)) ;
#66840=DIRECTION('ref_axis',(1.7763568394025E-14,1.,0.)) ;
#66841=DIRECTION('',(-1.7763568394025E-14,-1.,1.74315279842113E-32)) ;
#66842=DIRECTION('',(0.,0.,-1.)) ;
#66843=DIRECTION('center_axis',(0.,0.,-1.)) ;
#66844=DIRECTION('ref_axis',(0.,1.,0.)) ;
#66845=DIRECTION('center_axis',(-3.18850138855159E-46,-1.74315279842113E-32,
-1.)) ;
#66846=DIRECTION('ref_axis',(-5.55804511822336E-78,1.,-1.74315279842113E-32)) ;
#66847=DIRECTION('center_axis',(0.,0.,-1.)) ;
#66848=DIRECTION('ref_axis',(1.,0.,0.)) ;
#66849=DIRECTION('center_axis',(2.46519032881571E-32,4.87512283120816E-48,
-1.)) ;
#66850=DIRECTION('ref_axis',(1.,-1.2018105655283E-79,2.46519032881571E-32)) ;
#66851=DIRECTION('',(0.,0.,-1.)) ;
#66852=DIRECTION('',(0.,0.,-1.)) ;
#66853=DIRECTION('center_axis',(-1.,0.,0.)) ;
#66854=DIRECTION('ref_axis',(0.,1.,-1.76085023486835E-33)) ;
#66855=DIRECTION('',(0.,-1.,-4.87512283120816E-48)) ;
#66856=DIRECTION('',(0.,0.,-1.)) ;
#66857=DIRECTION('center_axis',(0.,0.,-1.)) ;
#66858=DIRECTION('ref_axis',(0.,1.,0.)) ;
#66859=DIRECTION('center_axis',(2.46519032881571E-32,4.87512283120816E-48,
-1.)) ;
#66860=DIRECTION('ref_axis',(-1.2018105655283E-79,1.,4.87512283120816E-48)) ;
#66861=DIRECTION('',(0.,0.,-1.)) ;
#66862=DIRECTION('center_axis',(-3.55271367880026E-13,-1.,0.)) ;
#66863=DIRECTION('ref_axis',(-1.,3.55271367880026E-13,9.05696233641872E-48)) ;
#66864=DIRECTION('',(1.,-3.55271367880026E-13,2.46519032881571E-32)) ;
#66865=DIRECTION('',(0.,0.,-1.)) ;
#66866=DIRECTION('center_axis',(-1.,1.53134210293125E-15,0.)) ;
#66867=DIRECTION('ref_axis',(1.53134210293125E-15,1.,0.)) ;
#66868=DIRECTION('',(-1.53134210293126E-15,-1.,-4.26256202537526E-47)) ;
#66869=DIRECTION('',(0.,0.,-1.)) ;
#66870=DIRECTION('center_axis',(0.,0.,-1.)) ;
#66871=DIRECTION('ref_axis',(0.,1.,0.)) ;
#66872=DIRECTION('center_axis',(2.46519032881571E-32,4.87512283120816E-48,
-1.)) ;
#66873=DIRECTION('ref_axis',(-1.2018105655283E-79,1.,4.87512283120816E-48)) ;
#66874=DIRECTION('',(0.,0.,-1.)) ;
#66875=DIRECTION('center_axis',(0.,-1.,0.)) ;
#66876=DIRECTION('ref_axis',(-1.,0.,1.62870009552296E-49)) ;
#66877=DIRECTION('',(1.,0.,2.46519032881571E-32)) ;
#66878=DIRECTION('',(0.,0.,-1.)) ;
#66879=DIRECTION('center_axis',(0.,0.,-1.)) ;
#66880=DIRECTION('ref_axis',(-1.,0.,0.)) ;
#66881=DIRECTION('center_axis',(2.46519032881571E-32,4.87512283120816E-48,
-1.)) ;
#66882=DIRECTION('ref_axis',(-1.,1.2018105655283E-79,-2.46519032881571E-32)) ;
#66883=DIRECTION('',(0.,0.,-1.)) ;
#66884=DIRECTION('center_axis',(1.,0.,0.)) ;
#66885=DIRECTION('ref_axis',(0.,-1.,8.50065630626093E-34)) ;
#66886=DIRECTION('',(0.,1.,4.87512283120816E-48)) ;
#66887=DIRECTION('',(0.,0.,-1.)) ;
#66888=DIRECTION('center_axis',(3.55271367880026E-13,-1.,0.)) ;
#66889=DIRECTION('ref_axis',(-1.,-3.55271367880026E-13,5.47382212626845E-48)) ;
#66890=DIRECTION('',(1.,3.55271367880026E-13,2.46519032881571E-32)) ;
#66891=DIRECTION('',(0.,0.,-1.)) ;
#66892=DIRECTION('center_axis',(0.,0.,-1.)) ;
#66893=DIRECTION('ref_axis',(-1.,0.,0.)) ;
#66894=DIRECTION('center_axis',(2.46519032881571E-32,4.87512283120816E-48,
-1.)) ;
#66895=DIRECTION('ref_axis',(-1.,1.2018105655283E-79,-2.46519032881571E-32)) ;
#66896=DIRECTION('',(0.,0.,-1.)) ;
#66897=DIRECTION('center_axis',(1.,0.,0.)) ;
#66898=DIRECTION('ref_axis',(0.,-1.,1.76085023486835E-33)) ;
#66899=DIRECTION('',(0.,1.,4.87512283120816E-48)) ;
#66900=DIRECTION('',(0.,0.,-1.)) ;
#66901=DIRECTION('center_axis',(0.,0.,-1.)) ;
#66902=DIRECTION('ref_axis',(0.,-1.,0.)) ;
#66903=DIRECTION('center_axis',(2.46519032881571E-32,4.87512283120816E-48,
-1.)) ;
#66904=DIRECTION('ref_axis',(1.2018105655283E-79,-1.,-4.87512283120816E-48)) ;
#66905=DIRECTION('',(0.,0.,-1.)) ;
#66906=DIRECTION('center_axis',(1.26882631385732E-14,1.,0.)) ;
#66907=DIRECTION('ref_axis',(1.,-1.26882631385732E-14,-1.27969293219661E-49)) ;
#66908=DIRECTION('',(-1.,1.26882631385732E-14,-2.46519032881571E-32)) ;
#66909=DIRECTION('center_axis',(2.46519032881571E-32,4.87512283120816E-48,
-1.)) ;
#66910=DIRECTION('ref_axis',(1.,3.7453410837561E-96,2.46519032881571E-32)) ;
#66911=DIRECTION('center_axis',(1.,0.,0.)) ;
#66912=DIRECTION('ref_axis',(0.,-1.,0.)) ;
#66913=DIRECTION('',(0.,1.,0.)) ;
#66914=DIRECTION('',(0.,0.,-1.)) ;
#66915=DIRECTION('',(0.,0.,-1.)) ;
#66916=DIRECTION('center_axis',(0.,1.,0.)) ;
#66917=DIRECTION('ref_axis',(1.,0.,0.)) ;
#66918=DIRECTION('',(-1.,0.,0.)) ;
#66919=DIRECTION('',(0.,0.,-1.)) ;
#66920=DIRECTION('center_axis',(0.,0.,-1.)) ;
#66921=DIRECTION('ref_axis',(0.707106781186459,-0.707106781186636,0.)) ;
#66922=DIRECTION('center_axis',(0.,0.,-1.)) ;
#66923=DIRECTION('ref_axis',(0.707106781186459,-0.707106781186636,0.)) ;
#66924=DIRECTION('',(0.,0.,-1.)) ;
#66925=DIRECTION('center_axis',(-0.707106781186573,0.707106781186522,0.)) ;
#66926=DIRECTION('ref_axis',(0.707106781186522,0.707106781186573,-4.31889331967372E-49)) ;
#66927=DIRECTION('',(-0.707106781186522,-0.707106781186573,0.)) ;
#66928=DIRECTION('',(0.,0.,-1.)) ;
#66929=DIRECTION('center_axis',(0.,0.,-1.)) ;
#66930=DIRECTION('ref_axis',(1.,0.,0.)) ;
#66931=DIRECTION('center_axis',(0.,0.,-1.)) ;
#66932=DIRECTION('ref_axis',(1.,0.,0.)) ;
#66933=DIRECTION('center_axis',(0.,0.,-1.)) ;
#66934=DIRECTION('ref_axis',(1.,0.,0.)) ;
#66935=DIRECTION('',(0.,0.,-1.)) ;
#66936=DIRECTION('center_axis',(1.,0.,0.)) ;
#66937=DIRECTION('ref_axis',(0.,-1.,0.)) ;
#66938=DIRECTION('',(0.,1.,0.)) ;
#66939=DIRECTION('',(0.,0.,-1.)) ;
#66940=DIRECTION('center_axis',(0.,-1.,0.)) ;
#66941=DIRECTION('ref_axis',(-1.,0.,0.)) ;
#66942=DIRECTION('',(1.,0.,0.)) ;
#66943=DIRECTION('',(0.,0.,-1.)) ;
#66944=DIRECTION('center_axis',(0.,0.,-1.)) ;
#66945=DIRECTION('ref_axis',(-1.,0.,0.)) ;
#66946=DIRECTION('center_axis',(0.,0.,-1.)) ;
#66947=DIRECTION('ref_axis',(-1.,0.,0.)) ;
#66948=DIRECTION('',(0.,0.,-1.)) ;
#66949=DIRECTION('center_axis',(1.,0.,0.)) ;
#66950=DIRECTION('ref_axis',(0.,-1.,1.76085023486835E-33)) ;
#66951=DIRECTION('',(0.,1.,0.)) ;
#66952=DIRECTION('',(0.,0.,-1.)) ;
#66953=DIRECTION('center_axis',(0.,0.,-1.)) ;
#66954=DIRECTION('ref_axis',(0.,-1.,0.)) ;
#66955=DIRECTION('center_axis',(0.,0.,-1.)) ;
#66956=DIRECTION('ref_axis',(0.,-1.,0.)) ;
#66957=DIRECTION('',(0.,0.,-1.)) ;
#66958=DIRECTION('center_axis',(0.,1.,0.)) ;
#66959=DIRECTION('ref_axis',(1.,0.,-4.0027363178395E-35)) ;
#66960=DIRECTION('',(-1.,0.,0.)) ;
#66961=DIRECTION('center_axis',(0.,0.,-1.)) ;
#66962=DIRECTION('ref_axis',(1.,0.,0.)) ;
#66963=DIRECTION('center_axis',(0.,0.,-1.)) ;
#66964=DIRECTION('ref_axis',(1.,0.,0.)) ;
#66965=DIRECTION('center_axis',(0.,0.,-1.)) ;
#66966=DIRECTION('ref_axis',(1.,0.,0.)) ;
#66967=DIRECTION('',(0.,0.,-1.)) ;
#66968=DIRECTION('center_axis',(-1.,0.,0.)) ;
#66969=DIRECTION('ref_axis',(0.,1.,0.)) ;
#66970=DIRECTION('',(0.,-1.,0.)) ;
#66971=DIRECTION('',(0.,0.,-1.)) ;
#66972=DIRECTION('center_axis',(0.,-1.,0.)) ;
#66973=DIRECTION('ref_axis',(-1.,0.,0.)) ;
#66974=DIRECTION('',(1.,0.,0.)) ;
#66975=DIRECTION('',(0.,0.,-1.)) ;
#66976=DIRECTION('center_axis',(-1.,-6.34413156929222E-15,0.)) ;
#66977=DIRECTION('ref_axis',(-6.34413156929222E-15,1.,0.)) ;
#66978=DIRECTION('',(6.34413156929222E-15,-1.,0.)) ;
#66979=DIRECTION('',(0.,0.,-1.)) ;
#66980=DIRECTION('center_axis',(0.,1.,0.)) ;
#66981=DIRECTION('ref_axis',(1.,0.,0.)) ;
#66982=DIRECTION('',(-1.,0.,0.)) ;
#66983=DIRECTION('',(0.,0.,-1.)) ;
#66984=DIRECTION('center_axis',(-1.,1.77635683940243E-14,0.)) ;
#66985=DIRECTION('ref_axis',(1.77635683940243E-14,1.,0.)) ;
#66986=DIRECTION('',(-1.77635683940243E-14,-1.,0.)) ;
#66987=DIRECTION('',(0.,0.,-1.)) ;
#66988=DIRECTION('center_axis',(0.,0.,-1.)) ;
#66989=DIRECTION('ref_axis',(0.,1.,0.)) ;
#66990=DIRECTION('center_axis',(0.,0.,-1.)) ;
#66991=DIRECTION('ref_axis',(0.,1.,0.)) ;
#66992=DIRECTION('',(0.,0.,-1.)) ;
#66993=DIRECTION('center_axis',(0.,0.,-1.)) ;
#66994=DIRECTION('ref_axis',(1.,0.,0.)) ;
#66995=DIRECTION('center_axis',(0.,0.,-1.)) ;
#66996=DIRECTION('ref_axis',(1.,0.,0.)) ;
#66997=DIRECTION('',(1.,0.,0.)) ;
#66998=DIRECTION('center_axis',(0.,0.,-1.)) ;
#66999=DIRECTION('ref_axis',(-1.,0.,0.)) ;
#67000=DIRECTION('center_axis',(2.46519032881571E-32,4.87512283120816E-48,
-1.)) ;
#67001=DIRECTION('ref_axis',(-1.,1.2018105655283E-79,-2.46519032881571E-32)) ;
#67002=DIRECTION('',(0.,0.,-1.)) ;
#67003=DIRECTION('center_axis',(1.,0.,0.)) ;
#67004=DIRECTION('ref_axis',(0.,-1.,8.50065630626093E-34)) ;
#67005=DIRECTION('',(0.,1.,4.87512283120816E-48)) ;
#67006=DIRECTION('',(0.,0.,-1.)) ;
#67007=DIRECTION('center_axis',(3.55271367880026E-13,-1.,0.)) ;
#67008=DIRECTION('ref_axis',(-1.,-3.55271367880026E-13,5.47382212626845E-48)) ;
#67009=DIRECTION('',(1.,3.55271367880026E-13,2.46519032881571E-32)) ;
#67010=DIRECTION('',(0.,0.,-1.)) ;
#67011=DIRECTION('center_axis',(0.,0.,-1.)) ;
#67012=DIRECTION('ref_axis',(-1.,0.,0.)) ;
#67013=DIRECTION('center_axis',(2.46519032881571E-32,4.87512283120816E-48,
-1.)) ;
#67014=DIRECTION('ref_axis',(-1.,1.2018105655283E-79,-2.46519032881571E-32)) ;
#67015=DIRECTION('',(0.,0.,-1.)) ;
#67016=DIRECTION('center_axis',(1.,0.,0.)) ;
#67017=DIRECTION('ref_axis',(0.,-1.,1.76085023486835E-33)) ;
#67018=DIRECTION('',(0.,1.,4.87512283120816E-48)) ;
#67019=DIRECTION('',(0.,0.,-1.)) ;
#67020=DIRECTION('center_axis',(0.,0.,-1.)) ;
#67021=DIRECTION('ref_axis',(0.,-1.,0.)) ;
#67022=DIRECTION('center_axis',(2.46519032881571E-32,4.87512283120816E-48,
-1.)) ;
#67023=DIRECTION('ref_axis',(1.2018105655283E-79,-1.,-4.87512283120816E-48)) ;
#67024=DIRECTION('',(0.,0.,-1.)) ;
#67025=DIRECTION('center_axis',(1.26882631385732E-14,1.,0.)) ;
#67026=DIRECTION('ref_axis',(1.,-1.26882631385732E-14,-1.27969293219661E-49)) ;
#67027=DIRECTION('',(-1.,1.26882631385732E-14,-2.46519032881571E-32)) ;
#67028=DIRECTION('center_axis',(2.46519032881571E-32,4.87512283120816E-48,
-1.)) ;
#67029=DIRECTION('ref_axis',(1.,3.7453410837561E-96,2.46519032881571E-32)) ;
#67030=DIRECTION('center_axis',(0.,0.,-1.)) ;
#67031=DIRECTION('ref_axis',(-0.707106781186636,0.707106781186459,0.)) ;
#67032=DIRECTION('center_axis',(-3.18850138855159E-46,-1.74315279842113E-32,
-1.)) ;
#67033=DIRECTION('ref_axis',(-0.707106781186636,0.707106781186459,-1.23259516440771E-32)) ;
#67034=DIRECTION('',(0.,0.,-1.)) ;
#67035=DIRECTION('center_axis',(0.707106781186556,-0.707106781186539,0.)) ;
#67036=DIRECTION('ref_axis',(-0.707106781186539,-0.707106781186556,1.17554800907501E-33)) ;
#67037=DIRECTION('',(0.707106781186539,0.707106781186556,-1.23259516440793E-32)) ;
#67038=DIRECTION('',(0.,0.,-1.)) ;
#67039=DIRECTION('center_axis',(0.,0.,-1.)) ;
#67040=DIRECTION('ref_axis',(-1.,0.,0.)) ;
#67041=DIRECTION('center_axis',(-3.18850138855159E-46,-1.74315279842113E-32,
-1.)) ;
#67042=DIRECTION('ref_axis',(-1.,5.55804511822336E-78,3.18850138855159E-46)) ;
#67043=DIRECTION('',(0.,0.,-1.)) ;
#67044=DIRECTION('center_axis',(1.,-5.35505761538786E-15,0.)) ;
#67045=DIRECTION('ref_axis',(-5.35505761538786E-15,-1.,7.43163532849736E-34)) ;
#67046=DIRECTION('',(5.35505761538786E-15,1.,-1.74315279842113E-32)) ;
#67047=DIRECTION('',(0.,0.,-1.)) ;
#67048=DIRECTION('center_axis',(0.,0.,-1.)) ;
#67049=DIRECTION('ref_axis',(-0.707106781186681,-0.707106781186414,0.)) ;
#67050=DIRECTION('center_axis',(-3.18850138855159E-46,-1.74315279842113E-32,
-1.)) ;
#67051=DIRECTION('ref_axis',(-0.707106781186681,-0.707106781186414,1.23259516440768E-32)) ;
#67052=DIRECTION('',(0.,0.,-1.)) ;
#67053=DIRECTION('center_axis',(0.707106781186509,0.707106781186586,0.)) ;
#67054=DIRECTION('ref_axis',(0.707106781186586,-0.707106781186509,-7.3914897815741E-47)) ;
#67055=DIRECTION('',(-0.707106781186586,0.707106781186509,-1.2325951644078E-32)) ;
#67056=DIRECTION('center_axis',(-3.18850138855159E-46,-1.74315279842113E-32,
-1.)) ;
#67057=DIRECTION('ref_axis',(1.,5.16381567742834E-95,-3.18850138855159E-46)) ;
#67058=DIRECTION('center_axis',(0.,0.,-1.)) ;
#67059=DIRECTION('ref_axis',(1.,0.,0.)) ;
#67060=DIRECTION('center_axis',(0.,0.,-1.)) ;
#67061=DIRECTION('ref_axis',(-1.,0.,0.)) ;
#67062=DIRECTION('center_axis',(-3.83260058933034E-30,-6.60793205056939E-32,
-1.)) ;
#67063=DIRECTION('ref_axis',(-1.,2.53255642712671E-61,3.83260058933034E-30)) ;
#67064=DIRECTION('',(0.,0.,-1.)) ;
#67065=DIRECTION('center_axis',(1.,-3.17206578464333E-15,0.)) ;
#67066=DIRECTION('ref_axis',(-3.17206578464333E-15,-1.,1.76085023486835E-33)) ;
#67067=DIRECTION('',(3.17206578464333E-15,1.,-6.60793205057061E-32)) ;
#67068=DIRECTION('',(0.,0.,-1.)) ;
#67069=DIRECTION('center_axis',(0.,0.,-1.)) ;
#67070=DIRECTION('ref_axis',(1.,0.,0.)) ;
#67071=DIRECTION('center_axis',(-0.599999999999998,0.800000000000002,0.)) ;
#67072=DIRECTION('ref_axis',(0.,0.,1.)) ;
#67073=DIRECTION('',(0.,0.,-1.)) ;
#67074=DIRECTION('',(0.,0.,-1.)) ;
#67075=DIRECTION('center_axis',(0.,1.,0.)) ;
#67076=DIRECTION('ref_axis',(1.,0.,3.20175569450239E-16)) ;
#67077=DIRECTION('',(0.,0.,1.)) ;
#67078=DIRECTION('',(1.,0.,0.)) ;
#67079=DIRECTION('center_axis',(0.800000000000014,0.599999999999982,0.)) ;
#67080=DIRECTION('ref_axis',(0.,0.,-1.)) ;
#67081=DIRECTION('',(0.,0.,1.)) ;
#67082=DIRECTION('center_axis',(-1.,0.,0.)) ;
#67083=DIRECTION('ref_axis',(0.,1.,0.)) ;
#67084=DIRECTION('',(0.,0.,-1.)) ;
#67085=DIRECTION('',(0.,0.,1.)) ;
#67086=DIRECTION('center_axis',(-1.,1.08152878803189E-14,0.)) ;
#67087=DIRECTION('ref_axis',(1.08152878803189E-14,1.,-2.09196947838501E-32)) ;
#67088=DIRECTION('center_axis',(0.,1.,0.)) ;
#67089=DIRECTION('ref_axis',(1.,0.,-2.99489585516063E-33)) ;
#67090=DIRECTION('',(0.,0.,-1.)) ;
#67091=DIRECTION('center_axis',(-0.766044443118928,-0.642787609686599,0.)) ;
#67092=DIRECTION('ref_axis',(-0.642787609686599,0.766044443118928,1.23259516440792E-32)) ;
#67093=DIRECTION('',(0.,0.,-1.)) ;
#67094=DIRECTION('center_axis',(0.,0.,-1.)) ;
#67095=DIRECTION('ref_axis',(1.42108547151988E-13,1.,0.)) ;
#67096=DIRECTION('',(0.,0.,-1.)) ;
#67097=DIRECTION('center_axis',(-1.28403006865249E-14,-1.,0.)) ;
#67098=DIRECTION('ref_axis',(-1.,1.28403006865249E-14,0.)) ;
#67099=DIRECTION('',(0.,0.,-1.)) ;
#67100=DIRECTION('center_axis',(0.,0.,-1.)) ;
#67101=DIRECTION('ref_axis',(1.,0.,0.)) ;
#67102=DIRECTION('',(0.,0.,-1.)) ;
#67103=DIRECTION('center_axis',(-1.,0.,0.)) ;
#67104=DIRECTION('ref_axis',(0.,1.,-2.39087358882206E-65)) ;
#67105=DIRECTION('center_axis',(-3.83260058933034E-30,-6.60793205056939E-32,
-1.)) ;
#67106=DIRECTION('ref_axis',(1.,1.51420860759427E-77,-3.83260058933034E-30)) ;
#67107=DIRECTION('center_axis',(-3.83260058933034E-30,-6.60793205056939E-32,
-1.)) ;
#67108=DIRECTION('ref_axis',(-1.,3.9474596431117E-14,3.83260058933034E-30)) ;
#67109=DIRECTION('center_axis',(-3.83260058933034E-30,-6.60793205056939E-32,
-1.)) ;
#67110=DIRECTION('ref_axis',(2.53255642712671E-61,-1.,6.60793205056939E-32)) ;
#67111=DIRECTION('center_axis',(0.,0.,-1.)) ;
#67112=DIRECTION('ref_axis',(0.,-1.,0.)) ;
#67113=DIRECTION('',(0.,0.,-1.)) ;
#67114=DIRECTION('center_axis',(-1.,0.,0.)) ;
#67115=DIRECTION('ref_axis',(0.,1.,0.)) ;
#67116=DIRECTION('center_axis',(0.,0.,-1.)) ;
#67117=DIRECTION('ref_axis',(-1.,3.9474596431117E-14,0.)) ;
#67118=DIRECTION('',(0.,0.,-1.)) ;
#67119=DIRECTION('center_axis',(3.55271367880048E-14,1.,0.)) ;
#67120=DIRECTION('ref_axis',(1.,-3.55271367880048E-14,0.)) ;
#67121=DIRECTION('',(0.,0.,-1.)) ;
#67122=DIRECTION('center_axis',(-1.,0.,0.)) ;
#67123=DIRECTION('ref_axis',(0.,1.,0.)) ;
#67124=DIRECTION('center_axis',(0.,-1.,0.)) ;
#67125=DIRECTION('ref_axis',(-1.,0.,-2.52374105052742E-18)) ;
#67126=DIRECTION('',(0.,0.,1.)) ;
#67127=DIRECTION('center_axis',(-1.,3.67742382159233E-14,0.)) ;
#67128=DIRECTION('ref_axis',(3.67742382159233E-14,1.,0.)) ;
#67129=DIRECTION('center_axis',(1.,-2.61228946970624E-14,0.)) ;
#67130=DIRECTION('ref_axis',(-2.61228946970624E-14,-1.,0.)) ;
#67131=DIRECTION('',(0.,0.,-1.)) ;
#67132=DIRECTION('center_axis',(0.,0.,-1.)) ;
#67133=DIRECTION('ref_axis',(0.948683298050522,0.316227766016813,0.)) ;
#67134=DIRECTION('center_axis',(-0.599999999999996,0.800000000000003,0.)) ;
#67135=DIRECTION('ref_axis',(0.,0.,1.)) ;
#67136=DIRECTION('',(0.,0.,-1.)) ;
#67137=DIRECTION('center_axis',(0.,0.,1.)) ;
#67138=DIRECTION('ref_axis',(-0.894427190999906,0.447213595499978,0.)) ;
#67139=DIRECTION('center_axis',(0.,0.780868809443031,-0.624695047554424)) ;
#67140=DIRECTION('ref_axis',(-1.,0.,0.)) ;
#67141=DIRECTION('center_axis',(-1.,0.,0.)) ;
#67142=DIRECTION('ref_axis',(0.,1.,0.)) ;
#67143=DIRECTION('',(0.,0.,1.)) ;
#67144=DIRECTION('center_axis',(0.,0.,1.)) ;
#67145=DIRECTION('ref_axis',(-0.89442719099992,0.44721359549995,0.)) ;
#67146=DIRECTION('center_axis',(0.,-1.,0.)) ;
#67147=DIRECTION('ref_axis',(-1.,0.,0.)) ;
#67148=DIRECTION('',(0.,-1.,0.)) ;
#67149=DIRECTION('center_axis',(0.,-1.,0.)) ;
#67150=DIRECTION('ref_axis',(-1.,0.,2.76147456380442E-35)) ;
#67151=DIRECTION('',(0.,0.,-1.)) ;
#67152=DIRECTION('center_axis',(0.,0.,-1.)) ;
#67153=DIRECTION('ref_axis',(1.,0.,0.)) ;
#67154=DIRECTION('',(0.,0.,1.)) ;
#67155=DIRECTION('center_axis',(-1.,0.,0.)) ;
#67156=DIRECTION('ref_axis',(0.,1.,0.)) ;
#67157=DIRECTION('',(0.,0.,-1.)) ;
#67158=DIRECTION('center_axis',(0.,0.,-1.)) ;
#67159=DIRECTION('ref_axis',(1.,0.,0.)) ;
#67160=DIRECTION('',(0.,0.,-1.)) ;
#67161=DIRECTION('center_axis',(1.,0.,0.)) ;
#67162=DIRECTION('ref_axis',(0.,-1.,0.)) ;
#67163=DIRECTION('center_axis',(1.,0.,0.)) ;
#67164=DIRECTION('ref_axis',(0.,-1.,0.)) ;
#67165=DIRECTION('',(0.,0.,-1.)) ;
#67166=DIRECTION('center_axis',(0.,0.,-1.)) ;
#67167=DIRECTION('ref_axis',(1.,0.,0.)) ;
#67168=DIRECTION('center_axis',(0.,0.,1.)) ;
#67169=DIRECTION('ref_axis',(1.,0.,0.)) ;
#67170=DIRECTION('',(1.,0.,0.)) ;
#67171=DIRECTION('',(0.,1.,0.)) ;
#67172=DIRECTION('center_axis',(1.,0.,0.)) ;
#67173=DIRECTION('ref_axis',(0.,1.,0.)) ;
#67174=DIRECTION('center_axis',(0.,1.,0.)) ;
#67175=DIRECTION('ref_axis',(-1.,0.,0.)) ;
#67176=DIRECTION('center_axis',(0.,0.,-1.)) ;
#67177=DIRECTION('ref_axis',(1.,0.,0.)) ;
#67178=DIRECTION('center_axis',(0.,-1.,0.)) ;
#67179=DIRECTION('ref_axis',(1.,0.,0.)) ;
#88999=CARTESIAN_POINT('',(0.,0.,0.)) ;
#89000=CARTESIAN_POINT('Ctrl Pts',(55.5095145719656,261.79455482774,20.2277364888237)) ;
#89001=CARTESIAN_POINT('Ctrl Pts',(55.5235850209285,261.795524155342,20.2176307773862)) ;
#89002=CARTESIAN_POINT('Ctrl Pts',(55.5532287114159,261.797064527402,20.1984257565318)) ;
#89003=CARTESIAN_POINT('Ctrl Pts',(55.6031763483208,261.798222507439,20.1723029608032)) ;
#89004=CARTESIAN_POINT('Ctrl Pts',(55.6599047282381,261.79814256388,20.1486416834275)) ;
#89005=CARTESIAN_POINT('Ctrl Pts',(55.7252078119995,261.796555096217,20.1272203634637)) ;
#89006=CARTESIAN_POINT('Ctrl Pts',(55.8010086453308,261.793278462298,20.1080994112902)) ;
#89007=CARTESIAN_POINT('Ctrl Pts',(55.8886521902875,261.788562905801,20.0918367827122)) ;
#89008=CARTESIAN_POINT('Ctrl Pts',(55.9864294144668,261.783244910011,20.0795560745166)) ;
#89009=CARTESIAN_POINT('Ctrl Pts',(56.0870864420511,261.778692438248,20.0723692404909)) ;
#89010=CARTESIAN_POINT('Ctrl Pts',(56.1809390611363,261.776355954665,20.0702679342639)) ;
#89011=CARTESIAN_POINT('Ctrl Pts',(56.2391336395509,261.776281941501,20.0706687254062)) ;
#89012=CARTESIAN_POINT('Ctrl Pts',(56.2695111541429,261.776281941501,20.0706687254062)) ;
#89013=CARTESIAN_POINT('Ctrl Pts',(55.5318704226011,261.835587804427,20.2336372451564)) ;
#89014=CARTESIAN_POINT('Ctrl Pts',(55.5459583366965,261.834973203121,20.2238071455774)) ;
#89015=CARTESIAN_POINT('Ctrl Pts',(55.5756021232183,261.833526932472,20.2050383428634)) ;
#89016=CARTESIAN_POINT('Ctrl Pts',(55.6253962312584,261.83064540612,20.1793520028903)) ;
#89017=CARTESIAN_POINT('Ctrl Pts',(55.6817877740942,261.826937340059,20.1560071692871)) ;
#89018=CARTESIAN_POINT('Ctrl Pts',(55.7465198445918,261.822171831918,20.1348521511824)) ;
#89019=CARTESIAN_POINT('Ctrl Pts',(55.8213429131526,261.816334347102,20.116044324121)) ;
#89020=CARTESIAN_POINT('Ctrl Pts',(55.9069737675768,261.809885023379,20.1002538676655)) ;
#89021=CARTESIAN_POINT('Ctrl Pts',(56.0006863128197,261.803760509541,20.0886458821796)) ;
#89022=CARTESIAN_POINT('Ctrl Pts',(56.0954683537023,261.799281373801,20.0821480955844)) ;
#89023=CARTESIAN_POINT('Ctrl Pts',(56.1840401677701,261.79765282798,20.0805472862567)) ;
#89024=CARTESIAN_POINT('Ctrl Pts',(56.2401954718791,261.798341867179,20.0812712738205)) ;
#89025=CARTESIAN_POINT('Ctrl Pts',(56.2695111541429,261.798715764224,20.0814509780309)) ;
#89026=CARTESIAN_POINT('Ctrl Pts',(55.5809822967928,261.905784092892,20.2463148514966)) ;
#89027=CARTESIAN_POINT('Ctrl Pts',(55.595241405465,261.902637928269,20.236906103947)) ;
#89028=CARTESIAN_POINT('Ctrl Pts',(55.6251695278679,261.896295106137,20.2188443093641)) ;
#89029=CARTESIAN_POINT('Ctrl Pts',(55.6752360499304,261.886680755071,20.1939945267448)) ;
#89030=CARTESIAN_POINT('Ctrl Pts',(55.7317648353249,261.877030049387,20.1714245134235)) ;
#89031=CARTESIAN_POINT('Ctrl Pts',(55.7963490542379,261.867339871692,20.151107208204)) ;
#89032=CARTESIAN_POINT('Ctrl Pts',(55.869636711629,261.857869603308,20.1333948641784)) ;
#89033=CARTESIAN_POINT('Ctrl Pts',(55.9501532362832,261.849298162689,20.1191525070167)) ;
#89034=CARTESIAN_POINT('Ctrl Pts',(56.0337736489394,261.842781264602,20.1094881093263)) ;
#89035=CARTESIAN_POINT('Ctrl Pts',(56.1152086370634,261.839299967236,20.1047811880335)) ;
#89036=CARTESIAN_POINT('Ctrl Pts',(56.1919043895799,261.839370541405,20.1044512199224)) ;
#89037=CARTESIAN_POINT('Ctrl Pts',(56.2427773792535,261.841154112132,20.1058420373569)) ;
#89038=CARTESIAN_POINT('Ctrl Pts',(56.2695111541429,261.841969944151,20.1063719286696)) ;
#89039=CARTESIAN_POINT('Ctrl Pts',(55.7142947487837,261.996615667805,20.2848817332965)) ;
#89040=CARTESIAN_POINT('Ctrl Pts',(55.727431023685,261.989690475884,20.2750630800784)) ;
#89041=CARTESIAN_POINT('Ctrl Pts',(55.7551316099311,261.976322682396,20.256254734585)) ;
#89042=CARTESIAN_POINT('Ctrl Pts',(55.801119679589,261.957993605918,20.2308429035396)) ;
#89043=CARTESIAN_POINT('Ctrl Pts',(55.8516376794038,261.941560611499,20.208427342522)) ;
#89044=CARTESIAN_POINT('Ctrl Pts',(55.9066495299668,261.92699687125,20.1889543815959)) ;
#89045=CARTESIAN_POINT('Ctrl Pts',(55.9650620575114,261.914742356923,20.1729029806023)) ;
#89046=CARTESIAN_POINT('Ctrl Pts',(56.0249859995935,261.905548305835,20.1610377158358)) ;
#89047=CARTESIAN_POINT('Ctrl Pts',(56.0846095008272,261.899969669763,20.1538028301126)) ;
#89048=CARTESIAN_POINT('Ctrl Pts',(56.1437294140665,261.897823268871,20.1507219087426)) ;
#89049=CARTESIAN_POINT('Ctrl Pts',(56.2045341748838,261.898451408471,20.1509202634277)) ;
#89050=CARTESIAN_POINT('Ctrl Pts',(56.2477208775326,261.899867602781,20.1523151226862)) ;
#89051=CARTESIAN_POINT('Ctrl Pts',(56.2695111541429,261.900567313948,20.1529909710202)) ;
#89052=CARTESIAN_POINT('Ctrl Pts',(55.8167520150608,262.046133815589,20.3289876130455)) ;
#89053=CARTESIAN_POINT('Ctrl Pts',(55.8272233753503,262.037515709941,20.3182149809853)) ;
#89054=CARTESIAN_POINT('Ctrl Pts',(55.8493213988809,262.02109949769,20.2976947156725)) ;
#89055=CARTESIAN_POINT('Ctrl Pts',(55.885680659634,261.999411922698,20.2705852469321)) ;
#89056=CARTESIAN_POINT('Ctrl Pts',(55.9253732866277,261.980738298363,20.2472432165129)) ;
#89057=CARTESIAN_POINT('Ctrl Pts',(55.9686042187112,261.964920001218,20.2274703450816)) ;
#89058=CARTESIAN_POINT('Ctrl Pts',(56.0147532633608,261.952242450621,20.2116234068352)) ;
#89059=CARTESIAN_POINT('Ctrl Pts',(56.062891123676,261.943048307455,20.2001307278784)) ;
#89060=CARTESIAN_POINT('Ctrl Pts',(56.1123369473664,261.937285799675,20.1929275931536)) ;
#89061=CARTESIAN_POINT('Ctrl Pts',(56.1631175051399,261.934403034741,20.1893241369859)) ;
#89062=CARTESIAN_POINT('Ctrl Pts',(56.2154844879084,261.933798091816,20.1885679583302)) ;
#89063=CARTESIAN_POINT('Ctrl Pts',(56.2514427323094,261.934313905503,20.1892127254389)) ;
#89064=CARTESIAN_POINT('Ctrl Pts',(56.2695111541429,261.934573054282,20.1895366614117)) ;
#89065=CARTESIAN_POINT('Ctrl Pts',(55.8638558727399,262.066371572297,20.3542848089307)) ;
#89066=CARTESIAN_POINT('Ctrl Pts',(55.872989551448,262.057390488197,20.343058453806)) ;
#89067=CARTESIAN_POINT('Ctrl Pts',(55.8924334380602,262.040313031316,20.321711632704)) ;
#89068=CARTESIAN_POINT('Ctrl Pts',(55.9246856684865,262.017918820106,20.2937188686917)) ;
#89069=CARTESIAN_POINT('Ctrl Pts',(55.960120463602,261.998755165223,20.2697643000883)) ;
#89070=CARTESIAN_POINT('Ctrl Pts',(55.9988335935537,261.982652502899,20.2496359721834)) ;
#89071=CARTESIAN_POINT('Ctrl Pts',(56.0401450285716,261.969868594253,20.2336560863755)) ;
#89072=CARTESIAN_POINT('Ctrl Pts',(56.0832318051021,261.960620595462,20.222096087887)) ;
#89073=CARTESIAN_POINT('Ctrl Pts',(56.1276386228793,261.954662126184,20.2146480012896)) ;
#89074=CARTESIAN_POINT('Ctrl Pts',(56.1734770209332,261.951373074562,20.2105366867623)) ;
#89075=CARTESIAN_POINT('Ctrl Pts',(56.2208605753121,261.950134902533,20.2089889717264)) ;
#89076=CARTESIAN_POINT('Ctrl Pts',(56.2532834268155,261.950121980978,20.2089728197824)) ;
#89077=CARTESIAN_POINT('Ctrl Pts',(56.2695111541429,261.950121980978,20.2089728197824)) ;
#89078=CARTESIAN_POINT('',(55.5095145719656,261.79455482774,20.2277364888237)) ;
#89079=CARTESIAN_POINT('',(56.2695111541429,261.776281941501,20.0706687254062)) ;
#89080=CARTESIAN_POINT('Ctrl Pts',(55.5095145719656,261.79455482774,20.2277364888237)) ;
#89081=CARTESIAN_POINT('Ctrl Pts',(55.5235850209285,261.795524155342,20.2176307773862)) ;
#89082=CARTESIAN_POINT('Ctrl Pts',(55.5532287114159,261.797064527402,20.1984257565318)) ;
#89083=CARTESIAN_POINT('Ctrl Pts',(55.6031763483208,261.79822250744,20.1723029608032)) ;
#89084=CARTESIAN_POINT('Ctrl Pts',(55.6599047282381,261.79814256388,20.1486416834275)) ;
#89085=CARTESIAN_POINT('Ctrl Pts',(55.7252078119995,261.796555096218,20.1272203634636)) ;
#89086=CARTESIAN_POINT('Ctrl Pts',(55.8010086453309,261.793278462297,20.1080994112902)) ;
#89087=CARTESIAN_POINT('Ctrl Pts',(55.8886521902874,261.788562905802,20.0918367827122)) ;
#89088=CARTESIAN_POINT('Ctrl Pts',(55.9864294144668,261.78324491001,20.0795560745165)) ;
#89089=CARTESIAN_POINT('Ctrl Pts',(56.0870864420511,261.778692438249,20.0723692404909)) ;
#89090=CARTESIAN_POINT('Ctrl Pts',(56.1809390611364,261.776355954664,20.0702679342639)) ;
#89091=CARTESIAN_POINT('Ctrl Pts',(56.2391336395509,261.776281941501,20.0706687254062)) ;
#89092=CARTESIAN_POINT('Ctrl Pts',(56.2695111541429,261.776281941501,20.0706687254062)) ;
#89093=CARTESIAN_POINT('',(55.8638558727399,262.066371572297,20.3542848089307)) ;
#89094=CARTESIAN_POINT('Ctrl Pts',(55.5095145719656,261.79455482774,20.2277364888237)) ;
#89095=CARTESIAN_POINT('Ctrl Pts',(55.5318704226011,261.835587804427,20.2336372451564)) ;
#89096=CARTESIAN_POINT('Ctrl Pts',(55.5809822967928,261.905784092892,20.2463148514966)) ;
#89097=CARTESIAN_POINT('Ctrl Pts',(55.7142947487837,261.996615667805,20.2848817332965)) ;
#89098=CARTESIAN_POINT('Ctrl Pts',(55.8167520150608,262.046133815589,20.3289876130455)) ;
#89099=CARTESIAN_POINT('Ctrl Pts',(55.8638558727399,262.066371572297,20.3542848089307)) ;
#89100=CARTESIAN_POINT('',(56.2695111541429,261.950121980978,20.2089728197824)) ;
#89101=CARTESIAN_POINT('Ctrl Pts',(55.8638558727399,262.066371572297,20.3542848089307)) ;
#89102=CARTESIAN_POINT('Ctrl Pts',(55.8713330463535,262.05901931838,20.345094491535)) ;
#89103=CARTESIAN_POINT('Ctrl Pts',(55.8792039017644,262.051963652932,20.336274909725)) ;
#89104=CARTESIAN_POINT('Ctrl Pts',(55.8874289902313,262.045256409105,20.3278908549412)) ;
#89105=CARTESIAN_POINT('Ctrl Pts',(55.8892510844872,262.043770561203,20.3260335450625)) ;
#89106=CARTESIAN_POINT('Ctrl Pts',(55.8910908387747,262.04230150103,20.3241972198463)) ;
#89107=CARTESIAN_POINT('Ctrl Pts',(55.8929476782012,262.040849955509,20.3223827879453)) ;
#89108=CARTESIAN_POINT('Ctrl Pts',(55.8986519339602,262.036390772459,20.3168088091333)) ;
#89109=CARTESIAN_POINT('Ctrl Pts',(55.9045175213531,262.0320969714,20.3114415578101)) ;
#89110=CARTESIAN_POINT('Ctrl Pts',(55.9105424868196,262.027972712684,20.3062862344144)) ;
#89111=CARTESIAN_POINT('Ctrl Pts',(55.9153320522155,262.024694120144,20.3021879937394)) ;
#89112=CARTESIAN_POINT('Ctrl Pts',(55.920221933305,262.021522772665,20.2982238093905)) ;
#89113=CARTESIAN_POINT('Ctrl Pts',(55.9252155779456,262.018456999749,20.2943915932464)) ;
#89114=CARTESIAN_POINT('Ctrl Pts',(55.9321214893699,262.014217219444,20.2890918678644)) ;
#89115=CARTESIAN_POINT('Ctrl Pts',(55.9392257846889,262.010179296389,20.2840444640455)) ;
#89116=CARTESIAN_POINT('Ctrl Pts',(55.9465389364433,262.006333296846,20.2792369646175)) ;
#89117=CARTESIAN_POINT('Ctrl Pts',(55.9511666186691,262.003899590515,20.2761948317038)) ;
#89118=CARTESIAN_POINT('Ctrl Pts',(55.9558757446086,262.001543949715,20.2732502807027)) ;
#89119=CARTESIAN_POINT('Ctrl Pts',(55.9606665897011,261.99926519383,20.2704018358466)) ;
#89120=CARTESIAN_POINT('Ctrl Pts',(55.9656406070482,261.996899312428,20.2674444840949)) ;
#89121=CARTESIAN_POINT('Ctrl Pts',(55.9707027113969,261.994616308741,20.2645907294863)) ;
#89122=CARTESIAN_POINT('Ctrl Pts',(55.9758446315117,261.992419381877,20.2618445709062)) ;
#89123=CARTESIAN_POINT('Ctrl Pts',(55.9834806996654,261.989156810136,20.2577663562296)) ;
#89124=CARTESIAN_POINT('Ctrl Pts',(55.9912961311385,261.986082334998,20.253923262308)) ;
#89125=CARTESIAN_POINT('Ctrl Pts',(55.9992662548239,261.983205399202,20.2503270925619)) ;
#89126=CARTESIAN_POINT('Ctrl Pts',(56.0062869640403,261.980671168811,20.2471593045731)) ;
#89127=CARTESIAN_POINT('Ctrl Pts',(56.0134277031511,261.978290217307,20.244183115193)) ;
#89128=CARTESIAN_POINT('Ctrl Pts',(56.0206680705166,261.976067940801,20.2414052695604)) ;
#89129=CARTESIAN_POINT('Ctrl Pts',(56.0271821933992,261.974068569566,20.2389060555169)) ;
#89130=CARTESIAN_POINT('Ctrl Pts',(56.0337779379306,261.972197164793,20.2365667995501)) ;
#89131=CARTESIAN_POINT('Ctrl Pts',(56.0404403335848,261.970457505536,20.23439222548)) ;
#89132=CARTESIAN_POINT('Ctrl Pts',(56.0445887481694,261.969374287395,20.2330382028047)) ;
#89133=CARTESIAN_POINT('Ctrl Pts',(56.0487630052482,261.96834214749,20.2317480279244)) ;
#89134=CARTESIAN_POINT('Ctrl Pts',(56.0529610797319,261.967360010175,20.2305203562874)) ;
#89135=CARTESIAN_POINT('Ctrl Pts',(56.0629996414285,261.965011493953,20.2275847110245)) ;
#89136=CARTESIAN_POINT('Ctrl Pts',(56.0731702750401,261.962953857029,20.2250126648544)) ;
#89137=CARTESIAN_POINT('Ctrl Pts',(56.083450668956,261.961167864353,20.2227801740048)) ;
#89138=CARTESIAN_POINT('Ctrl Pts',(56.0834769606655,261.961163296746,20.2227744644958)) ;
#89139=CARTESIAN_POINT('Ctrl Pts',(56.0835032530946,261.961158730916,20.2227687572091)) ;
#89140=CARTESIAN_POINT('Ctrl Pts',(56.0835295462434,261.961154166864,20.2227630521437)) ;
#89141=CARTESIAN_POINT('Ctrl Pts',(56.0980833454394,261.958627869948,20.2196051809913)) ;
#89142=CARTESIAN_POINT('Ctrl Pts',(56.1128624571979,261.956645585289,20.2171273251705)) ;
#89143=CARTESIAN_POINT('Ctrl Pts',(56.1278768193434,261.955106576005,20.215203563567)) ;
#89144=CARTESIAN_POINT('Ctrl Pts',(56.1299108979432,261.954898077914,20.2149429409531)) ;
#89145=CARTESIAN_POINT('Ctrl Pts',(56.1319492921022,261.954697711593,20.2146924830527)) ;
#89146=CARTESIAN_POINT('Ctrl Pts',(56.1339920253113,261.954505223791,20.2144518733006)) ;
#89147=CARTESIAN_POINT('Ctrl Pts',(56.1470546902204,261.953274322151,20.2129132462534)) ;
#89148=CARTESIAN_POINT('Ctrl Pts',(56.1602993589054,261.952367232026,20.2117793835923)) ;
#89149=CARTESIAN_POINT('Ctrl Pts',(56.1737344620585,261.951714748922,20.2109637797128)) ;
#89150=CARTESIAN_POINT('Ctrl Pts',(56.1744674056311,261.951679153118,20.210919284958)) ;
#89151=CARTESIAN_POINT('Ctrl Pts',(56.1752009165622,261.951644315065,20.210875737391)) ;
#89152=CARTESIAN_POINT('Ctrl Pts',(56.1759349892867,261.951610219791,20.210833118299)) ;
#89153=CARTESIAN_POINT('Ctrl Pts',(56.1882999108463,261.951035909686,20.2101152306677)) ;
#89154=CARTESIAN_POINT('Ctrl Pts',(56.2008266725393,261.950673148754,20.2096617795031)) ;
#89155=CARTESIAN_POINT('Ctrl Pts',(56.2134912420145,261.950453035381,20.2093866377862)) ;
#89156=CARTESIAN_POINT('Ctrl Pts',(56.2160120270313,261.950409223509,20.2093318729464)) ;
#89157=CARTESIAN_POINT('Ctrl Pts',(56.218537945353,261.950370958144,20.2092840412407)) ;
#89158=CARTESIAN_POINT('Ctrl Pts',(56.221068929131,261.950337727748,20.2092425032449)) ;
#89159=CARTESIAN_POINT('Ctrl Pts',(56.2299314802775,261.950221367424,20.2090970528413)) ;
#89160=CARTESIAN_POINT('Ctrl Pts',(56.2388562189851,261.95016674229,20.2090287714307)) ;
#89161=CARTESIAN_POINT('Ctrl Pts',(56.2478153214656,261.950142093806,20.2089979608233)) ;
#89162=CARTESIAN_POINT('Ctrl Pts',(56.2550320831194,261.950122238889,20.2089731421754)) ;
#89163=CARTESIAN_POINT('Ctrl Pts',(56.2622712892624,261.950121980978,20.2089728197824)) ;
#89164=CARTESIAN_POINT('Ctrl Pts',(56.2695111541429,261.950121980978,20.2089728197824)) ;
#89165=CARTESIAN_POINT('Origin',(56.2695111541429,261.559687576257,20.5213203435596)) ;
#89166=CARTESIAN_POINT('Ctrl Pts',(55.5095145719656,261.79455482774,20.2277364888237)) ;
#89167=CARTESIAN_POINT('Ctrl Pts',(55.5318704226011,261.835587804427,20.2336372451564)) ;
#89168=CARTESIAN_POINT('Ctrl Pts',(55.5809822967928,261.905784092892,20.2463148514966)) ;
#89169=CARTESIAN_POINT('Ctrl Pts',(55.7142947487837,261.996615667805,20.2848817332965)) ;
#89170=CARTESIAN_POINT('Ctrl Pts',(55.8167520150608,262.046133815589,20.3289876130455)) ;
#89171=CARTESIAN_POINT('Ctrl Pts',(55.8638558727399,262.066371572297,20.3542848089307)) ;
#89172=CARTESIAN_POINT('Ctrl Pts',(55.5021508781933,261.805895393144,20.239612427161)) ;
#89173=CARTESIAN_POINT('Ctrl Pts',(55.5245129486454,261.845948338582,20.2451930175294)) ;
#89174=CARTESIAN_POINT('Ctrl Pts',(55.5734190414891,261.915123351253,20.2575607551273)) ;
#89175=CARTESIAN_POINT('Ctrl Pts',(55.7070692316063,262.006295891711,20.2968962781282)) ;
#89176=CARTESIAN_POINT('Ctrl Pts',(55.8078507833606,262.055426513127,20.3406034849686)) ;
#89177=CARTESIAN_POINT('Ctrl Pts',(55.8547221940317,262.075352656397,20.3655111640554)) ;
#89178=CARTESIAN_POINT('Ctrl Pts',(55.4880735456019,261.829072700441,20.2645630186822)) ;
#89179=CARTESIAN_POINT('Ctrl Pts',(55.5104117488909,261.867380393505,20.2695523766429)) ;
#89180=CARTESIAN_POINT('Ctrl Pts',(55.559902068292,261.934673156301,20.2813591433882)) ;
#89181=CARTESIAN_POINT('Ctrl Pts',(55.6936488281965,262.02682092658,20.3223088243929)) ;
#89182=CARTESIAN_POINT('Ctrl Pts',(55.7912089494402,262.074940512162,20.3649959837617)) ;
#89183=CARTESIAN_POINT('Ctrl Pts',(55.8376310823803,262.094199248694,20.3890694044266)) ;
#89184=CARTESIAN_POINT('Ctrl Pts',(55.4699650328212,261.866144293726,20.3064310132397)) ;
#89185=CARTESIAN_POINT('Ctrl Pts',(55.4929957908261,261.902377349883,20.3106523286683)) ;
#89186=CARTESIAN_POINT('Ctrl Pts',(55.546126482402,261.967512823357,20.3217909930518)) ;
#89187=CARTESIAN_POINT('Ctrl Pts',(55.6762898619748,262.061105323079,20.3645153425193)) ;
#89188=CARTESIAN_POINT('Ctrl Pts',(55.7702332408511,262.106446960815,20.4043790445782)) ;
#89189=CARTESIAN_POINT('Ctrl Pts',(55.816111301075,262.12434494673,20.4267515269718)) ;
#89190=CARTESIAN_POINT('Ctrl Pts',(55.4520758007103,261.906852049728,20.3536557306369)) ;
#89191=CARTESIAN_POINT('Ctrl Pts',(55.4739718660818,261.941532580139,20.3569670015285)) ;
#89192=CARTESIAN_POINT('Ctrl Pts',(55.5356402846097,262.004945670765,20.3676331273513)) ;
#89193=CARTESIAN_POINT('Ctrl Pts',(55.6630577627351,262.098567808436,20.4105259197655)) ;
#89194=CARTESIAN_POINT('Ctrl Pts',(55.7537573949811,262.139559060658,20.4457691693816)) ;
#89195=CARTESIAN_POINT('Ctrl Pts',(55.7992124503129,262.155600230362,20.4658206315121)) ;
#89196=CARTESIAN_POINT('Ctrl Pts',(55.4413189890535,261.951943447046,20.4076656249392)) ;
#89197=CARTESIAN_POINT('Ctrl Pts',(55.4685727933187,261.985027606168,20.4101150870237)) ;
#89198=CARTESIAN_POINT('Ctrl Pts',(55.5256447361003,262.048195315495,20.4196062026645)) ;
#89199=CARTESIAN_POINT('Ctrl Pts',(55.655240746667,262.138550523405,20.4597488079456)) ;
#89200=CARTESIAN_POINT('Ctrl Pts',(55.7421185070325,262.173732522086,20.488485996167)) ;
#89201=CARTESIAN_POINT('Ctrl Pts',(55.7871294431314,262.187426540391,20.5056035190482)) ;
#89202=CARTESIAN_POINT('Ctrl Pts',(55.4339566679902,262.003588608482,20.4698817737906)) ;
#89203=CARTESIAN_POINT('Ctrl Pts',(55.4606880082801,262.035663654577,20.4708390649677)) ;
#89204=CARTESIAN_POINT('Ctrl Pts',(55.5235568044765,262.097388906199,20.4785782506978)) ;
#89205=CARTESIAN_POINT('Ctrl Pts',(55.6508626693057,262.180531558113,20.5114075592019)) ;
#89206=CARTESIAN_POINT('Ctrl Pts',(55.7350394275834,262.208890877721,20.5324339407107)) ;
#89207=CARTESIAN_POINT('Ctrl Pts',(55.7793466606563,262.219881088534,20.5461717042271)) ;
#89208=CARTESIAN_POINT('Ctrl Pts',(55.4320069322682,262.063615725155,20.5417594331499)) ;
#89209=CARTESIAN_POINT('Ctrl Pts',(55.4607036186458,262.094102965218,20.5405796731094)) ;
#89210=CARTESIAN_POINT('Ctrl Pts',(55.5260165932096,262.152758635894,20.5442555742965)) ;
#89211=CARTESIAN_POINT('Ctrl Pts',(55.6506170754938,262.223658860309,20.564760989951)) ;
#89212=CARTESIAN_POINT('Ctrl Pts',(55.7321897267531,262.244956725749,20.5775162507453)) ;
#89213=CARTESIAN_POINT('Ctrl Pts',(55.7755030403665,262.252890970876,20.5874340571549)) ;
#89214=CARTESIAN_POINT('Ctrl Pts',(55.4372381689899,262.132341396724,20.6226948020985)) ;
#89215=CARTESIAN_POINT('Ctrl Pts',(55.4672574673095,262.160051164332,20.6179839815041)) ;
#89216=CARTESIAN_POINT('Ctrl Pts',(55.535055068772,262.211948592104,20.6140283051287)) ;
#89217=CARTESIAN_POINT('Ctrl Pts',(55.6545305697442,262.266520428154,20.6180877115192)) ;
#89218=CARTESIAN_POINT('Ctrl Pts',(55.7339304470145,262.281174467558,20.6227884280072)) ;
#89219=CARTESIAN_POINT('Ctrl Pts',(55.7758592437434,262.285802712839,20.6285737346079)) ;
#89220=CARTESIAN_POINT('Ctrl Pts',(55.4523935735627,262.206184157921,20.7072597357073)) ;
#89221=CARTESIAN_POINT('Ctrl Pts',(55.4830627961843,262.229306963324,20.6976358460879)) ;
#89222=CARTESIAN_POINT('Ctrl Pts',(55.5507543239758,262.270631714132,20.6830746334434)) ;
#89223=CARTESIAN_POINT('Ctrl Pts',(55.6635699821141,262.307900047814,20.6697105532676)) ;
#89224=CARTESIAN_POINT('Ctrl Pts',(55.7406360766256,262.316640091316,20.6671204577043)) ;
#89225=CARTESIAN_POINT('Ctrl Pts',(55.7806429509047,262.317878574873,20.6686685621508)) ;
#89226=CARTESIAN_POINT('Ctrl Pts',(55.4781604356767,262.278168118765,20.7871118425305)) ;
#89227=CARTESIAN_POINT('Ctrl Pts',(55.5080300138342,262.295736009422,20.772627604968)) ;
#89228=CARTESIAN_POINT('Ctrl Pts',(55.5728717758892,262.325199710388,20.7472936904588)) ;
#89229=CARTESIAN_POINT('Ctrl Pts',(55.678507170532,262.34810030968,20.7195478001993)) ;
#89230=CARTESIAN_POINT('Ctrl Pts',(55.7521512287222,262.350721354057,20.7097220361308)) ;
#89231=CARTESIAN_POINT('Ctrl Pts',(55.789593096855,262.34862473989,20.7071012684221)) ;
#89232=CARTESIAN_POINT('Ctrl Pts',(55.5008488901186,262.323452680659,20.8366594790575)) ;
#89233=CARTESIAN_POINT('Ctrl Pts',(55.5294141416451,262.337477501983,20.8194278639549)) ;
#89234=CARTESIAN_POINT('Ctrl Pts',(55.5909766067113,262.35982539795,20.7880695269394)) ;
#89235=CARTESIAN_POINT('Ctrl Pts',(55.691882974598,262.375012422702,20.7524880639786)) ;
#89236=CARTESIAN_POINT('Ctrl Pts',(55.762148436109,262.372604836401,20.7370763890607)) ;
#89237=CARTESIAN_POINT('Ctrl Pts',(55.7975023182572,262.368314961946,20.7317140459925)) ;
#89238=CARTESIAN_POINT('Ctrl Pts',(55.5133169212987,262.347205304054,20.8621241336292)) ;
#89239=CARTESIAN_POINT('Ctrl Pts',(55.5408880083649,262.359266249537,20.8435414012517)) ;
#89240=CARTESIAN_POINT('Ctrl Pts',(55.6003710788384,262.377970841319,20.8093031768376)) ;
#89241=CARTESIAN_POINT('Ctrl Pts',(55.6986198286852,262.388518764252,20.7690288804046)) ;
#89242=CARTESIAN_POINT('Ctrl Pts',(55.7671947747017,262.3835623992,20.7507733425594)) ;
#89243=CARTESIAN_POINT('Ctrl Pts',(55.8014829417656,262.378142623667,20.743998623144)) ;
#89244=CARTESIAN_POINT('',(55.5133169212987,262.347205304054,20.8621241336292)) ;
#89245=CARTESIAN_POINT('Ctrl Pts',(55.5095145719656,261.79455482774,20.2277364888237)) ;
#89246=CARTESIAN_POINT('Ctrl Pts',(55.5021508781933,261.805895393144,20.239612427161)) ;
#89247=CARTESIAN_POINT('Ctrl Pts',(55.4880735456018,261.829072700441,20.2645630186821)) ;
#89248=CARTESIAN_POINT('Ctrl Pts',(55.4699650328212,261.866144293726,20.3064310132397)) ;
#89249=CARTESIAN_POINT('Ctrl Pts',(55.4520758007103,261.906852049728,20.3536557306369)) ;
#89250=CARTESIAN_POINT('Ctrl Pts',(55.4413189890535,261.951943447046,20.4076656249392)) ;
#89251=CARTESIAN_POINT('Ctrl Pts',(55.4339566679903,262.003588608482,20.4698817737906)) ;
#89252=CARTESIAN_POINT('Ctrl Pts',(55.4320069322682,262.063615725155,20.5417594331499)) ;
#89253=CARTESIAN_POINT('Ctrl Pts',(55.4372381689898,262.132341396724,20.6226948020985)) ;
#89254=CARTESIAN_POINT('Ctrl Pts',(55.4523935735627,262.206184157921,20.7072597357073)) ;
#89255=CARTESIAN_POINT('Ctrl Pts',(55.4781604356767,262.278168118765,20.7871118425305)) ;
#89256=CARTESIAN_POINT('Ctrl Pts',(55.5008488901186,262.323452680659,20.8366594790575)) ;
#89257=CARTESIAN_POINT('Ctrl Pts',(55.5133169212987,262.347205304054,20.8621241336292)) ;
#89258=CARTESIAN_POINT('',(55.8014829417656,262.378142623667,20.743998623144)) ;
#89259=CARTESIAN_POINT('Origin',(55.8014829417656,261.987708218946,21.0563461469212)) ;
#89260=CARTESIAN_POINT('Ctrl Pts',(55.8014829417656,262.378142623667,20.743998623144)) ;
#89261=CARTESIAN_POINT('Ctrl Pts',(55.7991573587302,262.372401049934,20.7368216559782)) ;
#89262=CARTESIAN_POINT('Ctrl Pts',(55.7968348028396,262.366657445889,20.7296421510009)) ;
#89263=CARTESIAN_POINT('Ctrl Pts',(55.7946197225382,262.360866471452,20.7224034329287)) ;
#89264=CARTESIAN_POINT('Ctrl Pts',(55.7930432612197,262.356745064571,20.7172516743091)) ;
#89265=CARTESIAN_POINT('Ctrl Pts',(55.7915186399541,262.352601013753,20.7120716107602)) ;
#89266=CARTESIAN_POINT('Ctrl Pts',(55.7900769583761,262.348423032613,20.7068491343307)) ;
#89267=CARTESIAN_POINT('Ctrl Pts',(55.7893457597689,262.346304025173,20.7042003750277)) ;
#89268=CARTESIAN_POINT('Ctrl Pts',(55.7886358870253,262.344176285044,20.7015406998662)) ;
#89269=CARTESIAN_POINT('Ctrl Pts',(55.7879489827639,262.342039856916,20.6988701647101)) ;
#89270=CARTESIAN_POINT('Ctrl Pts',(55.7857762248067,262.33528208662,20.6904229518515)) ;
#89271=CARTESIAN_POINT('Ctrl Pts',(55.7838412913505,262.328431054561,20.6818591617716)) ;
#89272=CARTESIAN_POINT('Ctrl Pts',(55.7822046176232,262.3214814517,20.673172158189)) ;
#89273=CARTESIAN_POINT('Ctrl Pts',(55.7819051330084,262.320209787654,20.6715825781292)) ;
#89274=CARTESIAN_POINT('Ctrl Pts',(55.7816155233921,262.318934967357,20.6699890527579)) ;
#89275=CARTESIAN_POINT('Ctrl Pts',(55.7813361907946,262.317656922226,20.6683914963437)) ;
#89276=CARTESIAN_POINT('Ctrl Pts',(55.7799457578442,262.311295201187,20.6604393450441)) ;
#89277=CARTESIAN_POINT('Ctrl Pts',(55.7788098142623,262.304853533795,20.6523872608128)) ;
#89278=CARTESIAN_POINT('Ctrl Pts',(55.7779419835549,262.298346676154,20.6442536887576)) ;
#89279=CARTESIAN_POINT('Ctrl Pts',(55.7773814313783,262.294143744426,20.6390000240963)) ;
#89280=CARTESIAN_POINT('Ctrl Pts',(55.7769320002345,262.289914226983,20.6337131272905)) ;
#89281=CARTESIAN_POINT('Ctrl Pts',(55.7765961607768,262.285663289202,20.6283994550628)) ;
#89282=CARTESIAN_POINT('Ctrl Pts',(55.7761841937201,262.280448755037,20.6218812873552)) ;
#89283=CARTESIAN_POINT('Ctrl Pts',(55.7759431555174,262.275201990712,20.615322831949)) ;
#89284=CARTESIAN_POINT('Ctrl Pts',(55.7758684038679,262.26993703184,20.608741633359)) ;
#89285=CARTESIAN_POINT('Ctrl Pts',(55.7757878800543,262.264265523994,20.6016522485523)) ;
#89286=CARTESIAN_POINT('Ctrl Pts',(55.7759011734486,262.258572201006,20.594535594817)) ;
#89287=CARTESIAN_POINT('Ctrl Pts',(55.7762026881147,262.252874555225,20.5874135375915)) ;
#89288=CARTESIAN_POINT('Ctrl Pts',(55.7764544426288,262.248117214352,20.5814668614997)) ;
#89289=CARTESIAN_POINT('Ctrl Pts',(55.7768374163714,262.243356859504,20.5755164179393)) ;
#89290=CARTESIAN_POINT('Ctrl Pts',(55.7773478415344,262.238602506964,20.5695734772651)) ;
#89291=CARTESIAN_POINT('Ctrl Pts',(55.7780162384643,262.23237672722,20.5617912525844)) ;
#89292=CARTESIAN_POINT('Ctrl Pts',(55.7789034723116,262.226161192034,20.5540218336032)) ;
#89293=CARTESIAN_POINT('Ctrl Pts',(55.7800025150514,262.219973478099,20.5462871911838)) ;
#89294=CARTESIAN_POINT('Ctrl Pts',(55.7803506975784,262.218013177743,20.5438368157386)) ;
#89295=CARTESIAN_POINT('Ctrl Pts',(55.7807201433493,262.216055670913,20.5413899322016)) ;
#89296=CARTESIAN_POINT('Ctrl Pts',(55.7811112438686,262.214100958861,20.5389465421364)) ;
#89297=CARTESIAN_POINT('Ctrl Pts',(55.7826261697489,262.206529391629,20.529482083096)) ;
#89298=CARTESIAN_POINT('Ctrl Pts',(55.7844636665024,262.199005975118,20.5200778124559)) ;
#89299=CARTESIAN_POINT('Ctrl Pts',(55.78664185792,262.191537798588,20.5107425917956)) ;
#89300=CARTESIAN_POINT('Ctrl Pts',(55.7870318798326,262.190200564188,20.5090710487957)) ;
#89301=CARTESIAN_POINT('Ctrl Pts',(55.7874328447887,262.188864923484,20.507401497916)) ;
#89302=CARTESIAN_POINT('Ctrl Pts',(55.7878449073235,262.187530870786,20.5057339320444)) ;
#89303=CARTESIAN_POINT('Ctrl Pts',(55.7898993187327,262.180879712646,20.4974199843724)) ;
#89304=CARTESIAN_POINT('Ctrl Pts',(55.7922294437967,262.174267976547,20.4891553142605)) ;
#89305=CARTESIAN_POINT('Ctrl Pts',(55.7948616136521,262.167690167664,20.4809330531478)) ;
#89306=CARTESIAN_POINT('Ctrl Pts',(55.7964672004132,262.163677796335,20.4759175889817)) ;
#89307=CARTESIAN_POINT('Ctrl Pts',(55.7981833380746,262.159679471643,20.4709196831148)) ;
#89308=CARTESIAN_POINT('Ctrl Pts',(55.8000143657964,262.155695146818,20.4659392770827)) ;
#89309=CARTESIAN_POINT('Ctrl Pts',(55.801824812773,262.15175560579,20.4610148507967)) ;
#89310=CARTESIAN_POINT('Ctrl Pts',(55.8037475810324,262.147829752407,20.4561075340681)) ;
#89311=CARTESIAN_POINT('Ctrl Pts',(55.8057805190409,262.143922743729,20.4512237732206)) ;
#89312=CARTESIAN_POINT('Ctrl Pts',(55.8091738951825,262.137401172497,20.4430718091804)) ;
#89313=CARTESIAN_POINT('Ctrl Pts',(55.8128771536114,262.130929204255,20.4349818488788)) ;
#89314=CARTESIAN_POINT('Ctrl Pts',(55.8168812880823,262.124529812421,20.4269826090862)) ;
#89315=CARTESIAN_POINT('Ctrl Pts',(55.8185339153892,262.121888590013,20.4236810810753)) ;
#89316=CARTESIAN_POINT('Ctrl Pts',(55.8202377903298,262.11925972928,20.4203950051593)) ;
#89317=CARTESIAN_POINT('Ctrl Pts',(55.8219913716022,262.116645490428,20.4171272065948)) ;
#89318=CARTESIAN_POINT('Ctrl Pts',(55.8270320588606,262.109130834177,20.4077338862809)) ;
#89319=CARTESIAN_POINT('Ctrl Pts',(55.8324856267513,262.101735225616,20.3984893755799)) ;
#89320=CARTESIAN_POINT('Ctrl Pts',(55.83831695648,262.094511770528,20.3894600567187)) ;
#89321=CARTESIAN_POINT('Ctrl Pts',(55.8429762944998,262.088740099143,20.3822454674877)) ;
#89322=CARTESIAN_POINT('Ctrl Pts',(55.8478767960498,262.083078335888,20.3751682634189)) ;
#89323=CARTESIAN_POINT('Ctrl Pts',(55.8529974353104,262.077553870314,20.368262681452)) ;
#89324=CARTESIAN_POINT('Ctrl Pts',(55.8565149891311,262.073758913474,20.3635189854023)) ;
#89325=CARTESIAN_POINT('Ctrl Pts',(55.8601365537588,262.070028753333,20.3588562852258)) ;
#89326=CARTESIAN_POINT('Ctrl Pts',(55.8638558727399,262.066371572297,20.3542848089307)) ;
#89327=CARTESIAN_POINT('Ctrl Pts',(55.5095145719656,261.79455482774,20.2277364888237)) ;
#89328=CARTESIAN_POINT('Ctrl Pts',(55.5021508781933,261.805895393144,20.239612427161)) ;
#89329=CARTESIAN_POINT('Ctrl Pts',(55.4880735456018,261.829072700441,20.2645630186821)) ;
#89330=CARTESIAN_POINT('Ctrl Pts',(55.4699650328212,261.866144293726,20.3064310132397)) ;
#89331=CARTESIAN_POINT('Ctrl Pts',(55.4520758007103,261.906852049728,20.3536557306369)) ;
#89332=CARTESIAN_POINT('Ctrl Pts',(55.4413189890535,261.951943447046,20.4076656249392)) ;
#89333=CARTESIAN_POINT('Ctrl Pts',(55.4339566679903,262.003588608482,20.4698817737906)) ;
#89334=CARTESIAN_POINT('Ctrl Pts',(55.4320069322682,262.063615725155,20.5417594331499)) ;
#89335=CARTESIAN_POINT('Ctrl Pts',(55.4372381689898,262.132341396724,20.6226948020985)) ;
#89336=CARTESIAN_POINT('Ctrl Pts',(55.4523935735627,262.206184157921,20.7072597357073)) ;
#89337=CARTESIAN_POINT('Ctrl Pts',(55.4781604356767,262.278168118765,20.7871118425305)) ;
#89338=CARTESIAN_POINT('Ctrl Pts',(55.5008488901186,262.323452680659,20.8366594790575)) ;
#89339=CARTESIAN_POINT('Ctrl Pts',(55.5133169212987,262.347205304054,20.8621241336292)) ;
#89340=CARTESIAN_POINT('Ctrl Pts',(55.4626130754224,261.791323735734,20.2614221936152)) ;
#89341=CARTESIAN_POINT('Ctrl Pts',(55.456933189044,261.80292645307,20.2736403319025)) ;
#89342=CARTESIAN_POINT('Ctrl Pts',(55.4459364134233,261.82662567018,20.299221698274)) ;
#89343=CARTESIAN_POINT('Ctrl Pts',(55.4318517617125,261.864376559775,20.3418755777896)) ;
#89344=CARTESIAN_POINT('Ctrl Pts',(55.4170849015297,261.905634161402,20.3897054228805)) ;
#89345=CARTESIAN_POINT('Ctrl Pts',(55.4094946332789,261.951022937766,20.4441389408264)) ;
#89346=CARTESIAN_POINT('Ctrl Pts',(55.4043163979937,262.002731372621,20.5064211995693)) ;
#89347=CARTESIAN_POINT('Ctrl Pts',(55.4041907996858,262.06216052464,20.5774476075643)) ;
#89348=CARTESIAN_POINT('Ctrl Pts',(55.410843827055,262.128931911869,20.65558394842)) ;
#89349=CARTESIAN_POINT('Ctrl Pts',(55.4267179821464,262.199434726762,20.7352219757316)) ;
#89350=CARTESIAN_POINT('Ctrl Pts',(55.4519739561487,262.268120582844,20.8098095523395)) ;
#89351=CARTESIAN_POINT('Ctrl Pts',(55.4736689753899,262.312067039713,20.8567205002237)) ;
#89352=CARTESIAN_POINT('Ctrl Pts',(55.4857458342326,262.33514435857,20.8807068660068)) ;
#89353=CARTESIAN_POINT('Ctrl Pts',(55.3860532767111,261.781008579942,20.3361055438638)) ;
#89354=CARTESIAN_POINT('Ctrl Pts',(55.3825955021332,261.793201335109,20.3488988744911)) ;
#89355=CARTESIAN_POINT('Ctrl Pts',(55.3757040049108,261.818043148829,20.3756388327424)) ;
#89356=CARTESIAN_POINT('Ctrl Pts',(55.3669780343311,261.857372312824,20.4202275315097)) ;
#89357=CARTESIAN_POINT('Ctrl Pts',(55.3559877265066,261.900120114085,20.4701859646172)) ;
#89358=CARTESIAN_POINT('Ctrl Pts',(55.3525696678913,261.946639790849,20.5267824467788)) ;
#89359=CARTESIAN_POINT('Ctrl Pts',(55.3501888273653,261.998688786346,20.5899899103179)) ;
#89360=CARTESIAN_POINT('Ctrl Pts',(55.353194091183,262.056267188396,20.6585894493622)) ;
#89361=CARTESIAN_POINT('Ctrl Pts',(55.3625023028779,262.118055719835,20.7292468247288)) ;
#89362=CARTESIAN_POINT('Ctrl Pts',(55.3795168054528,262.181156991198,20.7971576993123)) ;
#89363=CARTESIAN_POINT('Ctrl Pts',(55.4035892741016,262.242857727496,20.8596399172166)) ;
#89364=CARTESIAN_POINT('Ctrl Pts',(55.42361623327,262.283862452034,20.9001120203024)) ;
#89365=CARTESIAN_POINT('Ctrl Pts',(55.4349467887998,262.305606144961,20.9207980665079)) ;
#89366=CARTESIAN_POINT('Ctrl Pts',(55.2919386084249,261.742010571783,20.5272717802442)) ;
#89367=CARTESIAN_POINT('Ctrl Pts',(55.2905609388079,261.756084194904,20.5407912325947)) ;
#89368=CARTESIAN_POINT('Ctrl Pts',(55.2875844799747,261.784514567651,20.568652899067)) ;
#89369=CARTESIAN_POINT('Ctrl Pts',(55.2843693955679,261.828488818617,20.613161965571)) ;
#89370=CARTESIAN_POINT('Ctrl Pts',(55.2787014910525,261.874606326743,20.6598246389281)) ;
#89371=CARTESIAN_POINT('Ctrl Pts',(55.282339584292,261.922376601744,20.7084339193678)) ;
#89372=CARTESIAN_POINT('Ctrl Pts',(55.2867532550598,261.972820267034,20.7571463593862)) ;
#89373=CARTESIAN_POINT('Ctrl Pts',(55.2961707426459,262.025232807302,20.8049516990132)) ;
#89374=CARTESIAN_POINT('Ctrl Pts',(55.3097166755623,262.078984671258,20.8509463776884)) ;
#89375=CARTESIAN_POINT('Ctrl Pts',(55.3274619515341,262.133564899343,20.895158309429)) ;
#89376=CARTESIAN_POINT('Ctrl Pts',(55.3488908311421,262.189257575911,20.9398889939635)) ;
#89377=CARTESIAN_POINT('Ctrl Pts',(55.3657889087667,262.227536454716,20.9716659960487)) ;
#89378=CARTESIAN_POINT('Ctrl Pts',(55.3751920600054,262.247035598335,20.9870170813929)) ;
#89379=CARTESIAN_POINT('Ctrl Pts',(55.2649157169606,261.69184073163,20.6679797590307)) ;
#89380=CARTESIAN_POINT('Ctrl Pts',(55.2649086000589,261.708286029276,20.6789611373507)) ;
#89381=CARTESIAN_POINT('Ctrl Pts',(55.2648440073611,261.741176973179,20.7012707802754)) ;
#89382=CARTESIAN_POINT('Ctrl Pts',(55.2650501911457,261.790617905123,20.7359777828176)) ;
#89383=CARTESIAN_POINT('Ctrl Pts',(55.2647071106602,261.840419413326,20.7716773112338)) ;
#89384=CARTESIAN_POINT('Ctrl Pts',(55.2685704487611,261.890478004158,20.8085365763669)) ;
#89385=CARTESIAN_POINT('Ctrl Pts',(55.2743403282809,261.941338432843,20.8457412040926)) ;
#89386=CARTESIAN_POINT('Ctrl Pts',(55.2830463917309,261.992700907183,20.883401123301)) ;
#89387=CARTESIAN_POINT('Ctrl Pts',(55.2945926429713,262.04449713072,20.9211540604301)) ;
#89388=CARTESIAN_POINT('Ctrl Pts',(55.3091555672942,262.096549677205,20.9587162447594)) ;
#89389=CARTESIAN_POINT('Ctrl Pts',(55.326770477828,262.148491465379,20.9961671298381)) ;
#89390=CARTESIAN_POINT('Ctrl Pts',(55.3405568610208,262.182853784487,21.0212206455135)) ;
#89391=CARTESIAN_POINT('Ctrl Pts',(55.3481064294777,262.200232606203,21.0332361465525)) ;
#89392=CARTESIAN_POINT('Ctrl Pts',(55.2649122781271,261.665580342705,20.7284379454282)) ;
#89393=CARTESIAN_POINT('Ctrl Pts',(55.2649104802532,261.683350669897,20.7386049292427)) ;
#89394=CARTESIAN_POINT('Ctrl Pts',(55.264874404684,261.718678953952,20.7593137062813)) ;
#89395=CARTESIAN_POINT('Ctrl Pts',(55.2650136524204,261.771002970452,20.7914811683607)) ;
#89396=CARTESIAN_POINT('Ctrl Pts',(55.2646380837014,261.822823681129,20.8244650422272)) ;
#89397=CARTESIAN_POINT('Ctrl Pts',(55.267246242196,261.87415188769,20.8581387118653)) ;
#89398=CARTESIAN_POINT('Ctrl Pts',(55.2723439409786,261.925296254531,20.8917898342268)) ;
#89399=CARTESIAN_POINT('Ctrl Pts',(55.2800868920873,261.97606891941,20.9255063012982)) ;
#89400=CARTESIAN_POINT('Ctrl Pts',(55.2904575118652,262.026562708551,20.9589320611357)) ;
#89401=CARTESIAN_POINT('Ctrl Pts',(55.3034984602722,262.076742149292,20.9918978037114)) ;
#89402=CARTESIAN_POINT('Ctrl Pts',(55.3191977410406,262.126387158599,21.0245040383623)) ;
#89403=CARTESIAN_POINT('Ctrl Pts',(55.3314042901508,262.158997112573,21.0460840685968)) ;
#89404=CARTESIAN_POINT('Ctrl Pts',(55.3380548194638,262.175416437892,21.0563461469212)) ;
#89405=CARTESIAN_POINT('',(55.2649122781606,261.665580028629,20.7284377450722)) ;
#89406=CARTESIAN_POINT('Ctrl Pts',(55.5095145719656,261.79455482774,20.2277364888237)) ;
#89407=CARTESIAN_POINT('Ctrl Pts',(55.4626130754224,261.791323735734,20.2614221936152)) ;
#89408=CARTESIAN_POINT('Ctrl Pts',(55.3860532767111,261.781008579942,20.3361055438638)) ;
#89409=CARTESIAN_POINT('Ctrl Pts',(55.2919386177282,261.742010575638,20.5272717613472)) ;
#89410=CARTESIAN_POINT('Ctrl Pts',(55.2649157249743,261.691840746508,20.6679797173033)) ;
#89411=CARTESIAN_POINT('Ctrl Pts',(55.2649122781302,261.665580366068,20.728437891641)) ;
#89412=CARTESIAN_POINT('',(55.2648833765136,261.800000087205,20.8099471270963)) ;
#89413=CARTESIAN_POINT('Ctrl Pts',(55.264912278126,261.665580353186,20.728437951425)) ;
#89414=CARTESIAN_POINT('Ctrl Pts',(55.2649116845233,261.67144754861,20.7317947653228)) ;
#89415=CARTESIAN_POINT('Ctrl Pts',(55.2649094006061,261.6771004327,20.7350471228012)) ;
#89416=CARTESIAN_POINT('Ctrl Pts',(55.2649071885691,261.682520862898,20.7381870921931)) ;
#89417=CARTESIAN_POINT('Ctrl Pts',(55.2649051367789,261.687548620226,20.7410995924083)) ;
#89418=CARTESIAN_POINT('Ctrl Pts',(55.2649031330562,261.692375204843,20.7439171417652)) ;
#89419=CARTESIAN_POINT('Ctrl Pts',(55.2649020653765,261.697026581304,20.7466532077635)) ;
#89420=CARTESIAN_POINT('Ctrl Pts',(55.2649007202167,261.702886807363,20.7501003519362)) ;
#89421=CARTESIAN_POINT('Ctrl Pts',(55.2649008325002,261.708468494965,20.7534180622178)) ;
#89422=CARTESIAN_POINT('Ctrl Pts',(55.2649035864154,261.713918696501,20.7566853863074)) ;
#89423=CARTESIAN_POINT('Ctrl Pts',(55.2649043754765,261.715480306677,20.7576215510556)) ;
#89424=CARTESIAN_POINT('Ctrl Pts',(55.2649053808284,261.717031475024,20.7585537601388)) ;
#89425=CARTESIAN_POINT('Ctrl Pts',(55.2649066286006,261.718573526866,20.7594824355829)) ;
#89426=CARTESIAN_POINT('Ctrl Pts',(55.264908727046,261.721166878015,20.7610442388023)) ;
#89427=CARTESIAN_POINT('Ctrl Pts',(55.2649115070367,261.723734449957,20.7625960412854)) ;
#89428=CARTESIAN_POINT('Ctrl Pts',(55.264914577773,261.726282582634,20.7641397963417)) ;
#89429=CARTESIAN_POINT('Ctrl Pts',(55.2649199956029,261.730778360887,20.7668635086787)) ;
#89430=CARTESIAN_POINT('Ctrl Pts',(55.2649263016323,261.735213563686,20.7695605656014)) ;
#89431=CARTESIAN_POINT('Ctrl Pts',(55.2649315558431,261.739564585578,20.7722202638766)) ;
#89432=CARTESIAN_POINT('Ctrl Pts',(55.264939501443,261.746144351901,20.776242351924)) ;
#89433=CARTESIAN_POINT('Ctrl Pts',(55.2649447892793,261.752531922181,20.7801795081595)) ;
#89434=CARTESIAN_POINT('Ctrl Pts',(55.2649429787217,261.758523548692,20.7838956325582)) ;
#89435=CARTESIAN_POINT('Ctrl Pts',(55.2649417450228,261.762606193293,20.7864277688969)) ;
#89436=CARTESIAN_POINT('Ctrl Pts',(55.2649372853029,261.766502858534,20.788855812778)) ;
#89437=CARTESIAN_POINT('Ctrl Pts',(55.2649295433275,261.770147948255,20.791134949254)) ;
#89438=CARTESIAN_POINT('Ctrl Pts',(55.2649289946744,261.770406265999,20.7912964655502)) ;
#89439=CARTESIAN_POINT('Ctrl Pts',(55.2649284300825,261.770663330091,20.7914571915746)) ;
#89440=CARTESIAN_POINT('Ctrl Pts',(55.2649278497419,261.770919127213,20.7916171217019)) ;
#89441=CARTESIAN_POINT('Ctrl Pts',(55.2649207517931,261.774047694601,20.7935731725673)) ;
#89442=CARTESIAN_POINT('Ctrl Pts',(55.2649114923583,261.776986718916,20.7954101797538)) ;
#89443=CARTESIAN_POINT('Ctrl Pts',(55.2649033675045,261.779711801583,20.797117915298)) ;
#89444=CARTESIAN_POINT('Ctrl Pts',(55.2648952021657,261.782450462998,20.7988341602765)) ;
#89445=CARTESIAN_POINT('Ctrl Pts',(55.2648881394329,261.78497238351,20.8004196374816)) ;
#89446=CARTESIAN_POINT('Ctrl Pts',(55.2648833749291,261.7872887411,20.8018804120226)) ;
#89447=CARTESIAN_POINT('Ctrl Pts',(55.2648788571325,261.78948515714,20.8032655473092)) ;
#89448=CARTESIAN_POINT('Ctrl Pts',(55.2648763284609,261.79149632143,20.804538307404)) ;
#89449=CARTESIAN_POINT('Ctrl Pts',(55.2648758168632,261.793370917429,20.8057280000853)) ;
#89450=CARTESIAN_POINT('Ctrl Pts',(55.2648753337915,261.795140988699,20.806851357244)) ;
#89451=CARTESIAN_POINT('Ctrl Pts',(55.2648765899003,261.796789100496,20.8079005374401)) ;
#89452=CARTESIAN_POINT('Ctrl Pts',(55.2648796573053,261.798396281414,20.8089247864228)) ;
#89453=CARTESIAN_POINT('Ctrl Pts',(55.2648806830266,261.798933712801,20.8092672889662)) ;
#89454=CARTESIAN_POINT('Ctrl Pts',(55.264881915461,261.799466926199,20.8096072235845)) ;
#89455=CARTESIAN_POINT('Ctrl Pts',(55.2648833765136,261.800000087205,20.8099471270963)) ;
#89456=CARTESIAN_POINT('',(55.3380548194639,262.175416437892,21.0563461469212)) ;
#89457=CARTESIAN_POINT('Ctrl Pts',(55.2648833765465,261.800000099193,20.8099471347392)) ;
#89458=CARTESIAN_POINT('Ctrl Pts',(55.264887076765,261.801350363729,20.810807962245)) ;
#89459=CARTESIAN_POINT('Ctrl Pts',(55.2648921382654,261.802704527689,20.8116713360936)) ;
#89460=CARTESIAN_POINT('Ctrl Pts',(55.2648999326208,261.804196001596,20.8126249318168)) ;
#89461=CARTESIAN_POINT('Ctrl Pts',(55.2649079852912,261.805736904873,20.8136101309332)) ;
#89462=CARTESIAN_POINT('Ctrl Pts',(55.2649188903312,261.807424217338,20.8146915320592)) ;
#89463=CARTESIAN_POINT('Ctrl Pts',(55.2649360911695,261.809356367705,20.8159340062698)) ;
#89464=CARTESIAN_POINT('Ctrl Pts',(55.2649539728193,261.811364992857,20.8172256577855)) ;
#89465=CARTESIAN_POINT('Ctrl Pts',(55.2649785312904,261.813638039835,20.818691266036)) ;
#89466=CARTESIAN_POINT('Ctrl Pts',(55.2650171871798,261.816236845546,20.8203715342793)) ;
#89467=CARTESIAN_POINT('Ctrl Pts',(55.2650465915238,261.818213676981,20.8216496625624)) ;
#89468=CARTESIAN_POINT('Ctrl Pts',(55.265084237455,261.820379398754,20.8230503908865)) ;
#89469=CARTESIAN_POINT('Ctrl Pts',(55.2651353764379,261.822741913237,20.8245790678812)) ;
#89470=CARTESIAN_POINT('Ctrl Pts',(55.2651547797991,261.823638308109,20.8251590847361)) ;
#89471=CARTESIAN_POINT('Ctrl Pts',(55.2651761513239,261.824563031671,20.8257575242165)) ;
#89472=CARTESIAN_POINT('Ctrl Pts',(55.2651997562632,261.825516516964,20.8263746705597)) ;
#89473=CARTESIAN_POINT('Ctrl Pts',(55.2653002299749,261.829574998343,20.8290015353458)) ;
#89474=CARTESIAN_POINT('Ctrl Pts',(55.2654410724233,261.834152612198,20.8319735604999)) ;
#89475=CARTESIAN_POINT('Ctrl Pts',(55.2656422570234,261.839211915542,20.8352701409018)) ;
#89476=CARTESIAN_POINT('Ctrl Pts',(55.2658245152904,261.843795267643,20.8382565972742)) ;
#89477=CARTESIAN_POINT('Ctrl Pts',(55.2660564623741,261.848770288387,20.8415071128075)) ;
#89478=CARTESIAN_POINT('Ctrl Pts',(55.2663498860856,261.854070559063,20.8449782174637)) ;
#89479=CARTESIAN_POINT('Ctrl Pts',(55.2666975191413,261.860350042343,20.8490906005828)) ;
#89480=CARTESIAN_POINT('Ctrl Pts',(55.2671320468463,261.867085104201,20.8535121626097)) ;
#89481=CARTESIAN_POINT('Ctrl Pts',(55.2676612201599,261.874121981231,20.8581327504047)) ;
#89482=CARTESIAN_POINT('Ctrl Pts',(55.2677194642485,261.87489650345,20.8586413208826)) ;
#89483=CARTESIAN_POINT('Ctrl Pts',(55.2677788417528,261.875674684992,20.8591522975341)) ;
#89484=CARTESIAN_POINT('Ctrl Pts',(55.2678393634794,261.876456315003,20.8596655428744)) ;
#89485=CARTESIAN_POINT('Ctrl Pts',(55.2684840368388,261.884782185273,20.8651325976987)) ;
#89486=CARTESIAN_POINT('Ctrl Pts',(55.2692600300963,261.893493152603,20.870860923632)) ;
#89487=CARTESIAN_POINT('Ctrl Pts',(55.2701660419482,261.902315938472,20.8766742798029)) ;
#89488=CARTESIAN_POINT('Ctrl Pts',(55.2708959763049,261.90942407344,20.8813578481106)) ;
#89489=CARTESIAN_POINT('Ctrl Pts',(55.2717096489056,261.916603394402,20.8860956655889)) ;
#89490=CARTESIAN_POINT('Ctrl Pts',(55.2725968069079,261.923732793028,20.8908074049882)) ;
#89491=CARTESIAN_POINT('Ctrl Pts',(55.2726591307255,261.924233641061,20.8911384098222)) ;
#89492=CARTESIAN_POINT('Ctrl Pts',(55.2727218125129,261.924734239028,20.8914692811339)) ;
#89493=CARTESIAN_POINT('Ctrl Pts',(55.2727848485094,261.925234558655,20.8918000022097)) ;
#89494=CARTESIAN_POINT('Ctrl Pts',(55.273563027158,261.931410998673,20.89588275007)) ;
#89495=CARTESIAN_POINT('Ctrl Pts',(55.2743955029591,261.937544984512,20.899942595275)) ;
#89496=CARTESIAN_POINT('Ctrl Pts',(55.2752717329007,261.943585821033,20.9039445402612)) ;
#89497=CARTESIAN_POINT('Ctrl Pts',(55.2761597409042,261.949707856956,20.9080002783828)) ;
#89498=CARTESIAN_POINT('Ctrl Pts',(55.2770923617596,261.955733783538,20.9119962627578)) ;
#89499=CARTESIAN_POINT('Ctrl Pts',(55.2780621179994,261.961651586864,20.9159220749311)) ;
#89500=CARTESIAN_POINT('Ctrl Pts',(55.2788579412695,261.966507988299,20.9191437635918)) ;
#89501=CARTESIAN_POINT('Ctrl Pts',(55.2796785979965,261.971291439717,20.9223180969199)) ;
#89502=CARTESIAN_POINT('Ctrl Pts',(55.2805249392995,261.976023013032,20.9254564121947)) ;
#89503=CARTESIAN_POINT('Ctrl Pts',(55.2806454561434,261.976696777009,20.9259033002888)) ;
#89504=CARTESIAN_POINT('Ctrl Pts',(55.2807664959025,261.977369488772,20.9263494583211)) ;
#89505=CARTESIAN_POINT('Ctrl Pts',(55.2808880637497,261.978041207549,20.9267949212353)) ;
#89506=CARTESIAN_POINT('Ctrl Pts',(55.2819528718817,261.983924766677,20.9306967138914)) ;
#89507=CARTESIAN_POINT('Ctrl Pts',(55.2830575310507,261.989731884693,20.9345442358035)) ;
#89508=CARTESIAN_POINT('Ctrl Pts',(55.2842204372246,261.995563383192,20.9384046930442)) ;
#89509=CARTESIAN_POINT('Ctrl Pts',(55.2852766754412,262.000859985544,20.9419110485546)) ;
#89510=CARTESIAN_POINT('Ctrl Pts',(55.2863822704946,262.00618208714,20.9454316325777)) ;
#89511=CARTESIAN_POINT('Ctrl Pts',(55.2875502546595,262.011577672918,20.948997216028)) ;
#89512=CARTESIAN_POINT('Ctrl Pts',(55.288614318678,262.016493192202,20.9522455554906)) ;
#89513=CARTESIAN_POINT('Ctrl Pts',(55.2897303147452,262.021469464214,20.9555310700184)) ;
#89514=CARTESIAN_POINT('Ctrl Pts',(55.2909026141373,262.026510521406,20.9588549641176)) ;
#89515=CARTESIAN_POINT('Ctrl Pts',(55.2910848557811,262.027294186871,20.9593716852969)) ;
#89516=CARTESIAN_POINT('Ctrl Pts',(55.2912684588985,262.028079417904,20.9598893337448)) ;
#89517=CARTESIAN_POINT('Ctrl Pts',(55.2914534398696,262.028866226384,20.960407918366)) ;
#89518=CARTESIAN_POINT('Ctrl Pts',(55.2929248551374,262.035124826947,20.9645329552543)) ;
#89519=CARTESIAN_POINT('Ctrl Pts',(55.2944836292958,262.041482818636,20.9687171431804)) ;
#89520=CARTESIAN_POINT('Ctrl Pts',(55.296124351784,262.047894905047,20.9729342442153)) ;
#89521=CARTESIAN_POINT('Ctrl Pts',(55.2979374574581,262.054980679965,20.9775944167121)) ;
#89522=CARTESIAN_POINT('Ctrl Pts',(55.2998509444912,262.062131742623,20.9822943552114)) ;
#89523=CARTESIAN_POINT('Ctrl Pts',(55.3018372142892,262.069236566269,20.9869636166808)) ;
#89524=CARTESIAN_POINT('Ctrl Pts',(55.30253052279,262.071716508639,20.9885934248127)) ;
#89525=CARTESIAN_POINT('Ctrl Pts',(55.3032326176547,262.074190840947,20.9902192244433)) ;
#89526=CARTESIAN_POINT('Ctrl Pts',(55.3039416337351,262.076653487504,20.9918372019887)) ;
#89527=CARTESIAN_POINT('Ctrl Pts',(55.3058169380262,262.083167037455,20.9961166539192)) ;
#89528=CARTESIAN_POINT('Ctrl Pts',(55.3077412820762,262.089598675218,21.0003413330951)) ;
#89529=CARTESIAN_POINT('Ctrl Pts',(55.3096736304775,262.095837693835,21.0044415123092)) ;
#89530=CARTESIAN_POINT('Ctrl Pts',(55.3120993978905,262.103669825991,21.0095886592308)) ;
#89531=CARTESIAN_POINT('Ctrl Pts',(55.3145368697036,262.111194113669,21.014537052505)) ;
#89532=CARTESIAN_POINT('Ctrl Pts',(55.3168878208236,262.118199499406,21.0191481320322)) ;
#89533=CARTESIAN_POINT('Ctrl Pts',(55.3178189202186,262.120973997934,21.0209743602858)) ;
#89534=CARTESIAN_POINT('Ctrl Pts',(55.3187365177371,262.123667968671,21.0227460251729)) ;
#89535=CARTESIAN_POINT('Ctrl Pts',(55.3196347281987,262.126270973828,21.0244576618027)) ;
#89536=CARTESIAN_POINT('Ctrl Pts',(55.3206354767496,262.129171133369,21.026364695789)) ;
#89537=CARTESIAN_POINT('Ctrl Pts',(55.3216121837815,262.131958428654,21.0281971101326)) ;
#89538=CARTESIAN_POINT('Ctrl Pts',(55.3225568950698,262.134619639904,21.0299450085362)) ;
#89539=CARTESIAN_POINT('Ctrl Pts',(55.3241929769073,262.139228412388,21.0329720760301)) ;
#89540=CARTESIAN_POINT('Ctrl Pts',(55.325732568719,262.143457850253,21.0357467867831)) ;
#89541=CARTESIAN_POINT('Ctrl Pts',(55.3271454351735,262.147273177299,21.0382438986209)) ;
#89542=CARTESIAN_POINT('Ctrl Pts',(55.3285114456696,262.15096197377,21.0406581968508)) ;
#89543=CARTESIAN_POINT('Ctrl Pts',(55.3297585882148,262.154263201759,21.0428126342237)) ;
#89544=CARTESIAN_POINT('Ctrl Pts',(55.330876560063,262.157186132183,21.0447119352508)) ;
#89545=CARTESIAN_POINT('Ctrl Pts',(55.3318939799478,262.159846170126,21.0464404104672)) ;
#89546=CARTESIAN_POINT('Ctrl Pts',(55.3328043988932,262.162192988628,21.0479576178318)) ;
#89547=CARTESIAN_POINT('Ctrl Pts',(55.3336172586244,262.164270659442,21.0492908720446)) ;
#89548=CARTESIAN_POINT('Ctrl Pts',(55.3344062793214,262.166287397645,21.0505850254241)) ;
#89549=CARTESIAN_POINT('Ctrl Pts',(55.3351032841592,262.168050305835,21.0517057696937)) ;
#89550=CARTESIAN_POINT('Ctrl Pts',(55.3357328885529,262.169632717654,21.0527075249679)) ;
#89551=CARTESIAN_POINT('Ctrl Pts',(55.3363397180733,262.171157888403,21.0536730434406)) ;
#89552=CARTESIAN_POINT('Ctrl Pts',(55.3368838676364,262.172515205813,21.0545279586057)) ;
#89553=CARTESIAN_POINT('Ctrl Pts',(55.3374067785918,262.173812572095,21.0553418454806)) ;
#89554=CARTESIAN_POINT('Ctrl Pts',(55.3376249049078,262.174353753581,21.0556813490688)) ;
#89555=CARTESIAN_POINT('Ctrl Pts',(55.3378395674669,262.174885007626,21.0560140030048)) ;
#89556=CARTESIAN_POINT('Ctrl Pts',(55.3380548194638,262.175416437892,21.0563461469212)) ;
#89557=CARTESIAN_POINT('Origin',(55.8014829417656,261.987708218946,21.0563461469212)) ;
#89558=CARTESIAN_POINT('Ctrl Pts',(55.5095145719656,261.79455482774,20.2277364888237)) ;
#89559=CARTESIAN_POINT('Ctrl Pts',(55.4626130754224,261.791323735734,20.2614221936152)) ;
#89560=CARTESIAN_POINT('Ctrl Pts',(55.3860532767111,261.781008579942,20.3361055438638)) ;
#89561=CARTESIAN_POINT('Ctrl Pts',(55.2919386084249,261.742010571783,20.5272717802442)) ;
#89562=CARTESIAN_POINT('Ctrl Pts',(55.2649157169606,261.69184073163,20.6679797590307)) ;
#89563=CARTESIAN_POINT('Ctrl Pts',(55.2649122781271,261.665580342705,20.7284379454282)) ;
#89564=CARTESIAN_POINT('Ctrl Pts',(55.5011311279772,261.779167461482,20.2255237051989)) ;
#89565=CARTESIAN_POINT('Ctrl Pts',(55.456175278049,261.775186015806,20.2587821206896)) ;
#89566=CARTESIAN_POINT('Ctrl Pts',(55.382237274109,261.763499950179,20.3326971182674)) ;
#89567=CARTESIAN_POINT('Ctrl Pts',(55.29093472858,261.721392635792,20.5208133734021)) ;
#89568=CARTESIAN_POINT('Ctrl Pts',(55.2649244698029,261.670189926701,20.6567721272306)) ;
#89569=CARTESIAN_POINT('Ctrl Pts',(55.2649145254694,261.643367433716,20.71572921566)) ;
#89570=CARTESIAN_POINT('Ctrl Pts',(55.4854302237238,261.746721466304,20.2213211965547)) ;
#89571=CARTESIAN_POINT('Ctrl Pts',(55.4440536435622,261.74140119116,20.2537866714569)) ;
#89572=CARTESIAN_POINT('Ctrl Pts',(55.3749045745113,261.727021754684,20.3263522718821)) ;
#89573=CARTESIAN_POINT('Ctrl Pts',(55.2887959933571,261.678997151227,20.5082350012948)) ;
#89574=CARTESIAN_POINT('Ctrl Pts',(55.2649030138605,261.626302482539,20.6346570484583)) ;
#89575=CARTESIAN_POINT('Ctrl Pts',(55.26490889801,261.59862630945,20.690861256424)) ;
#89576=CARTESIAN_POINT('Ctrl Pts',(55.4649411121345,261.691374789118,20.2150379267643)) ;
#89577=CARTESIAN_POINT('Ctrl Pts',(55.428041263659,261.684353823492,20.2464932932028)) ;
#89578=CARTESIAN_POINT('Ctrl Pts',(55.3646008444798,261.665909068801,20.3175416220631)) ;
#89579=CARTESIAN_POINT('Ctrl Pts',(55.2856017188784,261.610888438487,20.4888635693427)) ;
#89580=CARTESIAN_POINT('Ctrl Pts',(55.2649132810963,261.558540491237,20.6020448190387)) ;
#89581=CARTESIAN_POINT('Ctrl Pts',(55.2649116963883,261.530698564893,20.6550488940796)) ;
#89582=CARTESIAN_POINT('Ctrl Pts',(55.4472141017732,261.626342713257,20.2085985316935)) ;
#89583=CARTESIAN_POINT('Ctrl Pts',(55.413733637549,261.617728456411,20.2392888290324)) ;
#89584=CARTESIAN_POINT('Ctrl Pts',(55.3548941740118,261.595684496215,20.3093684675433)) ;
#89585=CARTESIAN_POINT('Ctrl Pts',(55.2825837342738,261.536726216894,20.4692014769607)) ;
#89586=CARTESIAN_POINT('Ctrl Pts',(55.2649106528737,261.487796504572,20.5717207979694)) ;
#89587=CARTESIAN_POINT('Ctrl Pts',(55.2649109321867,261.461146834667,20.6224699580307)) ;
#89588=CARTESIAN_POINT('Ctrl Pts',(55.4320883309197,261.54761255968,20.2014661968594)) ;
#89589=CARTESIAN_POINT('Ctrl Pts',(55.4011858995745,261.538027697824,20.2316047928881)) ;
#89590=CARTESIAN_POINT('Ctrl Pts',(55.3459211189135,261.513570807188,20.300979608063)) ;
#89591=CARTESIAN_POINT('Ctrl Pts',(55.280186364588,261.456674374888,20.4483155522099)) ;
#89592=CARTESIAN_POINT('Ctrl Pts',(55.2649110500436,261.414367237008,20.5433352405049)) ;
#89593=CARTESIAN_POINT('Ctrl Pts',(55.2649110664895,261.390495196763,20.5924091979401)) ;
#89594=CARTESIAN_POINT('Ctrl Pts',(55.4201855327187,261.451485192532,20.1924774356911)) ;
#89595=CARTESIAN_POINT('Ctrl Pts',(55.3910693268253,261.442295282441,20.2221606966266)) ;
#89596=CARTESIAN_POINT('Ctrl Pts',(55.338286157701,261.418483405646,20.2905621884509)) ;
#89597=CARTESIAN_POINT('Ctrl Pts',(55.2788123134952,261.372468306853,20.4254128007512)) ;
#89598=CARTESIAN_POINT('Ctrl Pts',(55.2649111022978,261.338665106617,20.5164805332069)) ;
#89599=CARTESIAN_POINT('Ctrl Pts',(55.2649110733168,261.319006701877,20.5643405753509)) ;
#89600=CARTESIAN_POINT('Ctrl Pts',(55.4127834941959,261.337382234005,20.1809091598321)) ;
#89601=CARTESIAN_POINT('Ctrl Pts',(55.3844119930881,261.330754075371,20.2102651168952)) ;
#89602=CARTESIAN_POINT('Ctrl Pts',(55.332911951351,261.313654500188,20.2776533346949)) ;
#89603=CARTESIAN_POINT('Ctrl Pts',(55.2783408443739,261.285115029417,20.4035536370883)) ;
#89604=CARTESIAN_POINT('Ctrl Pts',(55.2649110495544,261.259955288591,20.4941009157673)) ;
#89605=CARTESIAN_POINT('Ctrl Pts',(55.2649110604085,261.245647194609,20.5412687298936)) ;
#89606=CARTESIAN_POINT('Ctrl Pts',(55.4106967194038,261.2145920902,20.1714615566787)) ;
#89607=CARTESIAN_POINT('Ctrl Pts',(55.3817726165835,261.212391231516,20.201117086952)) ;
#89608=CARTESIAN_POINT('Ctrl Pts',(55.3298548129479,261.205827465748,20.2688848493694)) ;
#89609=CARTESIAN_POINT('Ctrl Pts',(55.2778619848215,261.193338034809,20.3908691572262)) ;
#89610=CARTESIAN_POINT('Ctrl Pts',(55.2649110678744,261.177942527005,20.4808836390622)) ;
#89611=CARTESIAN_POINT('Ctrl Pts',(55.2649110649601,261.170167353101,20.5266939931165)) ;
#89612=CARTESIAN_POINT('Ctrl Pts',(55.4113576734741,261.13534727522,20.1677669529664)) ;
#89613=CARTESIAN_POINT('Ctrl Pts',(55.3811470979398,261.134705739364,20.1979775285007)) ;
#89614=CARTESIAN_POINT('Ctrl Pts',(55.3280699815944,261.132719886408,20.2666239963843)) ;
#89615=CARTESIAN_POINT('Ctrl Pts',(55.2768787444733,261.127286640832,20.3883249095729)) ;
#89616=CARTESIAN_POINT('Ctrl Pts',(55.2649110640675,261.121858235112,20.4767780866077)) ;
#89617=CARTESIAN_POINT('Ctrl Pts',(55.2649110640675,261.119141720484,20.5213203435597)) ;
#89618=CARTESIAN_POINT('Ctrl Pts',(55.4113576734741,261.093548013806,20.1677669529664)) ;
#89619=CARTESIAN_POINT('Ctrl Pts',(55.3805043197369,261.093548013806,20.1986203067036)) ;
#89620=CARTESIAN_POINT('Ctrl Pts',(55.3269240548999,261.093548013806,20.2684476752798)) ;
#89621=CARTESIAN_POINT('Ctrl Pts',(55.276399501296,261.093548013806,20.3904247378231)) ;
#89622=CARTESIAN_POINT('Ctrl Pts',(55.2649110640673,261.093548013806,20.4776871122598)) ;
#89623=CARTESIAN_POINT('Ctrl Pts',(55.2649110640673,261.093548013806,20.5213203435596)) ;
#89624=CARTESIAN_POINT('',(55.4113576734741,261.093548013806,20.1677669529664)) ;
#89625=CARTESIAN_POINT('Ctrl Pts',(55.5095145719656,261.79455482774,20.2277364888237)) ;
#89626=CARTESIAN_POINT('Ctrl Pts',(55.5011311279772,261.779167461482,20.2255237051989)) ;
#89627=CARTESIAN_POINT('Ctrl Pts',(55.4854302237238,261.746721466304,20.2213211965547)) ;
#89628=CARTESIAN_POINT('Ctrl Pts',(55.4649411121345,261.691374789118,20.2150379267643)) ;
#89629=CARTESIAN_POINT('Ctrl Pts',(55.4472141017732,261.626342713257,20.2085985316935)) ;
#89630=CARTESIAN_POINT('Ctrl Pts',(55.4320883309197,261.54761255968,20.2014661968594)) ;
#89631=CARTESIAN_POINT('Ctrl Pts',(55.4201855327187,261.451485192532,20.1924774356911)) ;
#89632=CARTESIAN_POINT('Ctrl Pts',(55.4127834941959,261.337382234005,20.1809091598321)) ;
#89633=CARTESIAN_POINT('Ctrl Pts',(55.4106967194038,261.2145920902,20.1714615566787)) ;
#89634=CARTESIAN_POINT('Ctrl Pts',(55.4113576734741,261.13534727522,20.1677669529664)) ;
#89635=CARTESIAN_POINT('Ctrl Pts',(55.4113576734741,261.093548013806,20.1677669529664)) ;
#89636=CARTESIAN_POINT('',(55.2649110640674,261.093548013806,20.5213203435596)) ;
#89637=CARTESIAN_POINT('Origin',(55.7649110640674,261.093548013806,20.5213203435596)) ;
#89638=CARTESIAN_POINT('Ctrl Pts',(55.2649110640673,261.093548013806,20.5213203435596)) ;
#89639=CARTESIAN_POINT('Ctrl Pts',(55.2649110640673,261.095953574552,20.5213203435596)) ;
#89640=CARTESIAN_POINT('Ctrl Pts',(55.2649110641555,261.098363829073,20.5213210869593)) ;
#89641=CARTESIAN_POINT('Ctrl Pts',(55.2649110658753,261.100914479524,20.5213508933325)) ;
#89642=CARTESIAN_POINT('Ctrl Pts',(55.264911067669,261.103574764907,20.5213819808768)) ;
#89643=CARTESIAN_POINT('Ctrl Pts',(55.2649110708674,261.106387547156,20.5214446439697)) ;
#89644=CARTESIAN_POINT('Ctrl Pts',(55.2649110723512,261.109447355915,20.5215616301146)) ;
#89645=CARTESIAN_POINT('Ctrl Pts',(55.2649110739158,261.112673890933,20.5216849907304)) ;
#89646=CARTESIAN_POINT('Ctrl Pts',(55.2649110731951,261.116174814157,20.5218687043635)) ;
#89647=CARTESIAN_POINT('Ctrl Pts',(55.2649110711966,261.120000151541,20.5221299119106)) ;
#89648=CARTESIAN_POINT('Ctrl Pts',(55.2649110690495,261.12410979266,20.522410532721)) ;
#89649=CARTESIAN_POINT('Ctrl Pts',(55.2649110661775,261.128593453019,20.5227805212708)) ;
#89650=CARTESIAN_POINT('Ctrl Pts',(55.264911065038,261.133450022732,20.5232513519634)) ;
#89651=CARTESIAN_POINT('Ctrl Pts',(55.2649110637655,261.138872992704,20.5237770935586)) ;
#89652=CARTESIAN_POINT('Ctrl Pts',(55.2649110642511,261.144761660323,20.5244152470584)) ;
#89653=CARTESIAN_POINT('Ctrl Pts',(55.2649110642177,261.151044919855,20.5251897158003)) ;
#89654=CARTESIAN_POINT('Ctrl Pts',(55.2649110641858,261.157035609164,20.5259281226079)) ;
#89655=CARTESIAN_POINT('Ctrl Pts',(55.264911064118,261.163382857385,20.5267957767956)) ;
#89656=CARTESIAN_POINT('Ctrl Pts',(55.2649110639784,261.169990918531,20.5277797035235)) ;
#89657=CARTESIAN_POINT('Ctrl Pts',(55.2649110637722,261.179745146691,20.5292320880557)) ;
#89658=CARTESIAN_POINT('Ctrl Pts',(55.2649110633954,261.190066022824,20.5309359022516)) ;
#89659=CARTESIAN_POINT('Ctrl Pts',(55.2649110631044,261.200632533083,20.5329114013934)) ;
#89660=CARTESIAN_POINT('Ctrl Pts',(55.2649110630817,261.201457066028,20.5330655548542)) ;
#89661=CARTESIAN_POINT('Ctrl Pts',(55.2649110630596,261.202283112817,20.5332213503105)) ;
#89662=CARTESIAN_POINT('Ctrl Pts',(55.2649110630382,261.203110526522,20.5333787899727)) ;
#89663=CARTESIAN_POINT('Ctrl Pts',(55.2649110628502,261.210386142706,20.5347631887907)) ;
#89664=CARTESIAN_POINT('Ctrl Pts',(55.2649110626976,261.217766083194,20.5362748858767)) ;
#89665=CARTESIAN_POINT('Ctrl Pts',(55.2649110627707,261.225190406921,20.5379151796448)) ;
#89666=CARTESIAN_POINT('Ctrl Pts',(55.2649110628364,261.231859050926,20.5393885172316)) ;
#89667=CARTESIAN_POINT('Ctrl Pts',(55.2649110632121,261.238564598798,20.5409601923757)) ;
#89668=CARTESIAN_POINT('Ctrl Pts',(55.264911064521,261.245304154603,20.5426504023542)) ;
#89669=CARTESIAN_POINT('Ctrl Pts',(55.2649110645244,261.245322028108,20.542654884842)) ;
#89670=CARTESIAN_POINT('Ctrl Pts',(55.2649110645279,261.245339901851,20.5426593681642)) ;
#89671=CARTESIAN_POINT('Ctrl Pts',(55.2649110645314,261.245357775832,20.542663852321)) ;
#89672=CARTESIAN_POINT('Ctrl Pts',(55.2649110657567,261.251646693871,20.5442415922823)) ;
#89673=CARTESIAN_POINT('Ctrl Pts',(55.2649110678177,261.25796485254,20.5459225583356)) ;
#89674=CARTESIAN_POINT('Ctrl Pts',(55.2649110689405,261.264356178618,20.5477254079163)) ;
#89675=CARTESIAN_POINT('Ctrl Pts',(55.2649110702031,261.271542625449,20.5497525432083)) ;
#89676=CARTESIAN_POINT('Ctrl Pts',(55.2649110698206,261.278827235558,20.5519354804463)) ;
#89677=CARTESIAN_POINT('Ctrl Pts',(55.2649110692137,261.286323385524,20.5543065199875)) ;
#89678=CARTESIAN_POINT('Ctrl Pts',(55.2649110686365,261.293453221298,20.5565616939928)) ;
#89679=CARTESIAN_POINT('Ctrl Pts',(55.2649110688686,261.300774597955,20.5589870012318)) ;
#89680=CARTESIAN_POINT('Ctrl Pts',(55.2649110694204,261.308334792425,20.5615715880227)) ;
#89681=CARTESIAN_POINT('Ctrl Pts',(55.2649110696691,261.311741518433,20.5627362378311)) ;
#89682=CARTESIAN_POINT('Ctrl Pts',(55.2649110698818,261.315195489647,20.5639367060361)) ;
#89683=CARTESIAN_POINT('Ctrl Pts',(55.2649110700281,261.318695106674,20.5651727800032)) ;
#89684=CARTESIAN_POINT('Ctrl Pts',(55.2649110702299,261.323522550396,20.5668778458623)) ;
#89685=CARTESIAN_POINT('Ctrl Pts',(55.2649110703085,261.328436825461,20.5686506966079)) ;
#89686=CARTESIAN_POINT('Ctrl Pts',(55.2649110700846,261.333434936416,20.570490540775)) ;
#89687=CARTESIAN_POINT('Ctrl Pts',(55.2649110696552,261.343017284311,20.574017878811)) ;
#89688=CARTESIAN_POINT('Ctrl Pts',(55.264911068135,261.352905770516,20.5777922330151)) ;
#89689=CARTESIAN_POINT('Ctrl Pts',(55.2649110639489,261.363017322083,20.5817650271008)) ;
#89690=CARTESIAN_POINT('Ctrl Pts',(55.2649110602374,261.371982469125,20.5852874027631)) ;
#89691=CARTESIAN_POINT('Ctrl Pts',(55.264911054406,261.381123415544,20.5889627139288)) ;
#89692=CARTESIAN_POINT('Ctrl Pts',(55.2649110452715,261.39035843418,20.5927355771868)) ;
#89693=CARTESIAN_POINT('Ctrl Pts',(55.2649110415572,261.394113550621,20.5942696878808)) ;
#89694=CARTESIAN_POINT('Ctrl Pts',(55.2649110372937,261.397884266899,20.5958197960011)) ;
#89695=CARTESIAN_POINT('Ctrl Pts',(55.2649110331729,261.401664355739,20.5973841568064)) ;
#89696=CARTESIAN_POINT('Ctrl Pts',(55.2649110199599,261.413784923579,20.6024001609441)) ;
#89697=CARTESIAN_POINT('Ctrl Pts',(55.2649110079949,261.425990648584,20.6075720219529)) ;
#89698=CARTESIAN_POINT('Ctrl Pts',(55.2649110211286,261.438076897157,20.6128139199388)) ;
#89699=CARTESIAN_POINT('Ctrl Pts',(55.2649110294867,261.445768305083,20.6161497420901)) ;
#89700=CARTESIAN_POINT('Ctrl Pts',(55.2649110480021,261.453410324451,20.619513524549)) ;
#89701=CARTESIAN_POINT('Ctrl Pts',(55.2649110819384,261.460963759829,20.622889185544)) ;
#89702=CARTESIAN_POINT('Ctrl Pts',(55.2649110946635,261.463796083617,20.6241549625655)) ;
#89703=CARTESIAN_POINT('Ctrl Pts',(55.2649111095407,261.466615960681,20.6254223899507)) ;
#89704=CARTESIAN_POINT('Ctrl Pts',(55.2649111252154,261.469421281671,20.6266906002001)) ;
#89705=CARTESIAN_POINT('Ctrl Pts',(55.2649111755076,261.478422182194,20.6307596655011)) ;
#89706=CARTESIAN_POINT('Ctrl Pts',(55.2649112334233,261.487272197075,20.6348384842092)) ;
#89707=CARTESIAN_POINT('Ctrl Pts',(55.2649112590157,261.49594352396,20.6389157230749)) ;
#89708=CARTESIAN_POINT('Ctrl Pts',(55.2649112823866,261.503862131913,20.6426390351511)) ;
#89709=CARTESIAN_POINT('Ctrl Pts',(55.2649112790021,261.511631875597,20.6463603736446)) ;
#89710=CARTESIAN_POINT('Ctrl Pts',(55.2649112238241,261.519270955283,20.6500882567231)) ;
#89711=CARTESIAN_POINT('Ctrl Pts',(55.2649111967476,261.523019534116,20.6519175691757)) ;
#89712=CARTESIAN_POINT('Ctrl Pts',(55.2649111572818,261.526736725872,20.6537480972418)) ;
#89713=CARTESIAN_POINT('Ctrl Pts',(55.2649111026463,261.53042995632,20.6555838410976)) ;
#89714=CARTESIAN_POINT('Ctrl Pts',(55.2649110493035,261.534035797492,20.6573761475535)) ;
#89715=CARTESIAN_POINT('Ctrl Pts',(55.2649109815467,261.537618800964,20.6591734205906)) ;
#89716=CARTESIAN_POINT('Ctrl Pts',(55.2649109089552,261.541186632215,20.6609780166873)) ;
#89717=CARTESIAN_POINT('Ctrl Pts',(55.2649107770721,261.547668610221,20.6642565776356)) ;
#89718=CARTESIAN_POINT('Ctrl Pts',(55.2649106289493,261.55410517783,20.66756295349)) ;
#89719=CARTESIAN_POINT('Ctrl Pts',(55.2649105198908,261.560555098686,20.6709200241745)) ;
#89720=CARTESIAN_POINT('Ctrl Pts',(55.2649104085869,261.567137817086,20.6743462136518)) ;
#89721=CARTESIAN_POINT('Ctrl Pts',(55.2649103378208,261.573734394714,20.6778251286652)) ;
#89722=CARTESIAN_POINT('Ctrl Pts',(55.264910370993,261.580353065022,20.6813531377929)) ;
#89723=CARTESIAN_POINT('Ctrl Pts',(55.264910401248,261.586389691437,20.6845708948508)) ;
#89724=CARTESIAN_POINT('Ctrl Pts',(55.264910518443,261.592444179297,20.6878294094783)) ;
#89725=CARTESIAN_POINT('Ctrl Pts',(55.2649107712449,261.598491907439,20.6911062231953)) ;
#89726=CARTESIAN_POINT('Ctrl Pts',(55.2649108250096,261.599778107717,20.6918031193877)) ;
#89727=CARTESIAN_POINT('Ctrl Pts',(55.2649108848975,261.601064003873,20.6925008394558)) ;
#89728=CARTESIAN_POINT('Ctrl Pts',(55.2649109496009,261.602349332226,20.693199220935)) ;
#89729=CARTESIAN_POINT('Ctrl Pts',(55.2649114635442,261.612558765541,20.6987465031727)) ;
#89730=CARTESIAN_POINT('Ctrl Pts',(55.2649122753921,261.622729303273,20.7043377443707)) ;
#89731=CARTESIAN_POINT('Ctrl Pts',(55.264912743211,261.632628552867,20.7098463844237)) ;
#89732=CARTESIAN_POINT('Ctrl Pts',(55.2649131534803,261.641310030782,20.7146773705005)) ;
#89733=CARTESIAN_POINT('Ctrl Pts',(55.2649132915559,261.649777221039,20.7194414819695)) ;
#89734=CARTESIAN_POINT('Ctrl Pts',(55.2649128645567,261.657885102421,20.7240497636966)) ;
#89735=CARTESIAN_POINT('Ctrl Pts',(55.2649127275021,261.660487501128,20.7255288907142)) ;
#89736=CARTESIAN_POINT('Ctrl Pts',(55.2649125337714,261.663053367234,20.7269921815504)) ;
#89737=CARTESIAN_POINT('Ctrl Pts',(55.2649122782257,261.665579368428,20.7284373880131)) ;
#89738=CARTESIAN_POINT('Ctrl Pts',(55.5095145719656,261.79455482774,20.2277364888237)) ;
#89739=CARTESIAN_POINT('Ctrl Pts',(55.5011311279772,261.779167461482,20.2255237051989)) ;
#89740=CARTESIAN_POINT('Ctrl Pts',(55.4854302237238,261.746721466304,20.2213211965547)) ;
#89741=CARTESIAN_POINT('Ctrl Pts',(55.4649411121345,261.691374789118,20.2150379267643)) ;
#89742=CARTESIAN_POINT('Ctrl Pts',(55.4472141017732,261.626342713257,20.2085985316935)) ;
#89743=CARTESIAN_POINT('Ctrl Pts',(55.4320883309197,261.54761255968,20.2014661968594)) ;
#89744=CARTESIAN_POINT('Ctrl Pts',(55.4201855327187,261.451485192532,20.1924774356911)) ;
#89745=CARTESIAN_POINT('Ctrl Pts',(55.4127834941959,261.337382234005,20.1809091598321)) ;
#89746=CARTESIAN_POINT('Ctrl Pts',(55.4106967194038,261.2145920902,20.1714615566787)) ;
#89747=CARTESIAN_POINT('Ctrl Pts',(55.4113576734741,261.13534727522,20.1677669529664)) ;
#89748=CARTESIAN_POINT('Ctrl Pts',(55.4113576734741,261.093548013806,20.1677669529664)) ;
#89749=CARTESIAN_POINT('Ctrl Pts',(55.5340602178732,261.756752943059,20.1881500276994)) ;
#89750=CARTESIAN_POINT('Ctrl Pts',(55.525623721009,261.742330395001,20.1868005704375)) ;
#89751=CARTESIAN_POINT('Ctrl Pts',(55.5097976144326,261.711615750798,20.1840390520077)) ;
#89752=CARTESIAN_POINT('Ctrl Pts',(55.4892611883365,261.658349413846,20.1793261680185)) ;
#89753=CARTESIAN_POINT('Ctrl Pts',(55.4716399351109,261.594887926556,20.1742186050668)) ;
#89754=CARTESIAN_POINT('Ctrl Pts',(55.4570261046371,261.517912475163,20.1677768004166)) ;
#89755=CARTESIAN_POINT('Ctrl Pts',(55.4461750352641,261.4248025452,20.1591893941808)) ;
#89756=CARTESIAN_POINT('Ctrl Pts',(55.4403075481406,261.316741549714,20.1490460444848)) ;
#89757=CARTESIAN_POINT('Ctrl Pts',(55.4397672990167,261.203533325761,20.1411593374996)) ;
#89758=CARTESIAN_POINT('Ctrl Pts',(55.4415682490085,261.131344448697,20.137556377432)) ;
#89759=CARTESIAN_POINT('Ctrl Pts',(55.4422110272113,261.093548013806,20.1369135992292)) ;
#89760=CARTESIAN_POINT('Ctrl Pts',(55.5890667713761,261.688545713664,20.1225709708889)) ;
#89761=CARTESIAN_POINT('Ctrl Pts',(55.5804415216983,261.674930230812,20.1219461679195)) ;
#89762=CARTESIAN_POINT('Ctrl Pts',(55.5643715025921,261.645549687186,20.1205101639258)) ;
#89763=CARTESIAN_POINT('Ctrl Pts',(55.5440004208549,261.593366839832,20.1174753224289)) ;
#89764=CARTESIAN_POINT('Ctrl Pts',(55.5275077045974,261.53074866982,20.1128786169289)) ;
#89765=CARTESIAN_POINT('Ctrl Pts',(55.5149582126142,261.455358101747,20.1065866956058)) ;
#89766=CARTESIAN_POINT('Ctrl Pts',(55.507071095585,261.367892543992,20.0991563518021)) ;
#89767=CARTESIAN_POINT('Ctrl Pts',(55.5044282154051,261.273712249443,20.0923731576416)) ;
#89768=CARTESIAN_POINT('Ctrl Pts',(55.5065870370321,261.181367979666,20.0871845682348)) ;
#89769=CARTESIAN_POINT('Ctrl Pts',(55.5102147168921,261.123669597378,20.0844792610867)) ;
#89770=CARTESIAN_POINT('Ctrl Pts',(55.5120383957876,261.093548013806,20.0833333343921)) ;
#89771=CARTESIAN_POINT('Ctrl Pts',(55.735413453564,261.557876251656,20.0417117307531)) ;
#89772=CARTESIAN_POINT('Ctrl Pts',(55.7249293160056,261.543907787696,20.0414514566473)) ;
#89773=CARTESIAN_POINT('Ctrl Pts',(55.7054852264464,261.513984623845,20.0407144700406)) ;
#89774=CARTESIAN_POINT('Ctrl Pts',(55.6810670160264,261.463017852386,20.0390718220181)) ;
#89775=CARTESIAN_POINT('Ctrl Pts',(55.6607837910255,261.405540716534,20.037276875508)) ;
#89776=CARTESIAN_POINT('Ctrl Pts',(55.644455495605,261.342979538332,20.0357888764937)) ;
#89777=CARTESIAN_POINT('Ctrl Pts',(55.6330565896902,261.279282393762,20.0349679385755)) ;
#89778=CARTESIAN_POINT('Ctrl Pts',(55.6274098727185,261.216744008419,20.0346779991369)) ;
#89779=CARTESIAN_POINT('Ctrl Pts',(55.6277776422459,261.155243093917,20.0342048062941)) ;
#89780=CARTESIAN_POINT('Ctrl Pts',(55.6319156300806,261.114107180235,20.0332880239655)) ;
#89781=CARTESIAN_POINT('Ctrl Pts',(55.6340154583308,261.093548013806,20.0328087807883)) ;
#89782=CARTESIAN_POINT('Ctrl Pts',(55.8502255851785,261.475529765423,20.0213203435596)) ;
#89783=CARTESIAN_POINT('Ctrl Pts',(55.8372875489689,261.46314325178,20.0213203435596)) ;
#89784=CARTESIAN_POINT('Ctrl Pts',(55.8129913200325,261.436965535865,20.0213203435596)) ;
#89785=CARTESIAN_POINT('Ctrl Pts',(55.782270802112,261.393871982293,20.0213203435596)) ;
#89786=CARTESIAN_POINT('Ctrl Pts',(55.757059342802,261.346599890857,20.0213203435596)) ;
#89787=CARTESIAN_POINT('Ctrl Pts',(55.7377798655275,261.296394503685,20.0213203435596)) ;
#89788=CARTESIAN_POINT('Ctrl Pts',(55.7253576978104,261.245518369142,20.0213203435596)) ;
#89789=CARTESIAN_POINT('Ctrl Pts',(55.7194104036995,261.194000747696,20.0213203435596)) ;
#89790=CARTESIAN_POINT('Ctrl Pts',(55.7186325494572,261.142659830188,20.0213203435596)) ;
#89791=CARTESIAN_POINT('Ctrl Pts',(55.7203688071154,261.109892648291,20.0213203435596)) ;
#89792=CARTESIAN_POINT('Ctrl Pts',(55.7212778327675,261.093548013806,20.0213203435596)) ;
#89793=CARTESIAN_POINT('Ctrl Pts',(55.9002853073786,261.439128427997,20.0213203435596)) ;
#89794=CARTESIAN_POINT('Ctrl Pts',(55.8870982395572,261.427398724874,20.0213203435596)) ;
#89795=CARTESIAN_POINT('Ctrl Pts',(55.8624074372275,261.402653034435,20.0213203435596)) ;
#89796=CARTESIAN_POINT('Ctrl Pts',(55.8314994101313,261.362343578996,20.0213203435596)) ;
#89797=CARTESIAN_POINT('Ctrl Pts',(55.8063264068976,261.318668579119,20.0213203435596)) ;
#89798=CARTESIAN_POINT('Ctrl Pts',(55.7871994190772,261.273156234995,20.0213203435596)) ;
#89799=CARTESIAN_POINT('Ctrl Pts',(55.7746083733825,261.227740270089,20.0213203435596)) ;
#89800=CARTESIAN_POINT('Ctrl Pts',(55.7676584903403,261.18196002793,20.0213203435596)) ;
#89801=CARTESIAN_POINT('Ctrl Pts',(55.7649476045566,261.136640551767,20.0213203435596)) ;
#89802=CARTESIAN_POINT('Ctrl Pts',(55.7649110640674,261.107859578892,20.0213203435596)) ;
#89803=CARTESIAN_POINT('Ctrl Pts',(55.7649110640674,261.093548013806,20.0213203435596)) ;
#89804=CARTESIAN_POINT('',(55.9002853073786,261.439128427997,20.0213203435596)) ;
#89805=CARTESIAN_POINT('Ctrl Pts',(55.5095145719656,261.79455482774,20.2277364888237)) ;
#89806=CARTESIAN_POINT('Ctrl Pts',(55.5340602178732,261.756752943059,20.1881500276994)) ;
#89807=CARTESIAN_POINT('Ctrl Pts',(55.5890667713761,261.688545713664,20.1225709708889)) ;
#89808=CARTESIAN_POINT('Ctrl Pts',(55.735413453564,261.557876251656,20.0417117307531)) ;
#89809=CARTESIAN_POINT('Ctrl Pts',(55.8502255851785,261.475529765423,20.0213203435596)) ;
#89810=CARTESIAN_POINT('Ctrl Pts',(55.9002853073786,261.439128427997,20.0213203435596)) ;
#89811=CARTESIAN_POINT('',(55.7649110640674,261.093548013806,20.0213203435596)) ;
#89812=CARTESIAN_POINT('Ctrl Pts',(55.9002853073786,261.439128427997,20.0213203435596)) ;
#89813=CARTESIAN_POINT('Ctrl Pts',(55.8911225255332,261.430978268137,20.0213203435596)) ;
#89814=CARTESIAN_POINT('Ctrl Pts',(55.8823626842497,261.422515001751,20.0213203435599)) ;
#89815=CARTESIAN_POINT('Ctrl Pts',(55.8740745391944,261.413782365245,20.0213203435597)) ;
#89816=CARTESIAN_POINT('Ctrl Pts',(55.8704346856053,261.409947307084,20.0213203435596)) ;
#89817=CARTESIAN_POINT('Ctrl Pts',(55.8668841554711,261.40605928624,20.0213203435596)) ;
#89818=CARTESIAN_POINT('Ctrl Pts',(55.8634283117518,261.402121551956,20.0213203435599)) ;
#89819=CARTESIAN_POINT('Ctrl Pts',(55.8597986175688,261.397985725112,20.0213203435603)) ;
#89820=CARTESIAN_POINT('Ctrl Pts',(55.8562733770184,261.393795057419,20.0213203435611)) ;
#89821=CARTESIAN_POINT('Ctrl Pts',(55.8528506936904,261.389548714247,20.0213203435638)) ;
#89822=CARTESIAN_POINT('Ctrl Pts',(55.8459105310129,261.380938419465,20.0213203435691)) ;
#89823=CARTESIAN_POINT('Ctrl Pts',(55.8393976147825,261.372099983805,20.0213203435612)) ;
#89824=CARTESIAN_POINT('Ctrl Pts',(55.8332886371026,261.36302684571,20.0213203435601)) ;
#89825=CARTESIAN_POINT('Ctrl Pts',(55.8330098051664,261.362612720664,20.0213203435601)) ;
#89826=CARTESIAN_POINT('Ctrl Pts',(55.8327318195274,261.362198112044,20.02132034356)) ;
#89827=CARTESIAN_POINT('Ctrl Pts',(55.8324546776944,261.361783017971,20.02132034356)) ;
#89828=CARTESIAN_POINT('Ctrl Pts',(55.8266846684896,261.353140884826,20.0213203435592)) ;
#89829=CARTESIAN_POINT('Ctrl Pts',(55.8212801248487,261.34428846144,20.0213203435596)) ;
#89830=CARTESIAN_POINT('Ctrl Pts',(55.816247995365,261.335274645693,20.0213203435596)) ;
#89831=CARTESIAN_POINT('Ctrl Pts',(55.8131313863721,261.329692011281,20.0213203435596)) ;
#89832=CARTESIAN_POINT('Ctrl Pts',(55.8101586733848,261.324049540243,20.0213203435596)) ;
#89833=CARTESIAN_POINT('Ctrl Pts',(55.8073336503441,261.318362594802,20.0213203435598)) ;
#89834=CARTESIAN_POINT('Ctrl Pts',(55.8037773390003,261.311203520949,20.0213203435601)) ;
#89835=CARTESIAN_POINT('Ctrl Pts',(55.8004550995969,261.303973971199,20.0213203435606)) ;
#89836=CARTESIAN_POINT('Ctrl Pts',(55.797377237718,261.296712332345,20.0213203435605)) ;
#89837=CARTESIAN_POINT('Ctrl Pts',(55.7940628302853,261.288892608544,20.0213203435603)) ;
#89838=CARTESIAN_POINT('Ctrl Pts',(55.7910310881517,261.281034638102,20.0213203435596)) ;
#89839=CARTESIAN_POINT('Ctrl Pts',(55.7882882555811,261.27317252627,20.0213203435598)) ;
#89840=CARTESIAN_POINT('Ctrl Pts',(55.7878705140813,261.271975103423,20.0213203435599)) ;
#89841=CARTESIAN_POINT('Ctrl Pts',(55.7874594806918,261.270777584212,20.0213203435599)) ;
#89842=CARTESIAN_POINT('Ctrl Pts',(55.7870550706068,261.26957989208,20.0213203435601)) ;
#89843=CARTESIAN_POINT('Ctrl Pts',(55.7842121766762,261.261160439104,20.0213203435609)) ;
#89844=CARTESIAN_POINT('Ctrl Pts',(55.7816995351282,261.252741436658,20.0213203435728)) ;
#89845=CARTESIAN_POINT('Ctrl Pts',(55.7795007628783,261.244326782953,20.0213203435689)) ;
#89846=CARTESIAN_POINT('Ctrl Pts',(55.7780513827448,261.238780036622,20.0213203435663)) ;
#89847=CARTESIAN_POINT('Ctrl Pts',(55.7767370713497,261.233234004934,20.0213203435613)) ;
#89848=CARTESIAN_POINT('Ctrl Pts',(55.7755477954306,261.227679835847,20.0213203435602)) ;
#89849=CARTESIAN_POINT('Ctrl Pts',(55.7748608844637,261.224471816921,20.0213203435595)) ;
#89850=CARTESIAN_POINT('Ctrl Pts',(55.7742157070453,261.221261079339,20.0213203435596)) ;
#89851=CARTESIAN_POINT('Ctrl Pts',(55.7736096920963,261.218047898293,20.0213203435596)) ;
#89852=CARTESIAN_POINT('Ctrl Pts',(55.7717399027023,261.2081339979,20.0213203435596)) ;
#89853=CARTESIAN_POINT('Ctrl Pts',(55.7702454216534,261.19819023561,20.0213203435596)) ;
#89854=CARTESIAN_POINT('Ctrl Pts',(55.7690653662697,261.188266727098,20.0213203435596)) ;
#89855=CARTESIAN_POINT('Ctrl Pts',(55.7688182504891,261.186188641962,20.0213203435596)) ;
#89856=CARTESIAN_POINT('Ctrl Pts',(55.7685848703948,261.184111917233,20.0213203435596)) ;
#89857=CARTESIAN_POINT('Ctrl Pts',(55.7683646635995,261.182036903631,20.0213203435597)) ;
#89858=CARTESIAN_POINT('Ctrl Pts',(55.76742212904,261.173155379204,20.0213203435601)) ;
#89859=CARTESIAN_POINT('Ctrl Pts',(55.7667209439631,261.164305165404,20.0213203435655)) ;
#89860=CARTESIAN_POINT('Ctrl Pts',(55.7662109000418,261.155542863057,20.021320343563)) ;
#89861=CARTESIAN_POINT('Ctrl Pts',(55.7658483474578,261.149314388948,20.0213203435611)) ;
#89862=CARTESIAN_POINT('Ctrl Pts',(55.765581273064,261.143128087237,20.0213203435599)) ;
#89863=CARTESIAN_POINT('Ctrl Pts',(55.7653895517551,261.136998650066,20.0213203435601)) ;
#89864=CARTESIAN_POINT('Ctrl Pts',(55.765319811409,261.134769012308,20.0213203435602)) ;
#89865=CARTESIAN_POINT('Ctrl Pts',(55.7652600481747,261.132546901807,20.0213203435604)) ;
#89866=CARTESIAN_POINT('Ctrl Pts',(55.7652087553039,261.130331096701,20.0213203435613)) ;
#89867=CARTESIAN_POINT('Ctrl Pts',(55.7650413523549,261.123099442408,20.0213203435642)) ;
#89868=CARTESIAN_POINT('Ctrl Pts',(55.7649659237062,261.1159466348,20.0213203435738)) ;
#89869=CARTESIAN_POINT('Ctrl Pts',(55.7649342294194,261.108847738531,20.0213203435675)) ;
#89870=CARTESIAN_POINT('Ctrl Pts',(55.7649113765851,261.10372915356,20.0213203435629)) ;
#89871=CARTESIAN_POINT('Ctrl Pts',(55.7649110640674,261.098637903367,20.0213203435596)) ;
#89872=CARTESIAN_POINT('Ctrl Pts',(55.7649110640674,261.093548013806,20.0213203435596)) ;
#89873=CARTESIAN_POINT('Origin',(55.7649110640674,261.093548013806,20.5213203435596)) ;
#89874=CARTESIAN_POINT('Origin',(65.2229283731508,226.843027476095,16.0213203435596)) ;
#89875=CARTESIAN_POINT('',(65.2229283731508,226.843027476095,16.0213203435596)) ;
#89876=CARTESIAN_POINT('',(63.9568984489966,226.843027476095,16.0213203435596)) ;
#89877=CARTESIAN_POINT('',(67.6578947220605,226.843027476095,16.0213203435596)) ;
#89878=CARTESIAN_POINT('',(65.2229283731508,226.843027476095,16.3213203435596)) ;
#89879=CARTESIAN_POINT('',(65.2229283731508,226.843027476095,16.0213203435596)) ;
#89880=CARTESIAN_POINT('',(63.9568984489966,226.843027476095,16.3213203435596)) ;
#89881=CARTESIAN_POINT('',(65.2229283731508,226.843027476095,16.3213203435596)) ;
#89882=CARTESIAN_POINT('',(63.9568984489966,226.843027476095,16.0213203435596)) ;
#89883=CARTESIAN_POINT('Ctrl Pts',(65.8723144214678,227.025837901854,16.0213203435596)) ;
#89884=CARTESIAN_POINT('Ctrl Pts',(65.8723144214678,227.025837901854,16.3813203435596)) ;
#89885=CARTESIAN_POINT('Ctrl Pts',(65.7863625985753,226.972747188495,16.0213203435596)) ;
#89886=CARTESIAN_POINT('Ctrl Pts',(65.7863625985753,226.972747188495,16.3813203435596)) ;
#89887=CARTESIAN_POINT('Ctrl Pts',(65.5886928398511,226.850650551717,16.0213203435596)) ;
#89888=CARTESIAN_POINT('Ctrl Pts',(65.5886928398511,226.850650551717,16.3813203435596)) ;
#89889=CARTESIAN_POINT('Ctrl Pts',(65.3550036041292,226.845780120393,16.0213203435596)) ;
#89890=CARTESIAN_POINT('Ctrl Pts',(65.3550036041292,226.845780120393,16.3813203435596)) ;
#89891=CARTESIAN_POINT('Ctrl Pts',(65.2229283731508,226.843027476095,16.0213203435596)) ;
#89892=CARTESIAN_POINT('Ctrl Pts',(65.2229283731508,226.843027476095,16.3813203435596)) ;
#89893=CARTESIAN_POINT('',(65.8723144214678,227.025837901854,16.0213203435596)) ;
#89894=CARTESIAN_POINT('Ctrl Pts',(65.8723144214678,227.025837901854,16.0213203435596)) ;
#89895=CARTESIAN_POINT('Ctrl Pts',(65.7863625985753,226.972747188495,16.0213203435596)) ;
#89896=CARTESIAN_POINT('Ctrl Pts',(65.5886928398511,226.850650551717,16.0213203435596)) ;
#89897=CARTESIAN_POINT('Ctrl Pts',(65.3550036041292,226.845780120393,16.0213203435596)) ;
#89898=CARTESIAN_POINT('Ctrl Pts',(65.2229283731508,226.843027476095,16.0213203435596)) ;
#89899=CARTESIAN_POINT('',(65.8723144214678,227.025837901854,16.3213203435596)) ;
#89900=CARTESIAN_POINT('',(65.8723144214678,227.025837901854,16.0213203435596)) ;
#89901=CARTESIAN_POINT('Ctrl Pts',(65.8723144214678,227.025837901854,16.3213203435596)) ;
#89902=CARTESIAN_POINT('Ctrl Pts',(65.7863625985753,226.972747188495,16.3213203435596)) ;
#89903=CARTESIAN_POINT('Ctrl Pts',(65.5886928398511,226.850650551717,16.3213203435596)) ;
#89904=CARTESIAN_POINT('Ctrl Pts',(65.3550036041292,226.845780120393,16.3213203435596)) ;
#89905=CARTESIAN_POINT('Ctrl Pts',(65.2229283731508,226.843027476095,16.3213203435596)) ;
#89906=CARTESIAN_POINT('Ctrl Pts',(66.0796813648272,227.492413524412,16.0213203435596)) ;
#89907=CARTESIAN_POINT('Ctrl Pts',(66.0796813648272,227.492413524412,16.3813203435596)) ;
#89908=CARTESIAN_POINT('Ctrl Pts',(66.0713027278811,227.402263576791,16.0213203435596)) ;
#89909=CARTESIAN_POINT('Ctrl Pts',(66.0713027278811,227.402263576791,16.3813203435596)) ;
#89910=CARTESIAN_POINT('Ctrl Pts',(66.0546699670268,227.22330337963,16.0213203435596)) ;
#89911=CARTESIAN_POINT('Ctrl Pts',(66.0546699670268,227.22330337963,16.3813203435596)) ;
#89912=CARTESIAN_POINT('Ctrl Pts',(65.9327954854,227.091330410728,16.0213203435596)) ;
#89913=CARTESIAN_POINT('Ctrl Pts',(65.9327954854,227.091330410728,16.3813203435596)) ;
#89914=CARTESIAN_POINT('Ctrl Pts',(65.8723144214678,227.025837901854,16.0213203435596)) ;
#89915=CARTESIAN_POINT('Ctrl Pts',(65.8723144214678,227.025837901854,16.3813203435596)) ;
#89916=CARTESIAN_POINT('',(66.0796813648272,227.492413524412,16.0213203435596)) ;
#89917=CARTESIAN_POINT('Ctrl Pts',(66.0796813648272,227.492413524412,16.0213203435596)) ;
#89918=CARTESIAN_POINT('Ctrl Pts',(66.0713027278811,227.402263576791,16.0213203435596)) ;
#89919=CARTESIAN_POINT('Ctrl Pts',(66.0546699670268,227.22330337963,16.0213203435596)) ;
#89920=CARTESIAN_POINT('Ctrl Pts',(65.9327954854,227.091330410728,16.0213203435596)) ;
#89921=CARTESIAN_POINT('Ctrl Pts',(65.8723144214678,227.025837901854,16.0213203435596)) ;
#89922=CARTESIAN_POINT('',(66.0796813648272,227.492413524412,16.3213203435596)) ;
#89923=CARTESIAN_POINT('',(66.0796813648272,227.492413524412,16.0213203435596)) ;
#89924=CARTESIAN_POINT('Ctrl Pts',(66.0796813648272,227.492413524412,16.3213203435596)) ;
#89925=CARTESIAN_POINT('Ctrl Pts',(66.0713027278811,227.402263576791,16.3213203435596)) ;
#89926=CARTESIAN_POINT('Ctrl Pts',(66.0546699670268,227.22330337963,16.3213203435596)) ;
#89927=CARTESIAN_POINT('Ctrl Pts',(65.9327954854,227.091330410728,16.3213203435596)) ;
#89928=CARTESIAN_POINT('Ctrl Pts',(65.8723144214678,227.025837901854,16.3213203435596)) ;
#89929=CARTESIAN_POINT('Ctrl Pts',(65.9732694905329,227.852577272677,16.0213203435596)) ;
#89930=CARTESIAN_POINT('Ctrl Pts',(65.9732694905329,227.852577272677,16.3813203435596)) ;
#89931=CARTESIAN_POINT('Ctrl Pts',(66.0043061588733,227.796130023554,16.0213203435596)) ;
#89932=CARTESIAN_POINT('Ctrl Pts',(66.0043061588733,227.796130023554,16.3813203435596)) ;
#89933=CARTESIAN_POINT('Ctrl Pts',(66.0660587532603,227.68381886821,16.0213203435596)) ;
#89934=CARTESIAN_POINT('Ctrl Pts',(66.0660587532603,227.68381886821,16.3813203435596)) ;
#89935=CARTESIAN_POINT('Ctrl Pts',(66.0751562450622,227.555993998691,16.0213203435596)) ;
#89936=CARTESIAN_POINT('Ctrl Pts',(66.0751562450622,227.555993998691,16.3813203435596)) ;
#89937=CARTESIAN_POINT('Ctrl Pts',(66.0796813648272,227.492413524412,16.0213203435596)) ;
#89938=CARTESIAN_POINT('Ctrl Pts',(66.0796813648272,227.492413524412,16.3813203435596)) ;
#89939=CARTESIAN_POINT('',(65.9732694905329,227.852577272677,16.0213203435596)) ;
#89940=CARTESIAN_POINT('Ctrl Pts',(65.9732694905329,227.852577272677,16.0213203435596)) ;
#89941=CARTESIAN_POINT('Ctrl Pts',(66.0043061588733,227.796130023554,16.0213203435596)) ;
#89942=CARTESIAN_POINT('Ctrl Pts',(66.0660587532603,227.68381886821,16.0213203435596)) ;
#89943=CARTESIAN_POINT('Ctrl Pts',(66.0751562450622,227.555993998691,16.0213203435596)) ;
#89944=CARTESIAN_POINT('Ctrl Pts',(66.0796813648272,227.492413524412,16.0213203435596)) ;
#89945=CARTESIAN_POINT('',(65.9732694905329,227.852577272677,16.3213203435596)) ;
#89946=CARTESIAN_POINT('',(65.9732694905329,227.852577272677,16.0213203435596)) ;
#89947=CARTESIAN_POINT('Ctrl Pts',(65.9732694905329,227.852577272677,16.3213203435596)) ;
#89948=CARTESIAN_POINT('Ctrl Pts',(66.0043061588733,227.796130023554,16.3213203435596)) ;
#89949=CARTESIAN_POINT('Ctrl Pts',(66.0660587532603,227.68381886821,16.3213203435596)) ;
#89950=CARTESIAN_POINT('Ctrl Pts',(66.0751562450622,227.555993998691,16.3213203435596)) ;
#89951=CARTESIAN_POINT('Ctrl Pts',(66.0796813648272,227.492413524412,16.3213203435596)) ;
#89952=CARTESIAN_POINT('Ctrl Pts',(65.6622190754938,228.092686537527,16.0213203435596)) ;
#89953=CARTESIAN_POINT('Ctrl Pts',(65.6622190754938,228.092686537527,16.3813203435596)) ;
#89954=CARTESIAN_POINT('Ctrl Pts',(65.7257617097583,228.064451825508,16.0213203435596)) ;
#89955=CARTESIAN_POINT('Ctrl Pts',(65.7257617097583,228.064451825508,16.3813203435596)) ;
#89956=CARTESIAN_POINT('Ctrl Pts',(65.8491174447405,228.009639592847,16.0213203435596)) ;
#89957=CARTESIAN_POINT('Ctrl Pts',(65.8491174447405,228.009639592847,16.3813203435596)) ;
#89958=CARTESIAN_POINT('Ctrl Pts',(65.932728102633,227.903865388034,16.0213203435596)) ;
#89959=CARTESIAN_POINT('Ctrl Pts',(65.932728102633,227.903865388034,16.3813203435596)) ;
#89960=CARTESIAN_POINT('Ctrl Pts',(65.9732694905329,227.852577272677,16.0213203435596)) ;
#89961=CARTESIAN_POINT('Ctrl Pts',(65.9732694905329,227.852577272677,16.3813203435596)) ;
#89962=CARTESIAN_POINT('',(65.6622190754938,228.092686537527,16.0213203435596)) ;
#89963=CARTESIAN_POINT('Ctrl Pts',(65.6622190754938,228.092686537527,16.0213203435596)) ;
#89964=CARTESIAN_POINT('Ctrl Pts',(65.7257617097583,228.064451825508,16.0213203435596)) ;
#89965=CARTESIAN_POINT('Ctrl Pts',(65.8491174447405,228.009639592847,16.0213203435596)) ;
#89966=CARTESIAN_POINT('Ctrl Pts',(65.932728102633,227.903865388034,16.0213203435596)) ;
#89967=CARTESIAN_POINT('Ctrl Pts',(65.9732694905329,227.852577272677,16.0213203435596)) ;
#89968=CARTESIAN_POINT('',(65.6622190754938,228.092686537527,16.3213203435596)) ;
#89969=CARTESIAN_POINT('',(65.6622190754938,228.092686537527,16.0213203435596)) ;
#89970=CARTESIAN_POINT('Ctrl Pts',(65.6622190754938,228.092686537527,16.3213203435596)) ;
#89971=CARTESIAN_POINT('Ctrl Pts',(65.7257617097583,228.064451825508,16.3213203435596)) ;
#89972=CARTESIAN_POINT('Ctrl Pts',(65.8491174447405,228.009639592847,16.3213203435596)) ;
#89973=CARTESIAN_POINT('Ctrl Pts',(65.932728102633,227.903865388034,16.3213203435596)) ;
#89974=CARTESIAN_POINT('Ctrl Pts',(65.9732694905329,227.852577272677,16.3213203435596)) ;
#89975=CARTESIAN_POINT('Ctrl Pts',(65.0946882348585,228.166356388354,16.0213203435596)) ;
#89976=CARTESIAN_POINT('Ctrl Pts',(65.0946882348585,228.166356388354,16.3813203435596)) ;
#89977=CARTESIAN_POINT('Ctrl Pts',(65.2031657201074,228.165203721958,16.0213203435596)) ;
#89978=CARTESIAN_POINT('Ctrl Pts',(65.2031657201074,228.165203721958,16.3813203435596)) ;
#89979=CARTESIAN_POINT('Ctrl Pts',(65.3955084524701,228.163159915324,16.0213203435596)) ;
#89980=CARTESIAN_POINT('Ctrl Pts',(65.3955084524701,228.163159915324,16.3813203435596)) ;
#89981=CARTESIAN_POINT('Ctrl Pts',(65.5812375182262,228.114084424928,16.0213203435596)) ;
#89982=CARTESIAN_POINT('Ctrl Pts',(65.5812375182262,228.114084424928,16.3813203435596)) ;
#89983=CARTESIAN_POINT('Ctrl Pts',(65.6622190754938,228.092686537527,16.0213203435596)) ;
#89984=CARTESIAN_POINT('Ctrl Pts',(65.6622190754938,228.092686537527,16.3813203435596)) ;
#89985=CARTESIAN_POINT('',(65.0946882348585,228.166356388354,16.0213203435596)) ;
#89986=CARTESIAN_POINT('Ctrl Pts',(65.0946882348585,228.166356388354,16.0213203435596)) ;
#89987=CARTESIAN_POINT('Ctrl Pts',(65.2031657201074,228.165203721958,16.0213203435596)) ;
#89988=CARTESIAN_POINT('Ctrl Pts',(65.3955084524701,228.163159915324,16.0213203435596)) ;
#89989=CARTESIAN_POINT('Ctrl Pts',(65.5812375182262,228.114084424928,16.0213203435596)) ;
#89990=CARTESIAN_POINT('Ctrl Pts',(65.6622190754938,228.092686537527,16.0213203435596)) ;
#89991=CARTESIAN_POINT('',(65.0946882348585,228.166356388354,16.3213203435596)) ;
#89992=CARTESIAN_POINT('',(65.0946882348585,228.166356388354,16.0213203435596)) ;
#89993=CARTESIAN_POINT('Ctrl Pts',(65.0946882348585,228.166356388354,16.3213203435596)) ;
#89994=CARTESIAN_POINT('Ctrl Pts',(65.2031657201074,228.165203721958,16.3213203435596)) ;
#89995=CARTESIAN_POINT('Ctrl Pts',(65.3955084524701,228.163159915324,16.3213203435596)) ;
#89996=CARTESIAN_POINT('Ctrl Pts',(65.5812375182262,228.114084424928,16.3213203435596)) ;
#89997=CARTESIAN_POINT('Ctrl Pts',(65.6622190754938,228.092686537527,16.3213203435596)) ;
#89998=CARTESIAN_POINT('Origin',(63.9568984489966,228.166356388354,16.0213203435596)) ;
#89999=CARTESIAN_POINT('',(63.9568984489966,228.166356388354,16.0213203435596)) ;
#90000=CARTESIAN_POINT('',(67.0248797599834,228.166356388354,16.0213203435596)) ;
#90001=CARTESIAN_POINT('',(63.9568984489966,228.166356388354,16.3213203435596)) ;
#90002=CARTESIAN_POINT('',(63.9568984489966,228.166356388354,16.0213203435596)) ;
#90003=CARTESIAN_POINT('',(63.9568984489966,228.166356388354,16.3213203435596)) ;
#90004=CARTESIAN_POINT('Origin',(63.9568984489966,226.843027476095,16.0213203435596)) ;
#90005=CARTESIAN_POINT('',(63.9568984489966,228.43789484464,16.0213203435596)) ;
#90006=CARTESIAN_POINT('',(63.9568984489966,226.843027476095,16.3213203435596)) ;
#90007=CARTESIAN_POINT('Origin',(63.9568984489966,228.624746505045,16.0213203435596)) ;
#90008=CARTESIAN_POINT('',(63.9568984489966,228.624746505045,16.0213203435596)) ;
#90009=CARTESIAN_POINT('',(63.9568984489966,230.401008430742,16.0213203435596)) ;
#90010=CARTESIAN_POINT('',(63.9568984489966,229.328754359115,16.0213203435596)) ;
#90011=CARTESIAN_POINT('',(63.9568984489966,228.624746505045,16.3213203435596)) ;
#90012=CARTESIAN_POINT('',(63.9568984489966,228.624746505045,16.0213203435596)) ;
#90013=CARTESIAN_POINT('',(63.9568984489966,230.401008430742,16.3213203435596)) ;
#90014=CARTESIAN_POINT('',(63.9568984489966,228.624746505045,16.3213203435596)) ;
#90015=CARTESIAN_POINT('',(63.9568984489966,230.401008430742,16.0213203435596)) ;
#90016=CARTESIAN_POINT('Origin',(64.5708137732077,228.624746505045,16.0213203435596)) ;
#90017=CARTESIAN_POINT('',(64.5708137732077,228.624746505045,16.0213203435596)) ;
#90018=CARTESIAN_POINT('',(67.3318374220889,228.624746505045,16.0213203435596)) ;
#90019=CARTESIAN_POINT('',(64.5708137732077,228.624746505045,16.3213203435596)) ;
#90020=CARTESIAN_POINT('',(64.5708137732077,228.624746505045,16.0213203435596)) ;
#90021=CARTESIAN_POINT('',(64.5708137732077,228.624746505045,16.3213203435596)) ;
#90022=CARTESIAN_POINT('Ctrl Pts',(64.8654931765127,228.643846217417,16.0213203435596)) ;
#90023=CARTESIAN_POINT('Ctrl Pts',(64.8654931765127,228.643846217417,16.3813203435596)) ;
#90024=CARTESIAN_POINT('Ctrl Pts',(64.8259848410755,228.638324287067,16.0213203435596)) ;
#90025=CARTESIAN_POINT('Ctrl Pts',(64.8259848410755,228.638324287067,16.3813203435596)) ;
#90026=CARTESIAN_POINT('Ctrl Pts',(64.7282957987508,228.624670659758,16.0213203435596)) ;
#90027=CARTESIAN_POINT('Ctrl Pts',(64.7282957987508,228.624670659758,16.3813203435596)) ;
#90028=CARTESIAN_POINT('Ctrl Pts',(64.6295962862642,228.624718194661,16.0213203435596)) ;
#90029=CARTESIAN_POINT('Ctrl Pts',(64.6295962862642,228.624718194661,16.3813203435596)) ;
#90030=CARTESIAN_POINT('Ctrl Pts',(64.5708137732077,228.624746505045,16.0213203435596)) ;
#90031=CARTESIAN_POINT('Ctrl Pts',(64.5708137732077,228.624746505045,16.3813203435596)) ;
#90032=CARTESIAN_POINT('',(64.8654931765127,228.643846217417,16.0213203435596)) ;
#90033=CARTESIAN_POINT('Ctrl Pts',(64.8654931765127,228.643846217417,16.0213203435596)) ;
#90034=CARTESIAN_POINT('Ctrl Pts',(64.8259848410755,228.638324287067,16.0213203435596)) ;
#90035=CARTESIAN_POINT('Ctrl Pts',(64.7282957987508,228.624670659758,16.0213203435596)) ;
#90036=CARTESIAN_POINT('Ctrl Pts',(64.6295962862642,228.624718194661,16.0213203435596)) ;
#90037=CARTESIAN_POINT('Ctrl Pts',(64.5708137732077,228.624746505045,16.0213203435596)) ;
#90038=CARTESIAN_POINT('',(64.8654931765127,228.643846217417,16.3213203435596)) ;
#90039=CARTESIAN_POINT('',(64.8654931765127,228.643846217417,16.0213203435596)) ;
#90040=CARTESIAN_POINT('Ctrl Pts',(64.8654931765127,228.643846217417,16.3213203435596)) ;
#90041=CARTESIAN_POINT('Ctrl Pts',(64.8259848410755,228.638324287067,16.3213203435596)) ;
#90042=CARTESIAN_POINT('Ctrl Pts',(64.7282957987508,228.624670659758,16.3213203435596)) ;
#90043=CARTESIAN_POINT('Ctrl Pts',(64.6295962862642,228.624718194661,16.3213203435596)) ;
#90044=CARTESIAN_POINT('Ctrl Pts',(64.5708137732077,228.624746505045,16.3213203435596)) ;
#90045=CARTESIAN_POINT('Ctrl Pts',(65.1056022923517,228.750258091711,16.0213203435596)) ;
#90046=CARTESIAN_POINT('Ctrl Pts',(65.1056022923517,228.750258091711,16.3813203435596)) ;
#90047=CARTESIAN_POINT('Ctrl Pts',(65.0668285289302,228.726864738102,16.0213203435596)) ;
#90048=CARTESIAN_POINT('Ctrl Pts',(65.0668285289302,228.726864738102,16.3813203435596)) ;
#90049=CARTESIAN_POINT('Ctrl Pts',(64.9912530832381,228.681267845533,16.0213203435596)) ;
#90050=CARTESIAN_POINT('Ctrl Pts',(64.9912530832381,228.681267845533,16.3813203435596)) ;
#90051=CARTESIAN_POINT('Ctrl Pts',(64.9066775012378,228.656101192188,16.0213203435596)) ;
#90052=CARTESIAN_POINT('Ctrl Pts',(64.9066775012378,228.656101192188,16.3813203435596)) ;
#90053=CARTESIAN_POINT('Ctrl Pts',(64.8654931765127,228.643846217417,16.0213203435596)) ;
#90054=CARTESIAN_POINT('Ctrl Pts',(64.8654931765127,228.643846217417,16.3813203435596)) ;
#90055=CARTESIAN_POINT('',(65.1056022923517,228.750258091711,16.0213203435596)) ;
#90056=CARTESIAN_POINT('Ctrl Pts',(65.1056022923517,228.750258091711,16.0213203435596)) ;
#90057=CARTESIAN_POINT('Ctrl Pts',(65.0668285289302,228.726864738102,16.0213203435596)) ;
#90058=CARTESIAN_POINT('Ctrl Pts',(64.9912530832381,228.681267845533,16.0213203435596)) ;
#90059=CARTESIAN_POINT('Ctrl Pts',(64.9066775012378,228.656101192188,16.0213203435596)) ;
#90060=CARTESIAN_POINT('Ctrl Pts',(64.8654931765127,228.643846217417,16.0213203435596)) ;
#90061=CARTESIAN_POINT('',(65.1056022923517,228.750258091711,16.3213203435596)) ;
#90062=CARTESIAN_POINT('',(65.1056022923517,228.750258091711,16.0213203435596)) ;
#90063=CARTESIAN_POINT('Ctrl Pts',(65.1056022923517,228.750258091711,16.3213203435596)) ;
#90064=CARTESIAN_POINT('Ctrl Pts',(65.0668285289302,228.726864738102,16.3213203435596)) ;
#90065=CARTESIAN_POINT('Ctrl Pts',(64.9912530832381,228.681267845533,16.3213203435596)) ;
#90066=CARTESIAN_POINT('Ctrl Pts',(64.9066775012378,228.656101192188,16.3213203435596)) ;
#90067=CARTESIAN_POINT('Ctrl Pts',(64.8654931765127,228.643846217417,16.3213203435596)) ;
#90068=CARTESIAN_POINT('Ctrl Pts',(65.3757251780558,229.017652574801,16.0213203435596)) ;
#90069=CARTESIAN_POINT('Ctrl Pts',(65.3757251780558,229.017652574801,16.3813203435596)) ;
#90070=CARTESIAN_POINT('Ctrl Pts',(65.3304906114513,228.961176354081,16.0213203435596)) ;
#90071=CARTESIAN_POINT('Ctrl Pts',(65.3304906114513,228.961176354081,16.3813203435596)) ;
#90072=CARTESIAN_POINT('Ctrl Pts',(65.2506597476853,228.861505995311,16.0213203435596)) ;
#90073=CARTESIAN_POINT('Ctrl Pts',(65.2506597476853,228.861505995311,16.3813203435596)) ;
#90074=CARTESIAN_POINT('Ctrl Pts',(65.1494594569405,228.783893161395,16.0213203435596)) ;
#90075=CARTESIAN_POINT('Ctrl Pts',(65.1494594569405,228.783893161395,16.3813203435596)) ;
#90076=CARTESIAN_POINT('Ctrl Pts',(65.1056022923517,228.750258091711,16.0213203435596)) ;
#90077=CARTESIAN_POINT('Ctrl Pts',(65.1056022923517,228.750258091711,16.3813203435596)) ;
#90078=CARTESIAN_POINT('',(65.3757251780558,229.017652574801,16.0213203435596)) ;
#90079=CARTESIAN_POINT('Ctrl Pts',(65.3757251780558,229.017652574801,16.0213203435596)) ;
#90080=CARTESIAN_POINT('Ctrl Pts',(65.3304906114513,228.961176354081,16.0213203435596)) ;
#90081=CARTESIAN_POINT('Ctrl Pts',(65.2506597476853,228.861505995311,16.0213203435596)) ;
#90082=CARTESIAN_POINT('Ctrl Pts',(65.1494594569405,228.783893161395,16.0213203435596)) ;
#90083=CARTESIAN_POINT('Ctrl Pts',(65.1056022923517,228.750258091711,16.0213203435596)) ;
#90084=CARTESIAN_POINT('',(65.3757251780558,229.017652574801,16.3213203435596)) ;
#90085=CARTESIAN_POINT('',(65.3757251780558,229.017652574801,16.0213203435596)) ;
#90086=CARTESIAN_POINT('Ctrl Pts',(65.3757251780558,229.017652574801,16.3213203435596)) ;
#90087=CARTESIAN_POINT('Ctrl Pts',(65.3304906114513,228.961176354081,16.3213203435596)) ;
#90088=CARTESIAN_POINT('Ctrl Pts',(65.2506597476853,228.861505995311,16.3213203435596)) ;
#90089=CARTESIAN_POINT('Ctrl Pts',(65.1494594569405,228.783893161395,16.3213203435596)) ;
#90090=CARTESIAN_POINT('Ctrl Pts',(65.1056022923517,228.750258091711,16.3213203435596)) ;
#90091=CARTESIAN_POINT('Ctrl Pts',(65.7577170413065,229.568811956667,16.0213203435596)) ;
#90092=CARTESIAN_POINT('Ctrl Pts',(65.7577170413065,229.568811956667,16.3813203435596)) ;
#90093=CARTESIAN_POINT('Ctrl Pts',(65.6885436027166,229.461938549579,16.0213203435596)) ;
#90094=CARTESIAN_POINT('Ctrl Pts',(65.6885436027166,229.461938549579,16.3813203435596)) ;
#90095=CARTESIAN_POINT('Ctrl Pts',(65.5670128336211,229.274172730444,16.0213203435596)) ;
#90096=CARTESIAN_POINT('Ctrl Pts',(65.5670128336211,229.274172730444,16.3813203435596)) ;
#90097=CARTESIAN_POINT('Ctrl Pts',(65.4333214772105,229.094890238569,16.0213203435596)) ;
#90098=CARTESIAN_POINT('Ctrl Pts',(65.4333214772105,229.094890238569,16.3813203435596)) ;
#90099=CARTESIAN_POINT('Ctrl Pts',(65.3757251780558,229.017652574801,16.0213203435596)) ;
#90100=CARTESIAN_POINT('Ctrl Pts',(65.3757251780558,229.017652574801,16.3813203435596)) ;
#90101=CARTESIAN_POINT('',(65.7577170413065,229.568811956667,16.0213203435596)) ;
#90102=CARTESIAN_POINT('Ctrl Pts',(65.7577170413065,229.568811956667,16.0213203435596)) ;
#90103=CARTESIAN_POINT('Ctrl Pts',(65.6885436027166,229.461938549579,16.0213203435596)) ;
#90104=CARTESIAN_POINT('Ctrl Pts',(65.5670128336211,229.274172730444,16.0213203435596)) ;
#90105=CARTESIAN_POINT('Ctrl Pts',(65.4333214772105,229.094890238569,16.0213203435596)) ;
#90106=CARTESIAN_POINT('Ctrl Pts',(65.3757251780558,229.017652574801,16.0213203435596)) ;
#90107=CARTESIAN_POINT('',(65.7577170413065,229.568811956667,16.3213203435596)) ;
#90108=CARTESIAN_POINT('',(65.7577170413065,229.568811956667,16.0213203435596)) ;
#90109=CARTESIAN_POINT('Ctrl Pts',(65.7577170413065,229.568811956667,16.3213203435596)) ;
#90110=CARTESIAN_POINT('Ctrl Pts',(65.6885436027166,229.461938549579,16.3213203435596)) ;
#90111=CARTESIAN_POINT('Ctrl Pts',(65.5670128336211,229.274172730444,16.3213203435596)) ;
#90112=CARTESIAN_POINT('Ctrl Pts',(65.4333214772105,229.094890238569,16.3213203435596)) ;
#90113=CARTESIAN_POINT('Ctrl Pts',(65.3757251780558,229.017652574801,16.3213203435596)) ;
#90114=CARTESIAN_POINT('Origin',(66.2870483081865,230.401008430742,16.0213203435596)) ;
#90115=CARTESIAN_POINT('',(66.2870483081865,230.401008430742,16.0213203435596)) ;
#90116=CARTESIAN_POINT('',(66.7517866175368,231.131654071021,16.0213203435596)) ;
#90117=CARTESIAN_POINT('',(66.2870483081865,230.401008430742,16.3213203435596)) ;
#90118=CARTESIAN_POINT('',(66.2870483081865,230.401008430742,16.0213203435596)) ;
#90119=CARTESIAN_POINT('',(66.2870483081865,230.401008430742,16.3213203435596)) ;
#90120=CARTESIAN_POINT('Origin',(66.9528056662607,230.401008430742,16.0213203435596)) ;
#90121=CARTESIAN_POINT('',(66.9528056662607,230.401008430742,16.0213203435596)) ;
#90122=CARTESIAN_POINT('',(68.5228333686155,230.401008430742,16.0213203435596)) ;
#90123=CARTESIAN_POINT('',(66.9528056662607,230.401008430742,16.3213203435596)) ;
#90124=CARTESIAN_POINT('',(66.9528056662607,230.401008430742,16.0213203435596)) ;
#90125=CARTESIAN_POINT('',(66.9528056662607,230.401008430742,16.3213203435596)) ;
#90126=CARTESIAN_POINT('Origin',(66.2570346873331,229.312331680082,16.0213203435596)) ;
#90127=CARTESIAN_POINT('',(66.2570346873331,229.312331680082,16.0213203435596)) ;
#90128=CARTESIAN_POINT('',(66.976676663234,230.438359513508,16.0213203435596)) ;
#90129=CARTESIAN_POINT('',(66.2570346873331,229.312331680082,16.3213203435596)) ;
#90130=CARTESIAN_POINT('',(66.2570346873331,229.312331680082,16.0213203435596)) ;
#90131=CARTESIAN_POINT('',(66.2570346873331,229.312331680082,16.3213203435596)) ;
#90132=CARTESIAN_POINT('Ctrl Pts',(65.8177442830134,228.780271712565,16.0213203435596)) ;
#90133=CARTESIAN_POINT('Ctrl Pts',(65.8177442830134,228.780271712565,16.3813203435596)) ;
#90134=CARTESIAN_POINT('Ctrl Pts',(65.8955297605029,228.857983910561,16.0213203435596)) ;
#90135=CARTESIAN_POINT('Ctrl Pts',(65.8955297605029,228.857983910561,16.3813203435596)) ;
#90136=CARTESIAN_POINT('Ctrl Pts',(66.0589351598689,229.021235370333,16.0213203435596)) ;
#90137=CARTESIAN_POINT('Ctrl Pts',(66.0589351598689,229.021235370333,16.3813203435596)) ;
#90138=CARTESIAN_POINT('Ctrl Pts',(66.1889240792206,229.212246904868,16.0213203435596)) ;
#90139=CARTESIAN_POINT('Ctrl Pts',(66.1889240792206,229.212246904868,16.3813203435596)) ;
#90140=CARTESIAN_POINT('Ctrl Pts',(66.2570346873331,229.312331680082,16.0213203435596)) ;
#90141=CARTESIAN_POINT('Ctrl Pts',(66.2570346873331,229.312331680082,16.3813203435596)) ;
#90142=CARTESIAN_POINT('',(65.8177442830134,228.780271712565,16.0213203435596)) ;
#90143=CARTESIAN_POINT('Ctrl Pts',(65.8177442830134,228.780271712565,16.0213203435596)) ;
#90144=CARTESIAN_POINT('Ctrl Pts',(65.8955297605029,228.857983910561,16.0213203435596)) ;
#90145=CARTESIAN_POINT('Ctrl Pts',(66.0589351598689,229.021235370333,16.0213203435596)) ;
#90146=CARTESIAN_POINT('Ctrl Pts',(66.1889240792206,229.212246904868,16.0213203435596)) ;
#90147=CARTESIAN_POINT('Ctrl Pts',(66.2570346873331,229.312331680082,16.0213203435596)) ;
#90148=CARTESIAN_POINT('',(65.8177442830134,228.780271712565,16.3213203435596)) ;
#90149=CARTESIAN_POINT('',(65.8177442830134,228.780271712565,16.0213203435596)) ;
#90150=CARTESIAN_POINT('Ctrl Pts',(65.8177442830134,228.780271712565,16.3213203435596)) ;
#90151=CARTESIAN_POINT('Ctrl Pts',(65.8955297605029,228.857983910561,16.3213203435596)) ;
#90152=CARTESIAN_POINT('Ctrl Pts',(66.0589351598689,229.021235370333,16.3213203435596)) ;
#90153=CARTESIAN_POINT('Ctrl Pts',(66.1889240792206,229.212246904868,16.3213203435596)) ;
#90154=CARTESIAN_POINT('Ctrl Pts',(66.2570346873331,229.312331680082,16.3213203435596)) ;
#90155=CARTESIAN_POINT('Ctrl Pts',(65.4985083621073,228.581090275072,16.0213203435596)) ;
#90156=CARTESIAN_POINT('Ctrl Pts',(65.4985083621073,228.581090275072,16.3813203435596)) ;
#90157=CARTESIAN_POINT('Ctrl Pts',(65.5615665458594,228.612247980149,16.0213203435596)) ;
#90158=CARTESIAN_POINT('Ctrl Pts',(65.5615665458594,228.612247980149,16.3813203435596)) ;
#90159=CARTESIAN_POINT('Ctrl Pts',(65.674655764364,228.668126540359,16.0213203435596)) ;
#90160=CARTESIAN_POINT('Ctrl Pts',(65.674655764364,228.668126540359,16.3813203435596)) ;
#90161=CARTESIAN_POINT('Ctrl Pts',(65.7738572333903,228.745875376758,16.0213203435596)) ;
#90162=CARTESIAN_POINT('Ctrl Pts',(65.7738572333903,228.745875376758,16.3813203435596)) ;
#90163=CARTESIAN_POINT('Ctrl Pts',(65.8177442830134,228.780271712565,16.0213203435596)) ;
#90164=CARTESIAN_POINT('Ctrl Pts',(65.8177442830134,228.780271712565,16.3813203435596)) ;
#90165=CARTESIAN_POINT('',(65.4985083621073,228.581090275072,16.0213203435596)) ;
#90166=CARTESIAN_POINT('Ctrl Pts',(65.4985083621073,228.581090275072,16.0213203435596)) ;
#90167=CARTESIAN_POINT('Ctrl Pts',(65.5615665458594,228.612247980149,16.0213203435596)) ;
#90168=CARTESIAN_POINT('Ctrl Pts',(65.674655764364,228.668126540359,16.0213203435596)) ;
#90169=CARTESIAN_POINT('Ctrl Pts',(65.7738572333903,228.745875376758,16.0213203435596)) ;
#90170=CARTESIAN_POINT('Ctrl Pts',(65.8177442830134,228.780271712565,16.0213203435596)) ;
#90171=CARTESIAN_POINT('',(65.4985083621073,228.581090275072,16.3213203435596)) ;
#90172=CARTESIAN_POINT('',(65.4985083621073,228.581090275072,16.0213203435596)) ;
#90173=CARTESIAN_POINT('Ctrl Pts',(65.4985083621073,228.581090275072,16.3213203435596)) ;
#90174=CARTESIAN_POINT('Ctrl Pts',(65.5615665458594,228.612247980149,16.3213203435596)) ;
#90175=CARTESIAN_POINT('Ctrl Pts',(65.674655764364,228.668126540359,16.3213203435596)) ;
#90176=CARTESIAN_POINT('Ctrl Pts',(65.7738572333903,228.745875376758,16.3213203435596)) ;
#90177=CARTESIAN_POINT('Ctrl Pts',(65.8177442830134,228.780271712565,16.3213203435596)) ;
#90178=CARTESIAN_POINT('Ctrl Pts',(66.3498042505312,228.210012618326,16.0213203435596)) ;
#90179=CARTESIAN_POINT('Ctrl Pts',(66.3498042505312,228.210012618326,16.3813203435596)) ;
#90180=CARTESIAN_POINT('Ctrl Pts',(66.2373969568096,228.299376555848,16.0213203435596)) ;
#90181=CARTESIAN_POINT('Ctrl Pts',(66.2373969568096,228.299376555848,16.3813203435596)) ;
#90182=CARTESIAN_POINT('Ctrl Pts',(65.9877534498724,228.497843452596,16.0213203435596)) ;
#90183=CARTESIAN_POINT('Ctrl Pts',(65.9877534498724,228.497843452596,16.3813203435596)) ;
#90184=CARTESIAN_POINT('Ctrl Pts',(65.6720562109134,228.551560480452,16.0213203435596)) ;
#90185=CARTESIAN_POINT('Ctrl Pts',(65.6720562109134,228.551560480452,16.3813203435596)) ;
#90186=CARTESIAN_POINT('Ctrl Pts',(65.4985083621073,228.581090275072,16.0213203435596)) ;
#90187=CARTESIAN_POINT('Ctrl Pts',(65.4985083621073,228.581090275072,16.3813203435596)) ;
#90188=CARTESIAN_POINT('',(66.3498042505312,228.210012618326,16.0213203435596)) ;
#90189=CARTESIAN_POINT('Ctrl Pts',(66.3498042505312,228.210012618326,16.0213203435596)) ;
#90190=CARTESIAN_POINT('Ctrl Pts',(66.2373969568096,228.299376555848,16.0213203435596)) ;
#90191=CARTESIAN_POINT('Ctrl Pts',(65.9877534498724,228.497843452596,16.0213203435596)) ;
#90192=CARTESIAN_POINT('Ctrl Pts',(65.6720562109134,228.551560480452,16.0213203435596)) ;
#90193=CARTESIAN_POINT('Ctrl Pts',(65.4985083621073,228.581090275072,16.0213203435596)) ;
#90194=CARTESIAN_POINT('',(66.3498042505312,228.210012618326,16.3213203435596)) ;
#90195=CARTESIAN_POINT('',(66.3498042505312,228.210012618326,16.0213203435596)) ;
#90196=CARTESIAN_POINT('Ctrl Pts',(66.3498042505312,228.210012618326,16.3213203435596)) ;
#90197=CARTESIAN_POINT('Ctrl Pts',(66.2373969568096,228.299376555848,16.3213203435596)) ;
#90198=CARTESIAN_POINT('Ctrl Pts',(65.9877534498724,228.497843452596,16.3213203435596)) ;
#90199=CARTESIAN_POINT('Ctrl Pts',(65.6720562109134,228.551560480452,16.3213203435596)) ;
#90200=CARTESIAN_POINT('Ctrl Pts',(65.4985083621073,228.581090275072,16.3213203435596)) ;
#90201=CARTESIAN_POINT('Ctrl Pts',(66.6253839414644,227.492413524412,16.0213203435596)) ;
#90202=CARTESIAN_POINT('Ctrl Pts',(66.6253839414644,227.492413524412,16.3813203435596)) ;
#90203=CARTESIAN_POINT('Ctrl Pts',(66.6146677208766,227.627904203831,16.0213203435596)) ;
#90204=CARTESIAN_POINT('Ctrl Pts',(66.6146677208766,227.627904203831,16.3813203435596)) ;
#90205=CARTESIAN_POINT('Ctrl Pts',(66.5935785953528,227.894544846597,16.0213203435596)) ;
#90206=CARTESIAN_POINT('Ctrl Pts',(66.5935785953528,227.894544846597,16.3813203435596)) ;
#90207=CARTESIAN_POINT('Ctrl Pts',(66.4301756718191,228.106004162461,16.0213203435596)) ;
#90208=CARTESIAN_POINT('Ctrl Pts',(66.4301756718191,228.106004162461,16.3813203435596)) ;
#90209=CARTESIAN_POINT('Ctrl Pts',(66.3498042505312,228.210012618326,16.0213203435596)) ;
#90210=CARTESIAN_POINT('Ctrl Pts',(66.3498042505312,228.210012618326,16.3813203435596)) ;
#90211=CARTESIAN_POINT('',(66.6253839414644,227.492413524412,16.0213203435596)) ;
#90212=CARTESIAN_POINT('Ctrl Pts',(66.6253839414644,227.492413524412,16.0213203435596)) ;
#90213=CARTESIAN_POINT('Ctrl Pts',(66.6146677208766,227.627904203831,16.0213203435596)) ;
#90214=CARTESIAN_POINT('Ctrl Pts',(66.5935785953528,227.894544846597,16.0213203435596)) ;
#90215=CARTESIAN_POINT('Ctrl Pts',(66.4301756718191,228.106004162461,16.0213203435596)) ;
#90216=CARTESIAN_POINT('Ctrl Pts',(66.3498042505312,228.210012618326,16.0213203435596)) ;
#90217=CARTESIAN_POINT('',(66.6253839414644,227.492413524412,16.3213203435596)) ;
#90218=CARTESIAN_POINT('',(66.6253839414644,227.492413524412,16.0213203435596)) ;
#90219=CARTESIAN_POINT('Ctrl Pts',(66.6253839414644,227.492413524412,16.3213203435596)) ;
#90220=CARTESIAN_POINT('Ctrl Pts',(66.6146677208766,227.627904203831,16.3213203435596)) ;
#90221=CARTESIAN_POINT('Ctrl Pts',(66.5935785953528,227.894544846597,16.3213203435596)) ;
#90222=CARTESIAN_POINT('Ctrl Pts',(66.4301756718191,228.106004162461,16.3213203435596)) ;
#90223=CARTESIAN_POINT('Ctrl Pts',(66.3498042505312,228.210012618326,16.3213203435596)) ;
#90224=CARTESIAN_POINT('Ctrl Pts',(66.4589448254633,226.889412406706,16.0213203435596)) ;
#90225=CARTESIAN_POINT('Ctrl Pts',(66.4589448254633,226.889412406706,16.3813203435596)) ;
#90226=CARTESIAN_POINT('Ctrl Pts',(66.5074885919051,226.983214870015,16.0213203435596)) ;
#90227=CARTESIAN_POINT('Ctrl Pts',(66.5074885919051,226.983214870015,16.3813203435596)) ;
#90228=CARTESIAN_POINT('Ctrl Pts',(66.605416512552,227.172443701166,16.0213203435596)) ;
#90229=CARTESIAN_POINT('Ctrl Pts',(66.605416512552,227.172443701166,16.3813203435596)) ;
#90230=CARTESIAN_POINT('Ctrl Pts',(66.6186901616811,227.385148460716,16.0213203435596)) ;
#90231=CARTESIAN_POINT('Ctrl Pts',(66.6186901616811,227.385148460716,16.3813203435596)) ;
#90232=CARTESIAN_POINT('Ctrl Pts',(66.6253839414644,227.492413524412,16.0213203435596)) ;
#90233=CARTESIAN_POINT('Ctrl Pts',(66.6253839414644,227.492413524412,16.3813203435596)) ;
#90234=CARTESIAN_POINT('',(66.4589448254633,226.889412406706,16.0213203435596)) ;
#90235=CARTESIAN_POINT('Ctrl Pts',(66.4589448254633,226.889412406706,16.0213203435596)) ;
#90236=CARTESIAN_POINT('Ctrl Pts',(66.5074885919051,226.983214870015,16.0213203435596)) ;
#90237=CARTESIAN_POINT('Ctrl Pts',(66.605416512552,227.172443701166,16.0213203435596)) ;
#90238=CARTESIAN_POINT('Ctrl Pts',(66.6186901616811,227.385148460716,16.0213203435596)) ;
#90239=CARTESIAN_POINT('Ctrl Pts',(66.6253839414644,227.492413524412,16.0213203435596)) ;
#90240=CARTESIAN_POINT('',(66.4589448254633,226.889412406706,16.3213203435596)) ;
#90241=CARTESIAN_POINT('',(66.4589448254633,226.889412406706,16.0213203435596)) ;
#90242=CARTESIAN_POINT('Ctrl Pts',(66.4589448254633,226.889412406706,16.3213203435596)) ;
#90243=CARTESIAN_POINT('Ctrl Pts',(66.5074885919051,226.983214870015,16.3213203435596)) ;
#90244=CARTESIAN_POINT('Ctrl Pts',(66.605416512552,227.172443701166,16.3213203435596)) ;
#90245=CARTESIAN_POINT('Ctrl Pts',(66.6186901616811,227.385148460716,16.3213203435596)) ;
#90246=CARTESIAN_POINT('Ctrl Pts',(66.6253839414644,227.492413524412,16.3213203435596)) ;
#90247=CARTESIAN_POINT('Ctrl Pts',(66.0141970198679,226.51014894607,16.0213203435596)) ;
#90248=CARTESIAN_POINT('Ctrl Pts',(66.0141970198679,226.51014894607,16.3813203435596)) ;
#90249=CARTESIAN_POINT('Ctrl Pts',(66.1028098485333,226.553391987607,16.0213203435596)) ;
#90250=CARTESIAN_POINT('Ctrl Pts',(66.1028098485333,226.553391987607,16.3813203435596)) ;
#90251=CARTESIAN_POINT('Ctrl Pts',(66.2834709021064,226.641554543316,16.0213203435596)) ;
#90252=CARTESIAN_POINT('Ctrl Pts',(66.2834709021064,226.641554543316,16.3813203435596)) ;
#90253=CARTESIAN_POINT('Ctrl Pts',(66.3997166860594,226.805752340273,16.0213203435596)) ;
#90254=CARTESIAN_POINT('Ctrl Pts',(66.3997166860594,226.805752340273,16.3813203435596)) ;
#90255=CARTESIAN_POINT('Ctrl Pts',(66.4589448254633,226.889412406706,16.0213203435596)) ;
#90256=CARTESIAN_POINT('Ctrl Pts',(66.4589448254633,226.889412406706,16.3813203435596)) ;
#90257=CARTESIAN_POINT('',(66.0141970198679,226.51014894607,16.0213203435596)) ;
#90258=CARTESIAN_POINT('Ctrl Pts',(66.0141970198679,226.51014894607,16.0213203435596)) ;
#90259=CARTESIAN_POINT('Ctrl Pts',(66.1028098485333,226.553391987607,16.0213203435596)) ;
#90260=CARTESIAN_POINT('Ctrl Pts',(66.2834709021064,226.641554543316,16.0213203435596)) ;
#90261=CARTESIAN_POINT('Ctrl Pts',(66.3997166860594,226.805752340273,16.0213203435596)) ;
#90262=CARTESIAN_POINT('Ctrl Pts',(66.4589448254633,226.889412406706,16.0213203435596)) ;
#90263=CARTESIAN_POINT('',(66.0141970198679,226.51014894607,16.3213203435596)) ;
#90264=CARTESIAN_POINT('',(66.0141970198679,226.51014894607,16.0213203435596)) ;
#90265=CARTESIAN_POINT('Ctrl Pts',(66.0141970198679,226.51014894607,16.3213203435596)) ;
#90266=CARTESIAN_POINT('Ctrl Pts',(66.1028098485333,226.553391987607,16.3213203435596)) ;
#90267=CARTESIAN_POINT('Ctrl Pts',(66.2834709021064,226.641554543316,16.3213203435596)) ;
#90268=CARTESIAN_POINT('Ctrl Pts',(66.3997166860594,226.805752340273,16.3213203435596)) ;
#90269=CARTESIAN_POINT('Ctrl Pts',(66.4589448254633,226.889412406706,16.3213203435596)) ;
#90270=CARTESIAN_POINT('Ctrl Pts',(65.2011002581644,226.401008371138,16.0213203435596)) ;
#90271=CARTESIAN_POINT('Ctrl Pts',(65.2011002581644,226.401008371138,16.3813203435596)) ;
#90272=CARTESIAN_POINT('Ctrl Pts',(65.3591469635349,226.402248397894,16.0213203435596)) ;
#90273=CARTESIAN_POINT('Ctrl Pts',(65.3591469635349,226.402248397894,16.3813203435596)) ;
#90274=CARTESIAN_POINT('Ctrl Pts',(65.6352198408299,226.404414452249,16.0213203435596)) ;
#90275=CARTESIAN_POINT('Ctrl Pts',(65.6352198408299,226.404414452249,16.3813203435596)) ;
#90276=CARTESIAN_POINT('Ctrl Pts',(65.9006995989094,226.47848320729,16.0213203435596)) ;
#90277=CARTESIAN_POINT('Ctrl Pts',(65.9006995989094,226.47848320729,16.3813203435596)) ;
#90278=CARTESIAN_POINT('Ctrl Pts',(66.0141970198679,226.51014894607,16.0213203435596)) ;
#90279=CARTESIAN_POINT('Ctrl Pts',(66.0141970198679,226.51014894607,16.3813203435596)) ;
#90280=CARTESIAN_POINT('',(65.2011002581644,226.401008371138,16.0213203435596)) ;
#90281=CARTESIAN_POINT('Ctrl Pts',(65.2011002581644,226.401008371138,16.0213203435596)) ;
#90282=CARTESIAN_POINT('Ctrl Pts',(65.3591469635349,226.402248397894,16.0213203435596)) ;
#90283=CARTESIAN_POINT('Ctrl Pts',(65.6352198408299,226.404414452249,16.0213203435596)) ;
#90284=CARTESIAN_POINT('Ctrl Pts',(65.9006995989094,226.47848320729,16.0213203435596)) ;
#90285=CARTESIAN_POINT('Ctrl Pts',(66.0141970198679,226.51014894607,16.0213203435596)) ;
#90286=CARTESIAN_POINT('',(65.2011002581644,226.401008371138,16.3213203435596)) ;
#90287=CARTESIAN_POINT('',(65.2011002581644,226.401008371138,16.0213203435596)) ;
#90288=CARTESIAN_POINT('Ctrl Pts',(65.2011002581644,226.401008371138,16.3213203435596)) ;
#90289=CARTESIAN_POINT('Ctrl Pts',(65.3591469635349,226.402248397894,16.3213203435596)) ;
#90290=CARTESIAN_POINT('Ctrl Pts',(65.6352198408299,226.404414452249,16.3213203435596)) ;
#90291=CARTESIAN_POINT('Ctrl Pts',(65.9006995989094,226.47848320729,16.3213203435596)) ;
#90292=CARTESIAN_POINT('Ctrl Pts',(66.0141970198679,226.51014894607,16.3213203435596)) ;
#90293=CARTESIAN_POINT('Origin',(63.4275669213462,226.401008371138,16.0213203435596)) ;
#90294=CARTESIAN_POINT('',(63.4275669213462,226.401008371138,16.0213203435596)) ;
#90295=CARTESIAN_POINT('',(66.7602139961582,226.401008371138,16.0213203435596)) ;
#90296=CARTESIAN_POINT('',(63.4275669213462,226.401008371138,16.3213203435596)) ;
#90297=CARTESIAN_POINT('',(63.4275669213462,226.401008371138,16.0213203435596)) ;
#90298=CARTESIAN_POINT('',(63.4275669213462,226.401008371138,16.3213203435596)) ;
#90299=CARTESIAN_POINT('Origin',(63.4275669213462,230.401008430742,16.0213203435596)) ;
#90300=CARTESIAN_POINT('',(63.4275669213462,230.401008430742,16.0213203435596)) ;
#90301=CARTESIAN_POINT('',(63.4275669213462,230.216885321963,16.0213203435596)) ;
#90302=CARTESIAN_POINT('',(63.4275669213462,230.401008430742,16.3213203435596)) ;
#90303=CARTESIAN_POINT('',(63.4275669213462,230.401008430742,16.0213203435596)) ;
#90304=CARTESIAN_POINT('',(63.4275669213462,230.401008430742,16.3213203435596)) ;
#90305=CARTESIAN_POINT('Origin',(63.9568984489966,230.401008430742,16.0213203435596)) ;
#90306=CARTESIAN_POINT('',(67.0248797599834,230.401008430742,16.0213203435596)) ;
#90307=CARTESIAN_POINT('',(63.9568984489966,230.401008430742,16.3213203435596)) ;
#90308=CARTESIAN_POINT('Origin',(65.1901862938035,228.40100840094,16.3213203435596)) ;
#90309=CARTESIAN_POINT('Origin',(70.0928610709702,230.032762213184,16.0213203435596)) ;
#90310=CARTESIAN_POINT('',(56.1573593128808,238.278291754874,16.0213203435596)) ;
#90311=CARTESIAN_POINT('',(56.1573593128808,226.261195155516,16.0213203435596)) ;
#90312=CARTESIAN_POINT('',(56.1573593128808,228.14697868435,16.0213203435596)) ;
#90313=CARTESIAN_POINT('',(68.4815231079478,238.278291754874,16.0213203435596)) ;
#90314=CARTESIAN_POINT('',(69.2696458032277,238.278291754874,16.0213203435596)) ;
#90315=CARTESIAN_POINT('',(80.5752025501715,238.278291754874,16.0213203435596)) ;
#90316=CARTESIAN_POINT('Origin',(74.5283628290597,239.4,16.0213203435596)) ;
#90317=CARTESIAN_POINT('',(81.3283036990481,238.278291755028,16.0213203435596)) ;
#90318=CARTESIAN_POINT('',(69.2696458032277,238.278291754874,16.0213203435596)) ;
#90319=CARTESIAN_POINT('',(81.1,237.60736287746,16.0213203435596)) ;
#90320=CARTESIAN_POINT('Origin',(82.2,237.60736287746,16.0213203435596)) ;
#90321=CARTESIAN_POINT('',(81.1,226.002365511524,16.0213203435596)) ;
#90322=CARTESIAN_POINT('',(81.1,234.318247777236,16.0213203435596)) ;
#90323=CARTESIAN_POINT('',(80.9535533905933,225.648812120931,16.0213203435596)) ;
#90324=CARTESIAN_POINT('Origin',(80.5999999999999,226.002365511524,16.0213203435596)) ;
#90325=CARTESIAN_POINT('',(80.1050252531694,224.800283983507,16.0213203435596)) ;
#90326=CARTESIAN_POINT('',(79.3343678337509,224.029626564088,16.0213203435596)) ;
#90327=CARTESIAN_POINT('',(80.0535626751402,224.742809236676,16.0213203435596)) ;
#90328=CARTESIAN_POINT('Origin',(80.6000000000002,224.305309236676,16.0213203435596)) ;
#90329=CARTESIAN_POINT('',(79.3510004003203,224.405309236676,16.0213203435596)) ;
#90330=CARTESIAN_POINT('Origin',(79.3510004003203,225.305309236676,16.0213203435596)) ;
#90331=CARTESIAN_POINT('',(75.,224.405309236676,16.0213203435596)) ;
#90332=CARTESIAN_POINT('',(75.046430535485,224.405309236676,16.0213203435596)) ;
#90333=CARTESIAN_POINT('',(70.8999999999999,220.305309236676,16.0213203435596)) ;
#90334=CARTESIAN_POINT('Origin',(74.9999999999998,220.305309236676,16.0213203435596)) ;
#90335=CARTESIAN_POINT('',(70.8999999999998,217.165524426368,16.0213203435596)) ;
#90336=CARTESIAN_POINT('',(70.9000000000001,225.16903572493,16.0213203435596)) ;
#90337=CARTESIAN_POINT('',(69.4079308494226,215.768555109772,16.0213203435596)) ;
#90338=CARTESIAN_POINT('Origin',(69.4999999999997,217.165524426368,16.0213203435596)) ;
#90339=CARTESIAN_POINT('',(63.3614933659285,216.167053742856,16.0213203435596)) ;
#90340=CARTESIAN_POINT('',(69.2808968287545,215.776927458569,16.0213203435596)) ;
#90341=CARTESIAN_POINT('',(61.3703326482681,217.618162279643,16.0213203435596)) ;
#90342=CARTESIAN_POINT('Origin',(64.4831104165663,219.797752737776,16.0213203435596)) ;
#90343=CARTESIAN_POINT('',(56.8445815445825,224.081604697382,16.0213203435596)) ;
#90344=CARTESIAN_POINT('',(59.3765805603019,220.465535350009,16.0213203435596)) ;
#90345=CARTESIAN_POINT('Origin',(59.9573593128806,226.261195155516,16.0213203435596)) ;
#90346=CARTESIAN_POINT('',(65.4568347953872,218.760590800757,16.0213203435596)) ;
#90347=CARTESIAN_POINT('',(65.4568347953872,216.846231446812,16.0213203435596)) ;
#90348=CARTESIAN_POINT('',(65.4568347953872,224.289496829998,16.0213203435596)) ;
#90349=CARTESIAN_POINT('',(62.8568347953872,218.760590800757,16.0213203435596)) ;
#90350=CARTESIAN_POINT('Origin',(64.1568347953872,220.146231446812,16.0213203435596)) ;
#90351=CARTESIAN_POINT('',(62.8568347953872,216.846231446812,16.0213203435596)) ;
#90352=CARTESIAN_POINT('',(62.8568347953872,223.489496829998,16.0213203435596)) ;
#90353=CARTESIAN_POINT('',(67.7248479331787,216.846231446812,16.0213203435596)) ;
#90354=CARTESIAN_POINT('Ctrl Pts',(62.4573593128808,235.849044700347,29.5213203435596)) ;
#90355=CARTESIAN_POINT('Ctrl Pts',(62.4573593128808,235.849044700347,24.9613203435596)) ;
#90356=CARTESIAN_POINT('Ctrl Pts',(62.4573593128808,235.882800482314,29.5213203435596)) ;
#90357=CARTESIAN_POINT('Ctrl Pts',(62.4573593128808,235.882800482314,24.9613203435596)) ;
#90358=CARTESIAN_POINT('Ctrl Pts',(62.4423298065164,235.916280466737,29.5213203435596)) ;
#90359=CARTESIAN_POINT('Ctrl Pts',(62.4423298065164,235.916280466737,24.9613203435596)) ;
#90360=CARTESIAN_POINT('Ctrl Pts',(62.4171062395287,235.938713132308,29.5213203435596)) ;
#90361=CARTESIAN_POINT('Ctrl Pts',(62.4171062395287,235.938713132308,24.9613203435596)) ;
#90362=CARTESIAN_POINT('',(62.4573593128808,235.849044700347,25.7213203435596)) ;
#90363=CARTESIAN_POINT('',(62.4169327150641,235.938516599365,25.7213203435596)) ;
#90364=CARTESIAN_POINT('Origin',(62.3640981990777,235.86104805899,25.7213203435596)) ;
#90365=CARTESIAN_POINT('',(62.4573593128808,235.849044700347,29.5213203435596)) ;
#90366=CARTESIAN_POINT('',(62.4573593128808,235.849044700347,25.7213203435596)) ;
#90367=CARTESIAN_POINT('',(62.4169327150641,235.938516599365,29.5213203435596)) ;
#90368=CARTESIAN_POINT('Origin',(62.3640981990903,235.861048058995,29.5213203435596)) ;
#90369=CARTESIAN_POINT('',(62.4169327140377,235.938516598221,29.5213203435596)) ;
#90370=CARTESIAN_POINT('Ctrl Pts',(62.4573593128808,235.9,29.5213203435596)) ;
#90371=CARTESIAN_POINT('Ctrl Pts',(62.4573593128808,235.9,18.1213203435596)) ;
#90372=CARTESIAN_POINT('Ctrl Pts',(62.4296494906727,235.927709822208,29.5213203435596)) ;
#90373=CARTESIAN_POINT('Ctrl Pts',(62.4296494906727,235.927709822208,18.1213203435596)) ;
#90374=CARTESIAN_POINT('Ctrl Pts',(62.3958369856604,235.960391271619,29.5213203435596)) ;
#90375=CARTESIAN_POINT('Ctrl Pts',(62.3958369856604,235.960391271619,18.1213203435596)) ;
#90376=CARTESIAN_POINT('Ctrl Pts',(62.3388862655657,235.99104280001,29.5213203435596)) ;
#90377=CARTESIAN_POINT('Ctrl Pts',(62.3388862655657,235.99104280001,18.1213203435596)) ;
#90378=CARTESIAN_POINT('Ctrl Pts',(62.3096419743114,236.,29.5213203435596)) ;
#90379=CARTESIAN_POINT('Ctrl Pts',(62.3096419743114,236.,18.1213203435596)) ;
#90380=CARTESIAN_POINT('Ctrl Pts',(62.2841542321239,236.,29.5213203435596)) ;
#90381=CARTESIAN_POINT('Ctrl Pts',(62.2841542321239,236.,18.1213203435596)) ;
#90382=CARTESIAN_POINT('',(62.2841542321239,236.,29.5213203435596)) ;
#90383=CARTESIAN_POINT('Ctrl Pts',(62.4169327140379,235.938516598221,29.5213203435596)) ;
#90384=CARTESIAN_POINT('Ctrl Pts',(62.3992166438732,235.954158616459,29.5213203435596)) ;
#90385=CARTESIAN_POINT('Ctrl Pts',(62.3803790823931,235.968710891811,29.5213203435596)) ;
#90386=CARTESIAN_POINT('Ctrl Pts',(62.3388862655657,235.99104280001,29.5213203435596)) ;
#90387=CARTESIAN_POINT('Ctrl Pts',(62.3096419743114,236.,29.5213203435596)) ;
#90388=CARTESIAN_POINT('Ctrl Pts',(62.2841542321239,236.,29.5213203435596)) ;
#90389=CARTESIAN_POINT('',(62.2841542321239,236.,25.7213203435596)) ;
#90390=CARTESIAN_POINT('',(62.2841542321239,236.,29.5213203435596)) ;
#90391=CARTESIAN_POINT('Ctrl Pts',(62.2841542321239,236.,25.7213203435596)) ;
#90392=CARTESIAN_POINT('Ctrl Pts',(62.3096419743114,236.,25.7213203435596)) ;
#90393=CARTESIAN_POINT('Ctrl Pts',(62.3388862655657,235.99104280001,25.7213203435596)) ;
#90394=CARTESIAN_POINT('Ctrl Pts',(62.3803790823931,235.968710891811,25.7213203435596)) ;
#90395=CARTESIAN_POINT('Ctrl Pts',(62.3992166438732,235.954158616459,25.7213203435596)) ;
#90396=CARTESIAN_POINT('Ctrl Pts',(62.4169327140379,235.938516598221,25.7213203435596)) ;
#90397=CARTESIAN_POINT('Origin',(66.56,251.44,19.7813203435596)) ;
#90398=CARTESIAN_POINT('',(66.56,251.2,20.2613203435596)) ;
#90399=CARTESIAN_POINT('',(66.56,251.44,20.0213203435596)) ;
#90400=CARTESIAN_POINT('Origin',(66.56,251.44,20.2613203435596)) ;
#90401=CARTESIAN_POINT('',(66.8,251.44,19.7813203435596)) ;
#90402=CARTESIAN_POINT('Origin',(66.56,251.44,19.7813203435596)) ;
#90403=CARTESIAN_POINT('',(66.8,251.2,20.1970125373762)) ;
#90404=CARTESIAN_POINT('Ctrl Pts',(66.8,251.2,20.1970125373761)) ;
#90405=CARTESIAN_POINT('Ctrl Pts',(66.8,251.2,20.1634772824134)) ;
#90406=CARTESIAN_POINT('Ctrl Pts',(66.8,251.206626505453,20.123784303008)) ;
#90407=CARTESIAN_POINT('Ctrl Pts',(66.8,251.228274899711,20.0539974766885)) ;
#90408=CARTESIAN_POINT('Ctrl Pts',(66.8,251.249130360957,20.011389083393)) ;
#90409=CARTESIAN_POINT('Ctrl Pts',(66.8,251.313969023646,19.9090950900013)) ;
#90410=CARTESIAN_POINT('Ctrl Pts',(66.8,251.382314385242,19.8390059583173)) ;
#90411=CARTESIAN_POINT('Ctrl Pts',(66.8,251.44,19.7813203435596)) ;
#90412=CARTESIAN_POINT('Origin',(66.56,251.2,19.7813203435596)) ;
#90413=CARTESIAN_POINT('Origin',(65.975,251.44,20.2613203435596)) ;
#90414=CARTESIAN_POINT('',(66.1,251.2,20.2613203435596)) ;
#90415=CARTESIAN_POINT('',(66.1,251.44,20.0213203435596)) ;
#90416=CARTESIAN_POINT('Origin',(66.1,251.44,20.2613203435596)) ;
#90417=CARTESIAN_POINT('',(65.975,251.44,20.0213203435596)) ;
#90418=CARTESIAN_POINT('',(65.975,251.2,20.2613203435596)) ;
#90419=CARTESIAN_POINT('Ctrl Pts',(65.9400000000002,251.6,20.0213203435596)) ;
#90420=CARTESIAN_POINT('Ctrl Pts',(65.9400000000003,251.44,20.0213203435596)) ;
#90421=CARTESIAN_POINT('Ctrl Pts',(66.1000000000004,251.44,20.0213203435596)) ;
#90422=CARTESIAN_POINT('Ctrl Pts',(65.7,251.6,20.0213203435594)) ;
#90423=CARTESIAN_POINT('Ctrl Pts',(65.7000000000003,251.2,20.0213203435594)) ;
#90424=CARTESIAN_POINT('Ctrl Pts',(66.1000000000004,251.2,20.0213203435594)) ;
#90425=CARTESIAN_POINT('Ctrl Pts',(65.7,251.6,20.2613203435596)) ;
#90426=CARTESIAN_POINT('Ctrl Pts',(65.7000000000003,251.2,20.2613203435596)) ;
#90427=CARTESIAN_POINT('Ctrl Pts',(66.1000000000004,251.2,20.2613203435596)) ;
#90428=CARTESIAN_POINT('',(65.7,251.6,20.2613203435596)) ;
#90429=CARTESIAN_POINT('',(65.94,251.6,20.0213203435596)) ;
#90430=CARTESIAN_POINT('Origin',(65.94,251.6,20.2613203435596)) ;
#90431=CARTESIAN_POINT('Origin',(66.1,251.6,20.0213203435596)) ;
#90432=CARTESIAN_POINT('Origin',(66.1,251.6,20.2613203435596)) ;
#90433=CARTESIAN_POINT('Origin',(65.94,252.4,20.2613203435596)) ;
#90434=CARTESIAN_POINT('',(65.7,253.055933015586,20.2613203435596)) ;
#90435=CARTESIAN_POINT('',(65.9396674027608,253.055812426285,20.0212455719998)) ;
#90436=CARTESIAN_POINT('Origin',(65.94,253.055933015586,20.2613203435596)) ;
#90437=CARTESIAN_POINT('',(65.94,253.053504693378,20.0213203435596)) ;
#90438=CARTESIAN_POINT('Ctrl Pts',(65.9396674027608,253.055812426285,20.0213203435596)) ;
#90439=CARTESIAN_POINT('Ctrl Pts',(65.9397782685072,253.055043181982,20.0213203435596)) ;
#90440=CARTESIAN_POINT('Ctrl Pts',(65.9398891342536,253.05427393768,20.0213203435596)) ;
#90441=CARTESIAN_POINT('Ctrl Pts',(65.94,253.053504693378,20.0213203435596)) ;
#90442=CARTESIAN_POINT('',(65.94,252.4,20.0213203435596)) ;
#90443=CARTESIAN_POINT('',(65.7,252.4,20.2613203435596)) ;
#90444=CARTESIAN_POINT('Ctrl Pts',(65.8787223053518,253.200000000043,20.0213203435596)) ;
#90445=CARTESIAN_POINT('Ctrl Pts',(65.8988550182207,253.152091884828,20.0213203435596)) ;
#90446=CARTESIAN_POINT('Ctrl Pts',(65.9192601391554,253.103601946723,20.0213203435596)) ;
#90447=CARTESIAN_POINT('Ctrl Pts',(65.9400000000004,253.055933015586,20.0213203435596)) ;
#90448=CARTESIAN_POINT('Ctrl Pts',(65.8279579835555,253.201487684761,20.0346431984532)) ;
#90449=CARTESIAN_POINT('Ctrl Pts',(65.8435615888772,253.152668920777,20.0311364548328)) ;
#90450=CARTESIAN_POINT('Ctrl Pts',(65.8598723347433,253.10358309864,20.0268717600141)) ;
#90451=CARTESIAN_POINT('Ctrl Pts',(65.8771681469285,253.055933015586,20.0213203435595)) ;
#90452=CARTESIAN_POINT('Ctrl Pts',(65.735859111132,253.208302568615,20.0956734070701)) ;
#90453=CARTESIAN_POINT('Ctrl Pts',(65.740788844418,253.156930054594,20.091034868245)) ;
#90454=CARTESIAN_POINT('Ctrl Pts',(65.7461509033861,253.105566496234,20.0836957459916)) ;
#90455=CARTESIAN_POINT('Ctrl Pts',(65.752215309716,253.055933015586,20.0735356532753)) ;
#90456=CARTESIAN_POINT('Ctrl Pts',(65.6999999999998,253.219924430328,20.1997521646846)) ;
#90457=CARTESIAN_POINT('Ctrl Pts',(65.6999351060341,253.165238884986,20.2023526749646)) ;
#90458=CARTESIAN_POINT('Ctrl Pts',(65.7001128677229,253.11025926159,20.2019758599767)) ;
#90459=CARTESIAN_POINT('Ctrl Pts',(65.7,253.055933015586,20.1984884904878)) ;
#90460=CARTESIAN_POINT('Ctrl Pts',(65.6999999999998,253.225751090982,20.2519324105771)) ;
#90461=CARTESIAN_POINT('Ctrl Pts',(65.6999999999998,253.16940880829,20.2582238213609)) ;
#90462=CARTESIAN_POINT('Ctrl Pts',(65.7,253.112625472478,20.2613203435597)) ;
#90463=CARTESIAN_POINT('Ctrl Pts',(65.7,253.055933015586,20.2613203435596)) ;
#90464=CARTESIAN_POINT('',(65.8787220969437,253.199999911797,20.021320809239)) ;
#90465=CARTESIAN_POINT('',(65.6999999999999,253.200000001188,20.2545830286245)) ;
#90466=CARTESIAN_POINT('Ctrl Pts',(65.8787219951101,253.2,20.0213204260013)) ;
#90467=CARTESIAN_POINT('Ctrl Pts',(65.8637513393088,253.2,20.0252984157073)) ;
#90468=CARTESIAN_POINT('Ctrl Pts',(65.8492674755271,253.2,20.0307646764352)) ;
#90469=CARTESIAN_POINT('Ctrl Pts',(65.8354281636608,253.2,20.0375555002856)) ;
#90470=CARTESIAN_POINT('Ctrl Pts',(65.8215887561901,253.2,20.0443463710483)) ;
#90471=CARTESIAN_POINT('Ctrl Pts',(65.8083925033119,253.2,20.0524630322388)) ;
#90472=CARTESIAN_POINT('Ctrl Pts',(65.7960263435029,253.2,20.0617902565927)) ;
#90473=CARTESIAN_POINT('Ctrl Pts',(65.7841216235844,253.2,20.0707694381062)) ;
#90474=CARTESIAN_POINT('Ctrl Pts',(65.7730938774418,253.2,20.0807890097741)) ;
#90475=CARTESIAN_POINT('Ctrl Pts',(65.7630914752968,253.2,20.0917318564667)) ;
#90476=CARTESIAN_POINT('Ctrl Pts',(65.7589082319733,253.2,20.0963084161475)) ;
#90477=CARTESIAN_POINT('Ctrl Pts',(65.7549047310405,253.2,20.101046950744)) ;
#90478=CARTESIAN_POINT('Ctrl Pts',(65.7510938065472,253.2,20.1059407077756)) ;
#90479=CARTESIAN_POINT('Ctrl Pts',(65.7448220996584,253.2,20.1139944516221)) ;
#90480=CARTESIAN_POINT('Ctrl Pts',(65.7390714447429,253.2,20.1224685139581)) ;
#90481=CARTESIAN_POINT('Ctrl Pts',(65.7338649261578,253.2,20.1313038355597)) ;
#90482=CARTESIAN_POINT('Ctrl Pts',(65.7261735242395,253.2,20.1443559371521)) ;
#90483=CARTESIAN_POINT('Ctrl Pts',(65.7197244243772,253.2,20.1580982486252)) ;
#90484=CARTESIAN_POINT('Ctrl Pts',(65.714572824113,253.2,20.1723335497224)) ;
#90485=CARTESIAN_POINT('Ctrl Pts',(65.7124421681154,253.2,20.1782211435001)) ;
#90486=CARTESIAN_POINT('Ctrl Pts',(65.7105340250227,253.2,20.1841933262792)) ;
#90487=CARTESIAN_POINT('Ctrl Pts',(65.7088547698819,253.2,20.1902368435495)) ;
#90488=CARTESIAN_POINT('Ctrl Pts',(65.7048015662676,253.2,20.2048240289322)) ;
#90489=CARTESIAN_POINT('Ctrl Pts',(65.7021029059883,253.2,20.2197377335324)) ;
#90490=CARTESIAN_POINT('Ctrl Pts',(65.7008336869791,253.2,20.2347908075204)) ;
#90491=CARTESIAN_POINT('Ctrl Pts',(65.7002792381749,253.2,20.2413666299846)) ;
#90492=CARTESIAN_POINT('Ctrl Pts',(65.6999982168404,253.2,20.247969183683)) ;
#90493=CARTESIAN_POINT('Ctrl Pts',(65.6999999999998,253.2,20.2545830064533)) ;
#90494=CARTESIAN_POINT('',(65.9054141138738,253.136644520473,20.0212807249742)) ;
#90495=CARTESIAN_POINT('Ctrl Pts',(65.8787223180024,253.200000004773,20.0213211815297)) ;
#90496=CARTESIAN_POINT('Ctrl Pts',(65.8875660862203,253.178955523856,20.0213256058334)) ;
#90497=CARTESIAN_POINT('Ctrl Pts',(65.8964675487447,253.157798296395,20.0213194598004)) ;
#90498=CARTESIAN_POINT('Ctrl Pts',(65.9054141138738,253.136644520473,20.0212807249742)) ;
#90499=CARTESIAN_POINT('Ctrl Pts',(65.9054141138738,253.136644520473,20.0212807249742)) ;
#90500=CARTESIAN_POINT('Ctrl Pts',(65.9147761239318,253.114508442539,20.0212401914478)) ;
#90501=CARTESIAN_POINT('Ctrl Pts',(65.9241869890751,253.09237636557,20.0211639482418)) ;
#90502=CARTESIAN_POINT('Ctrl Pts',(65.93365196153,253.07038006692,20.0210779520608)) ;
#90503=CARTESIAN_POINT('Ctrl Pts',(65.935730195249,253.065550317043,20.021059069791)) ;
#90504=CARTESIAN_POINT('Ctrl Pts',(65.9378111246201,253.060727099485,20.0210398990018)) ;
#90505=CARTESIAN_POINT('Ctrl Pts',(65.9398949529419,253.055911779844,20.0210210022763)) ;
#90506=CARTESIAN_POINT('Origin',(65.6999999999758,253.056278660127,18.7250135059453)) ;
#90507=CARTESIAN_POINT('Origin',(65.7,253.,24.0213203435596)) ;
#90508=CARTESIAN_POINT('',(65.7,251.6,23.0213203435596)) ;
#90509=CARTESIAN_POINT('',(65.7,251.6,20.0213203435596)) ;
#90510=CARTESIAN_POINT('',(65.7,253.1,23.0213203435596)) ;
#90511=CARTESIAN_POINT('',(65.7,252.4,23.0213203435596)) ;
#90512=CARTESIAN_POINT('',(65.7,253.1,24.0213203435596)) ;
#90513=CARTESIAN_POINT('',(65.7,253.1,24.0213203435596)) ;
#90514=CARTESIAN_POINT('',(65.7,253.2,24.0213203435596)) ;
#90515=CARTESIAN_POINT('',(65.7,253.,24.0213203435596)) ;
#90516=CARTESIAN_POINT('',(65.7,253.2,24.0213203435596)) ;
#90517=CARTESIAN_POINT('Origin',(66.1,251.6,20.0213203435596)) ;
#90518=CARTESIAN_POINT('',(66.1,251.2,23.0213203435596)) ;
#90519=CARTESIAN_POINT('',(66.1,251.2,20.0213203435596)) ;
#90520=CARTESIAN_POINT('Origin',(66.1,251.6,23.0213203435596)) ;
#90521=CARTESIAN_POINT('Origin',(65.7,251.2,20.0213203435596)) ;
#90522=CARTESIAN_POINT('',(66.8,251.2,23.0213203435596)) ;
#90523=CARTESIAN_POINT('',(66.8,251.2,22.0213203435596)) ;
#90524=CARTESIAN_POINT('',(65.975,251.2,23.0213203435596)) ;
#90525=CARTESIAN_POINT('Ctrl Pts',(59.4599709502105,252.66176631391,20.0213203406956)) ;
#90526=CARTESIAN_POINT('Ctrl Pts',(59.4862791845716,252.73300766342,20.0213255280724)) ;
#90527=CARTESIAN_POINT('Ctrl Pts',(59.5476801368282,252.899278293364,20.0048984182032)) ;
#90528=CARTESIAN_POINT('Ctrl Pts',(59.5942467666672,253.025378338935,19.9538218787239)) ;
#90529=CARTESIAN_POINT('Ctrl Pts',(59.6112632622918,253.071458136446,19.9183779157918)) ;
#90530=CARTESIAN_POINT('Ctrl Pts',(59.5228076267856,252.661766373174,20.0213125642804)) ;
#90531=CARTESIAN_POINT('Ctrl Pts',(59.5447480140858,252.732953219279,20.0283608967158)) ;
#90532=CARTESIAN_POINT('Ctrl Pts',(59.5931584269531,252.904373903459,20.0244169597432)) ;
#90533=CARTESIAN_POINT('Ctrl Pts',(59.6267463142549,253.039426939223,19.9717522594694)) ;
#90534=CARTESIAN_POINT('Ctrl Pts',(59.6388683863242,253.088950591174,19.9323854375313)) ;
#90535=CARTESIAN_POINT('Ctrl Pts',(59.6477975268572,252.661760233233,20.0735298372816)) ;
#90536=CARTESIAN_POINT('Ctrl Pts',(59.6554884901573,252.738506902787,20.0864278965363)) ;
#90537=CARTESIAN_POINT('Ctrl Pts',(59.6711001024041,252.927116008415,20.0875757744157)) ;
#90538=CARTESIAN_POINT('Ctrl Pts',(59.6805415396398,253.078232351583,20.0199472449724)) ;
#90539=CARTESIAN_POINT('Ctrl Pts',(59.6839102088974,253.133679100257,19.9682029127294)) ;
#90540=CARTESIAN_POINT('Ctrl Pts',(59.7000176946533,252.661745701756,20.1985255688626)) ;
#90541=CARTESIAN_POINT('Ctrl Pts',(59.6998718034678,252.75165343376,20.2029571135977)) ;
#90542=CARTESIAN_POINT('Ctrl Pts',(59.6998122444854,252.964737640422,20.1793702220234)) ;
#90543=CARTESIAN_POINT('Ctrl Pts',(59.7000270806329,253.129051719149,20.0818652291328)) ;
#90544=CARTESIAN_POINT('Ctrl Pts',(59.7000054052531,253.189168023934,20.012637059726)) ;
#90545=CARTESIAN_POINT('Ctrl Pts',(59.6999999910052,252.66173837404,20.2613836458743)) ;
#90546=CARTESIAN_POINT('Ctrl Pts',(59.7000001367147,252.758282786987,20.2613906018571)) ;
#90547=CARTESIAN_POINT('Ctrl Pts',(59.7000001940885,252.983605119967,20.2252383047188)) ;
#90548=CARTESIAN_POINT('Ctrl Pts',(59.699999976005,253.154487386442,20.1128549327947)) ;
#90549=CARTESIAN_POINT('Ctrl Pts',(59.6999999972766,253.216931543521,20.0348693941943)) ;
#90550=CARTESIAN_POINT('',(59.7,253.2,20.0547106776782)) ;
#90551=CARTESIAN_POINT('',(59.6989357893727,253.198893220947,20.0213203435596)) ;
#90552=CARTESIAN_POINT('Ctrl Pts',(59.7,253.2,20.0546787338963)) ;
#90553=CARTESIAN_POINT('Ctrl Pts',(59.7000002277722,253.2,20.0491133758029)) ;
#90554=CARTESIAN_POINT('Ctrl Pts',(59.6999115519515,253.2,20.0435500952352)) ;
#90555=CARTESIAN_POINT('Ctrl Pts',(59.6995747351395,253.2,20.0324243353057)) ;
#90556=CARTESIAN_POINT('Ctrl Pts',(59.6993268096966,253.2,20.0268679068488)) ;
#90557=CARTESIAN_POINT('Ctrl Pts',(59.6990088056403,253.2,20.021311332408)) ;
#90558=CARTESIAN_POINT('',(59.7,252.66184497925,20.2613203435596)) ;
#90559=CARTESIAN_POINT('Origin',(59.7,252.66184497925,19.8213203435596)) ;
#90560=CARTESIAN_POINT('',(59.46,252.66184497925,20.0213203435596)) ;
#90561=CARTESIAN_POINT('Origin',(59.46,252.66184497925,20.2613203435596)) ;
#90562=CARTESIAN_POINT('',(59.542455661465,252.885254883942,19.9972444447401)) ;
#90563=CARTESIAN_POINT('Origin',(59.46,252.66184497925,19.8213203435596)) ;
#90564=CARTESIAN_POINT('',(59.6074881670737,252.973767115183,19.9952481069197)) ;
#90565=CARTESIAN_POINT('Ctrl Pts',(59.5424456954486,252.885275820812,19.9972326388961)) ;
#90566=CARTESIAN_POINT('Ctrl Pts',(59.542916942341,252.885870023412,19.9971914059271)) ;
#90567=CARTESIAN_POINT('Ctrl Pts',(59.5433878129887,252.886464556907,19.9971507181093)) ;
#90568=CARTESIAN_POINT('Ctrl Pts',(59.5438575843988,252.887058515381,19.9971106340598)) ;
#90569=CARTESIAN_POINT('Ctrl Pts',(59.5530969190852,252.898740327019,19.996322272015)) ;
#90570=CARTESIAN_POINT('Ctrl Pts',(59.5624673714554,252.910908714203,19.9957195274863)) ;
#90571=CARTESIAN_POINT('Ctrl Pts',(59.571742193056,252.923362468785,19.995356358669)) ;
#90572=CARTESIAN_POINT('Ctrl Pts',(59.5806730652746,252.935354385784,19.9950066576785)) ;
#90573=CARTESIAN_POINT('Ctrl Pts',(59.5895141940076,252.947611011629,19.9948775133271)) ;
#90574=CARTESIAN_POINT('Ctrl Pts',(59.5980894303711,252.95998930852,19.9950028035369)) ;
#90575=CARTESIAN_POINT('Ctrl Pts',(59.6012608458573,252.964567225768,19.9950491401386)) ;
#90576=CARTESIAN_POINT('Ctrl Pts',(59.6043962457373,252.969162147482,19.9951302491092)) ;
#90577=CARTESIAN_POINT('Ctrl Pts',(59.6074880869828,252.97376808314,19.9952479713636)) ;
#90578=CARTESIAN_POINT('',(59.6445121748197,252.999999508894,20.021320114607)) ;
#90579=CARTESIAN_POINT('Ctrl Pts',(59.6075096705789,252.973853981228,19.9951743247871)) ;
#90580=CARTESIAN_POINT('Ctrl Pts',(59.6142809805769,252.977720686039,19.9990410295982)) ;
#90581=CARTESIAN_POINT('Ctrl Pts',(59.6207622195018,252.981841745709,20.0031620892954)) ;
#90582=CARTESIAN_POINT('Ctrl Pts',(59.6331221952063,252.990570656193,20.0118909997797)) ;
#90583=CARTESIAN_POINT('Ctrl Pts',(59.6389969882328,252.99518214824,20.0165024917991)) ;
#90584=CARTESIAN_POINT('Ctrl Pts',(59.6445120247841,252.999999313142,20.0213196567018)) ;
#90585=CARTESIAN_POINT('Ctrl Pts',(59.6445125319219,252.999999354438,20.0213203435596)) ;
#90586=CARTESIAN_POINT('Ctrl Pts',(59.6583065581309,253.031891118753,20.0213203435596)) ;
#90587=CARTESIAN_POINT('Ctrl Pts',(59.6707567119401,253.064944388245,20.021320344362)) ;
#90588=CARTESIAN_POINT('Ctrl Pts',(59.6896400105539,253.131227832493,20.021320344362)) ;
#90589=CARTESIAN_POINT('Ctrl Pts',(59.6964171938951,253.164990946491,20.0213203435596)) ;
#90590=CARTESIAN_POINT('Ctrl Pts',(59.6989291504472,253.198897505808,20.0213203435596)) ;
#90591=CARTESIAN_POINT('Origin',(59.46,251.2,20.2613203435596)) ;
#90592=CARTESIAN_POINT('',(59.7,251.6,20.2613203435596)) ;
#90593=CARTESIAN_POINT('',(59.46,251.6,20.0213203435596)) ;
#90594=CARTESIAN_POINT('Origin',(59.46,251.6,20.2613203435596)) ;
#90595=CARTESIAN_POINT('',(59.46,251.2,20.0213203435596)) ;
#90596=CARTESIAN_POINT('',(59.7,251.2,20.2613203435596)) ;
#90597=CARTESIAN_POINT('Ctrl Pts',(59.2999999999997,251.44,20.0213203435596)) ;
#90598=CARTESIAN_POINT('Ctrl Pts',(59.4599999999999,251.44,20.0213203435596)) ;
#90599=CARTESIAN_POINT('Ctrl Pts',(59.46,251.6,20.0213203435596)) ;
#90600=CARTESIAN_POINT('Ctrl Pts',(59.2999999999997,251.2,20.0213203435595)) ;
#90601=CARTESIAN_POINT('Ctrl Pts',(59.6999999999999,251.2,20.0213203435594)) ;
#90602=CARTESIAN_POINT('Ctrl Pts',(59.7000000000001,251.6,20.0213203435595)) ;
#90603=CARTESIAN_POINT('Ctrl Pts',(59.2999999999998,251.2,20.2613203435596)) ;
#90604=CARTESIAN_POINT('Ctrl Pts',(59.6999999999999,251.2,20.2613203435595)) ;
#90605=CARTESIAN_POINT('Ctrl Pts',(59.7000000000001,251.6,20.2613203435596)) ;
#90606=CARTESIAN_POINT('',(59.3,251.2,20.2613203435596)) ;
#90607=CARTESIAN_POINT('',(59.3,251.44,20.0213203435596)) ;
#90608=CARTESIAN_POINT('Origin',(59.3,251.44,20.2613203435596)) ;
#90609=CARTESIAN_POINT('Origin',(59.3,251.6,20.0213203435596)) ;
#90610=CARTESIAN_POINT('Origin',(59.3,251.6,20.2613203435596)) ;
#90611=CARTESIAN_POINT('Origin',(65.975,251.44,20.2613203435596)) ;
#90612=CARTESIAN_POINT('',(58.84,251.2,20.2613203435596)) ;
#90613=CARTESIAN_POINT('',(58.84,251.44,20.0213203435596)) ;
#90614=CARTESIAN_POINT('Origin',(58.84,251.44,20.2613203435596)) ;
#90615=CARTESIAN_POINT('',(65.975,251.44,20.0213203435596)) ;
#90616=CARTESIAN_POINT('',(65.975,251.2,20.2613203435596)) ;
#90617=CARTESIAN_POINT('Origin',(58.84,251.44,19.7813203435596)) ;
#90618=CARTESIAN_POINT('',(58.6,251.2,20.1970125373762)) ;
#90619=CARTESIAN_POINT('',(58.6,251.44,19.7813203435596)) ;
#90620=CARTESIAN_POINT('Ctrl Pts',(58.6000000000001,251.44,19.7813203435596)) ;
#90621=CARTESIAN_POINT('Ctrl Pts',(58.6000000000001,251.373496426701,19.847823916859)) ;
#90622=CARTESIAN_POINT('Ctrl Pts',(58.6000000000001,251.295060948115,19.9289739288886)) ;
#90623=CARTESIAN_POINT('Ctrl Pts',(58.6000000000001,251.221497279975,20.0656556571159)) ;
#90624=CARTESIAN_POINT('Ctrl Pts',(58.6000000000001,251.2,20.135841956126)) ;
#90625=CARTESIAN_POINT('Ctrl Pts',(58.6000000000001,251.2,20.1970125373762)) ;
#90626=CARTESIAN_POINT('Origin',(58.84,251.44,19.7813203435596)) ;
#90627=CARTESIAN_POINT('Origin',(58.84,251.2,19.7813203435596)) ;
#90628=CARTESIAN_POINT('Origin',(65.7,251.2,20.0213203435596)) ;
#90629=CARTESIAN_POINT('',(59.3,251.2,23.0213203435596)) ;
#90630=CARTESIAN_POINT('',(59.3,251.2,20.0213203435596)) ;
#90631=CARTESIAN_POINT('',(58.6,251.2,23.0213203435596)) ;
#90632=CARTESIAN_POINT('',(65.975,251.2,23.0213203435596)) ;
#90633=CARTESIAN_POINT('',(58.6,251.2,22.0213203435596)) ;
#90634=CARTESIAN_POINT('Origin',(59.3,251.6,20.0213203435596)) ;
#90635=CARTESIAN_POINT('',(59.7,251.6,23.0213203435596)) ;
#90636=CARTESIAN_POINT('',(59.7,251.6,20.0213203435596)) ;
#90637=CARTESIAN_POINT('Origin',(59.3,251.6,23.0213203435596)) ;
#90638=CARTESIAN_POINT('Origin',(59.7,250.6,20.0213203435596)) ;
#90639=CARTESIAN_POINT('',(59.7,253.2,23.0213203435596)) ;
#90640=CARTESIAN_POINT('',(59.7,253.2,22.0213203435596)) ;
#90641=CARTESIAN_POINT('',(59.7,242.,23.0213203435596)) ;
#90642=CARTESIAN_POINT('Ctrl Pts',(59.6983561413947,253.201132335348,20.0213068391943)) ;
#90643=CARTESIAN_POINT('Ctrl Pts',(59.6405833573623,253.138206691657,20.0213203435596)) ;
#90644=CARTESIAN_POINT('Ctrl Pts',(59.5229242400133,253.015841209614,20.0213203435596)) ;
#90645=CARTESIAN_POINT('Ctrl Pts',(59.3615012183121,252.847961267045,20.0213203435596)) ;
#90646=CARTESIAN_POINT('Ctrl Pts',(59.2467429329946,252.728612650314,20.0213203435596)) ;
#90647=CARTESIAN_POINT('Ctrl Pts',(59.1766245450661,252.655689526869,20.0213203435596)) ;
#90648=CARTESIAN_POINT('Ctrl Pts',(59.1427392883506,252.620448859885,20.0213203435596)) ;
#90649=CARTESIAN_POINT('Ctrl Pts',(59.1198396721444,252.59663325903,20.0213203435596)) ;
#90650=CARTESIAN_POINT('Ctrl Pts',(59.1070160194856,252.583296660265,20.0213203435596)) ;
#90651=CARTESIAN_POINT('Ctrl Pts',(59.100742188597,252.576771876141,20.0213203435596)) ;
#90652=CARTESIAN_POINT('Ctrl Pts',(59.0976481299957,252.573554055196,20.0213203435596)) ;
#90653=CARTESIAN_POINT('Ctrl Pts',(59.6983561413947,253.201132335348,20.0213068391943)) ;
#90654=CARTESIAN_POINT('Ctrl Pts',(59.6387389889223,253.141348443802,20.0212943049799)) ;
#90655=CARTESIAN_POINT('Ctrl Pts',(59.5177887613006,253.024552101869,20.0188009859938)) ;
#90656=CARTESIAN_POINT('Ctrl Pts',(59.3547417480892,252.862674067239,20.0094198699614)) ;
#90657=CARTESIAN_POINT('Ctrl Pts',(59.2436260334543,252.74520130829,19.9993245938688)) ;
#90658=CARTESIAN_POINT('Ctrl Pts',(59.1797745588704,252.672296794036,19.9930704302621)) ;
#90659=CARTESIAN_POINT('Ctrl Pts',(59.150461980661,252.636868221831,19.990450276081)) ;
#90660=CARTESIAN_POINT('Ctrl Pts',(59.1317791109331,252.612984832977,19.9893039012676)) ;
#90661=CARTESIAN_POINT('Ctrl Pts',(59.1217337199043,252.599697553955,19.9889950808986)) ;
#90662=CARTESIAN_POINT('Ctrl Pts',(59.1169697132597,252.593243019353,19.9889876151247)) ;
#90663=CARTESIAN_POINT('Ctrl Pts',(59.114661714354,252.590077279297,19.9890311381653)) ;
#90664=CARTESIAN_POINT('Ctrl Pts',(59.6983561413947,253.201132335348,20.0213068391943)) ;
#90665=CARTESIAN_POINT('Ctrl Pts',(59.6350498031855,253.147632380457,20.0212422231911)) ;
#90666=CARTESIAN_POINT('Ctrl Pts',(59.5075447508945,253.041891485879,20.0149253757923)) ;
#90667=CARTESIAN_POINT('Ctrl Pts',(59.3390921011038,252.89406358936,19.9902535879186)) ;
#90668=CARTESIAN_POINT('Ctrl Pts',(59.2306666331395,252.784723922575,19.9617875770576)) ;
#90669=CARTESIAN_POINT('Ctrl Pts',(59.174826300634,252.71614725735,19.942028468966)) ;
#90670=CARTESIAN_POINT('Ctrl Pts',(59.151995644535,252.682857965521,19.9327134222409)) ;
#90671=CARTESIAN_POINT('Ctrl Pts',(59.1397130985584,252.660746974676,19.9274872737863)) ;
#90672=CARTESIAN_POINT('Ctrl Pts',(59.1340298579112,252.648674214786,19.9252363474521)) ;
#90673=CARTESIAN_POINT('Ctrl Pts',(59.1316869209399,252.642917043708,19.9244431805881)) ;
#90674=CARTESIAN_POINT('Ctrl Pts',(59.1306535459891,252.640131701431,19.9241575626337)) ;
#90675=CARTESIAN_POINT('Ctrl Pts',(59.6983561413947,253.201132335348,20.0213068391943)) ;
#90676=CARTESIAN_POINT('Ctrl Pts',(59.6250143371155,253.164724381672,20.0211005575757)) ;
#90677=CARTESIAN_POINT('Ctrl Pts',(59.479716487384,253.089447846023,20.0098769411972)) ;
#90678=CARTESIAN_POINT('Ctrl Pts',(59.2877528595915,252.985613790057,19.9648062300671)) ;
#90679=CARTESIAN_POINT('Ctrl Pts',(59.1649824243651,252.911156238581,19.9083610107024)) ;
#90680=CARTESIAN_POINT('Ctrl Pts',(59.1038826177998,252.866722375844,19.8630066618772)) ;
#90681=CARTESIAN_POINT('Ctrl Pts',(59.0801924624728,252.846166525223,19.8385056723018)) ;
#90682=CARTESIAN_POINT('Ctrl Pts',(59.0688119787604,252.833471233285,19.8212764972742)) ;
#90683=CARTESIAN_POINT('Ctrl Pts',(59.0642587414283,252.826989190829,19.8117477346005)) ;
#90684=CARTESIAN_POINT('Ctrl Pts',(59.0627109533308,252.824088799222,19.8072083560344)) ;
#90685=CARTESIAN_POINT('Ctrl Pts',(59.0621414351439,252.822747469555,19.8050299254675)) ;
#90686=CARTESIAN_POINT('Ctrl Pts',(59.6983561413947,253.201132335348,20.0213068391943)) ;
#90687=CARTESIAN_POINT('Ctrl Pts',(59.6168230991084,253.17867209478,20.0209849428196)) ;
#90688=CARTESIAN_POINT('Ctrl Pts',(59.4566744266614,253.127543443304,20.0173244896171)) ;
#90689=CARTESIAN_POINT('Ctrl Pts',(59.235417471757,253.058718839497,19.9973837843722)) ;
#90690=CARTESIAN_POINT('Ctrl Pts',(59.0741608580319,253.010488324297,19.9709643752037)) ;
#90691=CARTESIAN_POINT('Ctrl Pts',(58.970763369431,252.979409797583,19.944956093994)) ;
#90692=CARTESIAN_POINT('Ctrl Pts',(58.9186367041767,252.963112203106,19.928060513653)) ;
#90693=CARTESIAN_POINT('Ctrl Pts',(58.8817163868829,252.950491410093,19.9126774778034)) ;
#90694=CARTESIAN_POINT('Ctrl Pts',(58.8604121341276,252.942597577878,19.9022589536899)) ;
#90695=CARTESIAN_POINT('Ctrl Pts',(58.8497660624433,252.938375656177,19.8964295097095)) ;
#90696=CARTESIAN_POINT('Ctrl Pts',(58.8444584671265,252.936177800295,19.8933199111082)) ;
#90697=CARTESIAN_POINT('Ctrl Pts',(59.6983561413947,253.201132335348,20.0213068391943)) ;
#90698=CARTESIAN_POINT('Ctrl Pts',(59.6104804032961,253.18947021835,20.0208954293076)) ;
#90699=CARTESIAN_POINT('Ctrl Pts',(59.4409767120307,253.161409042463,20.0226915082758)) ;
#90700=CARTESIAN_POINT('Ctrl Pts',(59.2056496041379,253.099665034983,20.0428866978387)) ;
#90701=CARTESIAN_POINT('Ctrl Pts',(59.0351181159364,253.021807165115,20.0645075503816)) ;
#90702=CARTESIAN_POINT('Ctrl Pts',(58.9263998406049,252.945184792316,20.0751016605283)) ;
#90703=CARTESIAN_POINT('Ctrl Pts',(58.8717548724627,252.896835253805,20.0775118985888)) ;
#90704=CARTESIAN_POINT('Ctrl Pts',(58.8331279718619,252.855453382999,20.0755760868657)) ;
#90705=CARTESIAN_POINT('Ctrl Pts',(58.8108414175582,252.828814232857,20.0726724433716)) ;
#90706=CARTESIAN_POINT('Ctrl Pts',(58.7997165407889,252.814483766437,20.0704334854542)) ;
#90707=CARTESIAN_POINT('Ctrl Pts',(58.7941662396937,252.80702403625,20.069077982382)) ;
#90708=CARTESIAN_POINT('',(59.5076923076923,253.,20.0213203435596)) ;
#90709=CARTESIAN_POINT('',(58.5931591083782,252.048885472713,20.0213203435596)) ;
#90710=CARTESIAN_POINT('',(58.9535270326722,252.853553390409,19.8748737339686)) ;
#90711=CARTESIAN_POINT('Ctrl Pts',(58.9535270332697,252.853553390621,19.8748737341804)) ;
#90712=CARTESIAN_POINT('Ctrl Pts',(58.9544812639864,252.853959618843,19.8752799624022)) ;
#90713=CARTESIAN_POINT('Ctrl Pts',(58.9554377472264,252.854363438162,19.8756837817213)) ;
#90714=CARTESIAN_POINT('Ctrl Pts',(59.0080837204097,252.876415266471,19.8977356100307)) ;
#90715=CARTESIAN_POINT('Ctrl Pts',(59.0819911038653,252.898174251807,19.9194945953742)) ;
#90716=CARTESIAN_POINT('Ctrl Pts',(59.2187094508916,252.931982805319,19.9533031488854)) ;
#90717=CARTESIAN_POINT('Ctrl Pts',(59.2544798933849,252.940439100737,19.9617594442965)) ;
#90718=CARTESIAN_POINT('Ctrl Pts',(59.3184078361109,252.955441546707,19.9767618902667)) ;
#90719=CARTESIAN_POINT('Ctrl Pts',(59.3580711003919,252.964683338623,19.9860036821827)) ;
#90720=CARTESIAN_POINT('Ctrl Pts',(59.430373614325,252.981655902742,20.0029762463013)) ;
#90721=CARTESIAN_POINT('Ctrl Pts',(59.4733907178604,252.991778140936,20.0130984844959)) ;
#90722=CARTESIAN_POINT('Ctrl Pts',(59.5076923076922,253.,20.0213203435596)) ;
#90723=CARTESIAN_POINT('',(59.6906222915952,253.199677791956,20.0212702067469)) ;
#90724=CARTESIAN_POINT('Ctrl Pts',(58.9535270325137,252.853553390013,19.8748737335726)) ;
#90725=CARTESIAN_POINT('Ctrl Pts',(58.9565617584117,252.855892584028,19.8772129275957)) ;
#90726=CARTESIAN_POINT('Ctrl Pts',(58.9596988881571,252.858222716888,19.8794965005046)) ;
#90727=CARTESIAN_POINT('Ctrl Pts',(58.9629217338132,252.860543300927,19.8817279974797)) ;
#90728=CARTESIAN_POINT('Ctrl Pts',(58.9661445794694,252.862863884965,19.8839594944547)) ;
#90729=CARTESIAN_POINT('Ctrl Pts',(58.9694531410364,252.865174920183,19.8861389154958)) ;
#90730=CARTESIAN_POINT('Ctrl Pts',(58.9728284392491,252.867471315475,19.8882643714541)) ;
#90731=CARTESIAN_POINT('Ctrl Pts',(58.9795790356745,252.872064106058,19.8925152833706)) ;
#90732=CARTESIAN_POINT('Ctrl Pts',(58.9865965786828,252.876598336938,19.8965503349557)) ;
#90733=CARTESIAN_POINT('Ctrl Pts',(58.9938251766377,252.881099271588,19.9004208018149)) ;
#90734=CARTESIAN_POINT('Ctrl Pts',(59.0082823725472,252.890101140888,19.9081617355332)) ;
#90735=CARTESIAN_POINT('Ctrl Pts',(59.0235837882427,252.898969825267,19.9152443303478)) ;
#90736=CARTESIAN_POINT('Ctrl Pts',(59.0394887827122,252.907759632436,19.9218109468869)) ;
#90737=CARTESIAN_POINT('Ctrl Pts',(59.0553937771816,252.916549439604,19.9283775634259)) ;
#90738=CARTESIAN_POINT('Ctrl Pts',(59.071902350425,252.925260369562,19.9344282016893)) ;
#90739=CARTESIAN_POINT('Ctrl Pts',(59.0887153135157,252.933877010233,19.940052639116)) ;
#90740=CARTESIAN_POINT('Ctrl Pts',(59.1391542027878,252.959726932244,19.9569259513962)) ;
#90741=CARTESIAN_POINT('Ctrl Pts',(59.1923326006852,252.984728250665,19.9699634561467)) ;
#90742=CARTESIAN_POINT('Ctrl Pts',(59.2467899675908,253.009457808401,19.980592445341)) ;
#90743=CARTESIAN_POINT('Ctrl Pts',(59.3193997901315,253.042430552049,19.9947644309334)) ;
#90744=CARTESIAN_POINT('Ctrl Pts',(59.3942833353535,253.074920165588,20.0046546110925)) ;
#90745=CARTESIAN_POINT('Ctrl Pts',(59.4697367320825,253.107111524934,20.0112252313073)) ;
#90746=CARTESIAN_POINT('Ctrl Pts',(59.4792622083269,253.111175464293,20.0120547272542)) ;
#90747=CARTESIAN_POINT('Ctrl Pts',(59.4887968912323,253.115234454755,20.0128312408816)) ;
#90748=CARTESIAN_POINT('Ctrl Pts',(59.4983287695347,253.119280138962,20.01355466622)) ;
#90749=CARTESIAN_POINT('Ctrl Pts',(59.5618746248842,253.146251367004,20.0183775018095)) ;
#90750=CARTESIAN_POINT('Ctrl Pts',(59.6258593253504,253.172858346708,20.0208838985848)) ;
#90751=CARTESIAN_POINT('Ctrl Pts',(59.6906214872845,253.198122842305,20.0212707200625)) ;
#90752=CARTESIAN_POINT('Origin',(59.695235655795,253.2,20.1326604265405)) ;
#90753=CARTESIAN_POINT('Origin',(66.25,251.8,20.0213203435596)) ;
#90754=CARTESIAN_POINT('',(57.7535453536325,253.,20.0213203435596)) ;
#90755=CARTESIAN_POINT('Origin',(49.257090707265,252.,19.0213203435596)) ;
#90756=CARTESIAN_POINT('',(59.4538479685896,252.944303048062,19.965623391622)) ;
#90757=CARTESIAN_POINT('Ctrl Pts',(59.4538479685897,252.944303048062,19.965623391622)) ;
#90758=CARTESIAN_POINT('Ctrl Pts',(59.4795957437549,252.949199657807,19.9705200013664)) ;
#90759=CARTESIAN_POINT('Ctrl Pts',(59.5039155081045,252.953845010205,19.9751653550366)) ;
#90760=CARTESIAN_POINT('Ctrl Pts',(59.5551459406205,252.9637107836,19.9850311284307)) ;
#90761=CARTESIAN_POINT('Ctrl Pts',(59.5822031562559,252.968956670847,19.9902770144069)) ;
#90762=CARTESIAN_POINT('Ctrl Pts',(59.60747650753,252.973908029254,19.9952283728131)) ;
#90763=CARTESIAN_POINT('',(59.0238256449734,252.853553390593,19.8748737341529)) ;
#90764=CARTESIAN_POINT('Ctrl Pts',(59.4538479685896,252.944303048062,19.965623391622)) ;
#90765=CARTESIAN_POINT('Ctrl Pts',(59.3652369852379,252.927451362751,19.9487717063111)) ;
#90766=CARTESIAN_POINT('Ctrl Pts',(59.3092068635467,252.917036967626,19.9383573111849)) ;
#90767=CARTESIAN_POINT('Ctrl Pts',(59.1694500968853,252.888903295121,19.91022363868)) ;
#90768=CARTESIAN_POINT('Ctrl Pts',(59.096657519322,252.8730579694,19.8943783129598)) ;
#90769=CARTESIAN_POINT('Ctrl Pts',(59.0254737954579,252.853996221768,19.8753165653275)) ;
#90770=CARTESIAN_POINT('Ctrl Pts',(59.0246496511332,252.853775036505,19.8750953800646)) ;
#90771=CARTESIAN_POINT('Ctrl Pts',(59.0238256449756,252.853553390593,19.874873734153)) ;
#90772=CARTESIAN_POINT('',(58.7659637180533,252.658578643763,19.6798989873223)) ;
#90773=CARTESIAN_POINT('Origin',(59.3208772194954,252.658578643763,19.6798989873223)) ;
#90774=CARTESIAN_POINT('',(58.508445556536,252.390759755785,19.4120800993443)) ;
#90775=CARTESIAN_POINT('',(57.5854307313793,251.430824337622,18.4521446811814)) ;
#90776=CARTESIAN_POINT('',(58.3670916964374,252.229977120843,19.2512974644025)) ;
#90777=CARTESIAN_POINT('Ctrl Pts',(58.3670916964374,252.229977120843,19.2512974644025)) ;
#90778=CARTESIAN_POINT('Ctrl Pts',(58.3959491235504,252.259719824999,19.2810401685591)) ;
#90779=CARTESIAN_POINT('Ctrl Pts',(58.4427197527521,252.313512630762,19.3348329743217)) ;
#90780=CARTESIAN_POINT('Ctrl Pts',(58.4869349700687,252.368388745859,19.3897090894184)) ;
#90781=CARTESIAN_POINT('Ctrl Pts',(58.508445556536,252.390759755785,19.4120800993443)) ;
#90782=CARTESIAN_POINT('',(57.3882337581722,251.21966991411,18.2409902576697)) ;
#90783=CARTESIAN_POINT('Origin',(62.771739895016,256.247475826304,23.2687961698638)) ;
#90784=CARTESIAN_POINT('',(46.,251.21966991411,18.2409902576697)) ;
#90785=CARTESIAN_POINT('',(52.2356360608974,251.21966991411,18.2409902576697)) ;
#90786=CARTESIAN_POINT('',(46.,252.270294372515,19.2916147160749)) ;
#90787=CARTESIAN_POINT('',(46.,249.975,16.9963203435596)) ;
#90788=CARTESIAN_POINT('',(43.4,252.270294372515,19.2916147160749)) ;
#90789=CARTESIAN_POINT('',(44.7285453536325,252.270294372515,19.2916147160749)) ;
#90790=CARTESIAN_POINT('',(43.4,252.670710678119,19.6920310216783)) ;
#90791=CARTESIAN_POINT('',(43.4,254.65,21.6713203435596)) ;
#90792=CARTESIAN_POINT('',(43.4621585770309,252.85355339061,19.8748737341699)) ;
#90793=CARTESIAN_POINT('Origin',(43.7,252.670710678119,19.6920310216783)) ;
#90794=CARTESIAN_POINT('',(47.7791083033805,252.853553390593,19.8748737341529)) ;
#90795=CARTESIAN_POINT('',(52.2356360608974,252.853553390593,19.8748737341529)) ;
#90796=CARTESIAN_POINT('',(54.6208916966195,252.853553390593,19.8748737341529)) ;
#90797=CARTESIAN_POINT('Origin',(51.2,255.853553390593,22.8748737341529)) ;
#90798=CARTESIAN_POINT('',(52.2356360608974,252.853553390593,19.8748737341529)) ;
#90799=CARTESIAN_POINT('Ctrl Pts',(34.7000000219136,245.200029079685,18.9812108522455)) ;
#90800=CARTESIAN_POINT('Ctrl Pts',(34.7000093384897,245.17006613755,18.9811792211247)) ;
#90801=CARTESIAN_POINT('Ctrl Pts',(34.6748288409442,245.118261285358,19.0666706061063)) ;
#90802=CARTESIAN_POINT('Ctrl Pts',(34.6224243037673,245.1,19.2450088782142)) ;
#90803=CARTESIAN_POINT('Ctrl Pts',(34.6,245.1,19.3213203435596)) ;
#90804=CARTESIAN_POINT('Ctrl Pts',(34.6999696741166,245.200010627956,19.0440796070764)) ;
#90805=CARTESIAN_POINT('Ctrl Pts',(34.6999676399907,245.18906525137,19.0440605781652)) ;
#90806=CARTESIAN_POINT('Ctrl Pts',(34.7054733072358,245.140987432299,19.095486456445)) ;
#90807=CARTESIAN_POINT('Ctrl Pts',(34.6314054973637,245.1,19.2539900718105)) ;
#90808=CARTESIAN_POINT('Ctrl Pts',(34.6,245.1,19.3213203435596)) ;
#90809=CARTESIAN_POINT('Ctrl Pts',(34.7521917241297,245.199989665103,19.16912861943)) ;
#90810=CARTESIAN_POINT('Ctrl Pts',(34.7521859728801,245.210650489643,19.1691343706795)) ;
#90811=CARTESIAN_POINT('Ctrl Pts',(34.7677441747257,245.164070188481,19.153576168834)) ;
#90812=CARTESIAN_POINT('Ctrl Pts',(34.6493678845564,245.1,19.2719524590032)) ;
#90813=CARTESIAN_POINT('Ctrl Pts',(34.6,245.1,19.3213203435596)) ;
#90814=CARTESIAN_POINT('Ctrl Pts',(34.8772407364833,245.200010627956,19.221350669443)) ;
#90815=CARTESIAN_POINT('Ctrl Pts',(34.8772597653945,245.18906525137,19.2213527035689)) ;
#90816=CARTESIAN_POINT('Ctrl Pts',(34.8258338871147,245.140987432298,19.2158470363238)) ;
#90817=CARTESIAN_POINT('Ctrl Pts',(34.6673302717491,245.1,19.2899148461959)) ;
#90818=CARTESIAN_POINT('Ctrl Pts',(34.6,245.1,19.3213203435596)) ;
#90819=CARTESIAN_POINT('Ctrl Pts',(34.9401094913142,245.200029079685,19.2213203216461)) ;
#90820=CARTESIAN_POINT('Ctrl Pts',(34.940141122435,245.17006613755,19.2213110050699)) ;
#90821=CARTESIAN_POINT('Ctrl Pts',(34.8546497374533,245.118261285358,19.2464915026154)) ;
#90822=CARTESIAN_POINT('Ctrl Pts',(34.6763114653455,245.1,19.2988960397923)) ;
#90823=CARTESIAN_POINT('Ctrl Pts',(34.6,245.1,19.3213203435596)) ;
#90824=CARTESIAN_POINT('',(34.7,245.2,18.9813203435596)) ;
#90825=CARTESIAN_POINT('',(34.94,245.2,19.2213203435596)) ;
#90826=CARTESIAN_POINT('Origin',(34.94,245.2,18.9813203435596)) ;
#90827=CARTESIAN_POINT('',(34.812048130896,245.121831303122,19.2589532462372)) ;
#90828=CARTESIAN_POINT('Origin',(34.6,245.2,19.3213203435596)) ;
#90829=CARTESIAN_POINT('',(34.6,245.1,19.3213203435596)) ;
#90830=CARTESIAN_POINT('Origin',(34.6,245.2,19.3213203435596)) ;
#90831=CARTESIAN_POINT('',(34.6623670973224,245.121831303122,19.1092722126636)) ;
#90832=CARTESIAN_POINT('Origin',(34.6,245.2,19.3213203435596)) ;
#90833=CARTESIAN_POINT('Origin',(34.6,245.2,19.3213203435596)) ;
#90834=CARTESIAN_POINT('Origin',(34.94,252.4,18.9813203435596)) ;
#90835=CARTESIAN_POINT('',(34.7,251.535735931288,18.9813203435596)) ;
#90836=CARTESIAN_POINT('',(34.94,251.535735931288,19.2213203435596)) ;
#90837=CARTESIAN_POINT('Origin',(34.94,251.535735931288,18.9813203435596)) ;
#90838=CARTESIAN_POINT('',(34.94,252.4,19.2213203435596)) ;
#90839=CARTESIAN_POINT('',(34.7,252.4,18.9813203435596)) ;
#90840=CARTESIAN_POINT('Ctrl Pts',(34.6017339105327,251.97522832562,19.1067953741799)) ;
#90841=CARTESIAN_POINT('Ctrl Pts',(34.6634134588563,251.864241814735,19.0750536538863)) ;
#90842=CARTESIAN_POINT('Ctrl Pts',(34.7000061973417,251.700474278475,19.028221281181)) ;
#90843=CARTESIAN_POINT('Ctrl Pts',(34.7000001095966,251.535435370687,18.9810436611381)) ;
#90844=CARTESIAN_POINT('Ctrl Pts',(34.6185891138952,251.988340545982,19.1416152707518)) ;
#90845=CARTESIAN_POINT('Ctrl Pts',(34.6820644896349,251.871454352969,19.118504383798)) ;
#90846=CARTESIAN_POINT('Ctrl Pts',(34.7125874913099,251.700356151572,19.0833081167134)) ;
#90847=CARTESIAN_POINT('Ctrl Pts',(34.6999241628191,251.535435577959,19.0439540541464)) ;
#90848=CARTESIAN_POINT('Ctrl Pts',(34.6666204996312,252.025705917447,19.1999857849512)) ;
#90849=CARTESIAN_POINT('Ctrl Pts',(34.7426835812045,251.897727354795,19.1933392410231)) ;
#90850=CARTESIAN_POINT('Ctrl Pts',(34.7752829676017,251.710693056027,19.1828544398397)) ;
#90851=CARTESIAN_POINT('Ctrl Pts',(34.752107940643,251.535416712293,19.1690554827065)) ;
#90852=CARTESIAN_POINT('Ctrl Pts',(34.7310058064877,252.075793529964,19.2213202461027)) ;
#90853=CARTESIAN_POINT('Ctrl Pts',(34.8303563319875,251.937975750104,19.2213739807519)) ;
#90854=CARTESIAN_POINT('Ctrl Pts',(34.8851586497759,251.735194021102,19.2210635103389)) ;
#90855=CARTESIAN_POINT('Ctrl Pts',(34.8771536379644,251.535372020486,19.2213208115184)) ;
#90856=CARTESIAN_POINT('Ctrl Pts',(34.7632130987747,252.100848735699,19.2213203435596)) ;
#90857=CARTESIAN_POINT('Ctrl Pts',(34.8742461148383,251.958128788049,19.2213203435596)) ;
#90858=CARTESIAN_POINT('Ctrl Pts',(34.9400799458861,251.747541937871,19.2213203435596)) ;
#90859=CARTESIAN_POINT('Ctrl Pts',(34.9399999271389,251.535349497,19.2213203435596)) ;
#90860=CARTESIAN_POINT('',(34.6018973652929,251.975065897532,19.1068431910579)) ;
#90861=CARTESIAN_POINT('',(34.7634152575273,252.100588745031,19.2213203435596)) ;
#90862=CARTESIAN_POINT('Origin',(34.7634152575273,252.100588745031,18.9813203435596)) ;
#90863=CARTESIAN_POINT('Origin',(34.4,251.535735931288,19.2213203435596)) ;
#90864=CARTESIAN_POINT('Origin',(34.4,251.535735931288,18.9813203435596)) ;
#90865=CARTESIAN_POINT('Ctrl Pts',(34.7634152575273,252.100588745031,19.2213203435596)) ;
#90866=CARTESIAN_POINT('Ctrl Pts',(34.6573341599048,252.168839249362,19.2213203435596)) ;
#90867=CARTESIAN_POINT('Ctrl Pts',(34.528261189473,252.227295182387,19.2491278924933)) ;
#90868=CARTESIAN_POINT('Ctrl Pts',(34.4017755136714,252.269701879201,19.2910234275852)) ;
#90869=CARTESIAN_POINT('Ctrl Pts',(34.4008872944232,252.269998607705,19.2913189512647)) ;
#90870=CARTESIAN_POINT('Ctrl Pts',(34.4,252.270294372515,19.2916147160749)) ;
#90871=CARTESIAN_POINT('Ctrl Pts',(34.6989581230585,252.050496195232,19.2213203435596)) ;
#90872=CARTESIAN_POINT('Ctrl Pts',(34.6197281326642,252.126885662221,19.2061907587185)) ;
#90873=CARTESIAN_POINT('Ctrl Pts',(34.5092623007076,252.213208210922,19.2345935259517)) ;
#90874=CARTESIAN_POINT('Ctrl Pts',(34.401512470054,252.269502550543,19.2908287731336)) ;
#90875=CARTESIAN_POINT('Ctrl Pts',(34.4007558433964,252.269900019436,19.2912203629956)) ;
#90876=CARTESIAN_POINT('Ctrl Pts',(34.4,252.270294372515,19.2916147160749)) ;
#90877=CARTESIAN_POINT('Ctrl Pts',(34.6356092113767,252.001264895404,19.1764212743414)) ;
#90878=CARTESIAN_POINT('Ctrl Pts',(34.5811287956459,252.097389804567,19.177622597453)) ;
#90879=CARTESIAN_POINT('Ctrl Pts',(34.4903264917909,252.198996115397,19.2204192832181)) ;
#90880=CARTESIAN_POINT('Ctrl Pts',(34.4012491049424,252.269305008193,19.290631181609)) ;
#90881=CARTESIAN_POINT('Ctrl Pts',(34.4006243923697,252.269801431167,19.2911217747264)) ;
#90882=CARTESIAN_POINT('Ctrl Pts',(34.4,252.270294372515,19.2916147160749)) ;
#90883=CARTESIAN_POINT('Ctrl Pts',(34.6018973652929,251.975065897532,19.106843191058)) ;
#90884=CARTESIAN_POINT('Ctrl Pts',(34.5429634221693,252.081233348715,19.1371767485388)) ;
#90885=CARTESIAN_POINT('Ctrl Pts',(34.4712562163731,252.184523710722,19.2064133504464)) ;
#90886=CARTESIAN_POINT('Ctrl Pts',(34.4009863964841,252.269109921364,19.2904316036179)) ;
#90887=CARTESIAN_POINT('Ctrl Pts',(34.4004929413429,252.269702842897,19.2910231864568)) ;
#90888=CARTESIAN_POINT('Ctrl Pts',(34.4,252.270294372515,19.2916147160749)) ;
#90889=CARTESIAN_POINT('',(34.4,252.270294372515,19.2916147160749)) ;
#90890=CARTESIAN_POINT('Ctrl Pts',(34.6018973652929,251.975065897532,19.106843191058)) ;
#90891=CARTESIAN_POINT('Ctrl Pts',(34.5429634221693,252.081233348715,19.1371767485388)) ;
#90892=CARTESIAN_POINT('Ctrl Pts',(34.4712562163731,252.184523710722,19.2064133504464)) ;
#90893=CARTESIAN_POINT('Ctrl Pts',(34.4009863964841,252.269109921364,19.2904316036179)) ;
#90894=CARTESIAN_POINT('Ctrl Pts',(34.4004929413429,252.269702842897,19.2910231864568)) ;
#90895=CARTESIAN_POINT('Ctrl Pts',(34.4,252.270294372515,19.2916147160749)) ;
#90896=CARTESIAN_POINT('Ctrl Pts',(34.4,252.270294372515,19.2916147160749)) ;
#90897=CARTESIAN_POINT('Ctrl Pts',(34.4008872944232,252.269998607705,19.2913189512647)) ;
#90898=CARTESIAN_POINT('Ctrl Pts',(34.4017755136714,252.269701879201,19.2910234275852)) ;
#90899=CARTESIAN_POINT('Ctrl Pts',(34.528261189473,252.227295182387,19.2491278924933)) ;
#90900=CARTESIAN_POINT('Ctrl Pts',(34.6573341599048,252.168839249362,19.2213203435596)) ;
#90901=CARTESIAN_POINT('Ctrl Pts',(34.7634152575273,252.100588745031,19.2213203435596)) ;
#90902=CARTESIAN_POINT('Origin',(34.4,252.262867965644,19.7084523779156)) ;
#90903=CARTESIAN_POINT('',(34.7,251.007537879754,18.4531222920257)) ;
#90904=CARTESIAN_POINT('',(34.7,252.262867965644,19.7084523779156)) ;
#90905=CARTESIAN_POINT('',(34.4,251.21966991411,18.2409902576697)) ;
#90906=CARTESIAN_POINT('Origin',(34.4,251.007537879754,18.4531222920257)) ;
#90907=CARTESIAN_POINT('',(34.4,252.475,19.4963203435596)) ;
#90908=CARTESIAN_POINT('Origin',(34.7,254.9,18.0213203435596)) ;
#90909=CARTESIAN_POINT('',(34.7,245.2,18.3213203435596)) ;
#90910=CARTESIAN_POINT('',(34.7,245.2,23.7713203435596)) ;
#90911=CARTESIAN_POINT('',(34.7,250.68933982822,18.3213203435596)) ;
#90912=CARTESIAN_POINT('',(34.7,251.975,18.3213203435596)) ;
#90913=CARTESIAN_POINT('Origin',(34.7,250.68933982822,18.7713203435596)) ;
#90914=CARTESIAN_POINT('Origin',(34.6,245.2,23.7713203435596)) ;
#90915=CARTESIAN_POINT('',(34.6,245.1,18.3213203435596)) ;
#90916=CARTESIAN_POINT('',(34.6,245.1,23.7713203435596)) ;
#90917=CARTESIAN_POINT('Origin',(34.6,245.2,18.3213203435596)) ;
#90918=CARTESIAN_POINT('Ctrl Pts',(45.8,245.1,19.3213203435596)) ;
#90919=CARTESIAN_POINT('Ctrl Pts',(45.7701101736509,245.1,19.2195624777583)) ;
#90920=CARTESIAN_POINT('Ctrl Pts',(45.7183540340142,245.125062832338,19.0433988064518)) ;
#90921=CARTESIAN_POINT('Ctrl Pts',(45.6999901429942,245.177552241659,18.9811290612227)) ;
#90922=CARTESIAN_POINT('Ctrl Pts',(45.6999999540947,245.200041989469,18.9811623295317)) ;
#90923=CARTESIAN_POINT('Ctrl Pts',(45.8,245.1,19.3213203435596)) ;
#90924=CARTESIAN_POINT('Ctrl Pts',(45.7581321670755,245.1,19.2315404843337)) ;
#90925=CARTESIAN_POINT('Ctrl Pts',(45.6904763225037,245.153565681928,19.0780179164569)) ;
#90926=CARTESIAN_POINT('Ctrl Pts',(45.7000488684854,245.19180184345,19.0440292695842)) ;
#90927=CARTESIAN_POINT('Ctrl Pts',(45.7000437609983,245.200015344509,19.0440474324887)) ;
#90928=CARTESIAN_POINT('Ctrl Pts',(45.8,245.1,19.3213203435596)) ;
#90929=CARTESIAN_POINT('Ctrl Pts',(45.7341761539248,245.1,19.2554964974844)) ;
#90930=CARTESIAN_POINT('Ctrl Pts',(45.6263979131407,245.183234588789,19.1477182567004)) ;
#90931=CARTESIAN_POINT('Ctrl Pts',(45.6478283493969,245.207992331203,19.1691486929565)) ;
#90932=CARTESIAN_POINT('Ctrl Pts',(45.6478169119502,245.199985071692,19.1691372555099)) ;
#90933=CARTESIAN_POINT('Ctrl Pts',(45.8,245.1,19.3213203435596)) ;
#90934=CARTESIAN_POINT('Ctrl Pts',(45.710220140774,245.1,19.2794525106351)) ;
#90935=CARTESIAN_POINT('Ctrl Pts',(45.5566975728973,245.153565681928,19.2117966660634)) ;
#90936=CARTESIAN_POINT('Ctrl Pts',(45.5227089260246,245.19180184345,19.221369212045)) ;
#90937=CARTESIAN_POINT('Ctrl Pts',(45.522727088929,245.200015344509,19.2213641045579)) ;
#90938=CARTESIAN_POINT('Ctrl Pts',(45.8,245.1,19.3213203435596)) ;
#90939=CARTESIAN_POINT('Ctrl Pts',(45.6982421341987,245.1,19.2914305172105)) ;
#90940=CARTESIAN_POINT('Ctrl Pts',(45.5220784628922,245.125062832338,19.2396743775738)) ;
#90941=CARTESIAN_POINT('Ctrl Pts',(45.4598087176631,245.177552241659,19.2213104865538)) ;
#90942=CARTESIAN_POINT('Ctrl Pts',(45.459841985972,245.200041989469,19.2213202976544)) ;
#90943=CARTESIAN_POINT('',(45.46,245.2,19.2213203435596)) ;
#90944=CARTESIAN_POINT('',(45.7,245.2,18.9813203435596)) ;
#90945=CARTESIAN_POINT('Origin',(45.46,245.2,18.9813203435596)) ;
#90946=CARTESIAN_POINT('',(45.7337685111545,245.125077440745,19.0961332814849)) ;
#90947=CARTESIAN_POINT('Origin',(45.8,245.2,19.3213203435596)) ;
#90948=CARTESIAN_POINT('',(45.8,245.1,19.3213203435596)) ;
#90949=CARTESIAN_POINT('Origin',(45.8,245.2,19.3213203435596)) ;
#90950=CARTESIAN_POINT('',(45.5748129379279,245.125077440744,19.2550888547148)) ;
#90951=CARTESIAN_POINT('Origin',(45.8,245.2,19.3213203435596)) ;
#90952=CARTESIAN_POINT('Origin',(45.8,245.2,19.3213203435596)) ;
#90953=CARTESIAN_POINT('Origin',(45.46,247.4,18.9813203435596)) ;
#90954=CARTESIAN_POINT('',(45.46,251.535735931288,19.2213203435596)) ;
#90955=CARTESIAN_POINT('',(45.7,251.535735931288,18.9813203435596)) ;
#90956=CARTESIAN_POINT('Origin',(45.46,251.535735931288,18.9813203435596)) ;
#90957=CARTESIAN_POINT('',(45.7,247.4,18.9813203435596)) ;
#90958=CARTESIAN_POINT('',(45.46,247.4,19.2213203435596)) ;
#90959=CARTESIAN_POINT('Ctrl Pts',(45.6999998904024,251.535435370679,18.9810436611296)) ;
#90960=CARTESIAN_POINT('Ctrl Pts',(45.699993802657,251.700474278472,19.0282212811746)) ;
#90961=CARTESIAN_POINT('Ctrl Pts',(45.7365865411453,251.864241814738,19.0750536538836)) ;
#90962=CARTESIAN_POINT('Ctrl Pts',(45.7982660894715,251.975228325624,19.1067953741784)) ;
#90963=CARTESIAN_POINT('Ctrl Pts',(45.7000758378912,251.535435577951,19.0439540548493)) ;
#90964=CARTESIAN_POINT('Ctrl Pts',(45.6874125093996,251.700356151569,19.083308117419)) ;
#90965=CARTESIAN_POINT('Ctrl Pts',(45.7179355104384,251.871454352916,19.1185043839603)) ;
#90966=CARTESIAN_POINT('Ctrl Pts',(45.7814108861818,251.98834054593,19.1416152709156)) ;
#90967=CARTESIAN_POINT('Ctrl Pts',(45.647891359541,251.535416712284,19.1690547828863)) ;
#90968=CARTESIAN_POINT('Ctrl Pts',(45.6247163318147,251.710693055956,19.1828537393655)) ;
#90969=CARTESIAN_POINT('Ctrl Pts',(45.6573163478517,251.897727410595,19.1933390793962)) ;
#90970=CARTESIAN_POINT('Ctrl Pts',(45.7333794286637,252.025705973181,19.1999856226698)) ;
#90971=CARTESIAN_POINT('Ctrl Pts',(45.522846362036,251.535372020476,19.2213208115184)) ;
#90972=CARTESIAN_POINT('Ctrl Pts',(45.5148413502221,251.735194021099,19.2210635103388)) ;
#90973=CARTESIAN_POINT('Ctrl Pts',(45.5696436680127,251.937975750109,19.2213739807519)) ;
#90974=CARTESIAN_POINT('Ctrl Pts',(45.6689941935172,252.075793529971,19.2213202461027)) ;
#90975=CARTESIAN_POINT('Ctrl Pts',(45.4600000728611,251.535349496989,19.2213203435596)) ;
#90976=CARTESIAN_POINT('Ctrl Pts',(45.4599200541118,251.747541937868,19.2213203435596)) ;
#90977=CARTESIAN_POINT('Ctrl Pts',(45.525753885162,251.958128788054,19.2213203435596)) ;
#90978=CARTESIAN_POINT('Ctrl Pts',(45.6367869012307,252.100848735706,19.2213203435596)) ;
#90979=CARTESIAN_POINT('',(45.6365847424727,252.100588745031,19.2213203435596)) ;
#90980=CARTESIAN_POINT('',(45.798102634707,251.975065897532,19.1068431910579)) ;
#90981=CARTESIAN_POINT('Origin',(45.6365847424727,252.100588745031,18.9813203435596)) ;
#90982=CARTESIAN_POINT('Origin',(46.,251.535735931288,18.9813203435596)) ;
#90983=CARTESIAN_POINT('Origin',(46.,251.535735931288,19.2213203435596)) ;
#90984=CARTESIAN_POINT('Ctrl Pts',(46.,252.270294372515,19.2916147160749)) ;
#90985=CARTESIAN_POINT('Ctrl Pts',(45.9991127055774,252.269998607706,19.2913189512654)) ;
#90986=CARTESIAN_POINT('Ctrl Pts',(45.9982244863323,252.269701879202,19.2910234275873)) ;
#90987=CARTESIAN_POINT('Ctrl Pts',(45.87173880933,252.22729518208,19.2491278919541)) ;
#90988=CARTESIAN_POINT('Ctrl Pts',(45.7426658400944,252.168839249362,19.2213203435596)) ;
#90989=CARTESIAN_POINT('Ctrl Pts',(45.6365847424727,252.100588745031,19.2213203435596)) ;
#90990=CARTESIAN_POINT('Ctrl Pts',(46.,252.270294372515,19.2916147160749)) ;
#90991=CARTESIAN_POINT('Ctrl Pts',(45.9992432480265,252.269899128634,19.2912194721931)) ;
#90992=CARTESIAN_POINT('Ctrl Pts',(45.9984881400231,252.269484042833,19.2908487161059)) ;
#90993=CARTESIAN_POINT('Ctrl Pts',(45.8908075064141,252.213536269908,19.2342664523398)) ;
#90994=CARTESIAN_POINT('Ctrl Pts',(45.7804734503348,252.127653985431,19.205962938089)) ;
#90995=CARTESIAN_POINT('Ctrl Pts',(45.7010418769414,252.050496195232,19.2213203435596)) ;
#90996=CARTESIAN_POINT('Ctrl Pts',(46.,252.270294372515,19.2916147160749)) ;
#90997=CARTESIAN_POINT('Ctrl Pts',(45.9993751441279,252.269800058411,19.2911204019704)) ;
#90998=CARTESIAN_POINT('Ctrl Pts',(45.9987511914088,252.269287284606,19.290651085124)) ;
#90999=CARTESIAN_POINT('Ctrl Pts',(45.9096857659592,252.199356446256,19.2201402522094)) ;
#91000=CARTESIAN_POINT('Ctrl Pts',(45.8192755842025,252.09797381701,19.1772675246916)) ;
#91001=CARTESIAN_POINT('Ctrl Pts',(45.7643907886233,252.001264895404,19.1764212743414)) ;
#91002=CARTESIAN_POINT('Ctrl Pts',(46.,252.270294372515,19.2916147160749)) ;
#91003=CARTESIAN_POINT('Ctrl Pts',(45.9995070586569,252.269702842898,19.2910231864577)) ;
#91004=CARTESIAN_POINT('Ctrl Pts',(45.999013603518,252.269109921366,19.2904316036215)) ;
#91005=CARTESIAN_POINT('Ctrl Pts',(45.9287437829605,252.184523710006,19.2064133494711)) ;
#91006=CARTESIAN_POINT('Ctrl Pts',(45.8570365778302,252.081233348715,19.1371767485386)) ;
#91007=CARTESIAN_POINT('Ctrl Pts',(45.798102634707,251.975065897532,19.106843191058)) ;
#91008=CARTESIAN_POINT('',(45.9943955116219,252.2684153652,19.2897579022715)) ;
#91009=CARTESIAN_POINT('Ctrl Pts',(45.6365847424727,252.100588745031,19.2213203435596)) ;
#91010=CARTESIAN_POINT('Ctrl Pts',(45.7418374703499,252.168306292463,19.2213203435596)) ;
#91011=CARTESIAN_POINT('Ctrl Pts',(45.8697243923924,252.226381639409,19.2486952985084)) ;
#91012=CARTESIAN_POINT('Ctrl Pts',(45.9943955116219,252.2684153652,19.2897579022714)) ;
#91013=CARTESIAN_POINT('Ctrl Pts',(45.9943955116219,252.2684153652,19.2897579022714)) ;
#91014=CARTESIAN_POINT('Ctrl Pts',(45.9953767097843,252.268746182913,19.2900810769698)) ;
#91015=CARTESIAN_POINT('Ctrl Pts',(45.996357708755,252.269076006983,19.2904050995018)) ;
#91016=CARTESIAN_POINT('Ctrl Pts',(45.9982244863323,252.269701879202,19.2910234275873)) ;
#91017=CARTESIAN_POINT('Ctrl Pts',(45.9991127055774,252.269998607706,19.2913189512654)) ;
#91018=CARTESIAN_POINT('Ctrl Pts',(46.,252.270294372515,19.2916147160749)) ;
#91019=CARTESIAN_POINT('',(45.996886678812,252.266546563962,19.287891562564)) ;
#91020=CARTESIAN_POINT('Ctrl Pts',(46.,252.270294372515,19.2916147160749)) ;
#91021=CARTESIAN_POINT('Ctrl Pts',(45.9995070586569,252.269702842898,19.2910231864577)) ;
#91022=CARTESIAN_POINT('Ctrl Pts',(45.999013603518,252.269109921366,19.2904316036215)) ;
#91023=CARTESIAN_POINT('Ctrl Pts',(45.9979765993132,252.267861643568,19.2891917074307)) ;
#91024=CARTESIAN_POINT('Ctrl Pts',(45.9974316943751,252.267204687989,19.2885411965337)) ;
#91025=CARTESIAN_POINT('Ctrl Pts',(45.996886678812,252.266546563962,19.287891562564)) ;
#91026=CARTESIAN_POINT('Ctrl Pts',(45.996886678812,252.266546563962,19.287891562564)) ;
#91027=CARTESIAN_POINT('Ctrl Pts',(45.9276248562919,252.182910659558,19.20533459398)) ;
#91028=CARTESIAN_POINT('Ctrl Pts',(45.8565764521882,252.080404448356,19.1369399198645)) ;
#91029=CARTESIAN_POINT('Ctrl Pts',(45.798102634707,251.975065897532,19.106843191058)) ;
#91030=CARTESIAN_POINT('Origin',(40.2,249.9,19.2213203435596)) ;
#91031=CARTESIAN_POINT('',(37.,252.100588745031,19.2213203435596)) ;
#91032=CARTESIAN_POINT('',(44.7285453536325,252.100588745031,19.2213203435596)) ;
#91033=CARTESIAN_POINT('',(37.,252.1,19.2213203435596)) ;
#91034=CARTESIAN_POINT('',(37.,254.9,19.2213203435596)) ;
#91035=CARTESIAN_POINT('',(37.3,251.8,19.2213203435596)) ;
#91036=CARTESIAN_POINT('Origin',(37.3,252.1,19.2213203435596)) ;
#91037=CARTESIAN_POINT('',(43.1,251.8,19.2213203435596)) ;
#91038=CARTESIAN_POINT('',(38.75,251.8,19.2213203435596)) ;
#91039=CARTESIAN_POINT('',(43.4,252.1,19.2213203435596)) ;
#91040=CARTESIAN_POINT('Origin',(43.1,252.1,19.2213203435596)) ;
#91041=CARTESIAN_POINT('',(43.4,252.100588745031,19.2213203435596)) ;
#91042=CARTESIAN_POINT('',(43.4,251.,19.2213203435596)) ;
#91043=CARTESIAN_POINT('',(44.7285453536325,252.100588745031,19.2213203435596)) ;
#91044=CARTESIAN_POINT('',(41.6,245.2,19.2213203435596)) ;
#91045=CARTESIAN_POINT('',(47.7786796564403,245.2,19.2213203435596)) ;
#91046=CARTESIAN_POINT('',(41.6000000000001,242.9,19.2213203435596)) ;
#91047=CARTESIAN_POINT('',(41.6,246.4,19.2213203435596)) ;
#91048=CARTESIAN_POINT('',(38.8,242.9,19.2213203435596)) ;
#91049=CARTESIAN_POINT('Origin',(40.2,242.9,19.2213203435596)) ;
#91050=CARTESIAN_POINT('',(38.8,245.2,19.2213203435596)) ;
#91051=CARTESIAN_POINT('',(38.8,247.5,19.2213203435596)) ;
#91052=CARTESIAN_POINT('',(47.7786796564403,245.2,19.2213203435596)) ;
#91053=CARTESIAN_POINT('Origin',(47.7786796564403,245.2,19.3213203435596)) ;
#91054=CARTESIAN_POINT('',(41.7,245.1,19.3213203435596)) ;
#91055=CARTESIAN_POINT('',(47.7786796564403,245.1,19.3213203435596)) ;
#91056=CARTESIAN_POINT('Origin',(41.6,245.2,19.3213203435596)) ;
#91057=CARTESIAN_POINT('Origin',(45.8,245.2,23.7713203435596)) ;
#91058=CARTESIAN_POINT('',(45.7,245.2,18.3213203435596)) ;
#91059=CARTESIAN_POINT('',(45.7,245.2,23.7713203435596)) ;
#91060=CARTESIAN_POINT('',(45.8,245.1,18.3213203435596)) ;
#91061=CARTESIAN_POINT('Origin',(45.8,245.2,18.3213203435596)) ;
#91062=CARTESIAN_POINT('',(45.8,245.1,23.7713203435596)) ;
#91063=CARTESIAN_POINT('Ctrl Pts',(79.19990306123,263.55551337303,30.6183190664329)) ;
#91064=CARTESIAN_POINT('Ctrl Pts',(79.2026802545332,263.681247332211,30.6199053561371)) ;
#91065=CARTESIAN_POINT('Ctrl Pts',(79.088180181727,263.8,30.5545045090528)) ;
#91066=CARTESIAN_POINT('Ctrl Pts',(78.96,263.8,30.4813203435596)) ;
#91067=CARTESIAN_POINT('Ctrl Pts',(79.2008868874385,263.554884893925,30.6492315412213)) ;
#91068=CARTESIAN_POINT('Ctrl Pts',(79.203944249311,263.698638059625,30.6513250951561)) ;
#91069=CARTESIAN_POINT('Ctrl Pts',(79.0777524976478,263.8,30.564932193132)) ;
#91070=CARTESIAN_POINT('Ctrl Pts',(78.96,263.8,30.4813203435596)) ;
#91071=CARTESIAN_POINT('Ctrl Pts',(79.1753437943954,263.554337258733,30.7036056868826)) ;
#91072=CARTESIAN_POINT('Ctrl Pts',(79.178220382535,263.713791744552,30.7065917747161)) ;
#91073=CARTESIAN_POINT('Ctrl Pts',(79.0594215416058,263.8,30.5832631491739)) ;
#91074=CARTESIAN_POINT('Ctrl Pts',(78.96,263.8,30.4813203435596)) ;
#91075=CARTESIAN_POINT('Ctrl Pts',(79.1204172721867,263.555043591858,30.7219456941975)) ;
#91076=CARTESIAN_POINT('Ctrl Pts',(79.122387689755,263.694246708396,30.7249347311953)) ;
#91077=CARTESIAN_POINT('Ctrl Pts',(79.0410905855638,263.8,30.6015941052159)) ;
#91078=CARTESIAN_POINT('Ctrl Pts',(78.96,263.8,30.4813203435596)) ;
#91079=CARTESIAN_POINT('Ctrl Pts',(79.0970093616256,263.555512320864,30.7212251114454)) ;
#91080=CARTESIAN_POINT('Ctrl Pts',(79.0985958367215,263.681276446828,30.7240024241314)) ;
#91081=CARTESIAN_POINT('Ctrl Pts',(79.0331873136011,263.8,30.6094973771787)) ;
#91082=CARTESIAN_POINT('Ctrl Pts',(78.96,263.8,30.4813203435596)) ;
#91083=CARTESIAN_POINT('',(79.2,263.56,30.6213203435596)) ;
#91084=CARTESIAN_POINT('',(78.96,263.8,30.4813203435596)) ;
#91085=CARTESIAN_POINT('Origin',(78.96,263.56,30.4813203435596)) ;
#91086=CARTESIAN_POINT('',(79.1,263.56,30.7213203435596)) ;
#91087=CARTESIAN_POINT('Origin',(78.96,263.56,30.4813203435596)) ;
#91088=CARTESIAN_POINT('Origin',(79.1,263.56,30.6213203435596)) ;
#91089=CARTESIAN_POINT('Origin',(80.5421241520375,263.56,30.4813203435596)) ;
#91090=CARTESIAN_POINT('',(78.7,263.8,30.4813203435596)) ;
#91091=CARTESIAN_POINT('',(80.5421241520375,263.8,30.4813203435596)) ;
#91092=CARTESIAN_POINT('',(78.7,263.56,30.7213203435596)) ;
#91093=CARTESIAN_POINT('Origin',(78.7,263.56,30.4813203435596)) ;
#91094=CARTESIAN_POINT('',(80.5421241520375,263.56,30.7213203435596)) ;
#91095=CARTESIAN_POINT('Origin',(78.96,263.56,30.1213203435596)) ;
#91096=CARTESIAN_POINT('',(79.2,263.56,22.4577516938163)) ;
#91097=CARTESIAN_POINT('',(79.2,263.56,30.1213203435596)) ;
#91098=CARTESIAN_POINT('',(79.1755756290597,263.665485298291,22.6717108729184)) ;
#91099=CARTESIAN_POINT('Ctrl Pts',(79.2,263.56,22.4577516938161)) ;
#91100=CARTESIAN_POINT('Ctrl Pts',(79.2,263.560387113803,22.4580922726939)) ;
#91101=CARTESIAN_POINT('Ctrl Pts',(79.1999990633892,263.560773655608,22.458433496925)) ;
#91102=CARTESIAN_POINT('Ctrl Pts',(79.1998704864085,263.587384235686,22.4820045990841)) ;
#91103=CARTESIAN_POINT('Ctrl Pts',(79.1954682388742,263.609945987182,22.5073822183424)) ;
#91104=CARTESIAN_POINT('Ctrl Pts',(79.1861715042083,263.641598026275,22.5602671403111)) ;
#91105=CARTESIAN_POINT('Ctrl Pts',(79.1817919077629,263.651962524966,22.5853229810386)) ;
#91106=CARTESIAN_POINT('Ctrl Pts',(79.176825633249,263.663019660801,22.6314067110977)) ;
#91107=CARTESIAN_POINT('Ctrl Pts',(79.1755756290598,263.665485298291,22.6515196535244)) ;
#91108=CARTESIAN_POINT('Ctrl Pts',(79.1755756290598,263.665485298291,22.6717108732387)) ;
#91109=CARTESIAN_POINT('',(79.1755756290598,263.665485298291,25.7213203435596)) ;
#91110=CARTESIAN_POINT('',(79.1755756290598,263.665485298291,30.1213203435596)) ;
#91111=CARTESIAN_POINT('',(78.96,263.8,25.7213203435596)) ;
#91112=CARTESIAN_POINT('Origin',(78.96,263.56,25.7213203435596)) ;
#91113=CARTESIAN_POINT('',(78.96,263.8,30.1213203435596)) ;
#91114=CARTESIAN_POINT('Origin',(78.7,258.202943725152,30.7213203435596)) ;
#91115=CARTESIAN_POINT('',(78.7,263.8,25.7213203435596)) ;
#91116=CARTESIAN_POINT('',(78.7,263.8,30.7213203435596)) ;
#91117=CARTESIAN_POINT('',(78.7,263.425,25.7213203435596)) ;
#91118=CARTESIAN_POINT('',(78.7,263.8,25.7213203435596)) ;
#91119=CARTESIAN_POINT('',(78.7,263.425,29.5213203435596)) ;
#91120=CARTESIAN_POINT('',(78.7,263.425,30.1213203435596)) ;
#91121=CARTESIAN_POINT('',(78.7,258.061522368915,29.5213203435596)) ;
#91122=CARTESIAN_POINT('',(78.7000000000001,249.459777528085,29.5213203435596)) ;
#91123=CARTESIAN_POINT('',(78.7,258.202943725152,29.6213203435596)) ;
#91124=CARTESIAN_POINT('Origin',(78.7,258.061522368915,29.6213203435596)) ;
#91125=CARTESIAN_POINT('',(78.7,258.202943725152,30.6213203435596)) ;
#91126=CARTESIAN_POINT('',(78.7,258.202943725152,30.7213203435596)) ;
#91127=CARTESIAN_POINT('',(78.7,258.34436508139,30.7213203435596)) ;
#91128=CARTESIAN_POINT('Origin',(78.7,258.34436508139,30.6213203435596)) ;
#91129=CARTESIAN_POINT('',(78.7,263.8,30.7213203435596)) ;
#91130=CARTESIAN_POINT('Origin',(78.7,263.8,30.7213203435596)) ;
#91131=CARTESIAN_POINT('',(77.2,263.8,25.7213203435596)) ;
#91132=CARTESIAN_POINT('Origin',(79.95,259.751471862576,25.7213203435596)) ;
#91133=CARTESIAN_POINT('',(79.04,263.68,25.7213203435596)) ;
#91134=CARTESIAN_POINT('Origin',(79.1,263.6,25.7213203435596)) ;
#91135=CARTESIAN_POINT('',(77.9683532470183,262.876264935264,25.7213203435596)) ;
#91136=CARTESIAN_POINT('Origin',(79.1,263.6,29.5213203435596)) ;
#91137=CARTESIAN_POINT('',(79.04,263.68,22.6717108732387)) ;
#91138=CARTESIAN_POINT('Origin',(79.1,263.6,22.6717108732387)) ;
#91139=CARTESIAN_POINT('',(79.04,263.68,29.5213203435596)) ;
#91140=CARTESIAN_POINT('Origin',(66.56,251.2,19.7813203435596)) ;
#91141=CARTESIAN_POINT('',(66.56,252.24,20.0213203435596)) ;
#91142=CARTESIAN_POINT('',(66.56,251.2,20.0213203435596)) ;
#91143=CARTESIAN_POINT('',(66.8,252.,19.7813203435596)) ;
#91144=CARTESIAN_POINT('Origin',(66.56,252.24,19.7813203435596)) ;
#91145=CARTESIAN_POINT('',(66.8,251.2,19.7813203435596)) ;
#91146=CARTESIAN_POINT('Origin',(66.25,251.8,20.0213203435596)) ;
#91147=CARTESIAN_POINT('',(66.2242118694392,252.575788130571,20.0213203435597)) ;
#91148=CARTESIAN_POINT('Ctrl Pts',(65.94,253.053504693378,20.0213203435596)) ;
#91149=CARTESIAN_POINT('Ctrl Pts',(65.9767477884387,252.96763867409,20.0213203435596)) ;
#91150=CARTESIAN_POINT('Ctrl Pts',(66.0176818440557,252.879704923853,20.0213203435596)) ;
#91151=CARTESIAN_POINT('Ctrl Pts',(66.1031725049829,252.727882430291,20.0213203435596)) ;
#91152=CARTESIAN_POINT('Ctrl Pts',(66.1572502182071,252.642747715263,20.0213203435596)) ;
#91153=CARTESIAN_POINT('Ctrl Pts',(66.2242112157523,252.575788784279,20.0213203435596)) ;
#91154=CARTESIAN_POINT('',(66.7875,252.0125,20.0213203435596)) ;
#91155=CARTESIAN_POINT('Ctrl Pts',(58.600000056816,251.975444989098,19.7811597661928)) ;
#91156=CARTESIAN_POINT('Ctrl Pts',(58.5999555541213,251.975437275298,19.8440457155357)) ;
#91157=CARTESIAN_POINT('Ctrl Pts',(58.6521580208533,251.984485702865,19.9691623227064)) ;
#91158=CARTESIAN_POINT('Ctrl Pts',(58.777274628024,252.006172581441,20.0213647894384)) ;
#91159=CARTESIAN_POINT('Ctrl Pts',(58.840160577367,252.01707281266,20.0213202867436)) ;
#91160=CARTESIAN_POINT('Ctrl Pts',(58.6000000433271,252.000971418317,19.7811775148673)) ;
#91161=CARTESIAN_POINT('Ctrl Pts',(58.5999661067172,252.000962555144,19.8371125691419)) ;
#91162=CARTESIAN_POINT('Ctrl Pts',(58.6397724916797,252.011358835424,19.9486050783821)) ;
#91163=CARTESIAN_POINT('Ctrl Pts',(58.7439794071885,252.03806921914,20.0112711346708)) ;
#91164=CARTESIAN_POINT('Ctrl Pts',(58.8024064475807,252.053375145924,20.0213461160323)) ;
#91165=CARTESIAN_POINT('Ctrl Pts',(58.6099157004014,252.052043043932,19.7812197015128)) ;
#91166=CARTESIAN_POINT('Ctrl Pts',(58.6098983376034,252.052031828423,19.8206333831451)) ;
#91167=CARTESIAN_POINT('Ctrl Pts',(58.630263078444,252.065186724936,19.8994186791738)) ;
#91168=CARTESIAN_POINT('Ctrl Pts',(58.6891074359545,252.101875712154,19.9593347509465)) ;
#91169=CARTESIAN_POINT('Ctrl Pts',(58.727245689281,252.125616817957,19.9778261025138)) ;
#91170=CARTESIAN_POINT('Ctrl Pts',(58.6381785959941,252.095724858518,19.7812690036197)) ;
#91171=CARTESIAN_POINT('Ctrl Pts',(58.6381689240718,252.095714970455,19.8013749227895)) ;
#91172=CARTESIAN_POINT('Ctrl Pts',(58.6495137915443,252.107313265173,19.8414536032633)) ;
#91173=CARTESIAN_POINT('Ctrl Pts',(58.6789249290458,252.137847807203,19.8672326888626)) ;
#91174=CARTESIAN_POINT('Ctrl Pts',(58.6958346094131,252.155752774615,19.8735570199477)) ;
#91175=CARTESIAN_POINT('Ctrl Pts',(58.6559044410999,252.114140580344,19.7812936795923)) ;
#91176=CARTESIAN_POINT('Ctrl Pts',(58.6558970330687,252.114132875287,19.7917359290227)) ;
#91177=CARTESIAN_POINT('Ctrl Pts',(58.6645867897606,252.123171048738,19.8125113086305)) ;
#91178=CARTESIAN_POINT('Ctrl Pts',(58.6854050755849,252.144822345019,19.821142975253)) ;
#91179=CARTESIAN_POINT('Ctrl Pts',(58.6958601680558,252.155694402978,19.8211100731203)) ;
#91180=CARTESIAN_POINT('',(58.6958333870197,252.1556667225,19.8213203435596)) ;
#91181=CARTESIAN_POINT('',(58.8400000000001,252.01704497925,20.0213203435596)) ;
#91182=CARTESIAN_POINT('Origin',(58.84,252.01704497925,19.8213203435596)) ;
#91183=CARTESIAN_POINT('',(58.6,251.97544497925,19.7813203435596)) ;
#91184=CARTESIAN_POINT('Origin',(58.84,252.01704497925,19.7813203435596)) ;
#91185=CARTESIAN_POINT('',(58.6558333870196,252.1140667225,19.7813203435596)) ;
#91186=CARTESIAN_POINT('Origin',(58.8,251.97544497925,19.7813203435596)) ;
#91187=CARTESIAN_POINT('Origin',(58.6958333870196,252.1556667225,19.7813203435596)) ;
#91188=CARTESIAN_POINT('Origin',(58.84,248.1,19.7813203435596)) ;
#91189=CARTESIAN_POINT('',(58.6,248.1,19.7813203435596)) ;
#91190=CARTESIAN_POINT('',(58.84,248.1,20.0213203435596)) ;
#91191=CARTESIAN_POINT('Origin',(58.45,251.9,24.0213203435596)) ;
#91192=CARTESIAN_POINT('',(58.6558333870196,252.1140667225,19.6041630560343)) ;
#91193=CARTESIAN_POINT('',(58.6558333870196,252.1140667225,24.0213203435596)) ;
#91194=CARTESIAN_POINT('',(58.6524986843825,252.11059862929,19.5535233690183)) ;
#91195=CARTESIAN_POINT('Origin',(58.2558333870196,251.6980667225,19.6041630560343)) ;
#91196=CARTESIAN_POINT('',(58.9101303310336,252.378535544275,19.8213203435596)) ;
#91197=CARTESIAN_POINT('',(57.7295973443597,251.150781238134,18.5935660374187)) ;
#91198=CARTESIAN_POINT('',(60.2985780169101,253.822521137587,19.8213203435596)) ;
#91199=CARTESIAN_POINT('Origin',(58.8,251.97544497925,24.0213203435596)) ;
#91200=CARTESIAN_POINT('',(58.6,251.97544497925,19.6041630560343)) ;
#91201=CARTESIAN_POINT('',(58.6,251.97544497925,24.0213203435596)) ;
#91202=CARTESIAN_POINT('Origin',(58.8,251.97544497925,19.6041630560343)) ;
#91203=CARTESIAN_POINT('Origin',(58.6000000000001,244.4,24.0213203435596)) ;
#91204=CARTESIAN_POINT('',(58.6,252.056,23.0213203435596)) ;
#91205=CARTESIAN_POINT('',(58.6,248.1,23.0213203435596)) ;
#91206=CARTESIAN_POINT('',(58.6,252.056,24.0213203435596)) ;
#91207=CARTESIAN_POINT('',(58.6,252.056,24.0213203435596)) ;
#91208=CARTESIAN_POINT('',(58.6,245.4,24.0213203435596)) ;
#91209=CARTESIAN_POINT('',(58.6,250.6,24.0213203435596)) ;
#91210=CARTESIAN_POINT('',(58.6,245.4,19.6041630560343)) ;
#91211=CARTESIAN_POINT('',(58.6,245.4,24.0213203435596)) ;
#91212=CARTESIAN_POINT('',(58.6,245.5625,19.6041630560343)) ;
#91213=CARTESIAN_POINT('Origin',(37.,252.100588745031,19.4613203435596)) ;
#91214=CARTESIAN_POINT('',(37.1,252.100588745031,19.3213203435596)) ;
#91215=CARTESIAN_POINT('Origin',(37.,252.100588745031,19.3213203435596)) ;
#91216=CARTESIAN_POINT('',(37.,252.270294372515,19.2916147160749)) ;
#91217=CARTESIAN_POINT('Origin',(37.,252.100588745031,19.4613203435596)) ;
#91218=CARTESIAN_POINT('',(37.1,252.199583694397,19.3623253941935)) ;
#91219=CARTESIAN_POINT('Origin',(37.,252.199583694397,19.3623253941935)) ;
#91220=CARTESIAN_POINT('Origin',(37.1,252.100588745031,19.4613203435596)) ;
#91221=CARTESIAN_POINT('Origin',(44.7285453536325,252.100588745031,19.4613203435596)) ;
#91222=CARTESIAN_POINT('',(44.7285453536325,252.270294372515,19.2916147160749)) ;
#91223=CARTESIAN_POINT('Origin',(37.,256.529289321881,23.6920310216783)) ;
#91224=CARTESIAN_POINT('',(37.,252.670710678119,19.6920310216783)) ;
#91225=CARTESIAN_POINT('',(37.,256.6,23.6213203435596)) ;
#91226=CARTESIAN_POINT('',(37.1,252.6,19.7627416997969)) ;
#91227=CARTESIAN_POINT('Origin',(37.,252.6,19.7627416997969)) ;
#91228=CARTESIAN_POINT('',(37.1,256.529289321881,23.6920310216783)) ;
#91229=CARTESIAN_POINT('Origin',(49.257090707265,252.,19.0213203435596)) ;
#91230=CARTESIAN_POINT('',(26.4,251.21966991411,18.2409902576697)) ;
#91231=CARTESIAN_POINT('',(52.2356360608974,251.21966991411,18.2409902576697)) ;
#91232=CARTESIAN_POINT('',(26.4,252.853553390593,19.8748737341529)) ;
#91233=CARTESIAN_POINT('',(26.4,253.025,20.0463203435596)) ;
#91234=CARTESIAN_POINT('',(36.9378414229691,252.85355339061,19.8748737341699)) ;
#91235=CARTESIAN_POINT('',(52.2356360608974,252.853553390593,19.8748737341529)) ;
#91236=CARTESIAN_POINT('Origin',(36.7,252.670710678119,19.6920310216783)) ;
#91237=CARTESIAN_POINT('Origin',(43.4,252.100588745031,19.4613203435596)) ;
#91238=CARTESIAN_POINT('',(43.3,252.100588745031,19.3213203435596)) ;
#91239=CARTESIAN_POINT('Origin',(43.4,252.100588745031,19.3213203435596)) ;
#91240=CARTESIAN_POINT('',(43.3,252.199583694397,19.3623253941935)) ;
#91241=CARTESIAN_POINT('Origin',(43.3,252.100588745031,19.4613203435596)) ;
#91242=CARTESIAN_POINT('Origin',(43.4,252.199583694397,19.3623253941935)) ;
#91243=CARTESIAN_POINT('Origin',(43.4,252.100588745031,19.4613203435596)) ;
#91244=CARTESIAN_POINT('Origin',(44.7285453536325,252.100588745031,19.4613203435596)) ;
#91245=CARTESIAN_POINT('Origin',(43.4,251.,19.3213203435596)) ;
#91246=CARTESIAN_POINT('',(43.3,252.1,19.3213203435596)) ;
#91247=CARTESIAN_POINT('Origin',(43.4,252.1,19.3213203435596)) ;
#91248=CARTESIAN_POINT('',(43.3,251.,19.3213203435596)) ;
#91249=CARTESIAN_POINT('Origin',(34.4,245.2,18.3213203435596)) ;
#91250=CARTESIAN_POINT('',(34.4,245.1,18.1213203435596)) ;
#91251=CARTESIAN_POINT('Origin',(34.4,245.1,18.3213203435596)) ;
#91252=CARTESIAN_POINT('',(34.4,245.2,18.0213203435596)) ;
#91253=CARTESIAN_POINT('Origin',(34.4,245.2,18.1213203435596)) ;
#91254=CARTESIAN_POINT('Origin',(34.4,245.2,18.3213203435596)) ;
#91255=CARTESIAN_POINT('Origin',(34.4,250.68933982822,18.7713203435596)) ;
#91256=CARTESIAN_POINT('',(34.4,250.68933982822,18.0213203435596)) ;
#91257=CARTESIAN_POINT('Origin',(34.4,250.68933982822,18.3213203435596)) ;
#91258=CARTESIAN_POINT('Origin',(34.4,250.68933982822,18.7713203435596)) ;
#91259=CARTESIAN_POINT('Origin',(34.4,251.975,18.3213203435596)) ;
#91260=CARTESIAN_POINT('',(34.4,251.975,18.0213203435596)) ;
#91261=CARTESIAN_POINT('Origin',(46.,245.2,18.3213203435596)) ;
#91262=CARTESIAN_POINT('',(46.,245.2,18.0213203435596)) ;
#91263=CARTESIAN_POINT('Origin',(46.,245.2,18.3213203435596)) ;
#91264=CARTESIAN_POINT('',(46.,245.1,18.1213203435596)) ;
#91265=CARTESIAN_POINT('Origin',(46.,245.2,18.1213203435596)) ;
#91266=CARTESIAN_POINT('Origin',(46.,245.1,18.3213203435596)) ;
#91267=CARTESIAN_POINT('Origin',(46.,246.975,18.3213203435596)) ;
#91268=CARTESIAN_POINT('',(45.7,250.68933982822,18.3213203435596)) ;
#91269=CARTESIAN_POINT('',(46.,250.68933982822,18.0213203435596)) ;
#91270=CARTESIAN_POINT('Origin',(46.,250.68933982822,18.3213203435596)) ;
#91271=CARTESIAN_POINT('',(46.,246.975,18.0213203435596)) ;
#91272=CARTESIAN_POINT('',(45.7,246.975,18.3213203435596)) ;
#91273=CARTESIAN_POINT('Origin',(46.,250.68933982822,18.7713203435596)) ;
#91274=CARTESIAN_POINT('',(45.7,251.007537879754,18.4531222920257)) ;
#91275=CARTESIAN_POINT('Origin',(46.,251.007537879754,18.4531222920257)) ;
#91276=CARTESIAN_POINT('Origin',(46.,250.68933982822,18.7713203435596)) ;
#91277=CARTESIAN_POINT('Origin',(45.7,250.68933982822,18.7713203435596)) ;
#91278=CARTESIAN_POINT('Origin',(46.,249.762867965644,17.2084523779156)) ;
#91279=CARTESIAN_POINT('',(45.7,249.762867965644,17.2084523779156)) ;
#91280=CARTESIAN_POINT('Origin',(55.3573593128808,245.1,29.5213203435596)) ;
#91281=CARTESIAN_POINT('',(55.3573593128808,245.1,18.1213203435596)) ;
#91282=CARTESIAN_POINT('',(55.2857703637053,245.1,18.1213203435596)) ;
#91283=CARTESIAN_POINT('',(55.3573593128808,245.1,30.7213203435596)) ;
#91284=CARTESIAN_POINT('',(55.3573593128808,245.1,29.5213203435596)) ;
#91285=CARTESIAN_POINT('',(46.8,245.1,30.7213203435596)) ;
#91286=CARTESIAN_POINT('',(55.3573593128808,245.1,30.7213203435596)) ;
#91287=CARTESIAN_POINT('',(46.8,245.1,20.0213203435596)) ;
#91288=CARTESIAN_POINT('',(46.8,245.1,29.5213203435596)) ;
#91289=CARTESIAN_POINT('',(41.7,245.1,20.0213203435596)) ;
#91290=CARTESIAN_POINT('',(55.3573593128808,245.1,20.0213203435596)) ;
#91291=CARTESIAN_POINT('',(41.7,245.1,24.3713203435596)) ;
#91292=CARTESIAN_POINT('Origin',(55.2857703637053,245.2,18.1213203435596)) ;
#91293=CARTESIAN_POINT('',(55.3573593128808,245.2,18.0213203435596)) ;
#91294=CARTESIAN_POINT('',(55.2857703637053,245.2,18.0213203435596)) ;
#91295=CARTESIAN_POINT('Origin',(55.3573593128808,245.2,18.1213203435596)) ;
#91296=CARTESIAN_POINT('Origin',(55.2141814145299,249.05,18.0213203435596)) ;
#91297=CARTESIAN_POINT('',(57.0469450846408,250.68933982822,18.0213203435596)) ;
#91298=CARTESIAN_POINT('',(52.2356360608974,250.68933982822,18.0213203435596)) ;
#91299=CARTESIAN_POINT('',(57.0171572875254,250.6,18.0213203435596)) ;
#91300=CARTESIAN_POINT('Origin',(57.36141013588,250.588334274672,18.0213203435596)) ;
#91301=CARTESIAN_POINT('',(57.0171572875254,244.208722493294,18.0213203435596)) ;
#91302=CARTESIAN_POINT('',(57.0171572875254,247.8875,18.0213203435596)) ;
#91303=CARTESIAN_POINT('',(56.1573593128807,244.208722493294,18.0213203435596)) ;
#91304=CARTESIAN_POINT('',(64.0732152677426,244.208722493294,18.0213203435596)) ;
#91305=CARTESIAN_POINT('',(56.1573593128807,244.4,18.0213203435596)) ;
#91306=CARTESIAN_POINT('',(56.1573593128808,237.655597577758,18.0213203435596)) ;
#91307=CARTESIAN_POINT('Origin',(55.3573593128808,244.4,18.0213203435596)) ;
#91308=CARTESIAN_POINT('Origin',(52.2356360608974,250.68933982822,18.7713203435596)) ;
#91309=CARTESIAN_POINT('',(57.1201778296089,250.775348215898,18.0261270789701)) ;
#91310=CARTESIAN_POINT('Ctrl Pts',(57.1201105354923,250.775384372087,18.0260789875623)) ;
#91311=CARTESIAN_POINT('Ctrl Pts',(57.1531938341603,250.850775222355,18.0345331819805)) ;
#91312=CARTESIAN_POINT('Ctrl Pts',(57.2453556003495,251.012930443534,18.0800899809205)) ;
#91313=CARTESIAN_POINT('Ctrl Pts',(57.3390787831373,251.150386903953,18.1717072475128)) ;
#91314=CARTESIAN_POINT('Ctrl Pts',(57.3882337581722,251.21966991411,18.2409902576698)) ;
#91315=CARTESIAN_POINT('Ctrl Pts',(57.046945084641,250.68933982822,18.0213203435596)) ;
#91316=CARTESIAN_POINT('Ctrl Pts',(57.0658007810727,250.725754870646,18.0213203435596)) ;
#91317=CARTESIAN_POINT('Ctrl Pts',(57.0917499983331,250.753564280112,18.0236645927849)) ;
#91318=CARTESIAN_POINT('Ctrl Pts',(57.1202270585269,250.775323946388,18.0262024909521)) ;
#91319=CARTESIAN_POINT('Origin',(81.1,238.503733341287,30.6213203435596)) ;
#91320=CARTESIAN_POINT('',(81.1,238.603733341287,30.6213203435596)) ;
#91321=CARTESIAN_POINT('',(81.2,238.503733341287,30.6213203435596)) ;
#91322=CARTESIAN_POINT('Origin',(81.1,238.503733341287,30.6213203435596)) ;
#91323=CARTESIAN_POINT('',(81.1,238.503733341287,30.7213203435596)) ;
#91324=CARTESIAN_POINT('Origin',(81.1,238.503733341287,30.6213203435596)) ;
#91325=CARTESIAN_POINT('Origin',(81.1,238.503733341287,30.6213203435596)) ;
#91326=CARTESIAN_POINT('Origin',(77.925,238.503733341287,30.6213203435596)) ;
#91327=CARTESIAN_POINT('',(80.,238.603733341287,30.6213203435596)) ;
#91328=CARTESIAN_POINT('',(80.1,238.503733341287,30.7213203435596)) ;
#91329=CARTESIAN_POINT('Origin',(80.1,238.503733341287,30.6213203435596)) ;
#91330=CARTESIAN_POINT('',(77.925,238.503733341287,30.7213203435596)) ;
#91331=CARTESIAN_POINT('',(77.925,238.603733341287,30.6213203435596)) ;
#91332=CARTESIAN_POINT('Origin',(74.9999999999998,220.305309236676,30.6213203435596)) ;
#91333=CARTESIAN_POINT('',(72.3072410949819,223.397080489445,30.7213203435596)) ;
#91334=CARTESIAN_POINT('',(72.4472638847366,223.384844644141,30.6213203435596)) ;
#91335=CARTESIAN_POINT('Ctrl Pts',(72.3072410949819,223.397080489445,30.7213203435596)) ;
#91336=CARTESIAN_POINT('Ctrl Pts',(72.3101340243119,223.393675929465,30.7213203435596)) ;
#91337=CARTESIAN_POINT('Ctrl Pts',(72.3132391000724,223.390484046919,30.7210210006498)) ;
#91338=CARTESIAN_POINT('Ctrl Pts',(72.3212552465528,223.38326583681,30.7195830340118)) ;
#91339=CARTESIAN_POINT('Ctrl Pts',(72.3262847482039,223.379552566922,30.7181499124324)) ;
#91340=CARTESIAN_POINT('Ctrl Pts',(72.3418384928136,223.37010049032,30.7123855270563)) ;
#91341=CARTESIAN_POINT('Ctrl Pts',(72.3526461080447,223.366083274383,30.7067053729914)) ;
#91342=CARTESIAN_POINT('Ctrl Pts',(72.3744712399842,223.361576323922,30.6928428900762)) ;
#91343=CARTESIAN_POINT('Ctrl Pts',(72.3854649216459,223.361319212967,30.6845254783462)) ;
#91344=CARTESIAN_POINT('Ctrl Pts',(72.4056828300951,223.363823007051,30.6672585994799)) ;
#91345=CARTESIAN_POINT('Ctrl Pts',(72.4150882865401,223.366503475073,30.6582230647311)) ;
#91346=CARTESIAN_POINT('Ctrl Pts',(72.4320205436683,223.373954425398,30.6402375869053)) ;
#91347=CARTESIAN_POINT('Ctrl Pts',(72.4396999602672,223.378679872843,30.631199149209)) ;
#91348=CARTESIAN_POINT('Ctrl Pts',(72.446817075448,223.384475902764,30.6219068564245)) ;
#91349=CARTESIAN_POINT('Ctrl Pts',(72.4470408822559,223.384659789476,30.6216135992287)) ;
#91350=CARTESIAN_POINT('Ctrl Pts',(72.4472638847366,223.384844644141,30.6213203435596)) ;
#91351=CARTESIAN_POINT('',(75.,224.305309236676,30.6213203435596)) ;
#91352=CARTESIAN_POINT('Origin',(74.9999999999998,220.305309236676,30.6213203435596)) ;
#91353=CARTESIAN_POINT('',(75.,224.405309236676,30.7213203435596)) ;
#91354=CARTESIAN_POINT('Origin',(75.,224.405309236676,30.6213203435596)) ;
#91355=CARTESIAN_POINT('Origin',(74.9999999999998,220.305309236676,30.7213203435596)) ;
#91356=CARTESIAN_POINT('Origin',(77.9249999999999,224.405309236676,30.6213203435596)) ;
#91357=CARTESIAN_POINT('',(79.3510004003203,224.305309236676,30.6213203435596)) ;
#91358=CARTESIAN_POINT('',(79.3510004003203,224.405309236676,30.7213203435596)) ;
#91359=CARTESIAN_POINT('Origin',(79.3510004003203,224.405309236676,30.6213203435596)) ;
#91360=CARTESIAN_POINT('',(77.9249999999999,224.405309236676,30.7213203435596)) ;
#91361=CARTESIAN_POINT('',(77.9249999999999,224.305309236676,30.6213203435596)) ;
#91362=CARTESIAN_POINT('Origin',(79.3510004003203,225.305309236676,30.6213203435596)) ;
#91363=CARTESIAN_POINT('',(80.1316251501201,224.680309236676,30.6213203435596)) ;
#91364=CARTESIAN_POINT('',(80.0535626751402,224.742809236676,30.7213203435596)) ;
#91365=CARTESIAN_POINT('Origin',(80.0535626751402,224.742809236676,30.6213203435596)) ;
#91366=CARTESIAN_POINT('Origin',(79.3510004003203,225.305309236676,30.7213203435596)) ;
#91367=CARTESIAN_POINT('Origin',(79.3510004003203,225.305309236676,30.6213203435596)) ;
#91368=CARTESIAN_POINT('Origin',(80.6000000000002,224.305309236676,30.6213203435596)) ;
#91369=CARTESIAN_POINT('',(80.1757359312881,224.729573305388,30.6213203435596)) ;
#91370=CARTESIAN_POINT('',(80.1050252531694,224.800283983507,30.7213203435596)) ;
#91371=CARTESIAN_POINT('Origin',(80.1050252531694,224.800283983507,30.6213203435596)) ;
#91372=CARTESIAN_POINT('Origin',(80.6000000000002,224.305309236676,30.7213203435596)) ;
#91373=CARTESIAN_POINT('Origin',(80.6000000000002,224.305309236676,30.6213203435596)) ;
#91374=CARTESIAN_POINT('Origin',(80.2950815131274,224.990340243465,30.6213203435596)) ;
#91375=CARTESIAN_POINT('',(81.024264068712,225.578101442812,30.6213203435596)) ;
#91376=CARTESIAN_POINT('',(80.9535533905933,225.648812120931,30.7213203435596)) ;
#91377=CARTESIAN_POINT('Origin',(80.9535533905933,225.648812120931,30.6213203435596)) ;
#91378=CARTESIAN_POINT('',(80.2950815131274,224.990340243465,30.7213203435596)) ;
#91379=CARTESIAN_POINT('',(80.3657921912461,224.919629565346,30.6213203435596)) ;
#91380=CARTESIAN_POINT('Origin',(80.5999999999999,226.002365511524,30.6213203435596)) ;
#91381=CARTESIAN_POINT('',(81.2,226.002365511524,30.6213203435596)) ;
#91382=CARTESIAN_POINT('',(81.1,226.002365511524,30.7213203435596)) ;
#91383=CARTESIAN_POINT('Origin',(81.1,226.002365511524,30.6213203435596)) ;
#91384=CARTESIAN_POINT('Origin',(80.5999999999999,226.002365511524,30.7213203435596)) ;
#91385=CARTESIAN_POINT('Origin',(80.5999999999999,226.002365511524,30.6213203435596)) ;
#91386=CARTESIAN_POINT('Origin',(81.1,233.361105671474,30.6213203435596)) ;
#91387=CARTESIAN_POINT('',(81.1,233.361105671474,30.7213203435596)) ;
#91388=CARTESIAN_POINT('',(81.2,233.361105671474,30.6213203435596)) ;
#91389=CARTESIAN_POINT('Origin',(81.1,238.503733341287,30.1213203435596)) ;
#91390=CARTESIAN_POINT('',(81.2,238.503733341287,29.6213203435596)) ;
#91391=CARTESIAN_POINT('',(81.1,238.603733341287,29.6213203435596)) ;
#91392=CARTESIAN_POINT('Origin',(81.1,238.503733341287,29.6213203435596)) ;
#91393=CARTESIAN_POINT('',(81.1,238.603733341287,30.1213203435596)) ;
#91394=CARTESIAN_POINT('',(81.2,238.503733341287,30.1213203435596)) ;
#91395=CARTESIAN_POINT('Origin',(81.3,238.503733341287,29.6213203435596)) ;
#91396=CARTESIAN_POINT('',(81.3,238.503733341287,29.5213203435596)) ;
#91397=CARTESIAN_POINT('',(81.1267949192431,238.603733341287,29.5213203435596)) ;
#91398=CARTESIAN_POINT('Ctrl Pts',(81.1267949192431,238.603733341287,29.5213203435596)) ;
#91399=CARTESIAN_POINT('Ctrl Pts',(81.1522826614307,238.603733341287,29.5213203435596)) ;
#91400=CARTESIAN_POINT('Ctrl Pts',(81.1815269526849,238.594776141297,29.5213203435596)) ;
#91401=CARTESIAN_POINT('Ctrl Pts',(81.2384776727796,238.564124612906,29.5213203435596)) ;
#91402=CARTESIAN_POINT('Ctrl Pts',(81.2722901777919,238.531443163495,29.5213203435596)) ;
#91403=CARTESIAN_POINT('Ctrl Pts',(81.3,238.503733341287,29.5213203435596)) ;
#91404=CARTESIAN_POINT('Origin',(81.3,238.603733341287,29.6213203435596)) ;
#91405=CARTESIAN_POINT('Origin',(81.3,238.503733341287,29.6213203435596)) ;
#91406=CARTESIAN_POINT('Origin',(75.8499999999999,228.11847800166,30.7213203435596)) ;
#91407=CARTESIAN_POINT('',(80.1,230.5,30.7213203435596)) ;
#91408=CARTESIAN_POINT('',(80.1,229.30923900083,30.7213203435596)) ;
#91409=CARTESIAN_POINT('',(80.2,230.4,30.7213203435596)) ;
#91410=CARTESIAN_POINT('Origin',(80.1,230.4,30.7213203435596)) ;
#91411=CARTESIAN_POINT('',(80.1999999999999,225.6,30.7213203435596)) ;
#91412=CARTESIAN_POINT('',(80.1999999999999,225.6,30.7213203435596)) ;
#91413=CARTESIAN_POINT('',(80.0999999999999,225.5,30.7213203435596)) ;
#91414=CARTESIAN_POINT('Origin',(80.0999999999999,225.6,30.7213203435596)) ;
#91415=CARTESIAN_POINT('',(80.,225.5,30.7213203435596)) ;
#91416=CARTESIAN_POINT('',(76.0414213562372,225.5,30.7213203435596)) ;
#91417=CARTESIAN_POINT('',(80.,224.805309236676,30.7213203435596)) ;
#91418=CARTESIAN_POINT('',(80.,224.305309236676,30.7213203435596)) ;
#91419=CARTESIAN_POINT('',(75.,224.805309236676,30.7213203435596)) ;
#91420=CARTESIAN_POINT('',(80.,224.805309236676,30.7213203435596)) ;
#91421=CARTESIAN_POINT('',(72.4201780792821,223.992383802967,30.7213203435596)) ;
#91422=CARTESIAN_POINT('Origin',(74.9999999999998,220.305309236676,30.7213203435596)) ;
#91423=CARTESIAN_POINT('',(72.2848151277479,223.47832706609,30.7213203435596)) ;
#91424=CARTESIAN_POINT('Origin',(75.1450953968556,223.000000000001,30.7213203435596)) ;
#91425=CARTESIAN_POINT('Origin',(72.383445481855,223.461833029328,30.7213203435596)) ;
#91426=CARTESIAN_POINT('Origin',(80.1,229.30923900083,30.6213203435596)) ;
#91427=CARTESIAN_POINT('',(80.,230.5,30.6213203435596)) ;
#91428=CARTESIAN_POINT('',(80.,229.30923900083,30.6213203435596)) ;
#91429=CARTESIAN_POINT('Origin',(80.1,230.5,30.6213203435596)) ;
#91430=CARTESIAN_POINT('Origin',(80.,238.603733341287,30.7213203435596)) ;
#91431=CARTESIAN_POINT('',(80.,238.603733341287,29.5213203435596)) ;
#91432=CARTESIAN_POINT('',(67.607090707265,238.603733341287,29.5213203435596)) ;
#91433=CARTESIAN_POINT('',(80.,238.603733341287,30.7213203435596)) ;
#91434=CARTESIAN_POINT('Origin',(82.8283628290597,247.448254073888,30.7213203435596)) ;
#91435=CARTESIAN_POINT('',(82.7745180379261,247.36398819427,29.5213203435596)) ;
#91436=CARTESIAN_POINT('',(82.8283628290597,247.348254073888,29.5213203435596)) ;
#91437=CARTESIAN_POINT('Origin',(82.8283628290597,247.448254073888,29.5213203435596)) ;
#91438=CARTESIAN_POINT('',(82.7745180379261,247.36398819427,30.6213203435596)) ;
#91439=CARTESIAN_POINT('',(82.7745180379261,247.36398819427,30.7213203435596)) ;
#91440=CARTESIAN_POINT('',(82.9283628290597,247.448254073888,30.6213203435596)) ;
#91441=CARTESIAN_POINT('Origin',(82.8283628290597,247.448254073888,30.6213203435596)) ;
#91442=CARTESIAN_POINT('',(82.9283628290597,247.448254073888,29.6213203435596)) ;
#91443=CARTESIAN_POINT('',(82.9283628290597,247.448254073888,30.7213203435596)) ;
#91444=CARTESIAN_POINT('Origin',(82.8283628290597,247.448254073888,29.6213203435596)) ;
#91445=CARTESIAN_POINT('Ctrl Pts',(82.9283628290597,247.448254073888,30.6213203435596)) ;
#91446=CARTESIAN_POINT('Ctrl Pts',(82.9283628290597,247.448254073888,30.6340619475287)) ;
#91447=CARTESIAN_POINT('Ctrl Pts',(82.9341320322739,247.440923371758,30.6638411974399)) ;
#91448=CARTESIAN_POINT('Ctrl Pts',(82.9684492173715,247.395367745016,30.7096337860914)) ;
#91449=CARTESIAN_POINT('Ctrl Pts',(83.0061199473635,247.33660142623,30.7213203435596)) ;
#91450=CARTESIAN_POINT('Ctrl Pts',(83.0283628290597,247.297155956632,30.7213203435596)) ;
#91451=CARTESIAN_POINT('Ctrl Pts',(82.9283628290597,247.427878926694,30.6213203435596)) ;
#91452=CARTESIAN_POINT('Ctrl Pts',(82.9283628290597,247.427878926694,30.632388067116)) ;
#91453=CARTESIAN_POINT('Ctrl Pts',(82.9325259207497,247.421320764645,30.658190436137)) ;
#91454=CARTESIAN_POINT('Ctrl Pts',(82.9597089455937,247.379792518138,30.7026967149053)) ;
#91455=CARTESIAN_POINT('Ctrl Pts',(82.9956823265646,247.323984315082,30.7191008858943)) ;
#91456=CARTESIAN_POINT('Ctrl Pts',(83.0184376715155,247.285962574613,30.7213203435596)) ;
#91457=CARTESIAN_POINT('Ctrl Pts',(82.917054183129,247.392349854163,30.6213203435596)) ;
#91458=CARTESIAN_POINT('Ctrl Pts',(82.917054183129,247.392349854163,30.6309476358367)) ;
#91459=CARTESIAN_POINT('Ctrl Pts',(82.9193460938706,247.387147989111,30.6532689555926)) ;
#91460=CARTESIAN_POINT('Ctrl Pts',(82.9395093507166,247.352576015412,30.6992100994537)) ;
#91461=CARTESIAN_POINT('Ctrl Pts',(82.9760987671946,247.301944703507,30.7224004125047)) ;
#91462=CARTESIAN_POINT('Ctrl Pts',(83.0010881693302,247.266396174287,30.7273204280171)) ;
#91463=CARTESIAN_POINT('Ctrl Pts',(82.8741969828184,247.353879677779,30.6213203435596)) ;
#91464=CARTESIAN_POINT('Ctrl Pts',(82.8741969828184,247.353879677779,30.6332771649992)) ;
#91465=CARTESIAN_POINT('Ctrl Pts',(82.8770528905548,247.349680555954,30.6610000049115)) ;
#91466=CARTESIAN_POINT('Ctrl Pts',(82.9023865039853,247.320424668727,30.7178542537679)) ;
#91467=CARTESIAN_POINT('Ctrl Pts',(82.9478254184405,247.274206387667,30.7458171439626)) ;
#91468=CARTESIAN_POINT('Ctrl Pts',(82.9784944719197,247.240915481893,30.7514576611934)) ;
#91469=CARTESIAN_POINT('Ctrl Pts',(82.8219342251982,247.343491305129,30.6213203435596)) ;
#91470=CARTESIAN_POINT('Ctrl Pts',(82.8219342251982,247.343491305129,30.6390908352506)) ;
#91471=CARTESIAN_POINT('Ctrl Pts',(82.8281131661804,247.338693418412,30.6804793222557)) ;
#91472=CARTESIAN_POINT('Ctrl Pts',(82.8704286563925,247.306698271771,30.7533053642045)) ;
#91473=CARTESIAN_POINT('Ctrl Pts',(82.9283403572097,247.2592292449,30.7803880252827)) ;
#91474=CARTESIAN_POINT('Ctrl Pts',(82.9649558842051,247.225646950021,30.7839087790904)) ;
#91475=CARTESIAN_POINT('Ctrl Pts',(82.7873950106811,247.355759977683,30.6213203435596)) ;
#91476=CARTESIAN_POINT('Ctrl Pts',(82.7873950106811,247.355759977683,30.6445020491678)) ;
#91477=CARTESIAN_POINT('Ctrl Pts',(82.7968362794067,247.349589080481,30.6986342225162)) ;
#91478=CARTESIAN_POINT('Ctrl Pts',(82.8547312920342,247.310456538834,30.784599297317)) ;
#91479=CARTESIAN_POINT('Ctrl Pts',(82.9217111420117,247.258080750493,30.8090524868466)) ;
#91480=CARTESIAN_POINT('Ctrl Pts',(82.9620180379262,247.222333709343,30.8101003697968)) ;
#91481=CARTESIAN_POINT('Ctrl Pts',(82.7745180379261,247.36398819427,30.6213203435596)) ;
#91482=CARTESIAN_POINT('Ctrl Pts',(82.7745180379261,247.36398819427,30.6468035514977)) ;
#91483=CARTESIAN_POINT('Ctrl Pts',(82.7853352939526,247.357115661024,30.7063620513201)) ;
#91484=CARTESIAN_POINT('Ctrl Pts',(82.8496800160108,247.314407260952,30.7979472286232)) ;
#91485=CARTESIAN_POINT('Ctrl Pts',(82.9203126347458,247.259313837091,30.8213203435596)) ;
#91486=CARTESIAN_POINT('Ctrl Pts',(82.9620180379262,247.222333709343,30.8213203435596)) ;
#91487=CARTESIAN_POINT('',(82.7995688863616,247.347612311413,30.7213203451448)) ;
#91488=CARTESIAN_POINT('',(83.0283628290571,247.297155956642,30.7213203435596)) ;
#91489=CARTESIAN_POINT('Ctrl Pts',(82.7995655199487,247.347607264512,30.7213203435596)) ;
#91490=CARTESIAN_POINT('Ctrl Pts',(82.8184849722079,247.334987503492,30.7213203435596)) ;
#91491=CARTESIAN_POINT('Ctrl Pts',(82.8384029440696,247.32796189855,30.7213203435596)) ;
#91492=CARTESIAN_POINT('Ctrl Pts',(82.86726782439,247.319640667715,30.7213203435596)) ;
#91493=CARTESIAN_POINT('Ctrl Pts',(82.8841494442442,247.316356042277,30.7213203435596)) ;
#91494=CARTESIAN_POINT('Ctrl Pts',(82.9198493149481,247.310901562837,30.7213203435596)) ;
#91495=CARTESIAN_POINT('Ctrl Pts',(82.9383255275291,247.308684133357,30.7213203435596)) ;
#91496=CARTESIAN_POINT('Ctrl Pts',(82.9901924598214,247.302694056846,30.7213203435596)) ;
#91497=CARTESIAN_POINT('Ctrl Pts',(83.0091658974097,247.300554835715,30.7213203435596)) ;
#91498=CARTESIAN_POINT('Ctrl Pts',(83.0278683017175,247.297244157736,30.7213203435596)) ;
#91499=CARTESIAN_POINT('Ctrl Pts',(83.0281155851111,247.297200164889,30.7213203435596)) ;
#91500=CARTESIAN_POINT('Ctrl Pts',(83.0283628290554,247.297155956633,30.7213203435596)) ;
#91501=CARTESIAN_POINT('Ctrl Pts',(83.0283628290597,247.297155956632,30.7213203435596)) ;
#91502=CARTESIAN_POINT('Ctrl Pts',(83.0061199473635,247.33660142623,30.7213203435596)) ;
#91503=CARTESIAN_POINT('Ctrl Pts',(82.9684492173715,247.395367745016,30.7096337860914)) ;
#91504=CARTESIAN_POINT('Ctrl Pts',(82.9341320322739,247.440923371758,30.6638411974399)) ;
#91505=CARTESIAN_POINT('Ctrl Pts',(82.9283628290597,247.448254073888,30.6340619475287)) ;
#91506=CARTESIAN_POINT('Ctrl Pts',(82.9283628290597,247.448254073888,30.6213203435596)) ;
#91507=CARTESIAN_POINT('Ctrl Pts',(82.7745180379261,247.36398819427,30.6213203435596)) ;
#91508=CARTESIAN_POINT('Ctrl Pts',(82.7745180379261,247.36398819427,30.6468035514977)) ;
#91509=CARTESIAN_POINT('Ctrl Pts',(82.7809835635818,247.359880448284,30.6824019516531)) ;
#91510=CARTESIAN_POINT('Ctrl Pts',(82.7950782219932,247.350599112262,30.7130824661876)) ;
#91511=CARTESIAN_POINT('Ctrl Pts',(82.799565516924,247.34760726653,30.7213203483033)) ;
#91512=CARTESIAN_POINT('Origin',(81.9668461709225,246.100000000001,30.7213203435596)) ;
#91513=CARTESIAN_POINT('',(81.9668461709226,247.600000000001,29.5213203435596)) ;
#91514=CARTESIAN_POINT('Origin',(81.9668461709225,246.100000000001,29.5213203435596)) ;
#91515=CARTESIAN_POINT('',(81.9668461709226,247.600000000001,30.7213203435596)) ;
#91516=CARTESIAN_POINT('',(81.9668461709226,247.600000000001,30.7213203435596)) ;
#91517=CARTESIAN_POINT('Origin',(81.9668461709225,246.100000000001,30.7213203435596)) ;
#91518=CARTESIAN_POINT('Origin',(81.3,239.660172336152,29.6213203435596)) ;
#91519=CARTESIAN_POINT('',(81.2,238.239818409494,29.6213203435596)) ;
#91520=CARTESIAN_POINT('',(81.2,239.660172336152,29.6213203435596)) ;
#91521=CARTESIAN_POINT('',(81.3,238.239818409494,29.5213203435596)) ;
#91522=CARTESIAN_POINT('Origin',(81.3,238.239818409494,29.6213203435596)) ;
#91523=CARTESIAN_POINT('',(81.3,239.660172336152,29.5213203435596)) ;
#91524=CARTESIAN_POINT('Ctrl Pts',(81.3,238.239818409494,29.5213203435596)) ;
#91525=CARTESIAN_POINT('Ctrl Pts',(81.2480070174032,238.055306843022,29.5213203435596)) ;
#91526=CARTESIAN_POINT('Ctrl Pts',(81.2000505692918,237.833945077818,29.4688545911561)) ;
#91527=CARTESIAN_POINT('Ctrl Pts',(81.2000038038563,237.610204859837,29.4219256048081)) ;
#91528=CARTESIAN_POINT('Ctrl Pts',(81.2,237.608784212583,29.4216218542709)) ;
#91529=CARTESIAN_POINT('Ctrl Pts',(81.2,237.60736287746,29.4213203435596)) ;
#91530=CARTESIAN_POINT('Ctrl Pts',(81.2700800699658,238.239818409494,29.5213203435596)) ;
#91531=CARTESIAN_POINT('Ctrl Pts',(81.2280389979125,238.055423609356,29.5373521064363)) ;
#91532=CARTESIAN_POINT('Ctrl Pts',(81.2001824531038,237.828764886114,29.4782935568788)) ;
#91533=CARTESIAN_POINT('Ctrl Pts',(81.2000016826941,237.610154623831,29.4220391644932)) ;
#91534=CARTESIAN_POINT('Ctrl Pts',(81.2,237.608757139533,29.4216792848826)) ;
#91535=CARTESIAN_POINT('Ctrl Pts',(81.2,237.60736287746,29.4213203435596)) ;
#91536=CARTESIAN_POINT('Ctrl Pts',(81.2183034919586,238.239818409494,29.5464528346232)) ;
#91537=CARTESIAN_POINT('Ctrl Pts',(81.2056400608213,238.046097430234,29.5711733353535)) ;
#91538=CARTESIAN_POINT('Ctrl Pts',(81.2001038970389,237.820640503915,29.494000356449)) ;
#91539=CARTESIAN_POINT('Ctrl Pts',(81.2000001080443,237.610062474299,29.4222415191829)) ;
#91540=CARTESIAN_POINT('Ctrl Pts',(81.2,237.608709761695,29.4217797884529)) ;
#91541=CARTESIAN_POINT('Ctrl Pts',(81.2,237.60736287746,29.4213203435596)) ;
#91542=CARTESIAN_POINT('Ctrl Pts',(81.2,238.239818409494,29.598880396034)) ;
#91543=CARTESIAN_POINT('Ctrl Pts',(81.2001340670536,238.026951998836,29.606243609608)) ;
#91544=CARTESIAN_POINT('Ctrl Pts',(81.2000050990089,237.81354631324,29.5096696755031)) ;
#91545=CARTESIAN_POINT('Ctrl Pts',(81.1999999804742,237.60996567801,29.4224440728427)) ;
#91546=CARTESIAN_POINT('Ctrl Pts',(81.2,237.608662383858,29.4218802920233)) ;
#91547=CARTESIAN_POINT('Ctrl Pts',(81.2,237.60736287746,29.4213203435596)) ;
#91548=CARTESIAN_POINT('Ctrl Pts',(81.2,238.239818409494,29.6213203435596)) ;
#91549=CARTESIAN_POINT('Ctrl Pts',(81.2,238.018769899166,29.6213203435596)) ;
#91550=CARTESIAN_POINT('Ctrl Pts',(81.2000000000001,237.810503044327,29.5163888387536)) ;
#91551=CARTESIAN_POINT('Ctrl Pts',(81.2,237.609924206993,29.4225308660566)) ;
#91552=CARTESIAN_POINT('Ctrl Pts',(81.2,237.60864207907,29.4219233649821)) ;
#91553=CARTESIAN_POINT('Ctrl Pts',(81.2,237.60736287746,29.4213203435596)) ;
#91554=CARTESIAN_POINT('',(81.2,237.60736287746,29.4213203435596)) ;
#91555=CARTESIAN_POINT('Ctrl Pts',(81.2,238.239818409494,29.6213203435596)) ;
#91556=CARTESIAN_POINT('Ctrl Pts',(81.2,238.018769899166,29.6213203435596)) ;
#91557=CARTESIAN_POINT('Ctrl Pts',(81.2000000000001,237.810503044327,29.5163888387536)) ;
#91558=CARTESIAN_POINT('Ctrl Pts',(81.2,237.609924206993,29.4225308660566)) ;
#91559=CARTESIAN_POINT('Ctrl Pts',(81.2,237.60864207907,29.4219233649821)) ;
#91560=CARTESIAN_POINT('Ctrl Pts',(81.2,237.60736287746,29.4213203435596)) ;
#91561=CARTESIAN_POINT('',(81.2011028227143,237.670362548256,29.4346494309995)) ;
#91562=CARTESIAN_POINT('Ctrl Pts',(81.2,237.60736287746,29.4213203435596)) ;
#91563=CARTESIAN_POINT('Ctrl Pts',(81.2,237.608784212583,29.4216218542709)) ;
#91564=CARTESIAN_POINT('Ctrl Pts',(81.2000038038563,237.610204859837,29.4219256048081)) ;
#91565=CARTESIAN_POINT('Ctrl Pts',(81.2000081966347,237.631221262085,29.426333745924)) ;
#91566=CARTESIAN_POINT('Ctrl Pts',(81.2003844493976,237.650807905606,29.4304888824184)) ;
#91567=CARTESIAN_POINT('Ctrl Pts',(81.2011028227143,237.670362548256,29.4346494309995)) ;
#91568=CARTESIAN_POINT('Ctrl Pts',(81.2011028227143,237.670362548256,29.4346494309995)) ;
#91569=CARTESIAN_POINT('Ctrl Pts',(81.2085352436464,237.872678436069,29.4776952229906)) ;
#91570=CARTESIAN_POINT('Ctrl Pts',(81.2525894384794,238.07156883933,29.5213203435596)) ;
#91571=CARTESIAN_POINT('Ctrl Pts',(81.3,238.239818409494,29.5213203435596)) ;
#91572=CARTESIAN_POINT('Origin',(81.2,238.603733341287,29.5213203435596)) ;
#91573=CARTESIAN_POINT('',(81.2,226.002365511524,16.1213203435596)) ;
#91574=CARTESIAN_POINT('',(81.2,226.002365511524,29.5213203435596)) ;
#91575=CARTESIAN_POINT('',(81.2,237.60736287746,16.1213203435596)) ;
#91576=CARTESIAN_POINT('',(81.2,234.318247777236,16.1213203435596)) ;
#91577=CARTESIAN_POINT('',(81.2,237.60736287746,29.5213203435596)) ;
#91578=CARTESIAN_POINT('Origin',(56.1573593128808,244.208722493294,17.9213203435596)) ;
#91579=CARTESIAN_POINT('',(56.0573593128807,244.077258377225,18.0720425588636)) ;
#91580=CARTESIAN_POINT('',(56.0573593128807,244.208722493294,18.1213203435596)) ;
#91581=CARTESIAN_POINT('Origin',(56.0573593128807,244.208722493294,17.9213203435596)) ;
#91582=CARTESIAN_POINT('Origin',(56.1573593128807,244.208722493294,18.1213203435596)) ;
#91583=CARTESIAN_POINT('',(56.1573593128808,244.142990435259,17.9966814512116)) ;
#91584=CARTESIAN_POINT('Origin',(56.1573593128808,244.208722493294,17.9213203435596)) ;
#91585=CARTESIAN_POINT('Origin',(56.1573593128808,244.077258377225,18.0720425588636)) ;
#91586=CARTESIAN_POINT('Origin',(56.1573593128808,237.655597577758,18.1213203435596)) ;
#91587=CARTESIAN_POINT('',(56.0573593128808,244.4,18.1213203435596)) ;
#91588=CARTESIAN_POINT('Origin',(56.1573593128807,244.4,18.1213203435596)) ;
#91589=CARTESIAN_POINT('',(56.0573593128807,237.655597577758,18.1213203435596)) ;
#91590=CARTESIAN_POINT('Origin',(55.3573593128808,244.4,18.1213203435596)) ;
#91591=CARTESIAN_POINT('Origin',(55.3573593128808,244.4,18.1213203435596)) ;
#91592=CARTESIAN_POINT('Origin',(64.0732152677426,244.208722493294,17.9213203435596)) ;
#91593=CARTESIAN_POINT('',(57.0171572875254,244.142990435259,17.9966814512116)) ;
#91594=CARTESIAN_POINT('Origin',(57.0171572875254,244.208722493294,17.9213203435596)) ;
#91595=CARTESIAN_POINT('',(64.0732152677426,244.142990435259,17.9966814512116)) ;
#91596=CARTESIAN_POINT('Ctrl Pts',(57.1585786437627,244.295771714953,18.0798989873223)) ;
#91597=CARTESIAN_POINT('Ctrl Pts',(57.1243722498753,244.251856993134,18.0456925934349)) ;
#91598=CARTESIAN_POINT('Ctrl Pts',(57.073701669366,244.208722493294,18.0213203435596)) ;
#91599=CARTESIAN_POINT('Ctrl Pts',(57.0171572875254,244.208722493294,18.0213203435596)) ;
#91600=CARTESIAN_POINT('Ctrl Pts',(57.1662010408867,244.277959825846,18.0875213844463)) ;
#91601=CARTESIAN_POINT('Ctrl Pts',(57.1322204912758,244.236496138881,18.0497812422628)) ;
#91602=CARTESIAN_POINT('Ctrl Pts',(57.0781267479544,244.195060440298,18.0213203435596)) ;
#91603=CARTESIAN_POINT('Ctrl Pts',(57.0171572875254,244.195060440298,18.0213203435596)) ;
#91604=CARTESIAN_POINT('Ctrl Pts',(57.1878308364965,244.246870893186,18.0924999052801)) ;
#91605=CARTESIAN_POINT('Ctrl Pts',(57.149399367403,244.209591803697,18.0494141685073)) ;
#91606=CARTESIAN_POINT('Ctrl Pts',(57.087283042415,244.171163525055,18.0163461021938)) ;
#91607=CARTESIAN_POINT('Ctrl Pts',(57.0171572875254,244.171163525055,18.0163461021938)) ;
#91608=CARTESIAN_POINT('Ctrl Pts',(57.2168557429681,244.225940828197,18.0813885694826)) ;
#91609=CARTESIAN_POINT('Ctrl Pts',(57.1694028080032,244.188418029924,18.0363775851873)) ;
#91610=CARTESIAN_POINT('Ctrl Pts',(57.0975672104142,244.150712341108,18.0034167126644)) ;
#91611=CARTESIAN_POINT('Ctrl Pts',(57.0171572875254,244.150712341108,18.0034167126644)) ;
#91612=CARTESIAN_POINT('Ctrl Pts',(57.2292893218813,244.219798572017,18.0742120091328)) ;
#91613=CARTESIAN_POINT('Ctrl Pts',(57.1779797310502,244.18105028806,18.0289388407524)) ;
#91614=CARTESIAN_POINT('Ctrl Pts',(57.1019738602863,244.142990435259,17.9966814512116)) ;
#91615=CARTESIAN_POINT('Ctrl Pts',(57.0171572875254,244.142990435259,17.9966814512116)) ;
#91616=CARTESIAN_POINT('',(57.1585786437627,244.295771714953,18.0798989873223)) ;
#91617=CARTESIAN_POINT('Ctrl Pts',(57.0171572875254,244.208722493294,18.0213203435596)) ;
#91618=CARTESIAN_POINT('Ctrl Pts',(57.073701669366,244.208722493294,18.0213203435596)) ;
#91619=CARTESIAN_POINT('Ctrl Pts',(57.1243722498753,244.251856993134,18.0456925934349)) ;
#91620=CARTESIAN_POINT('Ctrl Pts',(57.1585786437627,244.295771714953,18.0798989873223)) ;
#91621=CARTESIAN_POINT('',(57.2292893218813,244.219798572017,18.0742120091328)) ;
#91622=CARTESIAN_POINT('Origin',(57.2292893218813,244.295771714953,18.0091883092036)) ;
#91623=CARTESIAN_POINT('Ctrl Pts',(57.2292893218813,244.219798572017,18.0742120091328)) ;
#91624=CARTESIAN_POINT('Ctrl Pts',(57.1779797310502,244.18105028806,18.0289388407524)) ;
#91625=CARTESIAN_POINT('Ctrl Pts',(57.1019738602863,244.142990435259,17.9966814512116)) ;
#91626=CARTESIAN_POINT('Ctrl Pts',(57.0171572875254,244.142990435259,17.9966814512116)) ;
#91627=CARTESIAN_POINT('Ctrl Pts',(57.2287065774412,244.219244545601,18.0735653510966)) ;
#91628=CARTESIAN_POINT('Ctrl Pts',(57.3814006657422,244.334807512776,18.2082665041401)) ;
#91629=CARTESIAN_POINT('Ctrl Pts',(57.5818168023902,244.400164102786,18.3850706639092)) ;
#91630=CARTESIAN_POINT('Ctrl Pts',(57.7829936944083,244.399999844,18.5625564161474)) ;
#91631=CARTESIAN_POINT('Ctrl Pts',(57.2121022546918,244.227431353028,18.083148048922)) ;
#91632=CARTESIAN_POINT('Ctrl Pts',(57.3638432729406,244.342814703471,18.2222979585249)) ;
#91633=CARTESIAN_POINT('Ctrl Pts',(57.5629211478754,244.405277865753,18.4040655266567)) ;
#91634=CARTESIAN_POINT('Ctrl Pts',(57.7617874567952,244.399924414825,18.5837622386288)) ;
#91635=CARTESIAN_POINT('Ctrl Pts',(57.1831337441925,244.250669122844,18.0921857128824)) ;
#91636=CARTESIAN_POINT('Ctrl Pts',(57.3332794540229,244.370076607913,18.239051143939)) ;
#91637=CARTESIAN_POINT('Ctrl Pts',(57.5299105485602,244.433213916469,18.431067418715)) ;
#91638=CARTESIAN_POINT('Ctrl Pts',(57.7250965298064,244.425041966314,18.6204797878858)) ;
#91639=CARTESIAN_POINT('Ctrl Pts',(57.1636274644359,244.281850951555,18.0849477536176)) ;
#91640=CARTESIAN_POINT('Ctrl Pts',(57.3150551881256,244.409361005203,18.2363879364689)) ;
#91641=CARTESIAN_POINT('Ctrl Pts',(57.5136740096313,244.480134652266,18.4349332023547)) ;
#91642=CARTESIAN_POINT('Ctrl Pts',(57.7121552325777,244.477549127776,18.6334758460784)) ;
#91643=CARTESIAN_POINT('Ctrl Pts',(57.1579051025174,244.295194612823,18.079225446077)) ;
#91644=CARTESIAN_POINT('Ctrl Pts',(57.3105939795694,244.426164890483,18.231914323129)) ;
#91645=CARTESIAN_POINT('Ctrl Pts',(57.5110027976195,244.500217797822,18.4323231411791)) ;
#91646=CARTESIAN_POINT('Ctrl Pts',(57.712167056771,244.499999518812,18.6334874003306)) ;
#91647=CARTESIAN_POINT('',(57.7112800931608,244.5,18.6326004367204)) ;
#91648=CARTESIAN_POINT('',(57.7819907712794,244.4,18.5618897586017)) ;
#91649=CARTESIAN_POINT('Origin',(57.7819907712794,244.5,18.5618897586017)) ;
#91650=CARTESIAN_POINT('Origin',(57.7819907712794,243.65,18.5618897586017)) ;
#91651=CARTESIAN_POINT('Origin',(57.7112800931608,243.65,18.6326004367204)) ;
#91652=CARTESIAN_POINT('Origin',(59.6957106781187,244.5,20.475609665441)) ;
#91653=CARTESIAN_POINT('',(59.4877499598282,244.5,20.4090703033878)) ;
#91654=CARTESIAN_POINT('',(59.5584606379469,244.4,20.3383596252692)) ;
#91655=CARTESIAN_POINT('Origin',(59.5584606379469,244.5,20.3383596252692)) ;
#91656=CARTESIAN_POINT('',(59.6957106781187,244.4,20.475609665441)) ;
#91657=CARTESIAN_POINT('',(59.625,244.5,20.5463203435596)) ;
#91658=CARTESIAN_POINT('Ctrl Pts',(59.5584671942072,244.400000068279,20.338175912058)) ;
#91659=CARTESIAN_POINT('Ctrl Pts',(59.5733152046798,244.399998916975,20.3678850518884)) ;
#91660=CARTESIAN_POINT('Ctrl Pts',(59.6079639373555,244.392166720739,20.4372262890232)) ;
#91661=CARTESIAN_POINT('Ctrl Pts',(59.6346249869036,244.367754219918,20.4905963915537)) ;
#91662=CARTESIAN_POINT('Ctrl Pts',(59.6446565645846,244.350697787771,20.510678433286)) ;
#91663=CARTESIAN_POINT('Ctrl Pts',(59.537282725906,244.399957438475,20.3593605952471)) ;
#91664=CARTESIAN_POINT('Ctrl Pts',(59.5535226580609,244.403204576356,20.3876218149334)) ;
#91665=CARTESIAN_POINT('Ctrl Pts',(59.5939825862619,244.401172393675,20.4544573327192)) ;
#91666=CARTESIAN_POINT('Ctrl Pts',(59.6277898217881,244.376233246362,20.5066189259004)) ;
#91667=CARTESIAN_POINT('Ctrl Pts',(59.6406435698939,244.357497856102,20.5262463389736)) ;
#91668=CARTESIAN_POINT('Ctrl Pts',(59.5006111373498,244.425081428672,20.396017115008)) ;
#91669=CARTESIAN_POINT('Ctrl Pts',(59.5229458164964,244.430091479793,20.4219725732252)) ;
#91670=CARTESIAN_POINT('Ctrl Pts',(59.5781914473742,244.428908376005,20.4846291462517)) ;
#91671=CARTESIAN_POINT('Ctrl Pts',(59.6235364564538,244.397463327035,20.5345903902754)) ;
#91672=CARTESIAN_POINT('Ctrl Pts',(59.6406929112882,244.373534147426,20.5534465526952)) ;
#91673=CARTESIAN_POINT('Ctrl Pts',(59.4876383932168,244.477554105521,20.4089588892195)) ;
#91674=CARTESIAN_POINT('Ctrl Pts',(59.51569834688,244.479058256544,20.4369804578922)) ;
#91675=CARTESIAN_POINT('Ctrl Pts',(59.5819260984814,244.46774807284,20.5031955440028)) ;
#91676=CARTESIAN_POINT('Ctrl Pts',(59.6335489997903,244.424139894224,20.5548732787412)) ;
#91677=CARTESIAN_POINT('Ctrl Pts',(59.6530089235801,244.39307153877,20.5743292554704)) ;
#91678=CARTESIAN_POINT('Ctrl Pts',(59.4876318556191,244.499999964608,20.4089521991787)) ;
#91679=CARTESIAN_POINT('Ctrl Pts',(59.517336511604,244.500017767817,20.4386568551635)) ;
#91680=CARTESIAN_POINT('Ctrl Pts',(59.5866699888097,244.484389267076,20.5079903323693)) ;
#91681=CARTESIAN_POINT('Ctrl Pts',(59.6400363483859,244.435560982935,20.5613566919455)) ;
#91682=CARTESIAN_POINT('Ctrl Pts',(59.6601169821608,244.4014377108,20.5814373257204)) ;
#91683=CARTESIAN_POINT('',(59.5361382460763,244.470551010537,20.453396295288)) ;
#91684=CARTESIAN_POINT('',(59.6446141839292,244.350769740148,20.5106667172338)) ;
#91685=CARTESIAN_POINT('Ctrl Pts',(59.5361418751229,244.470548356227,20.4533975244613)) ;
#91686=CARTESIAN_POINT('Ctrl Pts',(59.5556542115485,244.456276801076,20.4696116159651)) ;
#91687=CARTESIAN_POINT('Ctrl Pts',(59.5754367551715,244.439013252497,20.48414635836)) ;
#91688=CARTESIAN_POINT('Ctrl Pts',(59.6043064288728,244.407760596003,20.500592829049)) ;
#91689=CARTESIAN_POINT('Ctrl Pts',(59.6145514147285,244.395323576303,20.5053596763027)) ;
#91690=CARTESIAN_POINT('Ctrl Pts',(59.6312403814749,244.372254380133,20.5102712030638)) ;
#91691=CARTESIAN_POINT('Ctrl Pts',(59.6380964847321,244.361802761066,20.5112975698589)) ;
#91692=CARTESIAN_POINT('Ctrl Pts',(59.6444658667391,244.351021269097,20.5106817644182)) ;
#91693=CARTESIAN_POINT('Ctrl Pts',(59.6445400561483,244.350895531046,20.5106743560996)) ;
#91694=CARTESIAN_POINT('Ctrl Pts',(59.6446141839293,244.350769740148,20.5106667172364)) ;
#91695=CARTESIAN_POINT('Origin',(59.5584606379469,244.3,20.3383596252692)) ;
#91696=CARTESIAN_POINT('',(59.5008788001387,244.499567297188,20.4221991441223)) ;
#91697=CARTESIAN_POINT('Origin',(59.4877499598282,244.3,20.4090703033878)) ;
#91698=CARTESIAN_POINT('Ctrl Pts',(59.5008803400812,244.499565874957,20.4222006849129)) ;
#91699=CARTESIAN_POINT('Ctrl Pts',(59.506343646892,244.494520221898,20.427660931309)) ;
#91700=CARTESIAN_POINT('Ctrl Pts',(59.5120512929965,244.489533320353,20.4328815347287)) ;
#91701=CARTESIAN_POINT('Ctrl Pts',(59.5238687470823,244.47979868564,20.4431905436275)) ;
#91702=CARTESIAN_POINT('Ctrl Pts',(59.5299380750016,244.47508550957,20.4482422082633)) ;
#91703=CARTESIAN_POINT('Ctrl Pts',(59.5361389131708,244.47055052273,20.4533950632053)) ;
#91704=CARTESIAN_POINT('Origin',(64.4831104165663,219.797752737776,16.1213203435596)) ;
#91705=CARTESIAN_POINT('',(63.3432752896628,216.068037482763,16.1213203435596)) ;
#91706=CARTESIAN_POINT('Origin',(63.3615337515762,216.16706261919,16.1213376927199)) ;
#91707=CARTESIAN_POINT('',(61.2884174438392,217.560804636007,16.1213203435596)) ;
#91708=CARTESIAN_POINT('Origin',(64.4831104165663,219.797752737776,16.1213203435596)) ;
#91709=CARTESIAN_POINT('Origin',(61.3703326482681,217.618162279643,16.1213203435596)) ;
#91710=CARTESIAN_POINT('Origin',(59.3765805603019,220.465535350009,16.1213203435596)) ;
#91711=CARTESIAN_POINT('',(56.7626663401537,224.024247053747,16.1213203435596)) ;
#91712=CARTESIAN_POINT('Origin',(56.8445815445825,224.081604697382,16.1213203435596)) ;
#91713=CARTESIAN_POINT('',(59.294665355873,220.408177706374,16.1213203435596)) ;
#91714=CARTESIAN_POINT('Origin',(59.9573593128806,226.261195155516,16.1213203435596)) ;
#91715=CARTESIAN_POINT('',(56.0573593128808,226.261195155516,16.1213203435596)) ;
#91716=CARTESIAN_POINT('Origin',(56.1573593128808,226.261195155516,16.1213203435596)) ;
#91717=CARTESIAN_POINT('Origin',(59.9573593128806,226.261195155516,16.1213203435596)) ;
#91718=CARTESIAN_POINT('Origin',(56.1573593128808,228.14697868435,16.1213203435596)) ;
#91719=CARTESIAN_POINT('',(56.0573593128807,238.278291754874,16.1213203435596)) ;
#91720=CARTESIAN_POINT('Origin',(56.1573593128808,238.278291754874,16.1213203435596)) ;
#91721=CARTESIAN_POINT('',(56.0573593128808,228.14697868435,16.1213203435596)) ;
#91722=CARTESIAN_POINT('Origin',(56.1573593128808,238.278291754874,16.7713203435596)) ;
#91723=CARTESIAN_POINT('',(56.0573593128807,238.483839802785,16.1546761998268)) ;
#91724=CARTESIAN_POINT('',(56.1573593128808,238.515462579386,16.0598078700217)) ;
#91725=CARTESIAN_POINT('Origin',(56.1573593128808,238.483839802785,16.1546761998268)) ;
#91726=CARTESIAN_POINT('Origin',(56.1573593128808,238.278291754874,16.7713203435596)) ;
#91727=CARTESIAN_POINT('Origin',(56.0573593128807,238.278291754874,16.7713203435596)) ;
#91728=CARTESIAN_POINT('Origin',(56.1573593128808,236.430915043381,15.4703679466921)) ;
#91729=CARTESIAN_POINT('',(56.0573593128807,243.855548047911,17.9452456148689)) ;
#91730=CARTESIAN_POINT('',(56.1573593128807,243.887170824513,17.8503772850638)) ;
#91731=CARTESIAN_POINT('Origin',(56.1573593128807,243.855548047911,17.9452456148689)) ;
#91732=CARTESIAN_POINT('',(56.1573593128808,236.462537819982,15.375499616887)) ;
#91733=CARTESIAN_POINT('',(56.0573593128807,236.430915043381,15.4703679466921)) ;
#91734=CARTESIAN_POINT('Origin',(56.1573593128808,243.65,18.5618897586017)) ;
#91735=CARTESIAN_POINT('Origin',(56.1573593128808,243.65,18.5618897586017)) ;
#91736=CARTESIAN_POINT('Origin',(56.0573593128807,243.65,18.5618897586017)) ;
#91737=CARTESIAN_POINT('Origin',(55.3573593128808,244.4,29.5213203435596)) ;
#91738=CARTESIAN_POINT('',(56.0573593128808,244.4,30.7213203435596)) ;
#91739=CARTESIAN_POINT('',(56.0573593128808,244.4,29.5213203435596)) ;
#91740=CARTESIAN_POINT('Origin',(55.3573593128808,244.4,30.7213203435596)) ;
#91741=CARTESIAN_POINT('Origin',(56.0573593128808,226.261195155516,29.5213203435596)) ;
#91742=CARTESIAN_POINT('',(56.0573593128808,226.261195155516,30.7213203435596)) ;
#91743=CARTESIAN_POINT('',(56.0573593128808,226.261195155516,29.5213203435596)) ;
#91744=CARTESIAN_POINT('',(56.0573593128808,226.261195155516,30.7213203435596)) ;
#91745=CARTESIAN_POINT('Origin',(59.9573593128806,226.261195155516,29.5213203435596)) ;
#91746=CARTESIAN_POINT('',(56.7626663401537,224.024247053747,30.7213203435596)) ;
#91747=CARTESIAN_POINT('',(56.7626663401537,224.024247053747,29.5213203435596)) ;
#91748=CARTESIAN_POINT('Origin',(59.9573593128806,226.261195155516,30.7213203435596)) ;
#91749=CARTESIAN_POINT('Origin',(60.2642432409823,219.023476982374,29.5213203435596)) ;
#91750=CARTESIAN_POINT('',(61.2884174438392,217.560804636007,23.2713203435596)) ;
#91751=CARTESIAN_POINT('',(61.2884174438392,217.560804636007,25.0213203435596)) ;
#91752=CARTESIAN_POINT('',(60.2642432409823,219.023476982374,23.2713203435596)) ;
#91753=CARTESIAN_POINT('',(60.8660775466133,218.163968518398,23.2713203435596)) ;
#91754=CARTESIAN_POINT('',(60.2642432409823,219.023476982374,30.7213203435596)) ;
#91755=CARTESIAN_POINT('',(60.2642432409823,219.023476982374,29.5213203435596)) ;
#91756=CARTESIAN_POINT('',(61.2884174438392,217.560804636007,30.7213203435596)) ;
#91757=CARTESIAN_POINT('Origin',(64.4831104165663,219.797752737776,25.0213203435596)) ;
#91758=CARTESIAN_POINT('',(63.3432752896628,216.068037482763,23.2713203435596)) ;
#91759=CARTESIAN_POINT('',(63.3432752896628,216.068037482763,25.0213203435596)) ;
#91760=CARTESIAN_POINT('Origin',(64.4831104165663,219.797752737776,23.2713203435596)) ;
#91761=CARTESIAN_POINT('Origin',(69.2808968287545,215.776927458569,16.1213203435596)) ;
#91762=CARTESIAN_POINT('',(69.4013544815242,215.668771587158,16.1213203435596)) ;
#91763=CARTESIAN_POINT('Origin',(69.4079308494226,215.768555109772,16.1213203435596)) ;
#91764=CARTESIAN_POINT('',(69.2743204608562,215.677143935955,16.1213203435596)) ;
#91765=CARTESIAN_POINT('Ctrl Pts',(68.4157280311031,244.326083322956,17.9953582499056)) ;
#91766=CARTESIAN_POINT('Ctrl Pts',(68.415503099048,244.326287996807,17.9954135499195)) ;
#91767=CARTESIAN_POINT('Ctrl Pts',(68.4152781349504,244.326493093575,17.9954686676332)) ;
#91768=CARTESIAN_POINT('Ctrl Pts',(68.3480453599995,244.387545954585,18.0121657700759)) ;
#91769=CARTESIAN_POINT('Ctrl Pts',(68.2868811696763,244.449692607864,18.0339989374688)) ;
#91770=CARTESIAN_POINT('Ctrl Pts',(68.2414978867463,244.482287915021,18.0798261741698)) ;
#91771=CARTESIAN_POINT('Ctrl Pts',(68.4157280311031,244.326083322956,17.9953582499056)) ;
#91772=CARTESIAN_POINT('Ctrl Pts',(68.4154763603613,244.326233226319,17.9953987516991)) ;
#91773=CARTESIAN_POINT('Ctrl Pts',(68.4152333288418,244.326412830281,17.9954758377209)) ;
#91774=CARTESIAN_POINT('Ctrl Pts',(68.3408356732327,244.374438578966,18.0076269476457)) ;
#91775=CARTESIAN_POINT('Ctrl Pts',(68.2707325615201,244.423538275651,18.0415477041581)) ;
#91776=CARTESIAN_POINT('Ctrl Pts',(68.2323584534764,244.441748530438,18.089128043464)) ;
#91777=CARTESIAN_POINT('Ctrl Pts',(68.4157280311031,244.326083322956,17.9953582499056)) ;
#91778=CARTESIAN_POINT('Ctrl Pts',(68.4154538754065,244.326202355367,17.9953904107993)) ;
#91779=CARTESIAN_POINT('Ctrl Pts',(68.415184345804,244.326316512137,17.9954511971732)) ;
#91780=CARTESIAN_POINT('Ctrl Pts',(68.3337700599932,244.3621377726,18.004245689451)) ;
#91781=CARTESIAN_POINT('Ctrl Pts',(68.2537549741851,244.397420595634,18.0357515724808)) ;
#91782=CARTESIAN_POINT('Ctrl Pts',(68.2020344914338,244.402854022253,18.0767019419474)) ;
#91783=CARTESIAN_POINT('Ctrl Pts',(68.4157280311031,244.326083322956,17.9953582499056)) ;
#91784=CARTESIAN_POINT('Ctrl Pts',(68.4154317761631,244.326160630694,17.9953791373758)) ;
#91785=CARTESIAN_POINT('Ctrl Pts',(68.4151352241728,244.326238449581,17.9954000300808)) ;
#91786=CARTESIAN_POINT('Ctrl Pts',(68.3266140510332,244.349168426876,18.0017543602468)) ;
#91787=CARTESIAN_POINT('Ctrl Pts',(68.237732147878,244.375710462253,18.0166982540741)) ;
#91788=CARTESIAN_POINT('Ctrl Pts',(68.1704101577868,244.39111820199,18.0506955811225)) ;
#91789=CARTESIAN_POINT('',(68.1715529942029,244.390856053509,18.050121315269)) ;
#91790=CARTESIAN_POINT('',(68.2422637392367,244.481712398084,18.0790566043223)) ;
#91791=CARTESIAN_POINT('Origin',(68.1715529942029,244.481712107019,18.0083459931195)) ;
#91792=CARTESIAN_POINT('',(68.4134930867977,244.32811526913,17.9959101696537)) ;
#91793=CARTESIAN_POINT('Ctrl Pts',(68.2422671027082,244.481712396327,18.0790532408515)) ;
#91794=CARTESIAN_POINT('Ctrl Pts',(68.2493325411649,244.476606556519,18.0719882407775)) ;
#91795=CARTESIAN_POINT('Ctrl Pts',(68.2568413561123,244.470680650291,18.0655175608582)) ;
#91796=CARTESIAN_POINT('Ctrl Pts',(68.2646955001455,244.464145311328,18.0595601342585)) ;
#91797=CARTESIAN_POINT('Ctrl Pts',(68.2727769201473,244.45742085876,18.0534303171481)) ;
#91798=CARTESIAN_POINT('Ctrl Pts',(68.2812243384575,244.450051298074,18.0478431272093)) ;
#91799=CARTESIAN_POINT('Ctrl Pts',(68.2899663542551,244.442222844725,18.0427061835484)) ;
#91800=CARTESIAN_POINT('Ctrl Pts',(68.2991681976564,244.433982616904,18.0372990380773)) ;
#91801=CARTESIAN_POINT('Ctrl Pts',(68.3086969039584,244.425234059554,18.0323900053085)) ;
#91802=CARTESIAN_POINT('Ctrl Pts',(68.3185014235944,244.416145218704,18.0278789496962)) ;
#91803=CARTESIAN_POINT('Ctrl Pts',(68.3285924324566,244.406790800846,18.0232360805041)) ;
#91804=CARTESIAN_POINT('Ctrl Pts',(68.3389763842491,244.397075734544,18.0190142970919)) ;
#91805=CARTESIAN_POINT('Ctrl Pts',(68.3496210593381,244.387133438654,18.0151221223351)) ;
#91806=CARTESIAN_POINT('Ctrl Pts',(68.3608979552043,244.376600638499,18.0109987790617)) ;
#91807=CARTESIAN_POINT('Ctrl Pts',(68.3724684244289,244.365812753876,18.0072451144521)) ;
#91808=CARTESIAN_POINT('Ctrl Pts',(68.3843064678103,244.354874916172,18.0037781849552)) ;
#91809=CARTESIAN_POINT('Ctrl Pts',(68.3938654112985,244.346042867739,18.0009787203757)) ;
#91810=CARTESIAN_POINT('Ctrl Pts',(68.403599256299,244.337111839492,17.9983668597683)) ;
#91811=CARTESIAN_POINT('Ctrl Pts',(68.4134930867977,244.32811526913,17.9959101696537)) ;
#91812=CARTESIAN_POINT('',(68.4157280311053,244.326083322956,17.9953582499056)) ;
#91813=CARTESIAN_POINT('Ctrl Pts',(68.4134930867977,244.32811526913,17.9959101696537)) ;
#91814=CARTESIAN_POINT('Ctrl Pts',(68.4140127841,244.32764270258,17.995781126082)) ;
#91815=CARTESIAN_POINT('Ctrl Pts',(68.414532921807,244.327169951285,17.995652512562)) ;
#91816=CARTESIAN_POINT('Ctrl Pts',(68.4150534973794,244.326697018831,17.9955243250024)) ;
#91817=CARTESIAN_POINT('Ctrl Pts',(68.4152781128779,244.326492960161,17.9954690152373)) ;
#91818=CARTESIAN_POINT('Ctrl Pts',(68.4155030853425,244.326287968735,17.9954135423348)) ;
#91819=CARTESIAN_POINT('Ctrl Pts',(68.415728031103,244.326083322956,17.9953582499058)) ;
#91820=CARTESIAN_POINT('',(68.4126406994004,244.326885339084,17.9955808747352)) ;
#91821=CARTESIAN_POINT('Ctrl Pts',(68.4157280311031,244.326083322956,17.9953582499056)) ;
#91822=CARTESIAN_POINT('Ctrl Pts',(68.4154317761631,244.326160630694,17.9953791373758)) ;
#91823=CARTESIAN_POINT('Ctrl Pts',(68.4151352241728,244.326238449581,17.9954000300808)) ;
#91824=CARTESIAN_POINT('Ctrl Pts',(68.4141066106842,244.326504895258,17.9954738672148)) ;
#91825=CARTESIAN_POINT('Ctrl Pts',(68.4133736713245,244.326694994148,17.9955270708784)) ;
#91826=CARTESIAN_POINT('Ctrl Pts',(68.4126406994004,244.326885339084,17.9955808747352)) ;
#91827=CARTESIAN_POINT('Ctrl Pts',(68.4126406994004,244.326885339084,17.9955808747352)) ;
#91828=CARTESIAN_POINT('Ctrl Pts',(68.3256372266032,244.349479206531,18.0019673709072)) ;
#91829=CARTESIAN_POINT('Ctrl Pts',(68.2381749361321,244.375539775844,18.0168103443043)) ;
#91830=CARTESIAN_POINT('Ctrl Pts',(68.1715529942029,244.390856053509,18.050121315269)) ;
#91831=CARTESIAN_POINT('Ctrl Pts',(68.2422636723215,244.481712107019,18.0790566712382)) ;
#91832=CARTESIAN_POINT('Ctrl Pts',(68.216159455498,244.493714742233,18.1051608880617)) ;
#91833=CARTESIAN_POINT('Ctrl Pts',(68.1874444287551,244.5,18.1338759148046)) ;
#91834=CARTESIAN_POINT('Ctrl Pts',(68.1587130280226,244.5,18.1626073155371)) ;
#91835=CARTESIAN_POINT('Ctrl Pts',(68.2369709753343,244.458690211032,18.0843493682253)) ;
#91836=CARTESIAN_POINT('Ctrl Pts',(68.2123052970946,244.468092133554,18.1090740358395)) ;
#91837=CARTESIAN_POINT('Ctrl Pts',(68.1852296346586,244.472056879549,18.1359779514075)) ;
#91838=CARTESIAN_POINT('Ctrl Pts',(68.1587130280226,244.470080069966,18.1626073155371)) ;
#91839=CARTESIAN_POINT('Ctrl Pts',(68.2163693612034,244.418594990287,18.0821834080608)) ;
#91840=CARTESIAN_POINT('Ctrl Pts',(68.1923316647305,244.423578999196,18.1025989413263)) ;
#91841=CARTESIAN_POINT('Ctrl Pts',(68.1662580373605,244.423426860681,18.1244213984655)) ;
#91842=CARTESIAN_POINT('Ctrl Pts',(68.1409417831407,244.418303305343,18.1448360706551)) ;
#91843=CARTESIAN_POINT('Ctrl Pts',(68.1849909585482,244.395956487844,18.0612141162575)) ;
#91844=CARTESIAN_POINT('Ctrl Pts',(68.1595025691414,244.400924816049,18.0762392209731)) ;
#91845=CARTESIAN_POINT('Ctrl Pts',(68.131583958965,244.402300999176,18.0923928210252)) ;
#91846=CARTESIAN_POINT('Ctrl Pts',(68.1038697889688,244.4,18.1077640764833)) ;
#91847=CARTESIAN_POINT('Ctrl Pts',(68.1715529942029,244.390856053509,18.050121315269)) ;
#91848=CARTESIAN_POINT('Ctrl Pts',(68.1454487773793,244.396857371116,18.0631734236807)) ;
#91849=CARTESIAN_POINT('Ctrl Pts',(68.1167337506364,244.4,18.0775309370522)) ;
#91850=CARTESIAN_POINT('Ctrl Pts',(68.088002349904,244.4,18.0918966374184)) ;
#91851=CARTESIAN_POINT('',(68.088002349904,244.4,18.0918966374184)) ;
#91852=CARTESIAN_POINT('',(68.1587130280226,244.5,18.1626073155371)) ;
#91853=CARTESIAN_POINT('Origin',(68.088002349904,244.5,18.0918966374184)) ;
#91854=CARTESIAN_POINT('Origin',(68.1587130280226,244.3,18.1626073155371)) ;
#91855=CARTESIAN_POINT('Origin',(68.088002349904,244.3,18.0918966374184)) ;
#91856=CARTESIAN_POINT('Origin',(65.9792893218814,244.5,20.200609665441)) ;
#91857=CARTESIAN_POINT('',(66.1,244.4,20.0798989873224)) ;
#91858=CARTESIAN_POINT('',(66.1707106781187,244.5,20.150609665441)) ;
#91859=CARTESIAN_POINT('Origin',(66.1,244.5,20.0798989873224)) ;
#91860=CARTESIAN_POINT('',(66.05,244.5,20.2713203435597)) ;
#91861=CARTESIAN_POINT('',(65.9792893218814,244.4,20.200609665441)) ;
#91862=CARTESIAN_POINT('Ctrl Pts',(66.1708868324018,244.499999967942,20.1504335111579)) ;
#91863=CARTESIAN_POINT('Ctrl Pts',(66.0635188884297,244.500039048421,20.25780145513)) ;
#91864=CARTESIAN_POINT('Ctrl Pts',(65.9564406808178,244.46434631255,20.3648796627419)) ;
#91865=CARTESIAN_POINT('Ctrl Pts',(65.8705697739276,244.399894281784,20.4507505696321)) ;
#91866=CARTESIAN_POINT('Ctrl Pts',(66.170881676644,244.470075190665,20.1504389438007)) ;
#91867=CARTESIAN_POINT('Ctrl Pts',(66.0666566269504,244.473068265832,20.2544950124528)) ;
#91868=CARTESIAN_POINT('Ctrl Pts',(65.9619739267268,244.441148453657,20.3594054251304)) ;
#91869=CARTESIAN_POINT('Ctrl Pts',(65.8777198541297,244.380841276891,20.4436003927159)) ;
#91870=CARTESIAN_POINT('Ctrl Pts',(66.1530889222118,244.418272466591,20.1326643833074)) ;
#91871=CARTESIAN_POINT('Ctrl Pts',(66.0581593621532,244.42596869334,20.2349249147586)) ;
#91872=CARTESIAN_POINT('Ctrl Pts',(65.9603621384066,244.400754686742,20.3386298810903)) ;
#91873=CARTESIAN_POINT('Ctrl Pts',(65.8812382246392,244.347587615883,20.4221602225383)) ;
#91874=CARTESIAN_POINT('Ctrl Pts',(66.1159846943527,244.399981442444,20.0955666391745)) ;
#91875=CARTESIAN_POINT('Ctrl Pts',(66.0285944646232,244.403450570881,20.2014160256478)) ;
#91876=CARTESIAN_POINT('Ctrl Pts',(65.9397032095956,244.377094235374,20.3074787984105)) ;
#91877=CARTESIAN_POINT('Ctrl Pts',(65.8679593077692,244.325965696746,20.3926529481467)) ;
#91878=CARTESIAN_POINT('Ctrl Pts',(66.1001017858144,244.400000004182,20.0796836953459)) ;
#91879=CARTESIAN_POINT('Ctrl Pts',(66.0142111292878,244.400022779608,20.1870553905182)) ;
#91880=CARTESIAN_POINT('Ctrl Pts',(65.9285565399426,244.371463165213,20.2941361064605)) ;
#91881=CARTESIAN_POINT('Ctrl Pts',(65.8598673418409,244.319900473437,20.3800087345052)) ;
#91882=CARTESIAN_POINT('',(65.8600000000003,244.32,20.3798989873221)) ;
#91883=CARTESIAN_POINT('',(65.870710678119,244.4,20.4506096654407)) ;
#91884=CARTESIAN_POINT('Origin',(65.8000000000003,244.4,20.3798989873221)) ;
#91885=CARTESIAN_POINT('Origin',(66.1707106781187,244.,20.150609665441)) ;
#91886=CARTESIAN_POINT('Origin',(66.1,244.,20.0798989873224)) ;
#91887=CARTESIAN_POINT('Ctrl Pts',(65.870710678119,244.4,20.4506096654407)) ;
#91888=CARTESIAN_POINT('Ctrl Pts',(65.8360427798554,244.36985400151,20.4852775637043)) ;
#91889=CARTESIAN_POINT('Ctrl Pts',(65.8021595990186,244.336414539989,20.5191607445411)) ;
#91890=CARTESIAN_POINT('Ctrl Pts',(65.7707106781184,244.3,20.5506096654413)) ;
#91891=CARTESIAN_POINT('Ctrl Pts',(65.8778581049433,244.380940195135,20.4434622386164)) ;
#91892=CARTESIAN_POINT('Ctrl Pts',(65.8430433343115,244.353134492895,20.4771176025337)) ;
#91893=CARTESIAN_POINT('Ctrl Pts',(65.8097520166116,244.321564032013,20.5105222764137)) ;
#91894=CARTESIAN_POINT('Ctrl Pts',(65.779668623883,244.286563081353,20.5416517196767)) ;
#91895=CARTESIAN_POINT('Ctrl Pts',(65.8813668211755,244.347686535338,20.4220307100008)) ;
#91896=CARTESIAN_POINT('Ctrl Pts',(65.8477072298486,244.32429083244,20.4556827577087)) ;
#91897=CARTESIAN_POINT('Ctrl Pts',(65.8162031922682,244.295932764198,20.4889255959091)) ;
#91898=CARTESIAN_POINT('Ctrl Pts',(65.7888149094442,244.263086758199,20.5194962410323)) ;
#91899=CARTESIAN_POINT('Ctrl Pts',(65.868086390361,244.326064792771,20.3925339722608)) ;
#91900=CARTESIAN_POINT('Ctrl Pts',(65.83765096067,244.304388217631,20.427955315655)) ;
#91901=CARTESIAN_POINT('Ctrl Pts',(65.8090916912018,244.277609164501,20.461748760347)) ;
#91902=CARTESIAN_POINT('Ctrl Pts',(65.7842756013319,244.245700801776,20.4917756576894)) ;
#91903=CARTESIAN_POINT('Ctrl Pts',(65.8600000000003,244.32,20.3798989873221)) ;
#91904=CARTESIAN_POINT('Ctrl Pts',(65.8310598414498,244.298294881087,20.4160741855102)) ;
#91905=CARTESIAN_POINT('Ctrl Pts',(65.8038349716294,244.271779962173,20.4501052727856)) ;
#91906=CARTESIAN_POINT('Ctrl Pts',(65.7799999999998,244.24,20.4798989873226)) ;
#91907=CARTESIAN_POINT('',(65.7799999999998,244.24,20.4798989873226)) ;
#91908=CARTESIAN_POINT('',(65.7707106781184,244.3,20.5506096654413)) ;
#91909=CARTESIAN_POINT('Origin',(65.6999999999998,244.3,20.4798989873226)) ;
#91910=CARTESIAN_POINT('Origin',(66.1832249621182,244.169671602392,20.1380953814425)) ;
#91911=CARTESIAN_POINT('Origin',(66.2266636446466,243.872582870471,19.9189605675217)) ;
#91912=CARTESIAN_POINT('Ctrl Pts',(65.7714515421241,244.300985201758,20.5498688014357)) ;
#91913=CARTESIAN_POINT('Ctrl Pts',(65.7063868734546,244.214691234227,20.6149334701051)) ;
#91914=CARTESIAN_POINT('Ctrl Pts',(65.6704368938516,244.106841295417,20.6508834497081)) ;
#91915=CARTESIAN_POINT('Ctrl Pts',(65.6707122482682,243.99876732019,20.6506080952915)) ;
#91916=CARTESIAN_POINT('Ctrl Pts',(65.7871454118088,244.27732415233,20.534176623468)) ;
#91917=CARTESIAN_POINT('Ctrl Pts',(65.7239411552949,244.198785882952,20.5972314295624)) ;
#91918=CARTESIAN_POINT('Ctrl Pts',(65.6890022448555,244.098898958229,20.6323192265238)) ;
#91919=CARTESIAN_POINT('Ctrl Pts',(65.6892698546687,243.998858952482,20.6320504824346)) ;
#91920=CARTESIAN_POINT('Ctrl Pts',(65.7906574856275,244.253999224632,20.5067481801081)) ;
#91921=CARTESIAN_POINT('Ctrl Pts',(65.7323922982686,244.182917249722,20.5707044860515)) ;
#91922=CARTESIAN_POINT('Ctrl Pts',(65.6998049270229,244.091013326971,20.6062210696643)) ;
#91923=CARTESIAN_POINT('Ctrl Pts',(65.700054515563,243.998949933896,20.6059490395096)) ;
#91924=CARTESIAN_POINT('Ctrl Pts',(65.7805181325764,244.240689785211,20.4789530628307)) ;
#91925=CARTESIAN_POINT('Ctrl Pts',(65.7285125559214,244.171669922872,20.5440259656052)) ;
#91926=CARTESIAN_POINT('Ctrl Pts',(65.6997809923943,244.085431815184,20.5799791663286)) ;
#91927=CARTESIAN_POINT('Ctrl Pts',(65.7000010583238,243.99901433175,20.5797037872052)) ;
#91928=CARTESIAN_POINT('',(65.7,244.,20.5798989873224)) ;
#91929=CARTESIAN_POINT('Origin',(66.1,244.,20.0798989873224)) ;
#91930=CARTESIAN_POINT('',(65.7000000000001,244.16843697471,20.6213203435596)) ;
#91931=CARTESIAN_POINT('Ctrl Pts',(65.7,244.,20.5798989873224)) ;
#91932=CARTESIAN_POINT('Ctrl Pts',(65.7,244.00020850453,20.5800024812788)) ;
#91933=CARTESIAN_POINT('Ctrl Pts',(65.7,244.000417086861,20.5801058143326)) ;
#91934=CARTESIAN_POINT('Ctrl Pts',(65.7,244.02719444846,20.5933458356417)) ;
#91935=CARTESIAN_POINT('Ctrl Pts',(65.7,244.054565273668,20.6036388887893)) ;
#91936=CARTESIAN_POINT('Ctrl Pts',(65.7,244.105754615284,20.6163080294349)) ;
#91937=CARTESIAN_POINT('Ctrl Pts',(65.7,244.128852047872,20.619808090116)) ;
#91938=CARTESIAN_POINT('Ctrl Pts',(65.7,244.157377176375,20.6211837882661)) ;
#91939=CARTESIAN_POINT('Ctrl Pts',(65.7,244.162669920017,20.621315414962)) ;
#91940=CARTESIAN_POINT('Ctrl Pts',(65.7,244.167963343701,20.6213203435597)) ;
#91941=CARTESIAN_POINT('Origin',(66.1707106781187,244.,20.150609665441)) ;
#91942=CARTESIAN_POINT('Origin',(66.1,244.,24.0213203435596)) ;
#91943=CARTESIAN_POINT('',(66.1,244.4,18.0918966374184)) ;
#91944=CARTESIAN_POINT('',(66.1,244.4,24.0213203435596)) ;
#91945=CARTESIAN_POINT('',(65.8848651777997,244.337219525349,18.0777011469026)) ;
#91946=CARTESIAN_POINT('Ctrl Pts',(65.8848651777997,244.337219525349,18.0777011469026)) ;
#91947=CARTESIAN_POINT('Ctrl Pts',(65.9479936757444,244.377493403818,18.0877696165197)) ;
#91948=CARTESIAN_POINT('Ctrl Pts',(66.0239249506928,244.4,18.0918966374184)) ;
#91949=CARTESIAN_POINT('Ctrl Pts',(66.1,244.4,18.0918966374184)) ;
#91950=CARTESIAN_POINT('',(65.7,244.,17.9933962655652)) ;
#91951=CARTESIAN_POINT('Origin',(66.1,244.,17.9933962655652)) ;
#91952=CARTESIAN_POINT('',(65.7,244.,24.0213203435596)) ;
#91953=CARTESIAN_POINT('Origin',(67.55,249.825,18.7713203435596)) ;
#91954=CARTESIAN_POINT('',(66.8292893218814,245.358578643763,19.4920310216783)) ;
#91955=CARTESIAN_POINT('',(66.8944035593729,245.423692881254,19.4269167841868)) ;
#91956=CARTESIAN_POINT('',(66.8292893218813,251.970710678119,19.4920310216783)) ;
#91957=CARTESIAN_POINT('',(66.8292893218813,250.2125,19.4920310216783)) ;
#91958=CARTESIAN_POINT('',(68.0684336611227,250.731566338877,18.2528866824369)) ;
#91959=CARTESIAN_POINT('',(66.7125,252.0875,19.6088203435596)) ;
#91960=CARTESIAN_POINT('',(68.2414088145807,250.644888384771,18.0799115289789)) ;
#91961=CARTESIAN_POINT('Ctrl Pts',(68.0684336611227,250.731566338877,18.2528866824369)) ;
#91962=CARTESIAN_POINT('Ctrl Pts',(68.0965609814737,250.703439018526,18.2247593620858)) ;
#91963=CARTESIAN_POINT('Ctrl Pts',(68.1259419662347,250.677664283059,18.1953783773249)) ;
#91964=CARTESIAN_POINT('Ctrl Pts',(68.1716540835089,250.650783089379,18.1496662600507)) ;
#91965=CARTESIAN_POINT('Ctrl Pts',(68.1899702972436,250.642873774853,18.131350046316)) ;
#91966=CARTESIAN_POINT('Ctrl Pts',(68.2192212579585,250.639466445032,18.1020990856011)) ;
#91967=CARTESIAN_POINT('Ctrl Pts',(68.2306528427947,250.640367277029,18.0906675007649)) ;
#91968=CARTESIAN_POINT('Ctrl Pts',(68.2413962729241,250.644887148136,18.0799240706355)) ;
#91969=CARTESIAN_POINT('',(68.2414213562374,244.521708245126,18.0798989873223)) ;
#91970=CARTESIAN_POINT('',(68.2414213562373,249.4375,18.0798989873223)) ;
#91971=CARTESIAN_POINT('Origin',(69.1914213562374,244.521708245126,17.1298989873223)) ;
#91972=CARTESIAN_POINT('Origin',(66.8000000000001,244.4,24.0213203435596)) ;
#91973=CARTESIAN_POINT('',(61.8303059750075,244.4,18.0918966374184)) ;
#91974=CARTESIAN_POINT('Origin',(61.8303059750075,244.3,18.0918966374184)) ;
#91975=CARTESIAN_POINT('',(66.1,244.326083322956,17.9953582499056)) ;
#91976=CARTESIAN_POINT('',(61.8303059750075,244.326083322956,17.9953582499056)) ;
#91977=CARTESIAN_POINT('Origin',(66.1,244.3,18.0918966374184)) ;
#91978=CARTESIAN_POINT('Origin',(65.4568347953872,224.289496829998,16.1213203435596)) ;
#91979=CARTESIAN_POINT('',(65.3568347953872,216.946231446812,16.1213203435596)) ;
#91980=CARTESIAN_POINT('Origin',(65.4568347953872,216.846231446812,16.1213203435596)) ;
#91981=CARTESIAN_POINT('',(65.3568347953872,218.546231446812,16.1213203435596)) ;
#91982=CARTESIAN_POINT('',(65.3568347953872,224.289496829998,16.1213203435596)) ;
#91983=CARTESIAN_POINT('Ctrl Pts',(65.3568347953872,218.546231446812,16.1213203435596)) ;
#91984=CARTESIAN_POINT('Ctrl Pts',(65.3568347953872,218.546231446812,16.1153496356238)) ;
#91985=CARTESIAN_POINT('Ctrl Pts',(65.3573695167032,218.547300046631,16.1095515196401)) ;
#91986=CARTESIAN_POINT('Ctrl Pts',(65.3595546370681,218.551678573484,16.0971310298406)) ;
#91987=CARTESIAN_POINT('Ctrl Pts',(65.3613915100209,218.555365057847,16.0908852637126)) ;
#91988=CARTESIAN_POINT('Ctrl Pts',(65.3670367701187,218.566751467664,16.0762602049506)) ;
#91989=CARTESIAN_POINT('Ctrl Pts',(65.3714692053955,218.57574568164,16.0686738511528)) ;
#91990=CARTESIAN_POINT('Ctrl Pts',(65.3839732164585,218.601374810389,16.0514969265816)) ;
#91991=CARTESIAN_POINT('Ctrl Pts',(65.3941167652591,218.622413030244,16.0422484417149)) ;
#91992=CARTESIAN_POINT('Ctrl Pts',(65.4209791942954,218.679766384964,16.0263264775169)) ;
#91993=CARTESIAN_POINT('Ctrl Pts',(65.4380196034223,218.717236626393,16.0215749505388)) ;
#91994=CARTESIAN_POINT('Ctrl Pts',(65.455898201062,218.758429093735,16.0213236297566)) ;
#91995=CARTESIAN_POINT('Ctrl Pts',(65.4563667355281,218.759509862814,16.0213203435596)) ;
#91996=CARTESIAN_POINT('Ctrl Pts',(65.4568347953872,218.760590800757,16.0213203435596)) ;
#91997=CARTESIAN_POINT('Origin',(64.1568347953872,220.146231446812,16.1213203435596)) ;
#91998=CARTESIAN_POINT('',(62.9568347953872,218.546231446812,16.1213203435596)) ;
#91999=CARTESIAN_POINT('Origin',(64.1568347953872,220.146231446812,16.1213203435596)) ;
#92000=CARTESIAN_POINT('Ctrl Pts',(62.9568347953872,218.546231446812,16.1213203435596)) ;
#92001=CARTESIAN_POINT('Ctrl Pts',(62.9568347953872,218.546231446812,16.1153496356239)) ;
#92002=CARTESIAN_POINT('Ctrl Pts',(62.9563000740712,218.547300046631,16.1095515196403)) ;
#92003=CARTESIAN_POINT('Ctrl Pts',(62.9541149537063,218.551678573484,16.0971310298406)) ;
#92004=CARTESIAN_POINT('Ctrl Pts',(62.9522780807535,218.555365057847,16.0908852637126)) ;
#92005=CARTESIAN_POINT('Ctrl Pts',(62.9466328206557,218.566751467664,16.0762602049506)) ;
#92006=CARTESIAN_POINT('Ctrl Pts',(62.942200385379,218.57574568164,16.0686738511528)) ;
#92007=CARTESIAN_POINT('Ctrl Pts',(62.929696374316,218.601374810389,16.0514969265817)) ;
#92008=CARTESIAN_POINT('Ctrl Pts',(62.9195528255154,218.622413030244,16.042248441715)) ;
#92009=CARTESIAN_POINT('Ctrl Pts',(62.8926903964743,218.679766384974,16.0263264775141)) ;
#92010=CARTESIAN_POINT('Ctrl Pts',(62.875649987346,218.717236626407,16.0215749505387)) ;
#92011=CARTESIAN_POINT('Ctrl Pts',(62.8577713897124,218.758429093735,16.0213236297566)) ;
#92012=CARTESIAN_POINT('Ctrl Pts',(62.8573028552463,218.759509862814,16.0213203435596)) ;
#92013=CARTESIAN_POINT('Ctrl Pts',(62.8568347953872,218.760590800757,16.0213203435596)) ;
#92014=CARTESIAN_POINT('Origin',(62.8568347953872,223.489496829998,16.1213203435596)) ;
#92015=CARTESIAN_POINT('',(62.9568347953872,216.946231446812,16.1213203435596)) ;
#92016=CARTESIAN_POINT('',(62.9568347953872,223.489496829998,16.1213203435596)) ;
#92017=CARTESIAN_POINT('Origin',(62.8568347953872,216.846231446812,16.1213203435596)) ;
#92018=CARTESIAN_POINT('Origin',(67.7248479331787,216.846231446812,16.1213203435596)) ;
#92019=CARTESIAN_POINT('',(67.7248479331787,216.946231446812,16.1213203435596)) ;
#92020=CARTESIAN_POINT('Origin',(64.1568347953872,220.146231446812,18.0213203435596)) ;
#92021=CARTESIAN_POINT('',(65.3568347953872,218.546231446812,23.3713203435596)) ;
#92022=CARTESIAN_POINT('',(65.3568347953872,218.546231446812,18.0213203435596)) ;
#92023=CARTESIAN_POINT('',(62.9568347953872,218.546231446812,23.3713203435596)) ;
#92024=CARTESIAN_POINT('Origin',(64.1568347953872,220.146231446812,23.3713203435596)) ;
#92025=CARTESIAN_POINT('',(62.9568347953872,218.546231446812,18.0213203435596)) ;
#92026=CARTESIAN_POINT('Origin',(65.3568347953872,218.546231446812,18.0213203435596)) ;
#92027=CARTESIAN_POINT('',(65.3568347953872,216.946231446812,23.3713203435596)) ;
#92028=CARTESIAN_POINT('',(65.3568347953872,216.946231446812,18.0213203435596)) ;
#92029=CARTESIAN_POINT('',(65.3568347953872,219.383251285823,23.3713203435596)) ;
#92030=CARTESIAN_POINT('Origin',(70.0928610709702,230.032762213184,16.0213203435596)) ;
#92031=CARTESIAN_POINT('Ctrl Pts',(70.9999999999998,217.874644018271,23.2713203435596)) ;
#92032=CARTESIAN_POINT('Ctrl Pts',(70.9999999999998,217.769924263151,23.3236802211194)) ;
#92033=CARTESIAN_POINT('Ctrl Pts',(70.9523598775596,217.674644018271,23.3713203435597)) ;
#92034=CARTESIAN_POINT('Ctrl Pts',(70.8999999999997,217.674644018271,23.3713203435596)) ;
#92035=CARTESIAN_POINT('Ctrl Pts',(70.9999999999998,217.874644018271,23.2713203435596)) ;
#92036=CARTESIAN_POINT('Ctrl Pts',(70.9999999999998,217.779897573163,23.3336535311308)) ;
#92037=CARTESIAN_POINT('Ctrl Pts',(70.9364586273346,217.704563948305,23.3713203435597)) ;
#92038=CARTESIAN_POINT('Ctrl Pts',(70.8999999999997,217.704563948305,23.3713203435596)) ;
#92039=CARTESIAN_POINT('Ctrl Pts',(70.9999999999998,217.874644018271,23.2713203435596)) ;
#92040=CARTESIAN_POINT('Ctrl Pts',(70.9999999999998,217.797350865682,23.3511068236508)) ;
#92041=CARTESIAN_POINT('Ctrl Pts',(70.9227974276425,217.756340925332,23.3964525020675)) ;
#92042=CARTESIAN_POINT('Ctrl Pts',(70.8999999999997,217.756340925332,23.3964525020674)) ;
#92043=CARTESIAN_POINT('Ctrl Pts',(70.9999999999998,217.874644018271,23.2713203435596)) ;
#92044=CARTESIAN_POINT('Ctrl Pts',(70.9999999999998,217.814804158202,23.3685601161707)) ;
#92045=CARTESIAN_POINT('Ctrl Pts',(70.9405918277816,217.774644018271,23.448880396034)) ;
#92046=CARTESIAN_POINT('Ctrl Pts',(70.8999999999998,217.774644018271,23.448880396034)) ;
#92047=CARTESIAN_POINT('Ctrl Pts',(70.9999999999998,217.874644018271,23.2713203435596)) ;
#92048=CARTESIAN_POINT('Ctrl Pts',(70.9999999999998,217.822284140711,23.3760400986793)) ;
#92049=CARTESIAN_POINT('Ctrl Pts',(70.9523598775596,217.774644018271,23.4713203435597)) ;
#92050=CARTESIAN_POINT('Ctrl Pts',(70.8999999999998,217.774644018271,23.4713203435596)) ;
#92051=CARTESIAN_POINT('',(70.8999999999998,217.774644018271,23.4713203435596)) ;
#92052=CARTESIAN_POINT('',(70.8999999999998,217.674644018271,23.3713203435596)) ;
#92053=CARTESIAN_POINT('Origin',(70.8999999999998,217.674644018271,23.4713203435596)) ;
#92054=CARTESIAN_POINT('',(70.9999999999998,217.874644018271,23.2713203435596)) ;
#92055=CARTESIAN_POINT('Origin',(70.8999999999998,217.874644018271,23.2713203435596)) ;
#92056=CARTESIAN_POINT('Origin',(70.8999999999998,217.874644018271,23.2713203435596)) ;
#92057=CARTESIAN_POINT('Origin',(70.8999999999998,217.874644018271,23.4713203435596)) ;
#92058=CARTESIAN_POINT('',(70.8292893218811,217.803933340152,23.4713203435596)) ;
#92059=CARTESIAN_POINT('',(70.7585786437625,217.733222662034,23.3713203435596)) ;
#92060=CARTESIAN_POINT('Origin',(70.7585786437625,217.733222662034,23.4713203435596)) ;
#92061=CARTESIAN_POINT('Origin',(70.8999999999998,217.874644018271,23.3713203435596)) ;
#92062=CARTESIAN_POINT('Origin',(70.8999999999998,217.874644018271,23.4713203435596)) ;
#92063=CARTESIAN_POINT('Origin',(68.9405576113038,219.551243694493,23.4713203435596)) ;
#92064=CARTESIAN_POINT('',(70.3022814706893,218.330941191344,23.4713203435596)) ;
#92065=CARTESIAN_POINT('',(70.2965036217263,218.19529768407,23.3713203435596)) ;
#92066=CARTESIAN_POINT('Ctrl Pts',(70.3022814706893,218.330941191344,23.4713203435596)) ;
#92067=CARTESIAN_POINT('Ctrl Pts',(70.3022814706893,218.330941191344,23.4686610045557)) ;
#92068=CARTESIAN_POINT('Ctrl Pts',(70.3022750583344,218.330797598238,23.4659926797098)) ;
#92069=CARTESIAN_POINT('Ctrl Pts',(70.3022621053397,218.330507410458,23.4633214758633)) ;
#92070=CARTESIAN_POINT('Ctrl Pts',(70.3022111056997,218.329364858277,23.4528041832813)) ;
#92071=CARTESIAN_POINT('Ctrl Pts',(70.3020610895237,218.326006195641,23.4427364614383)) ;
#92072=CARTESIAN_POINT('Ctrl Pts',(70.3018321156343,218.320842621681,23.4334247968396)) ;
#92073=CARTESIAN_POINT('Ctrl Pts',(70.3015498927103,218.314478232516,23.4219476576061)) ;
#92074=CARTESIAN_POINT('Ctrl Pts',(70.301157583221,218.305588184557,23.4119860626266)) ;
#92075=CARTESIAN_POINT('Ctrl Pts',(70.3007081862357,218.295273815532,23.4036949689328)) ;
#92076=CARTESIAN_POINT('Ctrl Pts',(70.3001000495539,218.281316120313,23.3924752269849)) ;
#92077=CARTESIAN_POINT('Ctrl Pts',(70.2993569279694,218.264052061823,23.3837359173529)) ;
#92078=CARTESIAN_POINT('Ctrl Pts',(70.2985424369338,218.244676672633,23.378163997948)) ;
#92079=CARTESIAN_POINT('Ctrl Pts',(70.298181690018,218.236095102564,23.3756961343958)) ;
#92080=CARTESIAN_POINT('Ctrl Pts',(70.2978143471974,218.227276100269,23.3739026646164)) ;
#92081=CARTESIAN_POINT('Ctrl Pts',(70.2974470041422,218.218368678155,23.372772614714)) ;
#92082=CARTESIAN_POINT('Ctrl Pts',(70.2972143560673,218.212727372083,23.3720569242152)) ;
#92083=CARTESIAN_POINT('Ctrl Pts',(70.2969809616316,218.207032740452,23.3716050323275)) ;
#92084=CARTESIAN_POINT('Ctrl Pts',(70.296748280518,218.201319022744,23.3714185485914)) ;
#92085=CARTESIAN_POINT('Ctrl Pts',(70.2966666747561,218.199315111556,23.3713531451423)) ;
#92086=CARTESIAN_POINT('Ctrl Pts',(70.296585101217,218.197307504869,23.3713203435596)) ;
#92087=CARTESIAN_POINT('Ctrl Pts',(70.2965036217263,218.19529768407,23.3713203435596)) ;
#92088=CARTESIAN_POINT('',(68.9405576113038,219.551243694493,23.3713203435596)) ;
#92089=CARTESIAN_POINT('',(69.0112682894225,219.621954372611,23.4713203435596)) ;
#92090=CARTESIAN_POINT('Origin',(70.9999999999998,217.633222662033,29.5213203435596)) ;
#92091=CARTESIAN_POINT('',(70.8292893218811,217.803933340152,30.7213203435596)) ;
#92092=CARTESIAN_POINT('',(70.8292893218811,217.803933340152,29.5213203435596)) ;
#92093=CARTESIAN_POINT('',(70.4999999999998,218.133222662034,30.7213203435596)) ;
#92094=CARTESIAN_POINT('',(70.9999999999998,217.633222662033,30.7213203435596)) ;
#92095=CARTESIAN_POINT('',(70.4999999999998,218.133222662034,29.5213203435596)) ;
#92096=CARTESIAN_POINT('',(70.4999999999998,218.133222662034,30.7213203435596)) ;
#92097=CARTESIAN_POINT('',(70.3022814706893,218.330941191344,29.5213203435596)) ;
#92098=CARTESIAN_POINT('',(70.9999999999998,217.633222662033,29.5213203435596)) ;
#92099=CARTESIAN_POINT('',(70.3022814706893,218.330941191344,23.3713203435596)) ;
#92100=CARTESIAN_POINT('Origin',(70.8999999999998,217.874644018271,29.5213203435596)) ;
#92101=CARTESIAN_POINT('',(70.9999999999998,217.874644018271,30.7213203435596)) ;
#92102=CARTESIAN_POINT('',(70.9999999999998,217.874644018271,29.5213203435596)) ;
#92103=CARTESIAN_POINT('Origin',(70.8999999999998,217.874644018271,30.7213203435596)) ;
#92104=CARTESIAN_POINT('Origin',(70.8999999999999,220.262790180756,23.2713203435596)) ;
#92105=CARTESIAN_POINT('',(70.8999999999998,217.165524426368,23.3713203435596)) ;
#92106=CARTESIAN_POINT('',(70.8999999999999,220.262790180756,23.3713203435596)) ;
#92107=CARTESIAN_POINT('',(70.9999999999998,217.165524426368,23.2713203435596)) ;
#92108=CARTESIAN_POINT('Origin',(70.8999999999998,217.165524426368,23.2713203435596)) ;
#92109=CARTESIAN_POINT('',(70.9999999999999,220.262790180756,23.2713203435596)) ;
#92110=CARTESIAN_POINT('Origin',(82.8283628290598,253.933159539856,29.6213203435596)) ;
#92111=CARTESIAN_POINT('',(82.8990735071784,254.003870217975,29.6213203435596)) ;
#92112=CARTESIAN_POINT('',(82.9283628290598,253.933159539856,29.6213203435596)) ;
#92113=CARTESIAN_POINT('Origin',(82.8283628290598,253.933159539856,29.6213203435596)) ;
#92114=CARTESIAN_POINT('',(82.8283628290598,253.933159539856,29.5213203435596)) ;
#92115=CARTESIAN_POINT('Origin',(82.8283628290598,253.933159539856,29.6213203435596)) ;
#92116=CARTESIAN_POINT('Origin',(82.8283628290598,253.933159539856,29.6213203435596)) ;
#92117=CARTESIAN_POINT('Origin',(79.2435991885767,257.517923180339,29.6213203435596)) ;
#92118=CARTESIAN_POINT('',(79.2435991885767,257.517923180339,29.5213203435596)) ;
#92119=CARTESIAN_POINT('',(79.3143098666953,257.588633858457,29.6213203435596)) ;
#92120=CARTESIAN_POINT('Origin',(82.8283628290597,243.983954368305,29.6213203435596)) ;
#92121=CARTESIAN_POINT('',(82.9283628290597,243.983954368305,29.6213203435596)) ;
#92122=CARTESIAN_POINT('',(82.8283628290597,243.983954368305,29.5213203435596)) ;
#92123=CARTESIAN_POINT('Origin',(82.8283628290598,253.933159539856,30.6213203435596)) ;
#92124=CARTESIAN_POINT('',(82.9283628290598,253.933159539856,30.6213203435596)) ;
#92125=CARTESIAN_POINT('',(82.8990735071784,254.003870217975,30.6213203435596)) ;
#92126=CARTESIAN_POINT('Origin',(82.8283628290598,253.933159539856,30.6213203435596)) ;
#92127=CARTESIAN_POINT('',(83.0283628290598,253.933159539856,30.7213203435596)) ;
#92128=CARTESIAN_POINT('Origin',(83.0283628290598,253.933159539856,30.6213203435596)) ;
#92129=CARTESIAN_POINT('',(82.9697841852971,254.074580896093,30.7213203435596)) ;
#92130=CARTESIAN_POINT('Origin',(82.8283628290598,253.933159539856,30.7213203435596)) ;
#92131=CARTESIAN_POINT('Origin',(82.9697841852971,254.074580896093,30.6213203435596)) ;
#92132=CARTESIAN_POINT('Origin',(83.0283628290597,249.051115370458,30.6213203435596)) ;
#92133=CARTESIAN_POINT('',(83.0283628290597,249.051115370458,30.7213203435596)) ;
#92134=CARTESIAN_POINT('',(82.9283628290597,249.051115370458,30.6213203435596)) ;
#92135=CARTESIAN_POINT('Origin',(83.6439567661249,253.400408315266,30.6213203435596)) ;
#92136=CARTESIAN_POINT('',(83.5732460880063,253.329697637147,30.6213203435596)) ;
#92137=CARTESIAN_POINT('',(83.6439567661249,253.400408315266,30.7213203435596)) ;
#92138=CARTESIAN_POINT('Origin',(82.8283628290598,253.933159539856,30.7213203435596)) ;
#92139=CARTESIAN_POINT('',(82.9283628290598,253.933159539856,30.7213203435596)) ;
#92140=CARTESIAN_POINT('',(82.8990735071784,254.003870217975,30.7213203435596)) ;
#92141=CARTESIAN_POINT('Origin',(55.2141814145299,240.716611331017,29.5213203435596)) ;
#92142=CARTESIAN_POINT('',(77.6,262.6,29.5213203435596)) ;
#92143=CARTESIAN_POINT('',(65.4845247720936,253.51339357907,29.5213203435596)) ;
#92144=CARTESIAN_POINT('',(77.2,261.8,29.5213203435596)) ;
#92145=CARTESIAN_POINT('Origin',(78.2,261.8,29.5213203435596)) ;
#92146=CARTESIAN_POINT('',(77.2,257.723534352175,29.5213203435596)) ;
#92147=CARTESIAN_POINT('',(77.2,257.,29.5213203435596)) ;
#92148=CARTESIAN_POINT('',(77.25,256.652146641849,29.5213203435596)) ;
#92149=CARTESIAN_POINT('Origin',(73.2,257.,29.5213203435596)) ;
#92150=CARTESIAN_POINT('',(77.25,255.5,29.5213203435596)) ;
#92151=CARTESIAN_POINT('',(77.25,248.684378986433,29.5213203435596)) ;
#92152=CARTESIAN_POINT('',(76.7766604535517,253.6,29.5213203435596)) ;
#92153=CARTESIAN_POINT('Origin',(73.2,255.5,29.5213203435596)) ;
#92154=CARTESIAN_POINT('',(80.1,253.6,29.5213203435596)) ;
#92155=CARTESIAN_POINT('',(80.1,253.6,29.5213203435596)) ;
#92156=CARTESIAN_POINT('',(80.3,253.4,29.5213203435596)) ;
#92157=CARTESIAN_POINT('Origin',(80.1,253.4,29.5213203435596)) ;
#92158=CARTESIAN_POINT('',(80.3,252.400000000001,29.5213203435596)) ;
#92159=CARTESIAN_POINT('',(80.3,252.400000000001,29.5213203435596)) ;
#92160=CARTESIAN_POINT('',(80.2,252.400000000001,29.5213203435596)) ;
#92161=CARTESIAN_POINT('',(80.2,252.400000000001,29.5213203435596)) ;
#92162=CARTESIAN_POINT('',(80.2,249.600000000004,29.5213203435596)) ;
#92163=CARTESIAN_POINT('',(80.2,249.600000000004,29.5213203435596)) ;
#92164=CARTESIAN_POINT('',(80.2999999999999,249.600000000004,29.5213203435596)) ;
#92165=CARTESIAN_POINT('',(80.2999999999999,249.600000000004,29.5213203435596)) ;
#92166=CARTESIAN_POINT('',(80.2999999999999,248.6,29.5213203435596)) ;
#92167=CARTESIAN_POINT('',(80.2999999999999,248.6,29.5213203435596)) ;
#92168=CARTESIAN_POINT('',(80.0999999999999,248.4,29.5213203435596)) ;
#92169=CARTESIAN_POINT('Origin',(80.0999999999999,248.6,29.5213203435596)) ;
#92170=CARTESIAN_POINT('',(76.0414213562372,248.4,29.5213203435596)) ;
#92171=CARTESIAN_POINT('',(76.0414213562372,248.4,29.5213203435596)) ;
#92172=CARTESIAN_POINT('',(75.8999999999999,248.458578643763,29.5213203435596)) ;
#92173=CARTESIAN_POINT('Origin',(76.0414213562372,248.6,29.5213203435596)) ;
#92174=CARTESIAN_POINT('',(75.1585786437627,249.2,29.5213203435596)) ;
#92175=CARTESIAN_POINT('',(75.1585786437627,249.2,29.5213203435596)) ;
#92176=CARTESIAN_POINT('',(75.1,249.341421356237,29.5213203435596)) ;
#92177=CARTESIAN_POINT('Origin',(75.3,249.341421356237,29.5213203435596)) ;
#92178=CARTESIAN_POINT('',(75.1,251.923339546448,29.5213203435596)) ;
#92179=CARTESIAN_POINT('',(75.1,252.658578643763,29.5213203435596)) ;
#92180=CARTESIAN_POINT('',(69.15,255.5,29.5213203435596)) ;
#92181=CARTESIAN_POINT('Origin',(73.2,255.5,29.5213203435596)) ;
#92182=CARTESIAN_POINT('',(69.15,256.652146641849,29.5213203435596)) ;
#92183=CARTESIAN_POINT('',(69.15,248.108305665508,29.5213203435596)) ;
#92184=CARTESIAN_POINT('',(69.1350889359327,257.,29.5213203435596)) ;
#92185=CARTESIAN_POINT('Origin',(73.2,257.,29.5213203435596)) ;
#92186=CARTESIAN_POINT('',(69.1350889359328,261.466666666667,29.5213203435596)) ;
#92187=CARTESIAN_POINT('',(69.1350889359327,257.,29.5213203435596)) ;
#92188=CARTESIAN_POINT('',(68.9350889359328,262.066666666667,29.5213203435596)) ;
#92189=CARTESIAN_POINT('Origin',(68.1350889359328,261.466666666667,29.5213203435596)) ;
#92190=CARTESIAN_POINT('',(67.6350889359328,263.8,29.5213203435596)) ;
#92191=CARTESIAN_POINT('',(71.3143388626363,258.894333431062,29.5213203435596)) ;
#92192=CARTESIAN_POINT('',(57.2649110640674,263.8,29.5213203435596)) ;
#92193=CARTESIAN_POINT('',(55.2649110640674,263.8,29.5213203435596)) ;
#92194=CARTESIAN_POINT('',(55.6649110640674,262.6,29.5213203435596)) ;
#92195=CARTESIAN_POINT('',(50.5686642956594,258.777814923694,29.5213203435596)) ;
#92196=CARTESIAN_POINT('',(55.2649110640674,261.8,29.5213203435596)) ;
#92197=CARTESIAN_POINT('Origin',(56.2649110640674,261.8,29.5213203435596)) ;
#92198=CARTESIAN_POINT('',(55.2649110640674,257.,29.5213203435596)) ;
#92199=CARTESIAN_POINT('',(55.2649110640674,257.,29.5213203435596)) ;
#92200=CARTESIAN_POINT('',(55.25,256.652146641849,29.5213203435596)) ;
#92201=CARTESIAN_POINT('Origin',(51.2,257.,29.5213203435596)) ;
#92202=CARTESIAN_POINT('',(55.25,255.5,29.5213203435596)) ;
#92203=CARTESIAN_POINT('',(55.25,248.684378986433,29.5213203435596)) ;
#92204=CARTESIAN_POINT('',(47.15,255.5,29.5213203435596)) ;
#92205=CARTESIAN_POINT('Origin',(51.2,255.5,29.5213203435596)) ;
#92206=CARTESIAN_POINT('',(47.15,256.652146641849,29.5213203435596)) ;
#92207=CARTESIAN_POINT('',(47.15,248.108305665508,29.5213203435596)) ;
#92208=CARTESIAN_POINT('',(47.1350889359327,257.,29.5213203435596)) ;
#92209=CARTESIAN_POINT('Origin',(51.2,257.,29.5213203435596)) ;
#92210=CARTESIAN_POINT('',(47.1350889359327,261.466666666667,29.5213203435596)) ;
#92211=CARTESIAN_POINT('',(47.1350889359327,259.8,29.5213203435596)) ;
#92212=CARTESIAN_POINT('',(46.9350889359326,262.066666666667,29.5213203435596)) ;
#92213=CARTESIAN_POINT('Origin',(46.1350889359327,261.466666666667,29.5213203435596)) ;
#92214=CARTESIAN_POINT('',(45.6350889359327,263.8,29.5213203435596)) ;
#92215=CARTESIAN_POINT('',(53.2743388626362,253.614333431062,29.5213203435596)) ;
#92216=CARTESIAN_POINT('',(26.7,263.8,29.5213203435596)) ;
#92217=CARTESIAN_POINT('',(47.1350889359327,263.8,29.5213203435596)) ;
#92218=CARTESIAN_POINT('',(26.7,245.5,29.5213203435596)) ;
#92219=CARTESIAN_POINT('',(26.7,252.258305665508,29.5213203435596)) ;
#92220=CARTESIAN_POINT('',(33.8,245.5,29.5213203435596)) ;
#92221=CARTESIAN_POINT('',(40.957090707265,245.5,29.5213203435596)) ;
#92222=CARTESIAN_POINT('',(33.8,248.9,29.5213203435596)) ;
#92223=CARTESIAN_POINT('',(33.8,243.108305665508,29.5213203435596)) ;
#92224=CARTESIAN_POINT('',(34.1,248.9,29.5213203435596)) ;
#92225=CARTESIAN_POINT('',(44.507090707265,248.9,29.5213203435596)) ;
#92226=CARTESIAN_POINT('',(34.2732050807569,249.,29.5213203435596)) ;
#92227=CARTESIAN_POINT('Ctrl Pts',(34.1,248.9,29.5213203435596)) ;
#92228=CARTESIAN_POINT('Ctrl Pts',(34.1277098222081,248.927709822208,29.5213203435596)) ;
#92229=CARTESIAN_POINT('Ctrl Pts',(34.1615223272204,248.960391271619,29.5213203435596)) ;
#92230=CARTESIAN_POINT('Ctrl Pts',(34.2184730473151,248.99104280001,29.5213203435596)) ;
#92231=CARTESIAN_POINT('Ctrl Pts',(34.2477173385693,249.,29.5213203435596)) ;
#92232=CARTESIAN_POINT('Ctrl Pts',(34.2732050807569,249.,29.5213203435596)) ;
#92233=CARTESIAN_POINT('',(46.1267949192431,249.,29.5213203435596)) ;
#92234=CARTESIAN_POINT('',(46.1267949192431,249.,29.5213203435596)) ;
#92235=CARTESIAN_POINT('',(46.3,248.9,29.5213203435596)) ;
#92236=CARTESIAN_POINT('Ctrl Pts',(46.1267949192431,249.,29.5213203435596)) ;
#92237=CARTESIAN_POINT('Ctrl Pts',(46.1522826614306,249.,29.5213203435596)) ;
#92238=CARTESIAN_POINT('Ctrl Pts',(46.1815269526849,248.99104280001,29.5213203435596)) ;
#92239=CARTESIAN_POINT('Ctrl Pts',(46.2384776727796,248.960391271619,29.5213203435596)) ;
#92240=CARTESIAN_POINT('Ctrl Pts',(46.2722901777919,248.927709822208,29.5213203435596)) ;
#92241=CARTESIAN_POINT('Ctrl Pts',(46.3,248.9,29.5213203435596)) ;
#92242=CARTESIAN_POINT('',(47.2,248.9,29.5213203435596)) ;
#92243=CARTESIAN_POINT('',(50.757090707265,248.9,29.5213203435596)) ;
#92244=CARTESIAN_POINT('',(47.2,246.,29.5213203435596)) ;
#92245=CARTESIAN_POINT('',(47.2,244.808305665508,29.5213203435596)) ;
#92246=CARTESIAN_POINT('',(55.3573593128808,246.,29.5213203435596)) ;
#92247=CARTESIAN_POINT('',(51.207090707265,246.,29.5213203435596)) ;
#92248=CARTESIAN_POINT('',(56.9573593128808,244.4,29.5213203435596)) ;
#92249=CARTESIAN_POINT('Origin',(55.3573593128808,244.4,29.5213203435596)) ;
#92250=CARTESIAN_POINT('',(56.9573593128807,226.261195155516,29.5213203435596)) ;
#92251=CARTESIAN_POINT('',(56.9573593128808,242.558305665508,29.5213203435596)) ;
#92252=CARTESIAN_POINT('',(57.4999031800138,224.540465846463,29.5213203435596)) ;
#92253=CARTESIAN_POINT('Origin',(59.9573593128807,226.261195155516,29.5213203435596)) ;
#92254=CARTESIAN_POINT('',(60.5916108526749,220.125049696322,29.5213203435596)) ;
#92255=CARTESIAN_POINT('',(53.3237623239525,230.504613085921,29.5213203435596)) ;
#92256=CARTESIAN_POINT('',(60.5916108526749,220.645409008718,29.5213203435596)) ;
#92257=CARTESIAN_POINT('',(60.5916108526749,230.681010169868,29.5213203435596)) ;
#92258=CARTESIAN_POINT('',(63.1200364144528,223.593701405679,29.5213203435596)) ;
#92259=CARTESIAN_POINT('Origin',(64.1568347953872,220.146231446812,29.5213203435596)) ;
#92260=CARTESIAN_POINT('',(63.8582048387328,224.775017823302,29.5213203435596)) ;
#92261=CARTESIAN_POINT('',(60.2066749117936,218.931348397394,29.5213203435596)) ;
#92262=CARTESIAN_POINT('',(64.9830939940346,223.650128668,29.5213203435596)) ;
#92263=CARTESIAN_POINT('',(70.9999999999998,217.633222662033,29.5213203435596)) ;
#92264=CARTESIAN_POINT('',(67.2791272966079,221.938238572027,29.5213203435596)) ;
#92265=CARTESIAN_POINT('Origin',(64.1568347953872,220.146231446812,29.5213203435596)) ;
#92266=CARTESIAN_POINT('',(70.3850625789433,219.622496965577,29.5213203435596)) ;
#92267=CARTESIAN_POINT('',(60.4556364138638,227.025737280796,29.5213203435596)) ;
#92268=CARTESIAN_POINT('Ctrl Pts',(70.3850625789433,219.622496965577,29.5213203435596)) ;
#92269=CARTESIAN_POINT('Ctrl Pts',(70.3511920182576,219.216626210409,29.5213203435596)) ;
#92270=CARTESIAN_POINT('Ctrl Pts',(70.3247455954692,218.811352574561,29.5213203435596)) ;
#92271=CARTESIAN_POINT('Ctrl Pts',(70.305749879039,218.406678194919,29.5213203435596)) ;
#92272=CARTESIAN_POINT('Ctrl Pts',(70.3045647190314,218.381430192685,29.5213203435596)) ;
#92273=CARTESIAN_POINT('Ctrl Pts',(70.3034085785548,218.356184524476,29.5213203435596)) ;
#92274=CARTESIAN_POINT('Ctrl Pts',(70.3022814706893,218.330941191344,29.5213203435596)) ;
#92275=CARTESIAN_POINT('',(70.4999999999999,220.262610236549,29.5213203435596)) ;
#92276=CARTESIAN_POINT('',(70.5000000000002,229.424916996525,29.5213203435596)) ;
#92277=CARTESIAN_POINT('',(70.8999999999999,220.262610236549,29.5213203435596)) ;
#92278=CARTESIAN_POINT('',(63.6796384056928,220.262610236549,29.5213203435596)) ;
#92279=CARTESIAN_POINT('',(70.8999999999999,220.305309236676,29.5213203435596)) ;
#92280=CARTESIAN_POINT('',(70.9000000000003,230.510960283846,29.5213203435596)) ;
#92281=CARTESIAN_POINT('',(72.156281453133,223.25882660182,29.5213203435596)) ;
#92282=CARTESIAN_POINT('Origin',(74.9999999999998,220.305309236676,29.5213203435596)) ;
#92283=CARTESIAN_POINT('',(72.2802893291429,223.890441572703,29.5213203435596)) ;
#92284=CARTESIAN_POINT('Origin',(75.1450953968556,223.000000000001,29.5213203435596)) ;
#92285=CARTESIAN_POINT('',(71.4146847058821,223.024778714675,29.5213203435596)) ;
#92286=CARTESIAN_POINT('Origin',(74.9999999999998,220.305309236676,29.5213203435596)) ;
#92287=CARTESIAN_POINT('',(71.4,223.1,29.5213203435596)) ;
#92288=CARTESIAN_POINT('Origin',(71.6,223.1,29.5213203435596)) ;
#92289=CARTESIAN_POINT('',(71.4,225.9,29.5213203435596)) ;
#92290=CARTESIAN_POINT('',(71.4,225.9,29.5213203435596)) ;
#92291=CARTESIAN_POINT('',(71.6,226.1,29.5213203435596)) ;
#92292=CARTESIAN_POINT('Origin',(71.6,225.9,29.5213203435596)) ;
#92293=CARTESIAN_POINT('',(71.7,226.1,29.5213203435596)) ;
#92294=CARTESIAN_POINT('',(71.7,226.1,29.5213203435596)) ;
#92295=CARTESIAN_POINT('',(71.7,231.9,29.5213203435596)) ;
#92296=CARTESIAN_POINT('',(71.7,231.9,29.5213203435596)) ;
#92297=CARTESIAN_POINT('',(71.9,232.1,29.5213203435596)) ;
#92298=CARTESIAN_POINT('Origin',(71.9,231.9,29.5213203435596)) ;
#92299=CARTESIAN_POINT('',(74.1,232.1,29.5213203435596)) ;
#92300=CARTESIAN_POINT('',(74.1,232.1,29.5213203435596)) ;
#92301=CARTESIAN_POINT('',(74.3,231.9,29.5213203435596)) ;
#92302=CARTESIAN_POINT('Origin',(74.1,231.9,29.5213203435596)) ;
#92303=CARTESIAN_POINT('',(74.3,226.1,29.5213203435596)) ;
#92304=CARTESIAN_POINT('',(74.3,226.1,29.5213203435596)) ;
#92305=CARTESIAN_POINT('',(74.4,226.1,29.5213203435596)) ;
#92306=CARTESIAN_POINT('',(74.4,226.1,29.5213203435596)) ;
#92307=CARTESIAN_POINT('',(74.6000000000001,225.9,29.5213203435596)) ;
#92308=CARTESIAN_POINT('Origin',(74.4,225.9,29.5213203435596)) ;
#92309=CARTESIAN_POINT('',(74.6,224.787496202879,29.5213203435596)) ;
#92310=CARTESIAN_POINT('',(74.6,223.1,29.5213203435596)) ;
#92311=CARTESIAN_POINT('',(75.,224.805309236676,29.5213203435596)) ;
#92312=CARTESIAN_POINT('Origin',(74.9999999999998,220.305309236676,29.5213203435596)) ;
#92313=CARTESIAN_POINT('',(80.,224.805309236676,29.5213203435596)) ;
#92314=CARTESIAN_POINT('',(65.1070907072647,224.805309236677,29.5213203435596)) ;
#92315=CARTESIAN_POINT('',(80.,225.5,29.5213203435596)) ;
#92316=CARTESIAN_POINT('',(80.,232.760960283846,29.5213203435596)) ;
#92317=CARTESIAN_POINT('',(76.0414213562372,225.5,29.5213203435596)) ;
#92318=CARTESIAN_POINT('',(76.0414213562372,225.5,29.5213203435596)) ;
#92319=CARTESIAN_POINT('',(75.9707106781185,225.529289321881,29.5213203435596)) ;
#92320=CARTESIAN_POINT('Origin',(76.0414213562372,225.6,29.5213203435596)) ;
#92321=CARTESIAN_POINT('',(75.2292893218813,226.270710678119,29.5213203435596)) ;
#92322=CARTESIAN_POINT('',(75.2292893218813,226.270710678119,29.5213203435596)) ;
#92323=CARTESIAN_POINT('',(75.1999999999999,226.341421356237,29.5213203435596)) ;
#92324=CARTESIAN_POINT('Origin',(75.2999999999999,226.341421356237,29.5213203435596)) ;
#92325=CARTESIAN_POINT('',(75.2,229.658578643763,29.5213203435596)) ;
#92326=CARTESIAN_POINT('',(75.2,229.658578643763,29.5213203435596)) ;
#92327=CARTESIAN_POINT('',(75.2292893218813,229.729289321881,29.5213203435596)) ;
#92328=CARTESIAN_POINT('Origin',(75.3,229.658578643763,29.5213203435596)) ;
#92329=CARTESIAN_POINT('',(75.9707106781186,230.470710678119,29.5213203435596)) ;
#92330=CARTESIAN_POINT('',(75.9707106781186,230.470710678119,29.5213203435596)) ;
#92331=CARTESIAN_POINT('',(76.0414213562372,230.5,29.5213203435596)) ;
#92332=CARTESIAN_POINT('Origin',(76.0414213562372,230.4,29.5213203435596)) ;
#92333=CARTESIAN_POINT('',(80.,230.5,29.5213203435596)) ;
#92334=CARTESIAN_POINT('',(80.1,230.5,29.5213203435596)) ;
#92335=CARTESIAN_POINT('',(80.,235.608305665508,29.5213203435596)) ;
#92336=CARTESIAN_POINT('',(82.1145102626716,238.704035802635,29.5213203435596)) ;
#92337=CARTESIAN_POINT('Origin',(82.2,237.60736287746,29.5213203435596)) ;
#92338=CARTESIAN_POINT('',(82.183342912681,238.739454580319,29.5213203435596)) ;
#92339=CARTESIAN_POINT('Origin',(82.106738468369,238.803733341288,29.5213203435596)) ;
#92340=CARTESIAN_POINT('',(83.9347806063072,240.826736743903,29.5213203435596)) ;
#92341=CARTESIAN_POINT('',(77.9743376460485,233.723357432561,29.5213203435596)) ;
#92342=CARTESIAN_POINT('',(84.0283628290596,241.083851787777,29.5213203435596)) ;
#92343=CARTESIAN_POINT('Origin',(83.6283628290597,241.083851787777,29.5213203435596)) ;
#92344=CARTESIAN_POINT('',(84.0283628290597,244.265469647218,29.5213203435596)) ;
#92345=CARTESIAN_POINT('',(84.0283628290597,247.594124250979,29.5213203435596)) ;
#92346=CARTESIAN_POINT('',(82.27326394817,246.357115043876,29.5213203435596)) ;
#92347=CARTESIAN_POINT('',(78.9611335727037,250.304358317977,29.5213203435596)) ;
#92348=CARTESIAN_POINT('',(81.9668461709225,246.500000000001,29.5213203435596)) ;
#92349=CARTESIAN_POINT('Origin',(81.9668461709225,246.100000000001,29.5213203435596)) ;
#92350=CARTESIAN_POINT('',(80.6401337790902,246.500000000001,29.5213203435596)) ;
#92351=CARTESIAN_POINT('',(68.5905137927262,246.500000000001,29.5213203435596)) ;
#92352=CARTESIAN_POINT('',(80.5401534070282,246.601981212341,29.5213203435596)) ;
#92353=CARTESIAN_POINT('Origin',(80.6401337790902,246.600000000001,29.5213203435596)) ;
#92354=CARTESIAN_POINT('',(81.1,247.098386676966,29.5213203435596)) ;
#92355=CARTESIAN_POINT('Origin',(80.6,247.098386676966,29.5213203435596)) ;
#92356=CARTESIAN_POINT('',(81.1,247.600000000001,29.5213203435596)) ;
#92357=CARTESIAN_POINT('',(81.1,243.907499003991,29.5213203435596)) ;
#92358=CARTESIAN_POINT('',(68.157090707265,247.600000000001,29.5213203435596)) ;
#92359=CARTESIAN_POINT('',(43.1,251.9,29.5213203435596)) ;
#92360=CARTESIAN_POINT('',(43.3,252.1,29.5213203435596)) ;
#92361=CARTESIAN_POINT('Origin',(43.1,252.1,29.5213203435596)) ;
#92362=CARTESIAN_POINT('',(37.3,251.9,29.5213203435596)) ;
#92363=CARTESIAN_POINT('',(37.3,251.9,29.5213203435596)) ;
#92364=CARTESIAN_POINT('',(37.1,252.1,29.5213203435596)) ;
#92365=CARTESIAN_POINT('Origin',(37.3,252.1,29.5213203435596)) ;
#92366=CARTESIAN_POINT('',(37.1,259.9,29.5213203435596)) ;
#92367=CARTESIAN_POINT('',(37.1,259.9,29.5213203435596)) ;
#92368=CARTESIAN_POINT('',(37.3,260.1,29.5213203435596)) ;
#92369=CARTESIAN_POINT('Origin',(37.3,259.9,29.5213203435596)) ;
#92370=CARTESIAN_POINT('',(43.1,260.1,29.5213203435596)) ;
#92371=CARTESIAN_POINT('',(43.1,260.1,29.5213203435596)) ;
#92372=CARTESIAN_POINT('',(43.3,259.9,29.5213203435596)) ;
#92373=CARTESIAN_POINT('Origin',(43.1,259.9,29.5213203435596)) ;
#92374=CARTESIAN_POINT('',(43.3,252.1,29.5213203435596)) ;
#92375=CARTESIAN_POINT('',(28.1,254.8,29.5213203435596)) ;
#92376=CARTESIAN_POINT('Origin',(30.7,254.8,29.5213203435596)) ;
#92377=CARTESIAN_POINT('',(56.8,257.1,29.5213203435596)) ;
#92378=CARTESIAN_POINT('',(56.6,256.9,29.5213203435596)) ;
#92379=CARTESIAN_POINT('Origin',(56.8,256.9,29.5213203435596)) ;
#92380=CARTESIAN_POINT('',(59.,257.1,29.5213203435596)) ;
#92381=CARTESIAN_POINT('',(59.,257.1,29.5213203435596)) ;
#92382=CARTESIAN_POINT('',(59.2,256.9,29.5213203435596)) ;
#92383=CARTESIAN_POINT('Origin',(59.,256.9,29.5213203435596)) ;
#92384=CARTESIAN_POINT('',(59.2,251.1,29.5213203435596)) ;
#92385=CARTESIAN_POINT('',(59.2,251.1,29.5213203435596)) ;
#92386=CARTESIAN_POINT('',(59.3,251.1,29.5213203435596)) ;
#92387=CARTESIAN_POINT('',(59.3,251.1,29.5213203435596)) ;
#92388=CARTESIAN_POINT('',(59.5,250.9,29.5213203435596)) ;
#92389=CARTESIAN_POINT('Origin',(59.3,250.9,29.5213203435596)) ;
#92390=CARTESIAN_POINT('',(59.5,248.1,29.5213203435596)) ;
#92391=CARTESIAN_POINT('',(59.5,248.1,29.5213203435596)) ;
#92392=CARTESIAN_POINT('',(59.3,247.9,29.5213203435596)) ;
#92393=CARTESIAN_POINT('Origin',(59.3,248.1,29.5213203435596)) ;
#92394=CARTESIAN_POINT('',(56.5,247.9,29.5213203435596)) ;
#92395=CARTESIAN_POINT('',(56.5,247.9,29.5213203435596)) ;
#92396=CARTESIAN_POINT('',(56.3,248.1,29.5213203435596)) ;
#92397=CARTESIAN_POINT('Origin',(56.5,248.1,29.5213203435596)) ;
#92398=CARTESIAN_POINT('',(56.3,250.9,29.5213203435596)) ;
#92399=CARTESIAN_POINT('',(56.3,250.9,29.5213203435596)) ;
#92400=CARTESIAN_POINT('',(56.5,251.1,29.5213203435596)) ;
#92401=CARTESIAN_POINT('Origin',(56.5,250.9,29.5213203435596)) ;
#92402=CARTESIAN_POINT('',(56.6,251.1,29.5213203435596)) ;
#92403=CARTESIAN_POINT('',(56.6,251.1,29.5213203435596)) ;
#92404=CARTESIAN_POINT('',(56.6,256.9,29.5213203435596)) ;
#92405=CARTESIAN_POINT('',(59.,261.2,29.5213203435596)) ;
#92406=CARTESIAN_POINT('Origin',(61.5,261.2,29.5213203435596)) ;
#92407=CARTESIAN_POINT('',(57.9573593128808,242.926794919243,29.5213203435596)) ;
#92408=CARTESIAN_POINT('',(57.9573593128808,238.073205080757,29.5213203435596)) ;
#92409=CARTESIAN_POINT('',(57.9573593128808,239.1,29.5213203435596)) ;
#92410=CARTESIAN_POINT('',(58.0573593128808,243.1,29.5213203435596)) ;
#92411=CARTESIAN_POINT('Ctrl Pts',(58.0573593128808,243.1,29.5213203435596)) ;
#92412=CARTESIAN_POINT('Ctrl Pts',(58.0296494906727,243.072290177792,29.5213203435596)) ;
#92413=CARTESIAN_POINT('Ctrl Pts',(57.9969680412619,243.03847767278,29.5213203435596)) ;
#92414=CARTESIAN_POINT('Ctrl Pts',(57.9663165128705,242.981526952685,29.5213203435596)) ;
#92415=CARTESIAN_POINT('Ctrl Pts',(57.9573593128807,242.952282661431,29.5213203435596)) ;
#92416=CARTESIAN_POINT('Ctrl Pts',(57.9573593128807,242.926794919243,29.5213203435596)) ;
#92417=CARTESIAN_POINT('',(62.1159379566435,243.1,29.5213203435596)) ;
#92418=CARTESIAN_POINT('',(62.1159379566435,243.1,29.5213203435596)) ;
#92419=CARTESIAN_POINT('',(62.2573593128808,243.041421356237,29.5213203435596)) ;
#92420=CARTESIAN_POINT('Origin',(62.1159379566435,242.9,29.5213203435596)) ;
#92421=CARTESIAN_POINT('',(62.9987806691181,242.3,29.5213203435596)) ;
#92422=CARTESIAN_POINT('',(62.9987806691181,242.3,29.5213203435596)) ;
#92423=CARTESIAN_POINT('',(63.0573593128808,242.158578643763,29.5213203435596)) ;
#92424=CARTESIAN_POINT('Origin',(62.8573593128808,242.158578643763,29.5213203435596)) ;
#92425=CARTESIAN_POINT('',(63.0573593128808,238.841421356237,29.5213203435596)) ;
#92426=CARTESIAN_POINT('',(63.0573593128808,238.841421356237,29.5213203435596)) ;
#92427=CARTESIAN_POINT('',(62.9987806691181,238.7,29.5213203435596)) ;
#92428=CARTESIAN_POINT('Origin',(62.8573593128808,238.841421356237,29.5213203435596)) ;
#92429=CARTESIAN_POINT('',(62.2573593128808,237.958578643763,29.5213203435596)) ;
#92430=CARTESIAN_POINT('',(62.2573593128808,237.958578643763,29.5213203435596)) ;
#92431=CARTESIAN_POINT('',(62.1159379566435,237.9,29.5213203435596)) ;
#92432=CARTESIAN_POINT('Origin',(62.1159379566435,238.1,29.5213203435596)) ;
#92433=CARTESIAN_POINT('',(58.0573593128808,237.9,29.5213203435596)) ;
#92434=CARTESIAN_POINT('',(58.0573593128808,237.9,29.5213203435596)) ;
#92435=CARTESIAN_POINT('Ctrl Pts',(57.9573593128807,238.073205080757,29.5213203435596)) ;
#92436=CARTESIAN_POINT('Ctrl Pts',(57.9573593128807,238.047717338569,29.5213203435596)) ;
#92437=CARTESIAN_POINT('Ctrl Pts',(57.9663165128705,238.018473047315,29.5213203435596)) ;
#92438=CARTESIAN_POINT('Ctrl Pts',(57.9969680412619,237.96152232722,29.5213203435596)) ;
#92439=CARTESIAN_POINT('Ctrl Pts',(58.0296494906727,237.927709822208,29.5213203435596)) ;
#92440=CARTESIAN_POINT('Ctrl Pts',(58.0573593128808,237.9,29.5213203435596)) ;
#92441=CARTESIAN_POINT('',(60.0305643936376,236.,29.5213203435596)) ;
#92442=CARTESIAN_POINT('',(59.8573593128808,235.9,29.5213203435596)) ;
#92443=CARTESIAN_POINT('Ctrl Pts',(60.0305643936376,236.,29.5213203435596)) ;
#92444=CARTESIAN_POINT('Ctrl Pts',(60.0050766514501,236.,29.5213203435596)) ;
#92445=CARTESIAN_POINT('Ctrl Pts',(59.9758323601959,235.99104280001,29.5213203435596)) ;
#92446=CARTESIAN_POINT('Ctrl Pts',(59.9188816401012,235.960391271619,29.5213203435596)) ;
#92447=CARTESIAN_POINT('Ctrl Pts',(59.8850691350889,235.927709822208,29.5213203435596)) ;
#92448=CARTESIAN_POINT('Ctrl Pts',(59.8573593128808,235.9,29.5213203435596)) ;
#92449=CARTESIAN_POINT('',(62.2841542321239,236.,29.5213203435596)) ;
#92450=CARTESIAN_POINT('',(62.4573593128808,230.1,29.5213203435596)) ;
#92451=CARTESIAN_POINT('',(62.4573593128808,230.1,29.5213203435596)) ;
#92452=CARTESIAN_POINT('',(62.5573593128808,230.1,29.5213203435596)) ;
#92453=CARTESIAN_POINT('',(62.5573593128808,230.1,29.5213203435596)) ;
#92454=CARTESIAN_POINT('',(62.7573593128808,229.9,29.5213203435596)) ;
#92455=CARTESIAN_POINT('Origin',(62.5573593128808,229.9,29.5213203435596)) ;
#92456=CARTESIAN_POINT('',(62.7573593128808,227.1,29.5213203435596)) ;
#92457=CARTESIAN_POINT('',(62.7573593128808,227.1,29.5213203435596)) ;
#92458=CARTESIAN_POINT('',(62.5573593128808,226.9,29.5213203435596)) ;
#92459=CARTESIAN_POINT('Origin',(62.5573593128808,227.1,29.5213203435596)) ;
#92460=CARTESIAN_POINT('',(59.7573593128808,226.9,29.5213203435596)) ;
#92461=CARTESIAN_POINT('',(59.7573593128808,226.9,29.5213203435596)) ;
#92462=CARTESIAN_POINT('',(59.5573593128807,227.1,29.5213203435596)) ;
#92463=CARTESIAN_POINT('Origin',(59.7573593128808,227.1,29.5213203435596)) ;
#92464=CARTESIAN_POINT('',(59.5573593128808,229.9,29.5213203435596)) ;
#92465=CARTESIAN_POINT('',(59.5573593128808,229.9,29.5213203435596)) ;
#92466=CARTESIAN_POINT('',(59.7573593128808,230.1,29.5213203435596)) ;
#92467=CARTESIAN_POINT('Origin',(59.7573593128808,229.9,29.5213203435596)) ;
#92468=CARTESIAN_POINT('',(59.8573593128808,230.1,29.5213203435596)) ;
#92469=CARTESIAN_POINT('',(59.8573593128808,230.1,29.5213203435596)) ;
#92470=CARTESIAN_POINT('',(59.8573593128808,235.9,29.5213203435596)) ;
#92471=CARTESIAN_POINT('',(64.8,257.1,29.5213203435596)) ;
#92472=CARTESIAN_POINT('',(64.6,256.9,29.5213203435596)) ;
#92473=CARTESIAN_POINT('Origin',(64.8,256.9,29.5213203435596)) ;
#92474=CARTESIAN_POINT('',(67.,257.1,29.5213203435596)) ;
#92475=CARTESIAN_POINT('',(67.,257.1,29.5213203435596)) ;
#92476=CARTESIAN_POINT('',(67.2,256.9,29.5213203435596)) ;
#92477=CARTESIAN_POINT('Origin',(67.,256.9,29.5213203435596)) ;
#92478=CARTESIAN_POINT('',(67.2,251.1,29.5213203435596)) ;
#92479=CARTESIAN_POINT('',(67.2,251.1,29.5213203435596)) ;
#92480=CARTESIAN_POINT('',(67.3,251.1,29.5213203435596)) ;
#92481=CARTESIAN_POINT('',(67.3,251.1,29.5213203435596)) ;
#92482=CARTESIAN_POINT('',(67.5,250.9,29.5213203435596)) ;
#92483=CARTESIAN_POINT('Origin',(67.3,250.9,29.5213203435596)) ;
#92484=CARTESIAN_POINT('',(67.5,248.1,29.5213203435596)) ;
#92485=CARTESIAN_POINT('',(67.5,248.1,29.5213203435596)) ;
#92486=CARTESIAN_POINT('',(67.3,247.9,29.5213203435596)) ;
#92487=CARTESIAN_POINT('Origin',(67.3,248.1,29.5213203435596)) ;
#92488=CARTESIAN_POINT('',(64.5,247.9,29.5213203435596)) ;
#92489=CARTESIAN_POINT('',(64.5,247.9,29.5213203435596)) ;
#92490=CARTESIAN_POINT('',(64.3,248.1,29.5213203435596)) ;
#92491=CARTESIAN_POINT('Origin',(64.5,248.1,29.5213203435596)) ;
#92492=CARTESIAN_POINT('',(64.3,250.9,29.5213203435596)) ;
#92493=CARTESIAN_POINT('',(64.3,250.9,29.5213203435596)) ;
#92494=CARTESIAN_POINT('',(64.5,251.1,29.5213203435596)) ;
#92495=CARTESIAN_POINT('Origin',(64.5,250.9,29.5213203435596)) ;
#92496=CARTESIAN_POINT('',(64.6,251.1,29.5213203435596)) ;
#92497=CARTESIAN_POINT('',(64.6,251.1,29.5213203435596)) ;
#92498=CARTESIAN_POINT('',(64.6,256.9,29.5213203435596)) ;
#92499=CARTESIAN_POINT('Origin',(82.9283628290598,253.974580896093,30.7213203435596)) ;
#92500=CARTESIAN_POINT('Ctrl Pts',(72.2848151277479,223.47832706609,29.6213203435596)) ;
#92501=CARTESIAN_POINT('Ctrl Pts',(72.2848151277479,223.47832706609,29.6117820586428)) ;
#92502=CARTESIAN_POINT('Ctrl Pts',(72.2808542722274,223.472044514469,29.5927809266332)) ;
#92503=CARTESIAN_POINT('Ctrl Pts',(72.2660826403646,223.448322669426,29.568915436412)) ;
#92504=CARTESIAN_POINT('Ctrl Pts',(72.2400335798865,223.405693978819,29.5444496865641)) ;
#92505=CARTESIAN_POINT('Ctrl Pts',(72.2020093099499,223.341346933962,29.5259708354515)) ;
#92506=CARTESIAN_POINT('Ctrl Pts',(72.1712632154036,223.286371940893,29.5213203435596)) ;
#92507=CARTESIAN_POINT('Ctrl Pts',(72.156281453133,223.25882660182,29.5213203435596)) ;
#92508=CARTESIAN_POINT('Ctrl Pts',(72.2810000867808,223.455514042998,29.6213203435596)) ;
#92509=CARTESIAN_POINT('Ctrl Pts',(72.2810000867808,223.455514042998,29.6143550630749)) ;
#92510=CARTESIAN_POINT('Ctrl Pts',(72.2789291556126,223.45022120786,29.6002951365768)) ;
#92511=CARTESIAN_POINT('Ctrl Pts',(72.2690858869446,223.429107117665,29.5790237734122)) ;
#92512=CARTESIAN_POINT('Ctrl Pts',(72.2482378360867,223.389557669006,29.5536298248665)) ;
#92513=CARTESIAN_POINT('Ctrl Pts',(72.213241144952,223.328135436704,29.5307455300177)) ;
#92514=CARTESIAN_POINT('Ctrl Pts',(72.1821614688016,223.274848566189,29.5227418738956)) ;
#92515=CARTESIAN_POINT('Ctrl Pts',(72.1666575336158,223.248049890488,29.5213203435596)) ;
#92516=CARTESIAN_POINT('Ctrl Pts',(72.2888679854647,223.413391262911,29.6213203435597)) ;
#92517=CARTESIAN_POINT('Ctrl Pts',(72.2888679854647,223.413391262911,29.6173756251696)) ;
#92518=CARTESIAN_POINT('Ctrl Pts',(72.2892555769235,223.409994519109,29.609053079611)) ;
#92519=CARTESIAN_POINT('Ctrl Pts',(72.2851493810959,223.39392773353,29.5895727666044)) ;
#92520=CARTESIAN_POINT('Ctrl Pts',(72.2693821576178,223.360449550633,29.5609780226199)) ;
#92521=CARTESIAN_POINT('Ctrl Pts',(72.2355055751497,223.30476013175,29.5309152737761)) ;
#92522=CARTESIAN_POINT('Ctrl Pts',(72.201962597952,223.25464893562,29.5184715285348)) ;
#92523=CARTESIAN_POINT('Ctrl Pts',(72.184795277803,223.229211829851,29.5153203301976)) ;
#92524=CARTESIAN_POINT('Ctrl Pts',(72.3355462445646,223.366840464368,29.6213203435596)) ;
#92525=CARTESIAN_POINT('Ctrl Pts',(72.3355462445646,223.366840464368,29.6164645616614)) ;
#92526=CARTESIAN_POINT('Ctrl Pts',(72.3360510372649,223.365000743143,29.6061878672546)) ;
#92527=CARTESIAN_POINT('Ctrl Pts',(72.3309634543418,223.353337548304,29.5818580530947)) ;
#92528=CARTESIAN_POINT('Ctrl Pts',(72.3114661600803,223.325571261253,29.5463312063646)) ;
#92529=CARTESIAN_POINT('Ctrl Pts',(72.2699544689077,223.275650758824,29.5095570918057)) ;
#92530=CARTESIAN_POINT('Ctrl Pts',(72.2292143217159,223.228761139121,29.4947957329644)) ;
#92531=CARTESIAN_POINT('Ctrl Pts',(72.2084154512032,223.204679657923,29.4911830637617)) ;
#92532=CARTESIAN_POINT('Ctrl Pts',(72.3958472601896,223.356104604207,29.6213203435596)) ;
#92533=CARTESIAN_POINT('Ctrl Pts',(72.3958472601896,223.356104604207,29.6106947817332)) ;
#92534=CARTESIAN_POINT('Ctrl Pts',(72.3933967836352,223.353510123056,29.5891261889309)) ;
#92535=CARTESIAN_POINT('Ctrl Pts',(72.3797193135333,223.340262757401,29.554538401925)) ;
#92536=CARTESIAN_POINT('Ctrl Pts',(72.3487860197444,223.311258504548,29.5122402365605)) ;
#92537=CARTESIAN_POINT('Ctrl Pts',(72.2951190991269,223.260961486717,29.4740143351241)) ;
#92538=CARTESIAN_POINT('Ctrl Pts',(72.2468169388032,223.214067870685,29.4609869305912)) ;
#92539=CARTESIAN_POINT('Ctrl Pts',(72.2225691253102,223.189979496298,29.4587319390131)) ;
#92540=CARTESIAN_POINT('Ctrl Pts',(72.433908428714,223.373773832992,29.6213203435596)) ;
#92541=CARTESIAN_POINT('Ctrl Pts',(72.433908428714,223.373773832992,29.6047572686629)) ;
#92542=CARTESIAN_POINT('Ctrl Pts',(72.4285124008623,223.369273781245,29.5716464499249)) ;
#92543=CARTESIAN_POINT('Ctrl Pts',(72.4069263743005,223.351045791115,29.5278439559481)) ;
#92544=CARTESIAN_POINT('Ctrl Pts',(72.3665979735026,223.31640834513,29.4809183052355)) ;
#92545=CARTESIAN_POINT('Ctrl Pts',(72.304473339827,223.261299627013,29.4436111538445)) ;
#92546=CARTESIAN_POINT('Ctrl Pts',(72.2517858004854,223.211967617058,29.4332114711027)) ;
#92547=CARTESIAN_POINT('Ctrl Pts',(72.225640442081,223.186789592914,29.4325403173224)) ;
#92548=CARTESIAN_POINT('Ctrl Pts',(72.4472638847366,223.384844644141,29.6213203435596)) ;
#92549=CARTESIAN_POINT('Ctrl Pts',(72.4472638847366,223.384844644141,29.6022437737259)) ;
#92550=CARTESIAN_POINT('Ctrl Pts',(72.4406894966491,223.379412576914,29.5642415097069)) ;
#92551=CARTESIAN_POINT('Ctrl Pts',(72.4160080913986,223.358747929883,29.5165105292643)) ;
#92552=CARTESIAN_POINT('Ctrl Pts',(72.3720483401316,223.321197129049,29.4675790295685)) ;
#92553=CARTESIAN_POINT('Ctrl Pts',(72.306745659313,223.263425781024,29.4306213273434)) ;
#92554=CARTESIAN_POINT('Ctrl Pts',(72.2524544719542,223.212606794792,29.4213203435596)) ;
#92555=CARTESIAN_POINT('Ctrl Pts',(72.225640442081,223.186789592914,29.4213203435596)) ;
#92556=CARTESIAN_POINT('',(72.2256404420809,223.186789592914,29.4213203435596)) ;
#92557=CARTESIAN_POINT('',(72.4472638847366,223.384844644141,29.6213203435596)) ;
#92558=CARTESIAN_POINT('Ctrl Pts',(72.225640442081,223.186789592914,29.4213203435596)) ;
#92559=CARTESIAN_POINT('Ctrl Pts',(72.2524544719542,223.212606794792,29.4213203435596)) ;
#92560=CARTESIAN_POINT('Ctrl Pts',(72.306745659313,223.263425781024,29.4306213273434)) ;
#92561=CARTESIAN_POINT('Ctrl Pts',(72.3720483401316,223.321197129049,29.4675790295685)) ;
#92562=CARTESIAN_POINT('Ctrl Pts',(72.4160080913986,223.358747929883,29.5165105292643)) ;
#92563=CARTESIAN_POINT('Ctrl Pts',(72.4406894966491,223.379412576914,29.5642415097069)) ;
#92564=CARTESIAN_POINT('Ctrl Pts',(72.4472638847366,223.384844644141,29.6022437737259)) ;
#92565=CARTESIAN_POINT('Ctrl Pts',(72.4472638847366,223.384844644141,29.6213203435596)) ;
#92566=CARTESIAN_POINT('',(72.2848151277479,223.47832706609,29.6213203435596)) ;
#92567=CARTESIAN_POINT('Origin',(72.383445481855,223.461833029328,29.6213203435596)) ;
#92568=CARTESIAN_POINT('Ctrl Pts',(72.2848151277479,223.47832706609,29.6213203435596)) ;
#92569=CARTESIAN_POINT('Ctrl Pts',(72.2848151277479,223.47832706609,29.6117820586428)) ;
#92570=CARTESIAN_POINT('Ctrl Pts',(72.2808542722274,223.472044514469,29.5927809266332)) ;
#92571=CARTESIAN_POINT('Ctrl Pts',(72.2660826403646,223.448322669426,29.568915436412)) ;
#92572=CARTESIAN_POINT('Ctrl Pts',(72.2400335798865,223.405693978819,29.5444496865641)) ;
#92573=CARTESIAN_POINT('Ctrl Pts',(72.2020093099499,223.341346933962,29.5259708354515)) ;
#92574=CARTESIAN_POINT('Ctrl Pts',(72.1712632154036,223.286371940893,29.5213203435596)) ;
#92575=CARTESIAN_POINT('Ctrl Pts',(72.156281453133,223.25882660182,29.5213203435596)) ;
#92576=CARTESIAN_POINT('Origin',(72.156281453133,223.25882660182,29.4213203435596)) ;
#92577=CARTESIAN_POINT('Origin',(72.383445481855,223.461833029328,29.5213203435596)) ;
#92578=CARTESIAN_POINT('',(72.2848151277479,223.47832706609,29.5213203435596)) ;
#92579=CARTESIAN_POINT('',(72.4472638847366,223.384844644141,29.5213203435596)) ;
#92580=CARTESIAN_POINT('Origin',(75.1450953968556,223.000000000001,29.6213203435596)) ;
#92581=CARTESIAN_POINT('',(72.4201780792821,223.992383802966,29.6213203435596)) ;
#92582=CARTESIAN_POINT('Ctrl Pts',(72.4201780792825,223.992383802966,29.6213203435596)) ;
#92583=CARTESIAN_POINT('Ctrl Pts',(72.4201780792825,223.992383802966,29.6145564866725)) ;
#92584=CARTESIAN_POINT('Ctrl Pts',(72.4191973948714,223.991698158942,29.6078620210061)) ;
#92585=CARTESIAN_POINT('Ctrl Pts',(72.417299229791,223.990367815798,29.601339025129)) ;
#92586=CARTESIAN_POINT('Ctrl Pts',(72.4148969906463,223.98868418859,29.5930837915886)) ;
#92587=CARTESIAN_POINT('Ctrl Pts',(72.4111225700089,223.986035531718,29.5854386000695)) ;
#92588=CARTESIAN_POINT('Ctrl Pts',(72.4064704600445,223.982754617015,29.5785304102571)) ;
#92589=CARTESIAN_POINT('Ctrl Pts',(72.3998148180006,223.97806070522,29.5686470586349)) ;
#92590=CARTESIAN_POINT('Ctrl Pts',(72.3913538115502,223.972063817752,29.5602421869295)) ;
#92591=CARTESIAN_POINT('Ctrl Pts',(72.3822927902472,223.965583675022,29.5533237804999)) ;
#92592=CARTESIAN_POINT('Ctrl Pts',(72.3685935368461,223.955786422111,29.5428639217664)) ;
#92593=CARTESIAN_POINT('Ctrl Pts',(72.3518149123848,223.943668481139,29.5344794129739)) ;
#92594=CARTESIAN_POINT('Ctrl Pts',(72.3330588183395,223.929867793737,29.528907978084)) ;
#92595=CARTESIAN_POINT('Ctrl Pts',(72.3174379333076,223.918373985338,29.5242678465264)) ;
#92596=CARTESIAN_POINT('Ctrl Pts',(72.301017128619,223.906130659284,29.5217464661521)) ;
#92597=CARTESIAN_POINT('Ctrl Pts',(72.2846076883626,223.893713421533,29.5213699088416)) ;
#92598=CARTESIAN_POINT('Ctrl Pts',(72.283167988846,223.892623982106,29.5213368711896)) ;
#92599=CARTESIAN_POINT('Ctrl Pts',(72.2817283570166,223.891533231001,29.5213203435596)) ;
#92600=CARTESIAN_POINT('Ctrl Pts',(72.2802893291429,223.890441572703,29.5213203435596)) ;
#92601=CARTESIAN_POINT('Origin',(75.1450953968556,223.000000000001,29.6213203435596)) ;
#92602=CARTESIAN_POINT('Origin',(74.9999999999998,220.305309236676,29.4213203435596)) ;
#92603=CARTESIAN_POINT('',(70.9999999999999,220.305309236676,29.4213203435596)) ;
#92604=CARTESIAN_POINT('Origin',(70.8999999999999,220.305309236676,29.4213203435596)) ;
#92605=CARTESIAN_POINT('Origin',(74.9999999999998,220.305309236676,29.4213203435596)) ;
#92606=CARTESIAN_POINT('Origin',(70.9000000000003,230.510960283846,29.4213203435596)) ;
#92607=CARTESIAN_POINT('',(70.9999999999999,220.262610236549,29.4213203435596)) ;
#92608=CARTESIAN_POINT('Origin',(70.8999999999999,220.262610236549,29.4213203435596)) ;
#92609=CARTESIAN_POINT('',(71.0000000000003,230.510960283846,29.4213203435596)) ;
#92610=CARTESIAN_POINT('Origin',(75.1450953968556,223.000000000001,30.7213203435596)) ;
#92611=CARTESIAN_POINT('',(72.4201780792821,223.992383802966,30.7213203435596)) ;
#92612=CARTESIAN_POINT('Origin',(74.9999999999998,220.305309236676,29.5213203435596)) ;
#92613=CARTESIAN_POINT('',(70.9999999999999,220.305309236676,16.1213203435596)) ;
#92614=CARTESIAN_POINT('',(70.9999999999999,220.305309236676,29.5213203435596)) ;
#92615=CARTESIAN_POINT('',(75.,224.305309236676,16.1213203435596)) ;
#92616=CARTESIAN_POINT('Origin',(74.9999999999998,220.305309236676,16.1213203435596)) ;
#92617=CARTESIAN_POINT('',(75.,224.305309236676,29.5213203435596)) ;
#92618=CARTESIAN_POINT('Origin',(70.9999999999999,220.305309236676,29.5213203435596)) ;
#92619=CARTESIAN_POINT('',(70.9999999999999,220.262610236549,30.7213203435596)) ;
#92620=CARTESIAN_POINT('',(70.9999999999999,220.262610236549,30.1213203435596)) ;
#92621=CARTESIAN_POINT('',(70.9999999999999,220.305309236676,30.7213203435596)) ;
#92622=CARTESIAN_POINT('',(70.9999999999998,217.165524426368,16.1213203435596)) ;
#92623=CARTESIAN_POINT('',(70.9999999999998,217.165524426368,25.0213203435596)) ;
#92624=CARTESIAN_POINT('',(71.0000000000001,225.16903572493,16.1213203435596)) ;
#92625=CARTESIAN_POINT('Origin',(80.1,230.5,29.5213203435596)) ;
#92626=CARTESIAN_POINT('',(80.,230.5,30.7213203435596)) ;
#92627=CARTESIAN_POINT('',(76.0414213562372,230.5,25.7213203435596)) ;
#92628=CARTESIAN_POINT('',(76.0414213562372,230.5,29.5213203435596)) ;
#92629=CARTESIAN_POINT('',(80.1,230.5,25.7213203435596)) ;
#92630=CARTESIAN_POINT('',(78.9,230.5,25.7213203435596)) ;
#92631=CARTESIAN_POINT('',(80.1,230.5,29.5213203435596)) ;
#92632=CARTESIAN_POINT('Origin',(84.0283628290597,244.57661441259,30.6213203435596)) ;
#92633=CARTESIAN_POINT('',(84.1283628290597,244.57661441259,30.6213203435596)) ;
#92634=CARTESIAN_POINT('',(83.9517583847478,244.512335651621,30.6213203435596)) ;
#92635=CARTESIAN_POINT('Origin',(84.0283628290597,244.57661441259,30.6213203435596)) ;
#92636=CARTESIAN_POINT('',(84.0283628290597,244.57661441259,30.7213203435596)) ;
#92637=CARTESIAN_POINT('Origin',(84.0283628290597,244.57661441259,30.6213203435596)) ;
#92638=CARTESIAN_POINT('Origin',(84.0283628290597,244.57661441259,30.6213203435596)) ;
#92639=CARTESIAN_POINT('Origin',(79.1,257.325466667661,30.6213203435596)) ;
#92640=CARTESIAN_POINT('',(79.1,259.648528137424,30.7213203435596)) ;
#92641=CARTESIAN_POINT('',(79.1,257.325466667661,30.7213203435596)) ;
#92642=CARTESIAN_POINT('',(79.2,259.648528137424,30.6213203435596)) ;
#92643=CARTESIAN_POINT('Origin',(79.1,259.648528137424,30.6213203435596)) ;
#92644=CARTESIAN_POINT('',(79.2,257.325466667661,30.6213203435596)) ;
#92645=CARTESIAN_POINT('Origin',(79.7999999999999,259.648528137424,30.6213203435596)) ;
#92646=CARTESIAN_POINT('',(79.3050252531695,259.153553390593,30.7213203435596)) ;
#92647=CARTESIAN_POINT('',(79.3757359312881,259.224264068712,30.6213203435596)) ;
#92648=CARTESIAN_POINT('Origin',(79.3050252531695,259.153553390593,30.6213203435596)) ;
#92649=CARTESIAN_POINT('Origin',(79.7999999999999,259.648528137424,30.6213203435596)) ;
#92650=CARTESIAN_POINT('Origin',(79.7999999999999,259.648528137424,30.7213203435596)) ;
#92651=CARTESIAN_POINT('Origin',(82.1504860297137,256.30809261405,30.6213203435596)) ;
#92652=CARTESIAN_POINT('',(83.7647589321277,254.693819711636,30.7213203435596)) ;
#92653=CARTESIAN_POINT('',(83.8354696102463,254.764530389755,30.6213203435596)) ;
#92654=CARTESIAN_POINT('Origin',(83.7647589321277,254.693819711636,30.6213203435596)) ;
#92655=CARTESIAN_POINT('',(82.2211967078324,256.378803292168,30.6213203435596)) ;
#92656=CARTESIAN_POINT('',(82.1504860297137,256.30809261405,30.7213203435596)) ;
#92657=CARTESIAN_POINT('Origin',(83.1283628290598,254.057423608568,30.6213203435596)) ;
#92658=CARTESIAN_POINT('',(84.0283628290598,254.057423608568,30.7213203435596)) ;
#92659=CARTESIAN_POINT('',(84.1283628290598,254.057423608568,30.6213203435596)) ;
#92660=CARTESIAN_POINT('Origin',(84.0283628290598,254.057423608568,30.6213203435596)) ;
#92661=CARTESIAN_POINT('Origin',(83.1283628290598,254.057423608568,30.6213203435596)) ;
#92662=CARTESIAN_POINT('Origin',(83.1283628290598,254.057423608568,30.7213203435596)) ;
#92663=CARTESIAN_POINT('Origin',(84.0283628290598,252.661285253132,30.6213203435596)) ;
#92664=CARTESIAN_POINT('',(84.1283628290598,252.661285253132,30.6213203435596)) ;
#92665=CARTESIAN_POINT('',(84.0283628290598,252.661285253132,30.7213203435596)) ;
#92666=CARTESIAN_POINT('Origin',(82.1755472374987,246.700000000001,30.6213203435596)) ;
#92667=CARTESIAN_POINT('',(80.9021391328793,246.700000000001,30.7213203435596)) ;
#92668=CARTESIAN_POINT('',(80.6401337790902,246.600000000001,30.6213203435596)) ;
#92669=CARTESIAN_POINT('Ctrl Pts',(80.9021391328789,246.700000000001,30.7213203435596)) ;
#92670=CARTESIAN_POINT('Ctrl Pts',(80.8546339956107,246.663971784673,30.7213203435597)) ;
#92671=CARTESIAN_POINT('Ctrl Pts',(80.7930243634798,246.633827705385,30.7009621255511)) ;
#92672=CARTESIAN_POINT('Ctrl Pts',(80.7145517409522,246.610975914622,30.6686175810887)) ;
#92673=CARTESIAN_POINT('Ctrl Pts',(80.6838650368446,246.60487069038,30.6554832196524)) ;
#92674=CARTESIAN_POINT('Ctrl Pts',(80.6554491801068,246.601452173645,30.6384990816338)) ;
#92675=CARTESIAN_POINT('Ctrl Pts',(80.6509273236865,246.60097285483,30.6355928657033)) ;
#92676=CARTESIAN_POINT('Ctrl Pts',(80.6453291232314,246.600442142126,30.6308486781643)) ;
#92677=CARTESIAN_POINT('Ctrl Pts',(80.6436891658207,246.600297421838,30.6292287985663)) ;
#92678=CARTESIAN_POINT('Ctrl Pts',(80.6417701542494,246.600134064326,30.6265722342026)) ;
#92679=CARTESIAN_POINT('Ctrl Pts',(80.6412262678027,246.600088990182,30.6256529368887)) ;
#92680=CARTESIAN_POINT('Ctrl Pts',(80.6404087807581,246.600022073172,30.6236520910468)) ;
#92681=CARTESIAN_POINT('Ctrl Pts',(80.640133779087,246.600000000001,30.6225711229527)) ;
#92682=CARTESIAN_POINT('Ctrl Pts',(80.640133779087,246.600000000001,30.6213203435596)) ;
#92683=CARTESIAN_POINT('',(81.9668461709225,246.600000000001,30.6213203435596)) ;
#92684=CARTESIAN_POINT('',(82.1755472374987,246.600000000001,30.6213203435596)) ;
#92685=CARTESIAN_POINT('',(81.9668461709225,246.700000000001,30.7213203435596)) ;
#92686=CARTESIAN_POINT('Origin',(81.9668461709225,246.700000000001,30.6213203435596)) ;
#92687=CARTESIAN_POINT('',(82.1755472374987,246.700000000001,30.7213203435596)) ;
#92688=CARTESIAN_POINT('Origin',(81.9668461709225,246.100000000001,30.6213203435596)) ;
#92689=CARTESIAN_POINT('',(82.349868392482,246.421393804845,30.6213203435596)) ;
#92690=CARTESIAN_POINT('',(82.4264728367939,246.485672565813,30.7213203435596)) ;
#92691=CARTESIAN_POINT('Origin',(82.4264728367939,246.485672565813,30.6213203435596)) ;
#92692=CARTESIAN_POINT('Origin',(81.9668461709225,246.100000000001,30.7213203435596)) ;
#92693=CARTESIAN_POINT('Origin',(81.9668461709225,246.100000000001,30.6213203435596)) ;
#92694=CARTESIAN_POINT('Origin',(82.2322613127596,246.717124847304,30.6213203435596)) ;
#92695=CARTESIAN_POINT('',(82.2322613127596,246.717124847304,30.7213203435596)) ;
#92696=CARTESIAN_POINT('',(82.1556568684477,246.652846086335,30.6213203435596)) ;
#92697=CARTESIAN_POINT('Ctrl Pts',(83.9517583847478,244.512335651621,29.6213203435595)) ;
#92698=CARTESIAN_POINT('Ctrl Pts',(83.9517583847478,244.512335651621,29.613840361051)) ;
#92699=CARTESIAN_POINT('Ctrl Pts',(83.9530558516882,244.508154425815,29.5988871513645)) ;
#92700=CARTESIAN_POINT('Ctrl Pts',(83.9606617048516,244.483643751566,29.5704781111071)) ;
#92701=CARTESIAN_POINT('Ctrl Pts',(83.9826176510995,244.412888369528,29.5344326612966)) ;
#92702=CARTESIAN_POINT('Ctrl Pts',(84.0111728319539,244.320866249065,29.5213203435597)) ;
#92703=CARTESIAN_POINT('Ctrl Pts',(84.0283628290598,244.265469647218,29.5213203435596)) ;
#92704=CARTESIAN_POINT('Ctrl Pts',(83.9667167316546,244.494508987956,29.6213203435595)) ;
#92705=CARTESIAN_POINT('Ctrl Pts',(83.9667167316546,244.494508987956,29.6159323314173)) ;
#92706=CARTESIAN_POINT('Ctrl Pts',(83.9682471994807,244.491531314103,29.6051243850722)) ;
#92707=CARTESIAN_POINT('Ctrl Pts',(83.9770416840541,244.472839452493,29.5814625789605)) ;
#92708=CARTESIAN_POINT('Ctrl Pts',(84.0006986135097,244.41106523898,29.5432109886374)) ;
#92709=CARTESIAN_POINT('Ctrl Pts',(84.0277697425286,244.320862018183,29.5239057259475)) ;
#92710=CARTESIAN_POINT('Ctrl Pts',(84.0433227940768,244.265469647218,29.5213203435596)) ;
#92711=CARTESIAN_POINT('Ctrl Pts',(84.0041531339772,244.473067607354,29.6213203435595)) ;
#92712=CARTESIAN_POINT('Ctrl Pts',(84.0041531339772,244.473067607354,29.6184142549133)) ;
#92713=CARTESIAN_POINT('Ctrl Pts',(84.0057214037908,244.471884181008,29.6125402628528)) ;
#92714=CARTESIAN_POINT('Ctrl Pts',(84.0144435090324,244.461429167618,29.5934423510192)) ;
#92715=CARTESIAN_POINT('Ctrl Pts',(84.0362406374818,244.411135552903,29.549141027461)) ;
#92716=CARTESIAN_POINT('Ctrl Pts',(84.0578024133386,244.321730700198,29.52105144863)) ;
#92717=CARTESIAN_POINT('Ctrl Pts',(84.0694733069034,244.265469647218,29.515320264092)) ;
#92718=CARTESIAN_POINT('Ctrl Pts',(84.0702660875844,244.47874053303,29.6213203435596)) ;
#92719=CARTESIAN_POINT('Ctrl Pts',(84.0702660875844,244.47874053303,29.6177518125551)) ;
#92720=CARTESIAN_POINT('Ctrl Pts',(84.0711700553681,244.478120540662,29.6105411574913)) ;
#92721=CARTESIAN_POINT('Ctrl Pts',(84.0761457278699,244.469857764949,29.5866990606539)) ;
#92722=CARTESIAN_POINT('Ctrl Pts',(84.0879165906551,244.419942996463,29.5315349805942)) ;
#92723=CARTESIAN_POINT('Ctrl Pts',(84.0982144992168,244.325212271724,29.4977535048477)) ;
#92724=CARTESIAN_POINT('Ctrl Pts',(84.1035282741147,244.265469647218,29.4911830285845)) ;
#92725=CARTESIAN_POINT('Ctrl Pts',(84.1175427362197,244.518332038038,29.6213203435597)) ;
#92726=CARTESIAN_POINT('Ctrl Pts',(84.1175427362197,244.518332038038,29.6131456262106)) ;
#92727=CARTESIAN_POINT('Ctrl Pts',(84.1177289017234,244.51602318248,29.5967539236182)) ;
#92728=CARTESIAN_POINT('Ctrl Pts',(84.1187237882151,244.499413268429,29.5589225324798)) ;
#92729=CARTESIAN_POINT('Ctrl Pts',(84.1210267578767,244.43415692223,29.4947295211468)) ;
#92730=CARTESIAN_POINT('Ctrl Pts',(84.1229625569563,244.329893500793,29.4628331350402)) ;
#92731=CARTESIAN_POINT('Ctrl Pts',(84.1239346802222,244.265469647218,29.45873191021)) ;
#92732=CARTESIAN_POINT('Ctrl Pts',(84.1283628290597,244.55916112007,29.6213203435597)) ;
#92733=CARTESIAN_POINT('Ctrl Pts',(84.1283628290597,244.55916112007,29.6083780388064)) ;
#92734=CARTESIAN_POINT('Ctrl Pts',(84.1283572386591,244.554786903413,29.5824972890339)) ;
#92735=CARTESIAN_POINT('Ctrl Pts',(84.1283610044671,244.528130184705,29.5313432230903)) ;
#92736=CARTESIAN_POINT('Ctrl Pts',(84.1283711082966,244.446079577053,29.4616562627835)) ;
#92737=CARTESIAN_POINT('Ctrl Pts',(84.1283567558621,244.333673921744,29.433760966027)) ;
#92738=CARTESIAN_POINT('Ctrl Pts',(84.1283628290597,244.265469647218,29.4325403173224)) ;
#92739=CARTESIAN_POINT('Ctrl Pts',(84.1283628290597,244.57661441259,29.6213203435597)) ;
#92740=CARTESIAN_POINT('Ctrl Pts',(84.1283628290597,244.57661441259,29.6063603785426)) ;
#92741=CARTESIAN_POINT('Ctrl Pts',(84.1283628290597,244.571344482752,29.5764539591696)) ;
#92742=CARTESIAN_POINT('Ctrl Pts',(84.1283628290597,244.54045173992,29.5196358786547)) ;
#92743=CARTESIAN_POINT('Ctrl Pts',(84.1283628290597,244.451273131483,29.4475449790337)) ;
#92744=CARTESIAN_POINT('Ctrl Pts',(84.1283628290597,244.335290369296,29.4213203435596)) ;
#92745=CARTESIAN_POINT('Ctrl Pts',(84.1283628290597,244.265469647218,29.4213203435596)) ;
#92746=CARTESIAN_POINT('',(83.9517583847478,244.512335651621,29.6213203435596)) ;
#92747=CARTESIAN_POINT('Origin',(84.0283628290597,244.265469647218,29.6213203435596)) ;
#92748=CARTESIAN_POINT('',(84.1283628290597,244.265469647218,29.4213203435596)) ;
#92749=CARTESIAN_POINT('Origin',(84.0283628290597,244.265469647218,29.4213203435596)) ;
#92750=CARTESIAN_POINT('',(84.1283628290597,244.57661441259,29.6213203435596)) ;
#92751=CARTESIAN_POINT('Origin',(84.1283628290597,244.265469647218,29.6213203435596)) ;
#92752=CARTESIAN_POINT('Origin',(84.0283628290597,244.57661441259,29.6213203435596)) ;
#92753=CARTESIAN_POINT('Origin',(82.2,237.60736287746,29.4213203435596)) ;
#92754=CARTESIAN_POINT('',(82.1222820569742,238.604338263983,29.4213203435596)) ;
#92755=CARTESIAN_POINT('Origin',(82.2,237.60736287746,29.4213203435596)) ;
#92756=CARTESIAN_POINT('Origin',(82.1145102626716,238.704035802635,29.4213203435596)) ;
#92757=CARTESIAN_POINT('Ctrl Pts',(82.1833429126806,238.739454580319,29.5213203435596)) ;
#92758=CARTESIAN_POINT('Ctrl Pts',(82.1563604922519,238.707298183835,29.5213203435596)) ;
#92759=CARTESIAN_POINT('Ctrl Pts',(82.1145102626715,238.704035802636,29.5213203435597)) ;
#92760=CARTESIAN_POINT('Ctrl Pts',(82.2599473569943,238.675175819352,29.5213203435603)) ;
#92761=CARTESIAN_POINT('Ctrl Pts',(82.2059825161353,238.610863026382,29.5213203435603)) ;
#92762=CARTESIAN_POINT('Ctrl Pts',(82.1222820569719,238.604338263983,29.5213203435605)) ;
#92763=CARTESIAN_POINT('Ctrl Pts',(82.2599473569942,238.675175819352,29.4213203435594)) ;
#92764=CARTESIAN_POINT('Ctrl Pts',(82.2059825161351,238.610863026382,29.4213203435594)) ;
#92765=CARTESIAN_POINT('Ctrl Pts',(82.1222820569716,238.604338263983,29.4213203435596)) ;
#92766=CARTESIAN_POINT('',(82.2599473569929,238.67517581935,29.4213203435596)) ;
#92767=CARTESIAN_POINT('Origin',(82.183342912681,238.739454580319,29.4213203435596)) ;
#92768=CARTESIAN_POINT('Origin',(82.106738468369,238.803733341288,29.4213203435596)) ;
#92769=CARTESIAN_POINT('Origin',(77.9743376460485,233.723357432561,29.4213203435596)) ;
#92770=CARTESIAN_POINT('',(84.0113850506191,240.762457982934,29.4213203435596)) ;
#92771=CARTESIAN_POINT('Origin',(83.9347806063072,240.826736743903,29.4213203435596)) ;
#92772=CARTESIAN_POINT('',(78.0509420903604,233.659078671593,29.4213203435596)) ;
#92773=CARTESIAN_POINT('Origin',(83.6283628290597,241.083851787777,29.4213203435596)) ;
#92774=CARTESIAN_POINT('',(84.1283628290596,241.083851787777,29.4213203435596)) ;
#92775=CARTESIAN_POINT('Origin',(84.0283628290596,241.083851787777,29.4213203435596)) ;
#92776=CARTESIAN_POINT('Origin',(83.6283628290597,241.083851787777,29.4213203435596)) ;
#92777=CARTESIAN_POINT('Origin',(84.0283628290597,247.594124250979,29.4213203435596)) ;
#92778=CARTESIAN_POINT('',(84.1283628290597,247.594124250979,29.4213203435596)) ;
#92779=CARTESIAN_POINT('Origin',(84.0283628290597,244.57661441259,30.1213203435596)) ;
#92780=CARTESIAN_POINT('',(84.1283628290597,244.57661441259,30.1213203435596)) ;
#92781=CARTESIAN_POINT('',(83.9517583847478,244.512335651621,30.1213203435596)) ;
#92782=CARTESIAN_POINT('Origin',(78.9611335727037,250.304358317977,29.6213203435596)) ;
#92783=CARTESIAN_POINT('',(82.349868392482,246.421393804845,29.6213203435596)) ;
#92784=CARTESIAN_POINT('Origin',(82.27326394817,246.357115043876,29.6213203435596)) ;
#92785=CARTESIAN_POINT('',(79.0377380170156,250.368637078946,29.6213203435596)) ;
#92786=CARTESIAN_POINT('Origin',(81.9668461709225,246.100000000001,29.6213203435596)) ;
#92787=CARTESIAN_POINT('',(81.9668461709225,246.600000000001,29.6213203435596)) ;
#92788=CARTESIAN_POINT('Origin',(81.9668461709225,246.500000000001,29.6213203435596)) ;
#92789=CARTESIAN_POINT('Origin',(81.9668461709225,246.100000000001,29.6213203435596)) ;
#92790=CARTESIAN_POINT('Origin',(68.5905137927262,246.500000000001,29.6213203435596)) ;
#92791=CARTESIAN_POINT('',(80.6401337790902,246.600000000001,29.6213203435596)) ;
#92792=CARTESIAN_POINT('Origin',(80.6401337790902,246.500000000001,29.6213203435596)) ;
#92793=CARTESIAN_POINT('',(68.5905137927262,246.600000000001,29.6213203435596)) ;
#92794=CARTESIAN_POINT('Ctrl Pts',(80.6401337790902,246.600000000001,29.6213203435597)) ;
#92795=CARTESIAN_POINT('Ctrl Pts',(80.6401337790902,246.600000000001,29.6213203435597)) ;
#92796=CARTESIAN_POINT('Ctrl Pts',(80.6401337790902,246.600000000001,29.6213203435597)) ;
#92797=CARTESIAN_POINT('Ctrl Pts',(80.6401337790902,246.600000000001,29.6213203435597)) ;
#92798=CARTESIAN_POINT('Ctrl Pts',(80.6401337790902,246.600000000001,29.6213203435597)) ;
#92799=CARTESIAN_POINT('Ctrl Pts',(80.6401337790903,246.600000000001,29.5213203435596)) ;
#92800=CARTESIAN_POINT('Ctrl Pts',(80.6401337790903,246.600000000001,29.5213203435596)) ;
#92801=CARTESIAN_POINT('Ctrl Pts',(80.6401337790903,246.600000000001,29.5213203435596)) ;
#92802=CARTESIAN_POINT('Ctrl Pts',(80.6401337790903,246.600000000001,29.5213203435596)) ;
#92803=CARTESIAN_POINT('Ctrl Pts',(80.6401337790903,246.600000000001,29.5213203435596)) ;
#92804=CARTESIAN_POINT('Ctrl Pts',(80.5401534070281,246.601981212341,29.5213203435596)) ;
#92805=CARTESIAN_POINT('Ctrl Pts',(80.5393212408706,246.559986580887,29.5213203435596)) ;
#92806=CARTESIAN_POINT('Ctrl Pts',(80.5687260721042,246.529993290444,29.5213203435596)) ;
#92807=CARTESIAN_POINT('Ctrl Pts',(80.5981309033378,246.500000000001,29.5213203435596)) ;
#92808=CARTESIAN_POINT('Ctrl Pts',(80.6401337790903,246.500000000001,29.5213203435596)) ;
#92809=CARTESIAN_POINT('',(80.6401238113489,246.599999197424,29.6199061653688)) ;
#92810=CARTESIAN_POINT('Ctrl Pts',(80.6401238113489,246.599999197424,29.6199061653688)) ;
#92811=CARTESIAN_POINT('Ctrl Pts',(80.6400214277435,246.599990954774,29.6126436721215)) ;
#92812=CARTESIAN_POINT('Ctrl Pts',(80.6391298693545,246.599917417426,29.6054249823856)) ;
#92813=CARTESIAN_POINT('Ctrl Pts',(80.6374776063121,246.599793218341,29.5983912376924)) ;
#92814=CARTESIAN_POINT('Ctrl Pts',(80.6360675394583,246.599687224918,29.5923885311043)) ;
#92815=CARTESIAN_POINT('Ctrl Pts',(80.6341044490985,246.599544836505,29.5865185837269)) ;
#92816=CARTESIAN_POINT('Ctrl Pts',(80.6316004329604,246.599386263502,29.5808495764825)) ;
#92817=CARTESIAN_POINT('Ctrl Pts',(80.6277164645829,246.599140301617,29.5720564043727)) ;
#92818=CARTESIAN_POINT('Ctrl Pts',(80.6225913378422,246.598858783748,29.563888015334)) ;
#92819=CARTESIAN_POINT('Ctrl Pts',(80.6163938828428,246.59865549242,29.5565886095391)) ;
#92820=CARTESIAN_POINT('Ctrl Pts',(80.6142499206385,246.598585165339,29.5540634358768)) ;
#92821=CARTESIAN_POINT('Ctrl Pts',(80.611977402984,246.598524419104,29.5516418882813)) ;
#92822=CARTESIAN_POINT('Ctrl Pts',(80.6095830539163,246.59847852032,29.5493338457366)) ;
#92823=CARTESIAN_POINT('Ctrl Pts',(80.6024960843674,246.598342665743,29.5425023325488)) ;
#92824=CARTESIAN_POINT('Ctrl Pts',(80.5944545576649,246.598341217034,29.5367728369097)) ;
#92825=CARTESIAN_POINT('Ctrl Pts',(80.5857225147289,246.598590611719,29.5323072497772)) ;
#92826=CARTESIAN_POINT('Ctrl Pts',(80.5830669391223,246.598666457252,29.5309491822156)) ;
#92827=CARTESIAN_POINT('Ctrl Pts',(80.5803476365109,246.598765322088,29.5297081953568)) ;
#92828=CARTESIAN_POINT('Ctrl Pts',(80.5775730890624,246.598889896522,29.5285893595314)) ;
#92829=CARTESIAN_POINT('Ctrl Pts',(80.570390042797,246.599212408188,29.5256927972462)) ;
#92830=CARTESIAN_POINT('Ctrl Pts',(80.5629312514651,246.599704883803,29.5236511049122)) ;
#92831=CARTESIAN_POINT('Ctrl Pts',(80.5553357905141,246.600386015029,29.5224824684264)) ;
#92832=CARTESIAN_POINT('Ctrl Pts',(80.5503172535888,246.600836057789,29.5217103170858)) ;
#92833=CARTESIAN_POINT('Ctrl Pts',(80.5452392666734,246.601368061613,29.5213203435596)) ;
#92834=CARTESIAN_POINT('Ctrl Pts',(80.5401534070282,246.601981212341,29.5213203435596)) ;
#92835=CARTESIAN_POINT('Ctrl Pts',(80.6401337790902,246.600000000001,29.6213203435596)) ;
#92836=CARTESIAN_POINT('Ctrl Pts',(80.6401337790902,246.600000000001,29.6208503040069)) ;
#92837=CARTESIAN_POINT('Ctrl Pts',(80.6401304771049,246.599999716412,29.6203788915336)) ;
#92838=CARTESIAN_POINT('Ctrl Pts',(80.6401238157683,246.599999144307,29.6199061653688)) ;
#92839=CARTESIAN_POINT('Origin',(82.384248304075,250.850933335322,30.7213203435596)) ;
#92840=CARTESIAN_POINT('',(81.1,247.600000000001,30.7213203435596)) ;
#92841=CARTESIAN_POINT('',(81.9668461709226,247.600000000001,30.7213203435596)) ;
#92842=CARTESIAN_POINT('',(81.1,247.098386676966,30.7213203435596)) ;
#92843=CARTESIAN_POINT('',(81.1,257.151471862576,30.7213203435596)) ;
#92844=CARTESIAN_POINT('Origin',(80.6,247.098386676966,30.7213203435596)) ;
#92845=CARTESIAN_POINT('Origin',(79.2,263.8,29.5213203435596)) ;
#92846=CARTESIAN_POINT('',(79.2,259.648528137424,20.1213203435596)) ;
#92847=CARTESIAN_POINT('',(79.2,259.648528137424,29.5213203435596)) ;
#92848=CARTESIAN_POINT('',(79.2,261.751937515251,20.1213203435596)) ;
#92849=CARTESIAN_POINT('',(79.2,252.258305665508,20.1213203435596)) ;
#92850=CARTESIAN_POINT('',(79.2,263.412347523777,22.196832854217)) ;
#92851=CARTESIAN_POINT('',(79.2,264.929230192226,24.0929361897785)) ;
#92852=CARTESIAN_POINT('Origin',(79.2,263.1,22.4467108732387)) ;
#92853=CARTESIAN_POINT('Origin',(79.7999999999999,259.648528137424,29.5213203435596)) ;
#92854=CARTESIAN_POINT('',(79.3757359312881,259.224264068712,20.1213203435596)) ;
#92855=CARTESIAN_POINT('',(79.3757359312881,259.224264068712,29.5213203435596)) ;
#92856=CARTESIAN_POINT('Origin',(79.7999999999999,259.648528137424,20.1213203435596)) ;
#92857=CARTESIAN_POINT('Origin',(79.3757359312881,259.224264068712,29.5213203435596)) ;
#92858=CARTESIAN_POINT('',(83.8354696102463,254.764530389755,20.1213203435596)) ;
#92859=CARTESIAN_POINT('',(83.8354696102463,254.764530389755,29.5213203435596)) ;
#92860=CARTESIAN_POINT('',(77.9622604865213,260.637739513478,20.1213203435596)) ;
#92861=CARTESIAN_POINT('Origin',(83.1283628290598,254.057423608568,29.5213203435596)) ;
#92862=CARTESIAN_POINT('',(84.1283628290598,254.057423608568,20.1213203435596)) ;
#92863=CARTESIAN_POINT('',(84.1283628290598,254.057423608568,29.5213203435596)) ;
#92864=CARTESIAN_POINT('Origin',(83.1283628290598,254.057423608568,20.1213203435596)) ;
#92865=CARTESIAN_POINT('Origin',(84.1283628290598,254.471637170941,29.5213203435596)) ;
#92866=CARTESIAN_POINT('',(84.1283628290596,241.083851787777,17.0213468614911)) ;
#92867=CARTESIAN_POINT('',(84.1283628290596,241.083851787777,29.5213203435596)) ;
#92868=CARTESIAN_POINT('',(84.1283628290597,244.252914644012,18.0777011469026)) ;
#92869=CARTESIAN_POINT('',(84.1283628290597,249.125613950322,19.7019342490059)) ;
#92870=CARTESIAN_POINT('',(84.1283628290597,244.521708245126,18.1213203435596)) ;
#92871=CARTESIAN_POINT('Origin',(84.1283628290597,244.521708245126,17.2713203435596)) ;
#92872=CARTESIAN_POINT('',(84.1283628290597,250.68933982822,18.1213203435596)) ;
#92873=CARTESIAN_POINT('',(84.1283628290598,251.76081858547,18.1213203435596)) ;
#92874=CARTESIAN_POINT('',(84.1283628290597,251.148959235991,18.3117009357884)) ;
#92875=CARTESIAN_POINT('Origin',(84.1283628290597,250.68933982822,18.7713203435596)) ;
#92876=CARTESIAN_POINT('',(84.1283628290598,252.782842712475,19.9455844122716)) ;
#92877=CARTESIAN_POINT('',(84.1283628290598,255.172198614617,22.3349403144135)) ;
#92878=CARTESIAN_POINT('',(84.1283628290598,253.207106781187,20.1213203435596)) ;
#92879=CARTESIAN_POINT('Origin',(84.1283628290598,253.207106781187,19.5213203435596)) ;
#92880=CARTESIAN_POINT('',(84.1283628290597,247.594124250979,20.1213203435596)) ;
#92881=CARTESIAN_POINT('Origin',(83.6283628290597,241.083851787777,29.5213203435596)) ;
#92882=CARTESIAN_POINT('',(84.0113850506191,240.762457982934,16.9356418468662)) ;
#92883=CARTESIAN_POINT('',(84.0113850506191,240.762457982934,29.5213203435596)) ;
#92884=CARTESIAN_POINT('Origin',(83.6283628290597,241.083851787777,17.0213468614911)) ;
#92885=CARTESIAN_POINT('Origin',(84.0113850506191,240.762457982934,29.5213203435596)) ;
#92886=CARTESIAN_POINT('',(82.2599473569929,238.67517581935,16.2398811256715)) ;
#92887=CARTESIAN_POINT('',(82.2599473569929,238.67517581935,29.5213203435596)) ;
#92888=CARTESIAN_POINT('',(82.1162867009651,238.503967716415,16.1828117580263)) ;
#92889=CARTESIAN_POINT('Origin',(82.106738468369,238.803733341288,29.5213203435596)) ;
#92890=CARTESIAN_POINT('',(82.1222820569742,238.604338263983,16.2280748664436)) ;
#92891=CARTESIAN_POINT('',(82.1222820569742,238.604338263983,29.5213203435596)) ;
#92892=CARTESIAN_POINT('Origin',(82.106738468369,238.803733341288,16.2613073793278)) ;
#92893=CARTESIAN_POINT('Origin',(82.2,237.60736287746,29.5213203435596)) ;
#92894=CARTESIAN_POINT('',(81.4075488173165,238.217298220807,16.1213203435596)) ;
#92895=CARTESIAN_POINT('Origin',(82.2,237.60736287746,16.1213203435596)) ;
#92896=CARTESIAN_POINT('',(81.5957531842379,238.404160082301,16.1546761998268)) ;
#92897=CARTESIAN_POINT('Ctrl Pts',(81.5957531842379,238.404160082301,16.1546761998268)) ;
#92898=CARTESIAN_POINT('Ctrl Pts',(81.5259305404763,238.351210461111,16.135261338724)) ;
#92899=CARTESIAN_POINT('Ctrl Pts',(81.4620702891285,238.288134589433,16.1213203435918)) ;
#92900=CARTESIAN_POINT('Ctrl Pts',(81.4075488173165,238.217298220807,16.1213203435596)) ;
#92901=CARTESIAN_POINT('Origin',(82.2,237.60736287746,15.8625172247187)) ;
#92902=CARTESIAN_POINT('Ctrl Pts',(34.7,253.1,20.1116830603904)) ;
#92903=CARTESIAN_POINT('Ctrl Pts',(34.7,253.073427194197,20.102041097524)) ;
#92904=CARTESIAN_POINT('Ctrl Pts',(34.7154525608087,253.037274993038,20.0767697983353)) ;
#92905=CARTESIAN_POINT('Ctrl Pts',(34.7577940821299,253.006604388018,20.0446943852455)) ;
#92906=CARTESIAN_POINT('Ctrl Pts',(34.7845676632082,253.,20.0367671642397)) ;
#92907=CARTESIAN_POINT('Ctrl Pts',(34.8,253.,20.0367671642397)) ;
#92908=CARTESIAN_POINT('Ctrl Pts',(34.7,253.105341045666,20.0822437084198)) ;
#92909=CARTESIAN_POINT('Ctrl Pts',(34.6985373524762,253.081350046773,20.0739929287702)) ;
#92910=CARTESIAN_POINT('Ctrl Pts',(34.7093726656571,253.044545930682,20.0527380915968)) ;
#92911=CARTESIAN_POINT('Ctrl Pts',(34.752901551485,253.008047944834,20.0242500678859)) ;
#92912=CARTESIAN_POINT('Ctrl Pts',(34.7827658172387,253.,20.0170821036701)) ;
#92913=CARTESIAN_POINT('Ctrl Pts',(34.8,253.,20.0170821036701)) ;
#92914=CARTESIAN_POINT('Ctrl Pts',(34.6748678850179,253.11458383057,20.0312983289888)) ;
#92915=CARTESIAN_POINT('Ctrl Pts',(34.6726125261121,253.088119687564,20.0253228616253)) ;
#92916=CARTESIAN_POINT('Ctrl Pts',(34.6847726429031,253.044720925911,20.0108918141144)) ;
#92917=CARTESIAN_POINT('Ctrl Pts',(34.7400669620698,252.999455928905,19.988446023804)) ;
#92918=CARTESIAN_POINT('Ctrl Pts',(34.7779762508729,252.989510818984,19.982705579958)) ;
#92919=CARTESIAN_POINT('Ctrl Pts',(34.8,252.989510818984,19.982705579958)) ;
#92920=CARTESIAN_POINT('Ctrl Pts',(34.6224399475256,253.117851130198,20.013289274252)) ;
#92921=CARTESIAN_POINT('Ctrl Pts',(34.6217681694945,253.0793292346,20.0063128558354)) ;
#92922=CARTESIAN_POINT('Ctrl Pts',(34.64705596785,253.024324397392,19.9886074342206)) ;
#92923=CARTESIAN_POINT('Ctrl Pts',(34.7229377514464,252.974645254944,19.9645026828736)) ;
#92924=CARTESIAN_POINT('Ctrl Pts',(34.7717862253283,252.963867715888,19.9584161302793)) ;
#92925=CARTESIAN_POINT('Ctrl Pts',(34.8,252.963867715888,19.9584161302793)) ;
#92926=CARTESIAN_POINT('Ctrl Pts',(34.6,253.117851130198,20.013289274252)) ;
#92927=CARTESIAN_POINT('Ctrl Pts',(34.6,253.073563120525,20.0052543051966)) ;
#92928=CARTESIAN_POINT('Ctrl Pts',(34.6309051216174,253.013309451927,19.984194889206)) ;
#92929=CARTESIAN_POINT('Ctrl Pts',(34.7155881642597,252.962191776895,19.9574653782978)) ;
#92930=CARTESIAN_POINT('Ctrl Pts',(34.7691353264163,252.951184463531,19.950859360793)) ;
#92931=CARTESIAN_POINT('Ctrl Pts',(34.8,252.951184463531,19.950859360793)) ;
#92932=CARTESIAN_POINT('',(34.7,253.1,20.1116830603904)) ;
#92933=CARTESIAN_POINT('',(34.6,253.117851130198,20.013289274252)) ;
#92934=CARTESIAN_POINT('Origin',(34.6,253.1,20.1116830603904)) ;
#92935=CARTESIAN_POINT('',(34.8,253.,20.0367671642397)) ;
#92936=CARTESIAN_POINT('Ctrl Pts',(34.7,253.1,20.1116830603904)) ;
#92937=CARTESIAN_POINT('Ctrl Pts',(34.7,253.090812284823,20.1083492909262)) ;
#92938=CARTESIAN_POINT('Ctrl Pts',(34.7012689280364,253.081748379892,20.104053410188)) ;
#92939=CARTESIAN_POINT('Ctrl Pts',(34.7036906162496,253.073083414005,20.0991758790423)) ;
#92940=CARTESIAN_POINT('Ctrl Pts',(34.7063605193339,253.06353031835,20.0937984174113)) ;
#92941=CARTESIAN_POINT('Ctrl Pts',(34.7104314447552,253.054461536474,20.087713960402)) ;
#92942=CARTESIAN_POINT('Ctrl Pts',(34.715711247738,253.046191020804,20.0814323572824)) ;
#92943=CARTESIAN_POINT('Ctrl Pts',(34.7194931489978,253.040266884291,20.0769328706863)) ;
#92944=CARTESIAN_POINT('Ctrl Pts',(34.723894682151,253.034751119387,20.0723322323984)) ;
#92945=CARTESIAN_POINT('Ctrl Pts',(34.7288341851766,253.029747407162,20.0678178206808)) ;
#92946=CARTESIAN_POINT('Ctrl Pts',(34.735485753755,253.023009374036,20.0617386829671)) ;
#92947=CARTESIAN_POINT('Ctrl Pts',(34.7431037307269,253.017203083895,20.0558159042037)) ;
#92948=CARTESIAN_POINT('Ctrl Pts',(34.7515160670353,253.012539676171,20.0508560690148)) ;
#92949=CARTESIAN_POINT('Ctrl Pts',(34.7529089921345,253.011767503325,20.0500348133411)) ;
#92950=CARTESIAN_POINT('Ctrl Pts',(34.7543236613454,253.011026776857,20.0492399588338)) ;
#92951=CARTESIAN_POINT('Ctrl Pts',(34.7557592220037,253.010318599686,20.0484751671979)) ;
#92952=CARTESIAN_POINT('Ctrl Pts',(34.7618259802646,253.007325804029,20.0452431157008)) ;
#92953=CARTESIAN_POINT('Ctrl Pts',(34.7682623077884,253.004920839274,20.0425479732772)) ;
#92954=CARTESIAN_POINT('Ctrl Pts',(34.7749219946318,253.003195590768,20.0405614926115)) ;
#92955=CARTESIAN_POINT('Ctrl Pts',(34.7815569385043,253.001476752139,20.038582392388)) ;
#92956=CARTESIAN_POINT('Ctrl Pts',(34.7884125679264,253.000433128784,20.0373066978724)) ;
#92957=CARTESIAN_POINT('Ctrl Pts',(34.795320947479,253.000109527644,20.0369042544962)) ;
#92958=CARTESIAN_POINT('Ctrl Pts',(34.7968786750153,253.000036560836,20.0368135100424)) ;
#92959=CARTESIAN_POINT('Ctrl Pts',(34.7984390268306,253.,20.0367671642397)) ;
#92960=CARTESIAN_POINT('Ctrl Pts',(34.8,253.,20.0367671642397)) ;
#92961=CARTESIAN_POINT('',(34.8,252.951184463531,19.950859360793)) ;
#92962=CARTESIAN_POINT('Origin',(34.8,252.9,20.0367671642397)) ;
#92963=CARTESIAN_POINT('Ctrl Pts',(34.8,252.951184463531,19.950859360793)) ;
#92964=CARTESIAN_POINT('Ctrl Pts',(34.7691353264163,252.951184463531,19.950859360793)) ;
#92965=CARTESIAN_POINT('Ctrl Pts',(34.7155881642597,252.962191776895,19.9574653782978)) ;
#92966=CARTESIAN_POINT('Ctrl Pts',(34.6309051216174,253.013309451927,19.984194889206)) ;
#92967=CARTESIAN_POINT('Ctrl Pts',(34.6,253.073563120525,20.0052543051966)) ;
#92968=CARTESIAN_POINT('Ctrl Pts',(34.6,253.117851130198,20.013289274252)) ;
#92969=CARTESIAN_POINT('Origin',(34.8,253.1,20.0213203435596)) ;
#92970=CARTESIAN_POINT('',(34.8,253.,25.7213203435596)) ;
#92971=CARTESIAN_POINT('',(34.7,253.1,25.7213203435596)) ;
#92972=CARTESIAN_POINT('Origin',(34.8,253.1,25.7213203435596)) ;
#92973=CARTESIAN_POINT('',(34.8,253.,20.0213203435596)) ;
#92974=CARTESIAN_POINT('',(34.7,253.1,20.0213203435596)) ;
#92975=CARTESIAN_POINT('Origin',(34.8,258.9,20.1213203435596)) ;
#92976=CARTESIAN_POINT('',(34.7,258.9,20.1213203435596)) ;
#92977=CARTESIAN_POINT('',(34.8,259.,20.1213203435596)) ;
#92978=CARTESIAN_POINT('Origin',(34.8,258.9,20.1213203435596)) ;
#92979=CARTESIAN_POINT('',(34.6,258.9,20.0213203435596)) ;
#92980=CARTESIAN_POINT('Origin',(34.6,258.9,20.1213203435596)) ;
#92981=CARTESIAN_POINT('',(34.8,259.1,20.0213203435596)) ;
#92982=CARTESIAN_POINT('Origin',(34.8,258.9,20.0213203435596)) ;
#92983=CARTESIAN_POINT('Origin',(34.8,259.1,20.1213203435596)) ;
#92984=CARTESIAN_POINT('Origin',(34.6,249.858305665508,20.1213203435596)) ;
#92985=CARTESIAN_POINT('',(34.7,253.207106781187,20.1213203435596)) ;
#92986=CARTESIAN_POINT('',(34.6,253.207106781187,20.0213203435596)) ;
#92987=CARTESIAN_POINT('Origin',(34.6,253.207106781187,20.1213203435596)) ;
#92988=CARTESIAN_POINT('',(34.6,249.858305665508,20.0213203435596)) ;
#92989=CARTESIAN_POINT('',(34.7,249.858305665508,20.1213203435596)) ;
#92990=CARTESIAN_POINT('Origin',(34.6,253.207106781187,19.5213203435596)) ;
#92991=CARTESIAN_POINT('Origin',(34.7,253.207106781187,19.5213203435596)) ;
#92992=CARTESIAN_POINT('Origin',(34.6,253.207106781187,19.5213203435596)) ;
#92993=CARTESIAN_POINT('Origin',(45.6,258.9,20.1213203435596)) ;
#92994=CARTESIAN_POINT('',(45.6,259.1,20.0213203435596)) ;
#92995=CARTESIAN_POINT('',(45.8,258.9,20.0213203435596)) ;
#92996=CARTESIAN_POINT('Origin',(45.6,258.9,20.0213203435596)) ;
#92997=CARTESIAN_POINT('',(45.7,258.9,20.1213203435596)) ;
#92998=CARTESIAN_POINT('Origin',(45.8,258.9,20.1213203435596)) ;
#92999=CARTESIAN_POINT('',(45.6,259.,20.1213203435596)) ;
#93000=CARTESIAN_POINT('Origin',(45.6,258.9,20.1213203435596)) ;
#93001=CARTESIAN_POINT('Origin',(45.6,259.1,20.1213203435596)) ;
#93002=CARTESIAN_POINT('Ctrl Pts',(45.6,253.,20.0367671642397)) ;
#93003=CARTESIAN_POINT('Ctrl Pts',(45.6154322006349,253.,20.0367671642397)) ;
#93004=CARTESIAN_POINT('Ctrl Pts',(45.6422059127972,253.006604965661,20.0446949534528)) ;
#93005=CARTESIAN_POINT('Ctrl Pts',(45.6845468602172,253.037276279324,20.0767704565364)) ;
#93006=CARTESIAN_POINT('Ctrl Pts',(45.7,253.073427428644,20.1020411825935)) ;
#93007=CARTESIAN_POINT('Ctrl Pts',(45.7,253.1,20.1116830603905)) ;
#93008=CARTESIAN_POINT('Ctrl Pts',(45.6,253.,20.0170821036701)) ;
#93009=CARTESIAN_POINT('Ctrl Pts',(45.617234030707,253.,20.0170821036701)) ;
#93010=CARTESIAN_POINT('Ctrl Pts',(45.6470983872308,253.008048616484,20.0242505760926)) ;
#93011=CARTESIAN_POINT('Ctrl Pts',(45.6906265314711,253.044547162949,20.0527386488428)) ;
#93012=CARTESIAN_POINT('Ctrl Pts',(45.7014626346191,253.081350258442,20.0739930015655)) ;
#93013=CARTESIAN_POINT('Ctrl Pts',(45.7,253.105341045666,20.0822437084198)) ;
#93014=CARTESIAN_POINT('Ctrl Pts',(45.6,252.989510790392,19.9827055984603)) ;
#93015=CARTESIAN_POINT('Ctrl Pts',(45.6220235548152,252.989510790392,19.9827055984603)) ;
#93016=CARTESIAN_POINT('Ctrl Pts',(45.6599330014319,252.99945672555,19.988446495824)) ;
#93017=CARTESIAN_POINT('Ctrl Pts',(45.7152263354696,253.044722306011,20.0108922593322)) ;
#93018=CARTESIAN_POINT('Ctrl Pts',(45.7273875638952,253.088119897512,20.0253230440994)) ;
#93019=CARTESIAN_POINT('Ctrl Pts',(45.7251322248881,253.114583807029,20.0312984587423)) ;
#93020=CARTESIAN_POINT('Ctrl Pts',(45.6,252.963867715888,19.9584161302793)) ;
#93021=CARTESIAN_POINT('Ctrl Pts',(45.6282135257462,252.963867715888,19.9584161302793)) ;
#93022=CARTESIAN_POINT('Ctrl Pts',(45.6770622165507,252.974646180414,19.9645031139485)) ;
#93023=CARTESIAN_POINT('Ctrl Pts',(45.7529429049027,253.024326306312,19.9886079012294)) ;
#93024=CARTESIAN_POINT('Ctrl Pts',(45.7782318245786,253.079329574472,20.0063129173872)) ;
#93025=CARTESIAN_POINT('Ctrl Pts',(45.7775600524744,253.117851130198,20.013289274252)) ;
#93026=CARTESIAN_POINT('Ctrl Pts',(45.6,252.951184463531,19.950859360793)) ;
#93027=CARTESIAN_POINT('Ctrl Pts',(45.6308644012698,252.951184463531,19.950859360793)) ;
#93028=CARTESIAN_POINT('Ctrl Pts',(45.6844118255944,252.962192739633,19.9574658518039)) ;
#93029=CARTESIAN_POINT('Ctrl Pts',(45.7690937204345,253.013311595737,19.9841954377069)) ;
#93030=CARTESIAN_POINT('Ctrl Pts',(45.8,253.073563511271,20.0052543760878)) ;
#93031=CARTESIAN_POINT('Ctrl Pts',(45.8,253.117851130198,20.013289274252)) ;
#93032=CARTESIAN_POINT('',(45.7,253.1,20.1116830603904)) ;
#93033=CARTESIAN_POINT('',(45.6,253.,20.0367671642397)) ;
#93034=CARTESIAN_POINT('Ctrl Pts',(45.6,253.,20.0367671642397)) ;
#93035=CARTESIAN_POINT('Ctrl Pts',(45.606919815088,253.,20.0367671642397)) ;
#93036=CARTESIAN_POINT('Ctrl Pts',(45.6138266569514,253.000722532008,20.0376780151623)) ;
#93037=CARTESIAN_POINT('Ctrl Pts',(45.6205496933934,253.002134224054,20.0393300400749)) ;
#93038=CARTESIAN_POINT('Ctrl Pts',(45.6272994466678,253.003551526057,20.0409886300082)) ;
#93039=CARTESIAN_POINT('Ctrl Pts',(45.6338628594197,253.005663017448,20.0433942963737)) ;
#93040=CARTESIAN_POINT('Ctrl Pts',(45.6400871492553,253.008386570501,20.0463753313402)) ;
#93041=CARTESIAN_POINT('Ctrl Pts',(45.641489340038,253.009000124993,20.0470468906447)) ;
#93042=CARTESIAN_POINT('Ctrl Pts',(45.6428744364713,253.009644566497,20.0477476498085)) ;
#93043=CARTESIAN_POINT('Ctrl Pts',(45.6442409123064,253.010318665943,20.0484756457334)) ;
#93044=CARTESIAN_POINT('Ctrl Pts',(45.6529108343034,253.014595645794,20.0530945842625)) ;
#93045=CARTESIAN_POINT('Ctrl Pts',(45.6608165325297,253.020055382737,20.0588099553703)) ;
#93046=CARTESIAN_POINT('Ctrl Pts',(45.6677833517525,253.026478457407,20.064815193976)) ;
#93047=CARTESIAN_POINT('Ctrl Pts',(45.6689369098378,253.027541982882,20.0658095346251)) ;
#93048=CARTESIAN_POINT('Ctrl Pts',(45.6700647610495,253.028632030776,20.0668118223869)) ;
#93049=CARTESIAN_POINT('Ctrl Pts',(45.6711661258947,253.029747722278,20.0678183958023)) ;
#93050=CARTESIAN_POINT('Ctrl Pts',(45.6781502406968,253.036822687096,20.0742014071367)) ;
#93051=CARTESIAN_POINT('Ctrl Pts',(45.6840571677146,253.044922670849,20.0807567550162)) ;
#93052=CARTESIAN_POINT('Ctrl Pts',(45.6886617904446,253.053749736053,20.0869548126948)) ;
#93053=CARTESIAN_POINT('Ctrl Pts',(45.6928454521279,253.061769818617,20.0925862352763)) ;
#93054=CARTESIAN_POINT('Ctrl Pts',(45.6959545781961,253.070390688776,20.0979227094103)) ;
#93055=CARTESIAN_POINT('Ctrl Pts',(45.6978463585031,253.079358049325,20.1025669910274)) ;
#93056=CARTESIAN_POINT('Ctrl Pts',(45.6992655848671,253.086085423777,20.1060511624654)) ;
#93057=CARTESIAN_POINT('Ctrl Pts',(45.7,253.09300731944,20.1091457609123)) ;
#93058=CARTESIAN_POINT('Ctrl Pts',(45.7,253.1,20.1116830603905)) ;
#93059=CARTESIAN_POINT('',(45.8,253.117851130198,20.013289274252)) ;
#93060=CARTESIAN_POINT('Origin',(45.8,253.1,20.1116830603904)) ;
#93061=CARTESIAN_POINT('',(45.6,252.951184463531,19.950859360793)) ;
#93062=CARTESIAN_POINT('Ctrl Pts',(45.8,253.117851130198,20.013289274252)) ;
#93063=CARTESIAN_POINT('Ctrl Pts',(45.8,253.073563511271,20.0052543760878)) ;
#93064=CARTESIAN_POINT('Ctrl Pts',(45.7690937204345,253.013311595737,19.9841954377069)) ;
#93065=CARTESIAN_POINT('Ctrl Pts',(45.6844118255944,252.962192739633,19.9574658518039)) ;
#93066=CARTESIAN_POINT('Ctrl Pts',(45.6308644012698,252.951184463531,19.950859360793)) ;
#93067=CARTESIAN_POINT('Ctrl Pts',(45.6,252.951184463531,19.950859360793)) ;
#93068=CARTESIAN_POINT('Origin',(45.6,252.9,20.0367671642397)) ;
#93069=CARTESIAN_POINT('Origin',(45.8,253.207106781187,19.5213203435596)) ;
#93070=CARTESIAN_POINT('',(45.7,253.207106781187,20.1213203435596)) ;
#93071=CARTESIAN_POINT('',(45.8,253.207106781187,20.0213203435596)) ;
#93072=CARTESIAN_POINT('Origin',(45.8,253.207106781187,20.1213203435596)) ;
#93073=CARTESIAN_POINT('Origin',(45.8,253.207106781187,19.5213203435596)) ;
#93074=CARTESIAN_POINT('Origin',(45.7,253.207106781187,19.5213203435596)) ;
#93075=CARTESIAN_POINT('Origin',(45.8,246.858305665508,20.1213203435596)) ;
#93076=CARTESIAN_POINT('',(45.8,246.858305665508,20.0213203435596)) ;
#93077=CARTESIAN_POINT('',(45.7,246.858305665508,20.1213203435596)) ;
#93078=CARTESIAN_POINT('Origin',(52.2356360608974,252.9,20.0367671642397)) ;
#93079=CARTESIAN_POINT('',(43.7,252.951184463531,19.950859360793)) ;
#93080=CARTESIAN_POINT('',(43.7,253.,20.0367671642397)) ;
#93081=CARTESIAN_POINT('Origin',(43.7,252.9,20.0367671642397)) ;
#93082=CARTESIAN_POINT('',(52.2356360608974,253.,20.0367671642397)) ;
#93083=CARTESIAN_POINT('',(52.2356360608974,252.951184463531,19.950859360793)) ;
#93084=CARTESIAN_POINT('Ctrl Pts',(43.7,252.951184463531,19.950859360793)) ;
#93085=CARTESIAN_POINT('Ctrl Pts',(43.6578667992531,252.951184463531,19.950859360793)) ;
#93086=CARTESIAN_POINT('Ctrl Pts',(43.5592720148238,252.933167716983,19.9409614991614)) ;
#93087=CARTESIAN_POINT('Ctrl Pts',(43.4889885639036,252.88263705024,19.9039573937935)) ;
#93088=CARTESIAN_POINT('Ctrl Pts',(43.4621585770309,252.853553390627,19.874873734187)) ;
#93089=CARTESIAN_POINT('Ctrl Pts',(43.7,252.968095466674,19.9609350534414)) ;
#93090=CARTESIAN_POINT('Ctrl Pts',(43.6546460334317,252.968095466674,19.9609350534414)) ;
#93091=CARTESIAN_POINT('Ctrl Pts',(43.5485580847433,252.947930175755,19.9508675198836)) ;
#93092=CARTESIAN_POINT('Ctrl Pts',(43.4726905198964,252.892278257511,19.9124287196735)) ;
#93093=CARTESIAN_POINT('Ctrl Pts',(43.4433278943641,252.860791518147,19.8821118617056)) ;
#93094=CARTESIAN_POINT('Ctrl Pts',(43.7,252.992258727451,19.987541529862)) ;
#93095=CARTESIAN_POINT('Ctrl Pts',(43.6490293347725,252.992258727451,19.987541529862)) ;
#93096=CARTESIAN_POINT('Ctrl Pts',(43.5298499627169,252.968039915603,19.9768771591682)) ;
#93097=CARTESIAN_POINT('Ctrl Pts',(43.4442147468097,252.9018819301,19.9359235128061)) ;
#93098=CARTESIAN_POINT('Ctrl Pts',(43.4104713759891,252.864580433427,19.9035816876055)) ;
#93099=CARTESIAN_POINT('Ctrl Pts',(43.7,253.,20.0220033688125)) ;
#93100=CARTESIAN_POINT('Ctrl Pts',(43.6450557170687,253.,20.0220033688125)) ;
#93101=CARTESIAN_POINT('Ctrl Pts',(43.5165377588455,252.972371460923,20.0104893451526)) ;
#93102=CARTESIAN_POINT('Ctrl Pts',(43.4245875894081,252.895637337396,19.9671199842894)) ;
#93103=CARTESIAN_POINT('Ctrl Pts',(43.3889646181901,252.851707610128,19.9329880225427)) ;
#93104=CARTESIAN_POINT('Ctrl Pts',(43.7,253.,20.0367671642397)) ;
#93105=CARTESIAN_POINT('Ctrl Pts',(43.6438223990041,253.,20.0367671642397)) ;
#93106=CARTESIAN_POINT('Ctrl Pts',(43.5123626864317,252.971173205522,20.0248897302817)) ;
#93107=CARTESIAN_POINT('Ctrl Pts',(43.4186514185382,252.890324138733,19.9804848038403)) ;
#93108=CARTESIAN_POINT('Ctrl Pts',(43.3828781027079,252.843790283354,19.9455844123125)) ;
#93109=CARTESIAN_POINT('',(43.3828781027079,252.843790283354,19.9455844123125)) ;
#93110=CARTESIAN_POINT('Origin',(43.4621585770309,252.782842712516,19.9455844123125)) ;
#93111=CARTESIAN_POINT('Ctrl Pts',(43.3828781027079,252.843790283354,19.9455844123125)) ;
#93112=CARTESIAN_POINT('Ctrl Pts',(43.4186514185382,252.890324138733,19.9804848038403)) ;
#93113=CARTESIAN_POINT('Ctrl Pts',(43.5123626864317,252.971173205522,20.0248897302817)) ;
#93114=CARTESIAN_POINT('Ctrl Pts',(43.6438223990041,253.,20.0367671642397)) ;
#93115=CARTESIAN_POINT('Ctrl Pts',(43.7,253.,20.0367671642397)) ;
#93116=CARTESIAN_POINT('Ctrl Pts',(43.7,252.951184463531,19.950859360793)) ;
#93117=CARTESIAN_POINT('Ctrl Pts',(43.6578667992531,252.951184463531,19.950859360793)) ;
#93118=CARTESIAN_POINT('Ctrl Pts',(43.5592720148238,252.933167716983,19.9409614991614)) ;
#93119=CARTESIAN_POINT('Ctrl Pts',(43.4889885639036,252.88263705024,19.9039573937935)) ;
#93120=CARTESIAN_POINT('Ctrl Pts',(43.4621585770309,252.853553390627,19.874873734187)) ;
#93121=CARTESIAN_POINT('Ctrl Pts',(43.4624808583665,252.853781762386,19.8751022254159)) ;
#93122=CARTESIAN_POINT('Ctrl Pts',(43.4223598267253,252.801696685177,19.8230175376221)) ;
#93123=CARTESIAN_POINT('Ctrl Pts',(43.400084060032,252.736117568422,19.7574370653152)) ;
#93124=CARTESIAN_POINT('Ctrl Pts',(43.4001799908286,252.670367473295,19.6916880667959)) ;
#93125=CARTESIAN_POINT('Ctrl Pts',(43.4436344606986,252.861063204372,19.8823434902912)) ;
#93126=CARTESIAN_POINT('Ctrl Pts',(43.3992601718949,252.807355530103,19.8285659598275)) ;
#93127=CARTESIAN_POINT('Ctrl Pts',(43.3731080437924,252.73934967782,19.7607787624628)) ;
#93128=CARTESIAN_POINT('Ctrl Pts',(43.3701830998102,252.670391495618,19.6916295804032)) ;
#93129=CARTESIAN_POINT('Ctrl Pts',(43.4107655857475,252.864902487303,19.9038322711337)) ;
#93130=CARTESIAN_POINT('Ctrl Pts',(43.359064232039,252.806033227451,19.8493878369772)) ;
#93131=CARTESIAN_POINT('Ctrl Pts',(43.3260192337239,252.731036352852,19.7803808851145)) ;
#93132=CARTESIAN_POINT('Ctrl Pts',(43.3182834834246,252.65257254548,19.709389345178)) ;
#93133=CARTESIAN_POINT('Ctrl Pts',(43.3892456815128,252.852053985775,19.9332636322348)) ;
#93134=CARTESIAN_POINT('Ctrl Pts',(43.3353433537132,252.785704020096,19.880468688359)) ;
#93135=CARTESIAN_POINT('Ctrl Pts',(43.3033941446389,252.701582066559,19.8138465043677)) ;
#93136=CARTESIAN_POINT('Ctrl Pts',(43.2999819361157,252.615417852383,19.7465229726415)) ;
#93137=CARTESIAN_POINT('Ctrl Pts',(43.383157199699,252.844152887956,19.9458563657641)) ;
#93138=CARTESIAN_POINT('Ctrl Pts',(43.329628501671,252.77469313003,19.8937615473196)) ;
#93139=CARTESIAN_POINT('Ctrl Pts',(43.2998965001866,252.687234889187,19.8281678666869)) ;
#93140=CARTESIAN_POINT('Ctrl Pts',(43.3000002707217,252.59954242249,19.7623985166642)) ;
#93141=CARTESIAN_POINT('',(43.3,252.6,19.7627416997969)) ;
#93142=CARTESIAN_POINT('Origin',(43.4,252.6,19.7627416997969)) ;
#93143=CARTESIAN_POINT('Origin',(43.7,252.6,19.7627416997969)) ;
#93144=CARTESIAN_POINT('Origin',(43.4,254.579289321881,21.7420310216783)) ;
#93145=CARTESIAN_POINT('',(43.3,254.579289321881,21.7420310216783)) ;
#93146=CARTESIAN_POINT('Origin',(45.6,253.1,20.0213203435596)) ;
#93147=CARTESIAN_POINT('',(45.7,253.1,25.7213203435596)) ;
#93148=CARTESIAN_POINT('',(45.6,253.,25.7213203435596)) ;
#93149=CARTESIAN_POINT('Origin',(45.6,253.1,25.7213203435596)) ;
#93150=CARTESIAN_POINT('',(45.7,253.1,20.0213203435596)) ;
#93151=CARTESIAN_POINT('',(45.6,253.,20.0213203435596)) ;
#93152=CARTESIAN_POINT('Origin',(43.1,252.1,19.3213203435596)) ;
#93153=CARTESIAN_POINT('',(43.1,251.9,19.3213203435596)) ;
#93154=CARTESIAN_POINT('Origin',(43.1,251.8,19.3213203435596)) ;
#93155=CARTESIAN_POINT('Origin',(43.1,252.1,19.3213203435596)) ;
#93156=CARTESIAN_POINT('Origin',(38.75,251.8,19.3213203435596)) ;
#93157=CARTESIAN_POINT('',(37.3,251.9,19.3213203435596)) ;
#93158=CARTESIAN_POINT('Origin',(37.3,251.8,19.3213203435596)) ;
#93159=CARTESIAN_POINT('',(38.75,251.9,19.3213203435596)) ;
#93160=CARTESIAN_POINT('Origin',(37.3,252.1,19.3213203435596)) ;
#93161=CARTESIAN_POINT('',(37.1,252.1,19.3213203435596)) ;
#93162=CARTESIAN_POINT('Origin',(37.,252.1,19.3213203435596)) ;
#93163=CARTESIAN_POINT('Origin',(37.3,252.1,19.3213203435596)) ;
#93164=CARTESIAN_POINT('Origin',(37.,254.9,19.3213203435596)) ;
#93165=CARTESIAN_POINT('',(37.1,254.9,19.3213203435596)) ;
#93166=CARTESIAN_POINT('Origin',(45.6,258.9,20.0213203435596)) ;
#93167=CARTESIAN_POINT('',(45.6,259.,25.7213203435596)) ;
#93168=CARTESIAN_POINT('',(45.7,258.9,25.7213203435596)) ;
#93169=CARTESIAN_POINT('Origin',(45.6,258.9,25.7213203435596)) ;
#93170=CARTESIAN_POINT('',(45.6,259.,20.0213203435596)) ;
#93171=CARTESIAN_POINT('',(45.7,258.9,20.0213203435596)) ;
#93172=CARTESIAN_POINT('Origin',(50.457090707265,259.1,20.1213203435596)) ;
#93173=CARTESIAN_POINT('',(43.7,259.,20.1213203435596)) ;
#93174=CARTESIAN_POINT('',(43.7,259.1,20.0213203435596)) ;
#93175=CARTESIAN_POINT('Origin',(43.7,259.1,20.1213203435596)) ;
#93176=CARTESIAN_POINT('',(50.457090707265,259.1,20.0213203435596)) ;
#93177=CARTESIAN_POINT('',(50.457090707265,259.,20.1213203435596)) ;
#93178=CARTESIAN_POINT('Origin',(43.7,259.4,20.1213203435596)) ;
#93179=CARTESIAN_POINT('',(43.3,259.4,20.1213203435596)) ;
#93180=CARTESIAN_POINT('',(43.4,259.4,20.0213203435596)) ;
#93181=CARTESIAN_POINT('Origin',(43.4,259.4,20.1213203435596)) ;
#93182=CARTESIAN_POINT('Origin',(43.7,259.4,20.0213203435596)) ;
#93183=CARTESIAN_POINT('Origin',(43.7,259.4,20.1213203435596)) ;
#93184=CARTESIAN_POINT('Origin',(43.4,246.408305665508,20.1213203435596)) ;
#93185=CARTESIAN_POINT('',(43.3,259.9,20.1213203435596)) ;
#93186=CARTESIAN_POINT('',(43.4,259.9,20.0213203435596)) ;
#93187=CARTESIAN_POINT('Origin',(43.4,259.9,20.1213203435596)) ;
#93188=CARTESIAN_POINT('',(43.4,246.408305665508,20.0213203435596)) ;
#93189=CARTESIAN_POINT('',(43.3,246.408305665508,20.1213203435596)) ;
#93190=CARTESIAN_POINT('Origin',(43.1,259.9,20.1213203435596)) ;
#93191=CARTESIAN_POINT('',(43.1,260.1,20.1213203435596)) ;
#93192=CARTESIAN_POINT('',(43.1,260.2,20.0213203435596)) ;
#93193=CARTESIAN_POINT('Origin',(43.1,260.2,20.1213203435596)) ;
#93194=CARTESIAN_POINT('Origin',(43.1,259.9,20.0213203435596)) ;
#93195=CARTESIAN_POINT('Origin',(43.1,259.9,20.1213203435596)) ;
#93196=CARTESIAN_POINT('Origin',(49.1570907072649,260.2,20.1213203435596)) ;
#93197=CARTESIAN_POINT('',(37.3,260.1,20.1213203435596)) ;
#93198=CARTESIAN_POINT('',(37.3,260.2,20.0213203435596)) ;
#93199=CARTESIAN_POINT('Origin',(37.3,260.2,20.1213203435596)) ;
#93200=CARTESIAN_POINT('',(49.1570907072649,260.2,20.0213203435596)) ;
#93201=CARTESIAN_POINT('',(49.1570907072649,260.1,20.1213203435596)) ;
#93202=CARTESIAN_POINT('Origin',(37.3,259.9,20.1213203435596)) ;
#93203=CARTESIAN_POINT('',(37.1,259.9,20.1213203435596)) ;
#93204=CARTESIAN_POINT('',(37.,259.9,20.0213203435596)) ;
#93205=CARTESIAN_POINT('Origin',(37.,259.9,20.1213203435596)) ;
#93206=CARTESIAN_POINT('Origin',(37.3,259.9,20.0213203435596)) ;
#93207=CARTESIAN_POINT('Origin',(37.3,259.9,20.1213203435596)) ;
#93208=CARTESIAN_POINT('Origin',(37.,250.308305665508,20.1213203435596)) ;
#93209=CARTESIAN_POINT('',(37.1,259.4,20.1213203435596)) ;
#93210=CARTESIAN_POINT('',(37.,259.4,20.0213203435596)) ;
#93211=CARTESIAN_POINT('Origin',(37.,259.4,20.1213203435596)) ;
#93212=CARTESIAN_POINT('',(37.,250.308305665508,20.0213203435596)) ;
#93213=CARTESIAN_POINT('',(37.1,250.308305665508,20.1213203435596)) ;
#93214=CARTESIAN_POINT('Origin',(36.7,259.4,20.1213203435596)) ;
#93215=CARTESIAN_POINT('',(36.7,259.,20.1213203435596)) ;
#93216=CARTESIAN_POINT('',(36.7,259.1,20.0213203435596)) ;
#93217=CARTESIAN_POINT('Origin',(36.7,259.1,20.1213203435596)) ;
#93218=CARTESIAN_POINT('Origin',(36.7,259.4,20.0213203435596)) ;
#93219=CARTESIAN_POINT('Origin',(36.7,259.4,20.1213203435596)) ;
#93220=CARTESIAN_POINT('Origin',(46.157090707265,259.1,20.1213203435596)) ;
#93221=CARTESIAN_POINT('',(46.157090707265,259.1,20.0213203435596)) ;
#93222=CARTESIAN_POINT('',(46.157090707265,259.,20.1213203435596)) ;
#93223=CARTESIAN_POINT('Origin',(52.2356360608974,252.9,20.0367671642397)) ;
#93224=CARTESIAN_POINT('',(36.7,253.,20.0367671642397)) ;
#93225=CARTESIAN_POINT('',(36.7,252.951184463531,19.950859360793)) ;
#93226=CARTESIAN_POINT('Origin',(36.7,252.9,20.0367671642397)) ;
#93227=CARTESIAN_POINT('',(52.2356360608974,252.951184463531,19.950859360793)) ;
#93228=CARTESIAN_POINT('',(52.2356360608974,253.,20.0367671642397)) ;
#93229=CARTESIAN_POINT('Ctrl Pts',(36.9378414229691,252.853553390627,19.874873734187)) ;
#93230=CARTESIAN_POINT('Ctrl Pts',(36.911011436074,252.882637050264,19.9039573938178)) ;
#93231=CARTESIAN_POINT('Ctrl Pts',(36.840727984334,252.933167717784,19.9409614997224)) ;
#93232=CARTESIAN_POINT('Ctrl Pts',(36.7421332007821,252.951184463531,19.950859360793)) ;
#93233=CARTESIAN_POINT('Ctrl Pts',(36.7,252.951184463531,19.950859360793)) ;
#93234=CARTESIAN_POINT('Ctrl Pts',(36.956672105636,252.860791518147,19.8821118617056)) ;
#93235=CARTESIAN_POINT('Ctrl Pts',(36.9273094800791,252.892278257538,19.9124287196988)) ;
#93236=CARTESIAN_POINT('Ctrl Pts',(36.8514419143484,252.947930176663,19.9508675204564)) ;
#93237=CARTESIAN_POINT('Ctrl Pts',(36.7453539666062,252.968095466674,19.9609350534414)) ;
#93238=CARTESIAN_POINT('Ctrl Pts',(36.7,252.968095466674,19.9609350534414)) ;
#93239=CARTESIAN_POINT('Ctrl Pts',(36.9895286392703,252.864580456291,19.9035816764723)) ;
#93240=CARTESIAN_POINT('Ctrl Pts',(36.9557852684216,252.901881952996,19.9359235017)) ;
#93241=CARTESIAN_POINT('Ctrl Pts',(36.8701500415939,252.968039937044,19.9768771497705)) ;
#93242=CARTESIAN_POINT('Ctrl Pts',(36.75097066527,252.99225874652,19.9875415204354)) ;
#93243=CARTESIAN_POINT('Ctrl Pts',(36.7,252.99225874652,19.9875415204354)) ;
#93244=CARTESIAN_POINT('Ctrl Pts',(37.0110353818099,252.851707610128,19.9329880225427)) ;
#93245=CARTESIAN_POINT('Ctrl Pts',(36.9754124105622,252.895637337432,19.9671199843179)) ;
#93246=CARTESIAN_POINT('Ctrl Pts',(36.8834622400518,252.972371462136,20.0104893458127)) ;
#93247=CARTESIAN_POINT('Ctrl Pts',(36.7549442829771,253.,20.0220033688125)) ;
#93248=CARTESIAN_POINT('Ctrl Pts',(36.7,253.,20.0220033688125)) ;
#93249=CARTESIAN_POINT('Ctrl Pts',(37.0171218972921,252.843790283354,19.9455844123125)) ;
#93250=CARTESIAN_POINT('Ctrl Pts',(36.981348581432,252.890324138772,19.9804848038695)) ;
#93251=CARTESIAN_POINT('Ctrl Pts',(36.8876373124453,252.971173206804,20.024889730955)) ;
#93252=CARTESIAN_POINT('Ctrl Pts',(36.7561776010428,253.,20.0367671642397)) ;
#93253=CARTESIAN_POINT('Ctrl Pts',(36.7,253.,20.0367671642397)) ;
#93254=CARTESIAN_POINT('',(37.0171218972921,252.843790283354,19.9455844123125)) ;
#93255=CARTESIAN_POINT('Ctrl Pts',(36.7,253.,20.0367671642397)) ;
#93256=CARTESIAN_POINT('Ctrl Pts',(36.7561776010428,253.,20.0367671642397)) ;
#93257=CARTESIAN_POINT('Ctrl Pts',(36.8876373124453,252.971173206804,20.024889730955)) ;
#93258=CARTESIAN_POINT('Ctrl Pts',(36.981348581432,252.890324138772,19.9804848038695)) ;
#93259=CARTESIAN_POINT('Ctrl Pts',(37.0171218972921,252.843790283354,19.9455844123125)) ;
#93260=CARTESIAN_POINT('Origin',(36.9378414229691,252.782842712516,19.9455844123125)) ;
#93261=CARTESIAN_POINT('Ctrl Pts',(36.9378414229691,252.853553390627,19.874873734187)) ;
#93262=CARTESIAN_POINT('Ctrl Pts',(36.911011436074,252.882637050264,19.9039573938178)) ;
#93263=CARTESIAN_POINT('Ctrl Pts',(36.840727984334,252.933167717784,19.9409614997224)) ;
#93264=CARTESIAN_POINT('Ctrl Pts',(36.7421332007821,252.951184463531,19.950859360793)) ;
#93265=CARTESIAN_POINT('Ctrl Pts',(36.7,252.951184463531,19.950859360793)) ;
#93266=CARTESIAN_POINT('Ctrl Pts',(36.9998200091722,252.670367473296,19.6916880667961)) ;
#93267=CARTESIAN_POINT('Ctrl Pts',(36.9999159399687,252.736117568423,19.7574370653151)) ;
#93268=CARTESIAN_POINT('Ctrl Pts',(36.9776401732752,252.801696685177,19.8230175376218)) ;
#93269=CARTESIAN_POINT('Ctrl Pts',(36.9375191416343,252.853781762386,19.8751022254155)) ;
#93270=CARTESIAN_POINT('Ctrl Pts',(37.0298169000146,252.670391495515,19.6916295805073)) ;
#93271=CARTESIAN_POINT('Ctrl Pts',(37.0268919560317,252.739349677716,19.7607787625668)) ;
#93272=CARTESIAN_POINT('Ctrl Pts',(37.0007398280733,252.807355530054,19.8285659598508)) ;
#93273=CARTESIAN_POINT('Ctrl Pts',(36.9563655392695,252.861063204323,19.8823434903145)) ;
#93274=CARTESIAN_POINT('Ctrl Pts',(37.0817165932468,252.652572590665,19.7093892999944)) ;
#93275=CARTESIAN_POINT('Ctrl Pts',(37.0739808431665,252.731036398121,19.7803808398083)) ;
#93276=CARTESIAN_POINT('Ctrl Pts',(37.0409357819462,252.806033248649,19.849387826736)) ;
#93277=CARTESIAN_POINT('Ctrl Pts',(36.9892344284572,252.864902508585,19.9038322607699)) ;
#93278=CARTESIAN_POINT('Ctrl Pts',(37.1000180638842,252.615417852384,19.7465229726421)) ;
#93279=CARTESIAN_POINT('Ctrl Pts',(37.096605855361,252.701582066559,19.8138465043679)) ;
#93280=CARTESIAN_POINT('Ctrl Pts',(37.0646566462868,252.785704020095,19.8804686883588)) ;
#93281=CARTESIAN_POINT('Ctrl Pts',(37.0107543184878,252.852053985775,19.9332636322344)) ;
#93282=CARTESIAN_POINT('Ctrl Pts',(37.0999997292783,252.599542422491,19.7623985166648)) ;
#93283=CARTESIAN_POINT('Ctrl Pts',(37.1001034998132,252.687234889187,19.8281678666871)) ;
#93284=CARTESIAN_POINT('Ctrl Pts',(37.0703714983291,252.77469313003,19.8937615473193)) ;
#93285=CARTESIAN_POINT('Ctrl Pts',(37.0168428003015,252.844152887956,19.9458563657635)) ;
#93286=CARTESIAN_POINT('Origin',(36.7,252.6,19.7627416997969)) ;
#93287=CARTESIAN_POINT('Origin',(34.8,258.9,20.0213203435596)) ;
#93288=CARTESIAN_POINT('',(34.7,258.9,25.7213203435596)) ;
#93289=CARTESIAN_POINT('',(34.8,259.,25.7213203435596)) ;
#93290=CARTESIAN_POINT('Origin',(34.8,258.9,25.7213203435596)) ;
#93291=CARTESIAN_POINT('',(34.7,258.9,20.0213203435596)) ;
#93292=CARTESIAN_POINT('',(34.8,259.,20.0213203435596)) ;
#93293=CARTESIAN_POINT('Origin',(52.2356360608974,253.207106781187,19.5213203435596)) ;
#93294=CARTESIAN_POINT('',(26.4,253.207106781187,20.0213203435596)) ;
#93295=CARTESIAN_POINT('Origin',(26.4,253.207106781187,19.5213203435596)) ;
#93296=CARTESIAN_POINT('',(52.2356360608974,253.207106781187,20.0213203435596)) ;
#93297=CARTESIAN_POINT('Origin',(52.2356360608974,253.207106781187,19.5213203435596)) ;
#93298=CARTESIAN_POINT('',(47.2699693783484,253.207106781187,20.0213203435596)) ;
#93299=CARTESIAN_POINT('',(52.2356360608974,253.207106781187,20.0213203435596)) ;
#93300=CARTESIAN_POINT('Ctrl Pts',(47.7791083033805,252.853553390593,19.8748737341529)) ;
#93301=CARTESIAN_POINT('Ctrl Pts',(47.6146576398327,252.947314708832,19.968635052392)) ;
#93302=CARTESIAN_POINT('Ctrl Pts',(47.4272201631483,253.072342459309,20.0213203435596)) ;
#93303=CARTESIAN_POINT('Ctrl Pts',(47.2699693783484,253.207106781187,20.0213203435596)) ;
#93304=CARTESIAN_POINT('Origin',(43.7,252.6,24.7713203435596)) ;
#93305=CARTESIAN_POINT('',(43.3,252.6,25.7213203435596)) ;
#93306=CARTESIAN_POINT('',(43.3,252.6,24.7713203435596)) ;
#93307=CARTESIAN_POINT('',(43.7,253.,25.7213203435596)) ;
#93308=CARTESIAN_POINT('Origin',(43.7,252.6,25.7213203435596)) ;
#93309=CARTESIAN_POINT('',(43.7,253.,24.7713203435596)) ;
#93310=CARTESIAN_POINT('Origin',(43.1,252.1,29.5213203435596)) ;
#93311=CARTESIAN_POINT('',(43.1,251.9,29.5213203435596)) ;
#93312=CARTESIAN_POINT('',(43.3,252.1,29.5213203435596)) ;
#93313=CARTESIAN_POINT('Origin',(37.3,251.9,29.5213203435596)) ;
#93314=CARTESIAN_POINT('',(37.3,251.9,29.5213203435596)) ;
#93315=CARTESIAN_POINT('Origin',(37.3,252.1,29.5213203435596)) ;
#93316=CARTESIAN_POINT('',(37.1,252.1,29.5213203435596)) ;
#93317=CARTESIAN_POINT('Origin',(36.7,252.6,24.7713203435596)) ;
#93318=CARTESIAN_POINT('',(36.7,253.,25.7213203435596)) ;
#93319=CARTESIAN_POINT('',(36.7,253.,24.7713203435596)) ;
#93320=CARTESIAN_POINT('',(37.1,252.6,25.7213203435596)) ;
#93321=CARTESIAN_POINT('Origin',(36.7,252.6,25.7213203435596)) ;
#93322=CARTESIAN_POINT('',(37.1,252.6,24.7713203435596)) ;
#93323=CARTESIAN_POINT('Origin',(43.3,252.1,29.5213203435596)) ;
#93324=CARTESIAN_POINT('',(43.3,259.9,29.5213203435596)) ;
#93325=CARTESIAN_POINT('',(43.3,259.4,25.7213203435596)) ;
#93326=CARTESIAN_POINT('',(43.3,259.4,24.7713203435596)) ;
#93327=CARTESIAN_POINT('',(43.3,254.05,25.7213203435596)) ;
#93328=CARTESIAN_POINT('Origin',(43.3,253.,20.0213203435596)) ;
#93329=CARTESIAN_POINT('',(45.7,253.,25.7213203435596)) ;
#93330=CARTESIAN_POINT('Origin',(37.1,259.9,29.5213203435596)) ;
#93331=CARTESIAN_POINT('',(37.1,259.4,25.7213203435596)) ;
#93332=CARTESIAN_POINT('',(37.1,257.95,25.7213203435596)) ;
#93333=CARTESIAN_POINT('',(37.1,259.4,24.7713203435596)) ;
#93334=CARTESIAN_POINT('',(37.1,259.9,29.5213203435596)) ;
#93335=CARTESIAN_POINT('Origin',(34.7,259.,20.0213203435596)) ;
#93336=CARTESIAN_POINT('',(34.7,253.,25.7213203435596)) ;
#93337=CARTESIAN_POINT('Origin',(35.9,256.,25.7213203435596)) ;
#93338=CARTESIAN_POINT('',(36.7,259.,25.7213203435596)) ;
#93339=CARTESIAN_POINT('',(34.7,259.,25.7213203435596)) ;
#93340=CARTESIAN_POINT('Origin',(36.7,259.4,25.7213203435596)) ;
#93341=CARTESIAN_POINT('Origin',(28.4,247.6,22.9713203435596)) ;
#93342=CARTESIAN_POINT('',(28.4,247.7,21.7213203435596)) ;
#93343=CARTESIAN_POINT('',(28.3,247.6,21.7213203435596)) ;
#93344=CARTESIAN_POINT('Origin',(28.4,247.6,21.7213203435596)) ;
#93345=CARTESIAN_POINT('',(28.3,247.6,26.7213203435596)) ;
#93346=CARTESIAN_POINT('',(28.3,247.6,22.9713203435596)) ;
#93347=CARTESIAN_POINT('',(28.4,247.7,26.7213203435596)) ;
#93348=CARTESIAN_POINT('Origin',(28.4,247.6,26.7213203435596)) ;
#93349=CARTESIAN_POINT('',(28.4,247.7,22.9713203435596)) ;
#93350=CARTESIAN_POINT('Origin',(28.3,246.7,24.2213203435596)) ;
#93351=CARTESIAN_POINT('',(28.3,245.8,21.7213203435596)) ;
#93352=CARTESIAN_POINT('',(28.3,245.9,21.7213203435596)) ;
#93353=CARTESIAN_POINT('',(28.3,245.8,26.7213203435596)) ;
#93354=CARTESIAN_POINT('',(28.3,245.8,25.4713203435596)) ;
#93355=CARTESIAN_POINT('',(28.3,249.25,26.7213203435596)) ;
#93356=CARTESIAN_POINT('Origin',(28.4,245.8,25.4713203435596)) ;
#93357=CARTESIAN_POINT('',(28.4,245.7,26.7213203435596)) ;
#93358=CARTESIAN_POINT('Origin',(28.4,245.8,26.7213203435596)) ;
#93359=CARTESIAN_POINT('',(28.4,245.7,21.7213203435596)) ;
#93360=CARTESIAN_POINT('Origin',(28.4,245.8,21.7213203435596)) ;
#93361=CARTESIAN_POINT('',(28.4,245.7,25.4713203435596)) ;
#93362=CARTESIAN_POINT('Origin',(26.4,251.7,26.6213203435596)) ;
#93363=CARTESIAN_POINT('',(26.3,251.7,26.8213203435596)) ;
#93364=CARTESIAN_POINT('',(26.3,251.9,26.6213203435596)) ;
#93365=CARTESIAN_POINT('Origin',(26.3,251.7,26.6213203435596)) ;
#93366=CARTESIAN_POINT('',(26.4,251.8,26.6213203435596)) ;
#93367=CARTESIAN_POINT('Origin',(26.4,251.9,26.6213203435596)) ;
#93368=CARTESIAN_POINT('',(26.4,251.7,26.7213203435596)) ;
#93369=CARTESIAN_POINT('Origin',(26.4,251.7,26.6213203435596)) ;
#93370=CARTESIAN_POINT('Origin',(26.4,251.7,26.8213203435596)) ;
#93371=CARTESIAN_POINT('Origin',(26.4,251.7,21.8213203435596)) ;
#93372=CARTESIAN_POINT('',(26.4,251.8,21.8213203435596)) ;
#93373=CARTESIAN_POINT('',(26.4,251.7,21.7213203435596)) ;
#93374=CARTESIAN_POINT('Origin',(26.4,251.7,21.8213203435596)) ;
#93375=CARTESIAN_POINT('',(26.3,251.9,21.8213203435596)) ;
#93376=CARTESIAN_POINT('Origin',(26.4,251.9,21.8213203435596)) ;
#93377=CARTESIAN_POINT('',(26.3,251.7,21.6213203435596)) ;
#93378=CARTESIAN_POINT('Origin',(26.3,251.7,21.8213203435596)) ;
#93379=CARTESIAN_POINT('Origin',(26.4,251.7,21.6213203435596)) ;
#93380=CARTESIAN_POINT('Origin',(26.4,251.9,25.6213203435596)) ;
#93381=CARTESIAN_POINT('',(26.3,251.9,25.6213203435596)) ;
#93382=CARTESIAN_POINT('',(26.4,251.8,25.6213203435596)) ;
#93383=CARTESIAN_POINT('Origin',(40.8286796564404,245.2,21.6213203435596)) ;
#93384=CARTESIAN_POINT('',(26.8,245.2,21.7213203435596)) ;
#93385=CARTESIAN_POINT('',(26.8,245.1,21.6213203435596)) ;
#93386=CARTESIAN_POINT('Origin',(26.8,245.2,21.6213203435596)) ;
#93387=CARTESIAN_POINT('',(31.8,245.1,21.6213203435596)) ;
#93388=CARTESIAN_POINT('',(40.8286796564404,245.1,21.6213203435596)) ;
#93389=CARTESIAN_POINT('',(31.8,245.2,21.7213203435596)) ;
#93390=CARTESIAN_POINT('Origin',(31.8,245.2,21.6213203435596)) ;
#93391=CARTESIAN_POINT('',(40.8286796564404,245.2,21.7213203435596)) ;
#93392=CARTESIAN_POINT('Origin',(26.8,245.6,21.6213203435596)) ;
#93393=CARTESIAN_POINT('',(26.4,245.6,21.7213203435596)) ;
#93394=CARTESIAN_POINT('',(26.3,245.6,21.6213203435596)) ;
#93395=CARTESIAN_POINT('Origin',(26.4,245.6,21.6213203435596)) ;
#93396=CARTESIAN_POINT('Origin',(26.8,245.6,21.6213203435596)) ;
#93397=CARTESIAN_POINT('Origin',(26.8,245.6,21.7213203435596)) ;
#93398=CARTESIAN_POINT('Origin',(26.4,245.35,21.6213203435596)) ;
#93399=CARTESIAN_POINT('',(26.3,245.35,21.6213203435596)) ;
#93400=CARTESIAN_POINT('',(26.4,245.35,21.7213203435596)) ;
#93401=CARTESIAN_POINT('Origin',(26.3,251.7,21.8213203435596)) ;
#93402=CARTESIAN_POINT('',(31.8,251.8,21.8213203435596)) ;
#93403=CARTESIAN_POINT('',(31.8,251.7,21.7213203435596)) ;
#93404=CARTESIAN_POINT('Origin',(31.8,251.7,21.8213203435596)) ;
#93405=CARTESIAN_POINT('',(26.3,251.8,21.8213203435596)) ;
#93406=CARTESIAN_POINT('',(26.3,251.7,21.7213203435596)) ;
#93407=CARTESIAN_POINT('Origin',(26.3,251.7,26.6213203435596)) ;
#93408=CARTESIAN_POINT('',(31.8,251.7,26.7213203435596)) ;
#93409=CARTESIAN_POINT('',(31.8,251.8,26.6213203435596)) ;
#93410=CARTESIAN_POINT('Origin',(31.8,251.7,26.6213203435596)) ;
#93411=CARTESIAN_POINT('',(26.3,251.7,26.7213203435596)) ;
#93412=CARTESIAN_POINT('',(26.3,251.8,26.6213203435596)) ;
#93413=CARTESIAN_POINT('Origin',(26.4,248.7,26.8213203435596)) ;
#93414=CARTESIAN_POINT('',(26.4,245.6,26.7213203435596)) ;
#93415=CARTESIAN_POINT('',(26.3,245.6,26.8213203435596)) ;
#93416=CARTESIAN_POINT('Origin',(26.4,245.6,26.8213203435596)) ;
#93417=CARTESIAN_POINT('',(26.3,248.7,26.8213203435596)) ;
#93418=CARTESIAN_POINT('',(26.4,248.7,26.7213203435596)) ;
#93419=CARTESIAN_POINT('Origin',(26.8,245.6,26.8213203435596)) ;
#93420=CARTESIAN_POINT('',(26.8,245.2,26.7213203435596)) ;
#93421=CARTESIAN_POINT('',(26.8,245.1,26.8213203435596)) ;
#93422=CARTESIAN_POINT('Origin',(26.8,245.2,26.8213203435596)) ;
#93423=CARTESIAN_POINT('Origin',(26.8,245.6,26.8213203435596)) ;
#93424=CARTESIAN_POINT('Origin',(26.8,245.6,26.7213203435596)) ;
#93425=CARTESIAN_POINT('Origin',(40.8286796564404,245.2,26.8213203435596)) ;
#93426=CARTESIAN_POINT('',(31.8,245.2,26.7213203435596)) ;
#93427=CARTESIAN_POINT('',(31.8,245.1,26.8213203435596)) ;
#93428=CARTESIAN_POINT('Origin',(31.8,245.2,26.8213203435596)) ;
#93429=CARTESIAN_POINT('',(40.8286796564404,245.1,26.8213203435596)) ;
#93430=CARTESIAN_POINT('',(40.8286796564404,245.2,26.7213203435596)) ;
#93431=CARTESIAN_POINT('Origin',(26.8,245.6,29.5213203435596)) ;
#93432=CARTESIAN_POINT('',(26.3,245.6,18.1213203435596)) ;
#93433=CARTESIAN_POINT('',(26.3,245.6,29.5213203435596)) ;
#93434=CARTESIAN_POINT('',(26.8,245.1,18.1213203435596)) ;
#93435=CARTESIAN_POINT('Origin',(26.8,245.6,18.1213203435596)) ;
#93436=CARTESIAN_POINT('',(26.8,245.1,29.5213203435596)) ;
#93437=CARTESIAN_POINT('Origin',(26.3,245.6,29.5213203435596)) ;
#93438=CARTESIAN_POINT('',(26.3,245.6,30.6213203435596)) ;
#93439=CARTESIAN_POINT('',(26.3,245.6,29.5213203435596)) ;
#93440=CARTESIAN_POINT('',(26.3,263.4,30.6213203435596)) ;
#93441=CARTESIAN_POINT('',(26.3,250.025,30.6213203435596)) ;
#93442=CARTESIAN_POINT('',(26.3,263.7,30.3213203435596)) ;
#93443=CARTESIAN_POINT('Origin',(26.3,263.4,30.3213203435596)) ;
#93444=CARTESIAN_POINT('',(26.3,263.7,22.5563984494954)) ;
#93445=CARTESIAN_POINT('',(26.3,263.7,29.5213203435596)) ;
#93446=CARTESIAN_POINT('',(26.3,261.872035100034,20.2714423245379)) ;
#93447=CARTESIAN_POINT('',(26.3,261.378010680031,19.6539117995346)) ;
#93448=CARTESIAN_POINT('',(26.3,261.559687576257,20.1213203435596)) ;
#93449=CARTESIAN_POINT('Origin',(26.3,261.559687576257,20.5213203435596)) ;
#93450=CARTESIAN_POINT('',(26.3,253.207106781187,20.1213203435596)) ;
#93451=CARTESIAN_POINT('',(26.3,243.158305665508,20.1213203435596)) ;
#93452=CARTESIAN_POINT('',(26.3,252.782842712475,19.9455844122715)) ;
#93453=CARTESIAN_POINT('Origin',(26.3,253.207106781187,19.5213203435596)) ;
#93454=CARTESIAN_POINT('',(26.3,251.148959235991,18.3117009357884)) ;
#93455=CARTESIAN_POINT('',(26.3,252.954289321881,20.1170310216783)) ;
#93456=CARTESIAN_POINT('',(26.3,250.68933982822,18.1213203435596)) ;
#93457=CARTESIAN_POINT('Origin',(26.3,250.68933982822,18.7713203435596)) ;
#93458=CARTESIAN_POINT('',(26.3,247.325,18.1213203435596)) ;
#93459=CARTESIAN_POINT('Origin',(26.8,245.6,29.5213203435596)) ;
#93460=CARTESIAN_POINT('',(26.8,245.1,30.6213203435596)) ;
#93461=CARTESIAN_POINT('',(26.8,245.1,29.5213203435596)) ;
#93462=CARTESIAN_POINT('Origin',(26.8,245.6,30.6213203435596)) ;
#93463=CARTESIAN_POINT('Origin',(55.3573593128808,245.1,29.5213203435596)) ;
#93464=CARTESIAN_POINT('',(38.7000000000001,245.1,19.3213203435596)) ;
#93465=CARTESIAN_POINT('',(47.7786796564403,245.1,19.3213203435596)) ;
#93466=CARTESIAN_POINT('',(38.7,245.1,20.0213203435596)) ;
#93467=CARTESIAN_POINT('',(38.7000000000001,245.1,24.3713203435596)) ;
#93468=CARTESIAN_POINT('',(33.6,245.1,20.0213203435596)) ;
#93469=CARTESIAN_POINT('',(55.3573593128808,245.1,20.0213203435596)) ;
#93470=CARTESIAN_POINT('',(33.6,245.1,30.6213203435596)) ;
#93471=CARTESIAN_POINT('',(33.6,245.1,29.5213203435596)) ;
#93472=CARTESIAN_POINT('',(42.7786796564403,245.1,30.6213203435596)) ;
#93473=CARTESIAN_POINT('',(31.8,245.1,26.8713203435596)) ;
#93474=CARTESIAN_POINT('',(55.2857703637053,245.1,18.1213203435596)) ;
#93475=CARTESIAN_POINT('Origin',(79.1,252.258305665508,20.1213203435596)) ;
#93476=CARTESIAN_POINT('',(79.1,259.648528137424,20.0213203435596)) ;
#93477=CARTESIAN_POINT('Origin',(79.1,259.648528137424,20.1213203435596)) ;
#93478=CARTESIAN_POINT('',(79.1,261.8,20.0213203435596)) ;
#93479=CARTESIAN_POINT('',(79.1,252.258305665508,20.0213203435596)) ;
#93480=CARTESIAN_POINT('Origin',(79.1,261.751937515251,20.1213203435596)) ;
#93481=CARTESIAN_POINT('Ctrl Pts',(79.199999980455,263.599938801554,22.6718380448513)) ;
#93482=CARTESIAN_POINT('Ctrl Pts',(79.2000000202887,263.599957412491,22.607806979346)) ;
#93483=CARTESIAN_POINT('Ctrl Pts',(79.2000000357465,263.570981980112,22.4453050487916)) ;
#93484=CARTESIAN_POINT('Ctrl Pts',(79.1999999617446,263.478889340347,22.2800545086636)) ;
#93485=CARTESIAN_POINT('Ctrl Pts',(79.1999999904279,263.412205761232,22.1967251384676)) ;
#93486=CARTESIAN_POINT('Ctrl Pts',(79.2000134423239,263.621049371538,22.6718434275057)) ;
#93487=CARTESIAN_POINT('Ctrl Pts',(79.1999992361883,263.620328867382,22.6051015125814)) ;
#93488=CARTESIAN_POINT('Ctrl Pts',(79.1999926902727,263.588298622545,22.438103534488)) ;
#93489=CARTESIAN_POINT('Ctrl Pts',(79.200017057909,263.492581805062,22.2711937694893)) ;
#93490=CARTESIAN_POINT('Ctrl Pts',(79.2000066111913,263.423895611839,22.1873698654484)) ;
#93491=CARTESIAN_POINT('Ctrl Pts',(79.1878716797392,263.657834283321,22.6718527795981)) ;
#93492=CARTESIAN_POINT('Ctrl Pts',(79.1887409558727,263.65586150683,22.6004009093503)) ;
#93493=CARTESIAN_POINT('Ctrl Pts',(79.1909463759846,263.618555604801,22.4255570063445)) ;
#93494=CARTESIAN_POINT('Ctrl Pts',(79.192991376968,263.516493911492,22.2557189726381)) ;
#93495=CARTESIAN_POINT('Ctrl Pts',(79.1940100432926,263.444323308611,22.1710217844746)) ;
#93496=CARTESIAN_POINT('Ctrl Pts',(79.1422513813381,263.696426316946,22.6718625902708)) ;
#93497=CARTESIAN_POINT('Ctrl Pts',(79.145958048235,263.694409856707,22.595470144496)) ;
#93498=CARTESIAN_POINT('Ctrl Pts',(79.1555689090378,263.654433984382,22.4112233680768)) ;
#93499=CARTESIAN_POINT('Ctrl Pts',(79.1650239211106,263.546732261694,22.2362869927029)) ;
#93500=CARTESIAN_POINT('Ctrl Pts',(79.1698705198354,263.470919230157,22.1497373351169)) ;
#93501=CARTESIAN_POINT('Ctrl Pts',(79.0875105354057,263.704588703717,22.6718646768523)) ;
#93502=CARTESIAN_POINT('Ctrl Pts',(79.0937026637392,263.704958374439,22.5944220758485)) ;
#93503=CARTESIAN_POINT('Ctrl Pts',(79.1102880705233,263.669990271037,22.4059549450491)) ;
#93504=CARTESIAN_POINT('Ctrl Pts',(79.1280035649932,263.563329571338,22.22586332057)) ;
#93505=CARTESIAN_POINT('Ctrl Pts',(79.1374152312722,263.486858568468,22.1369812396074)) ;
#93506=CARTESIAN_POINT('Ctrl Pts',(79.0526048408266,263.689467854776,22.6718608020123)) ;
#93507=CARTESIAN_POINT('Ctrl Pts',(79.0590423639633,263.692813185744,22.5963703264553)) ;
#93508=CARTESIAN_POINT('Ctrl Pts',(79.0771746363495,263.666059727285,22.4088436136315)) ;
#93509=CARTESIAN_POINT('Ctrl Pts',(79.0990228521318,263.564978741887,22.2251604086679)) ;
#93510=CARTESIAN_POINT('Ctrl Pts',(79.1112130439768,263.490317142384,22.1342133825315)) ;
#93511=CARTESIAN_POINT('Ctrl Pts',(79.0399427396021,263.679957003543,22.671858403052)) ;
#93512=CARTESIAN_POINT('Ctrl Pts',(79.0460881739513,263.68459203114,22.5975763648945)) ;
#93513=CARTESIAN_POINT('Ctrl Pts',(79.0639145191738,263.661746144572,22.4111497893181)) ;
#93514=CARTESIAN_POINT('Ctrl Pts',(79.0868564475194,263.563832003529,22.2260800781378)) ;
#93515=CARTESIAN_POINT('Ctrl Pts',(79.0999812750617,263.490315472764,22.1342147151094)) ;
#93516=CARTESIAN_POINT('',(79.1,263.490434404721,22.1343633494615)) ;
#93517=CARTESIAN_POINT('Origin',(79.1,263.412347523777,22.196832854217)) ;
#93518=CARTESIAN_POINT('Origin',(79.1,263.1,22.4467108732388)) ;
#93519=CARTESIAN_POINT('Origin',(79.1,264.929230192226,24.0929361897785)) ;
#93520=CARTESIAN_POINT('',(79.1,265.007317073171,24.030466685023)) ;
#93521=CARTESIAN_POINT('Origin',(79.7999999999999,259.648528137424,20.1213203435596)) ;
#93522=CARTESIAN_POINT('',(79.3050252531695,259.153553390593,20.0213203435596)) ;
#93523=CARTESIAN_POINT('Origin',(79.3050252531695,259.153553390593,20.1213203435596)) ;
#93524=CARTESIAN_POINT('Origin',(79.7999999999999,259.648528137424,20.0213203435596)) ;
#93525=CARTESIAN_POINT('Origin',(77.8915498084026,260.56702883536,20.1213203435596)) ;
#93526=CARTESIAN_POINT('',(83.7647589321277,254.693819711636,20.0213203435596)) ;
#93527=CARTESIAN_POINT('Origin',(83.7647589321277,254.693819711636,20.1213203435596)) ;
#93528=CARTESIAN_POINT('',(77.8915498084026,260.56702883536,20.0213203435596)) ;
#93529=CARTESIAN_POINT('Origin',(83.1283628290598,254.057423608568,20.1213203435596)) ;
#93530=CARTESIAN_POINT('',(84.0283628290598,254.057423608568,20.0213203435596)) ;
#93531=CARTESIAN_POINT('Origin',(84.0283628290598,254.057423608568,20.1213203435596)) ;
#93532=CARTESIAN_POINT('Origin',(83.1283628290598,254.057423608568,20.0213203435596)) ;
#93533=CARTESIAN_POINT('Origin',(84.0283628290597,247.594124250979,20.1213203435596)) ;
#93534=CARTESIAN_POINT('',(84.0283628290598,253.207106781187,20.0213203435596)) ;
#93535=CARTESIAN_POINT('Origin',(84.0283628290598,253.207106781187,20.1213203435596)) ;
#93536=CARTESIAN_POINT('',(84.0283628290597,247.594124250979,20.0213203435596)) ;
#93537=CARTESIAN_POINT('Origin',(84.0283628290598,253.207106781187,19.5213203435596)) ;
#93538=CARTESIAN_POINT('',(84.0283628290598,252.853553390593,19.8748737341529)) ;
#93539=CARTESIAN_POINT('Origin',(84.0283628290598,252.782842712475,19.9455844122716)) ;
#93540=CARTESIAN_POINT('Origin',(84.0283628290598,253.207106781187,19.5213203435596)) ;
#93541=CARTESIAN_POINT('Origin',(84.0283628290598,255.172198614617,22.3349403144135)) ;
#93542=CARTESIAN_POINT('',(84.0283628290598,251.21966991411,18.2409902576697)) ;
#93543=CARTESIAN_POINT('Origin',(84.0283628290597,251.148959235991,18.3117009357884)) ;
#93544=CARTESIAN_POINT('',(84.0283628290598,255.242909292735,22.2642296362948)) ;
#93545=CARTESIAN_POINT('Origin',(84.0283628290598,250.68933982822,18.7713203435596)) ;
#93546=CARTESIAN_POINT('',(84.0283628290598,250.68933982822,18.0213203435596)) ;
#93547=CARTESIAN_POINT('Origin',(84.0283628290598,250.68933982822,18.1213203435596)) ;
#93548=CARTESIAN_POINT('Origin',(84.0283628290598,250.68933982822,18.7713203435596)) ;
#93549=CARTESIAN_POINT('Origin',(84.0283628290598,251.76081858547,18.1213203435596)) ;
#93550=CARTESIAN_POINT('',(84.0283628290597,244.521708245126,18.0213203435596)) ;
#93551=CARTESIAN_POINT('Origin',(84.0283628290597,244.521708245126,18.1213203435596)) ;
#93552=CARTESIAN_POINT('',(84.0283628290598,251.76081858547,18.0213203435596)) ;
#93553=CARTESIAN_POINT('Origin',(84.0283628290598,244.521708245126,17.2713203435596)) ;
#93554=CARTESIAN_POINT('',(84.0283628290598,244.284537420614,17.9828328170975)) ;
#93555=CARTESIAN_POINT('Origin',(84.0283628290598,244.252914644012,18.0777011469026)) ;
#93556=CARTESIAN_POINT('Origin',(84.0283628290598,244.521708245126,17.2713203435596)) ;
#93557=CARTESIAN_POINT('Origin',(84.0283628290597,249.125613950322,19.7019342490059)) ;
#93558=CARTESIAN_POINT('',(84.0283628290596,241.115474564379,16.926478531686)) ;
#93559=CARTESIAN_POINT('Origin',(84.0283628290596,241.083851787777,17.0213468614911)) ;
#93560=CARTESIAN_POINT('',(84.0283628290597,249.157236726923,19.6070659192008)) ;
#93561=CARTESIAN_POINT('Ctrl Pts',(84.1283622645681,241.084586497772,17.0215693550394)) ;
#93562=CARTESIAN_POINT('Ctrl Pts',(84.1285407164372,240.967733802477,16.9904098877231)) ;
#93563=CARTESIAN_POINT('Ctrl Pts',(84.0861524474351,240.851280004504,16.9593566288536)) ;
#93564=CARTESIAN_POINT('Ctrl Pts',(84.0109024885665,240.761883803078,16.9355183842823)) ;
#93565=CARTESIAN_POINT('Ctrl Pts',(84.1283591396267,241.089318576984,17.0073731711595)) ;
#93566=CARTESIAN_POINT('Ctrl Pts',(84.1296466148509,240.972687875819,16.9755449829255)) ;
#93567=CARTESIAN_POINT('Ctrl Pts',(84.0885132271462,240.855600661952,16.9436904372174)) ;
#93568=CARTESIAN_POINT('Ctrl Pts',(84.0135991831494,240.765080061658,16.9191205527874)) ;
#93569=CARTESIAN_POINT('Ctrl Pts',(84.1215046355259,241.098751749129,16.9790430941334)) ;
#93570=CARTESIAN_POINT('Ctrl Pts',(84.124343019653,240.984169277709,16.9458857218838)) ;
#93571=CARTESIAN_POINT('Ctrl Pts',(84.0856125763432,240.867917187228,16.912452808833)) ;
#93572=CARTESIAN_POINT('Ctrl Pts',(84.0122486019915,240.777113726845,16.8864296181804)) ;
#93573=CARTESIAN_POINT('Ctrl Pts',(84.0879935149337,241.11202068738,16.9390868854387)) ;
#93574=CARTESIAN_POINT('Ctrl Pts',(84.0909415904953,241.005595606274,16.9049583584226)) ;
#93575=CARTESIAN_POINT('Ctrl Pts',(84.0552587945595,240.897417390581,16.8703689760042)) ;
#93576=CARTESIAN_POINT('Ctrl Pts',(83.9870257452385,240.812703535314,16.8433455584424)) ;
#93577=CARTESIAN_POINT('Ctrl Pts',(84.0506405361305,241.116115853192,16.9266350001795)) ;
#93578=CARTESIAN_POINT('Ctrl Pts',(84.0518474252873,241.017952351887,16.8938858976742)) ;
#93579=CARTESIAN_POINT('Ctrl Pts',(84.0172831579462,240.919342924437,16.8610569819731)) ;
#93580=CARTESIAN_POINT('Ctrl Pts',(83.9540867816564,240.843013317032,16.8355837036259)) ;
#93581=CARTESIAN_POINT('Ctrl Pts',(84.0281290686331,241.116068437914,16.9266767871987)) ;
#93582=CARTESIAN_POINT('Ctrl Pts',(84.0282622279932,241.022635623806,16.8955327774992)) ;
#93583=CARTESIAN_POINT('Ctrl Pts',(83.9943602020726,240.929528751412,16.8644966955634)) ;
#93584=CARTESIAN_POINT('Ctrl Pts',(83.9341920814085,240.858060634643,16.840674276805)) ;
#93585=CARTESIAN_POINT('',(83.9347806063072,240.858359520505,16.8407735170612)) ;
#93586=CARTESIAN_POINT('Origin',(83.9347806063072,240.826736743903,16.9356418468662)) ;
#93587=CARTESIAN_POINT('Origin',(83.6283628290597,241.115474564379,16.926478531686)) ;
#93588=CARTESIAN_POINT('Origin',(82.0396822566532,238.568246477383,16.1828117580263)) ;
#93589=CARTESIAN_POINT('',(82.183342912681,238.77107735692,16.1450127958665)) ;
#93590=CARTESIAN_POINT('Origin',(82.183342912681,238.739454580319,16.2398811256715)) ;
#93591=CARTESIAN_POINT('',(82.0396822566532,238.599869253985,16.0879434282213)) ;
#93592=CARTESIAN_POINT('Ctrl Pts',(82.2600174118103,238.675259362667,16.2399239332136)) ;
#93593=CARTESIAN_POINT('Ctrl Pts',(82.2259293366007,238.634587417089,16.2331463302158)) ;
#93594=CARTESIAN_POINT('Ctrl Pts',(82.1750738891123,238.608420964891,16.2287859646011)) ;
#93595=CARTESIAN_POINT('Ctrl Pts',(82.12216544278,238.604329214334,16.228104116753)) ;
#93596=CARTESIAN_POINT('Ctrl Pts',(82.2627110753973,238.678465563114,16.2235326723752)) ;
#93597=CARTESIAN_POINT('Ctrl Pts',(82.2290102704972,238.636513924476,16.2159238942483)) ;
#93598=CARTESIAN_POINT('Ctrl Pts',(82.1771259429379,238.608697992535,16.2108727836205)) ;
#93599=CARTESIAN_POINT('Ctrl Pts',(82.1226277921929,238.604359263907,16.2100849868948)) ;
#93600=CARTESIAN_POINT('Ctrl Pts',(82.2615149316266,238.689015344967,16.1948907345544)) ;
#93601=CARTESIAN_POINT('Ctrl Pts',(82.2293611646308,238.646803345078,16.1858377152017)) ;
#93602=CARTESIAN_POINT('Ctrl Pts',(82.1776767840732,238.617677482652,16.1795814374807)) ;
#93603=CARTESIAN_POINT('Ctrl Pts',(82.1227588786755,238.613157114129,16.1786097279244)) ;
#93604=CARTESIAN_POINT('Ctrl Pts',(82.2455628907713,238.713040050509,16.1629253456017)) ;
#93605=CARTESIAN_POINT('Ctrl Pts',(82.217310584656,238.675084611303,16.152902119824)) ;
#93606=CARTESIAN_POINT('Ctrl Pts',(82.1708850010324,238.648387550594,16.145860959752)) ;
#93607=CARTESIAN_POINT('Ctrl Pts',(82.1212259488329,238.644250453869,16.1447688539501)) ;
#93608=CARTESIAN_POINT('Ctrl Pts',(82.2197237261747,238.741281860249,16.1431681067147)) ;
#93609=CARTESIAN_POINT('Ctrl Pts',(82.1964342697029,238.710695018504,16.1335850929804)) ;
#93610=CARTESIAN_POINT('Ctrl Pts',(82.1586959941735,238.689424407277,16.1269372215605)) ;
#93611=CARTESIAN_POINT('Ctrl Pts',(82.1184726934836,238.686124239564,16.1259053349689)) ;
#93612=CARTESIAN_POINT('Ctrl Pts',(82.1965610315802,238.761185251271,16.1416966134236)) ;
#93613=CARTESIAN_POINT('Ctrl Pts',(82.1772535578776,238.737197314262,16.1336924132218)) ;
#93614=CARTESIAN_POINT('Ctrl Pts',(82.1473625086148,238.721189684919,16.1283631541481)) ;
#93615=CARTESIAN_POINT('Ctrl Pts',(82.1159107239231,238.718695884331,16.1275308599076)) ;
#93616=CARTESIAN_POINT('Ctrl Pts',(82.1832995175506,238.77118273482,16.1450479792177)) ;
#93617=CARTESIAN_POINT('Ctrl Pts',(82.1662696739662,238.750868029957,16.138276456763)) ;
#93618=CARTESIAN_POINT('Ctrl Pts',(82.1408684009841,238.737801298231,16.1339208359832)) ;
#93619=CARTESIAN_POINT('Ctrl Pts',(82.1144434187989,238.735757954236,16.1332397271054)) ;
#93620=CARTESIAN_POINT('',(82.1145102626716,238.735658579237,16.1332065366386)) ;
#93621=CARTESIAN_POINT('Origin',(82.1145102626716,238.704035802635,16.2280748664437)) ;
#93622=CARTESIAN_POINT('Origin',(82.106738468369,238.835356117889,16.1664390495227)) ;
#93623=CARTESIAN_POINT('Ctrl Pts',(82.1222820569742,238.604338263983,16.2280748664436)) ;
#93624=CARTESIAN_POINT('Ctrl Pts',(81.9325164757869,238.58954533045,16.2226507908148)) ;
#93625=CARTESIAN_POINT('Ctrl Pts',(81.7474165920903,238.519173200702,16.1968476765741)) ;
#93626=CARTESIAN_POINT('Ctrl Pts',(81.5957531842379,238.404160082301,16.1546761998268)) ;
#93627=CARTESIAN_POINT('Ctrl Pts',(82.1227471767039,238.604374521797,16.2100662527241)) ;
#93628=CARTESIAN_POINT('Ctrl Pts',(81.9341196170998,238.589760003749,16.2047187462123)) ;
#93629=CARTESIAN_POINT('Ctrl Pts',(81.749938274034,238.520260056156,16.1792855328002)) ;
#93630=CARTESIAN_POINT('Ctrl Pts',(81.5984884580874,238.40623436231,16.1376326562324)) ;
#93631=CARTESIAN_POINT('Ctrl Pts',(82.12287874392,238.61317412536,16.1786041604694)) ;
#93632=CARTESIAN_POINT('Ctrl Pts',(81.9345505882512,238.598690936658,16.1733895841157)) ;
#93633=CARTESIAN_POINT('Ctrl Pts',(81.7504624577361,238.529885387063,16.1486022464915)) ;
#93634=CARTESIAN_POINT('Ctrl Pts',(81.5983455559221,238.416350288722,16.1078501958846)) ;
#93635=CARTESIAN_POINT('Ctrl Pts',(82.1213346533239,238.644259546122,16.1447712536724)) ;
#93636=CARTESIAN_POINT('Ctrl Pts',(81.9292349728752,238.629499343051,16.1396437179694)) ;
#93637=CARTESIAN_POINT('Ctrl Pts',(81.7413930623854,238.559386993981,16.1152768526036)) ;
#93638=CARTESIAN_POINT('Ctrl Pts',(81.585998175509,238.443541210205,16.075123488759)) ;
#93639=CARTESIAN_POINT('Ctrl Pts',(82.1185629971472,238.686097469017,16.1259229298218)) ;
#93640=CARTESIAN_POINT('Ctrl Pts',(81.9197009618189,238.670732591567,16.1207518832949)) ;
#93641=CARTESIAN_POINT('Ctrl Pts',(81.7254002682814,238.597712993629,16.0961743956505)) ;
#93642=CARTESIAN_POINT('Ctrl Pts',(81.565153486231,238.477490209425,16.055737778703)) ;
#93643=CARTESIAN_POINT('Ctrl Pts',(82.1159855626141,238.718625782101,16.1275289375935)) ;
#93644=CARTESIAN_POINT('Ctrl Pts',(81.9108414388129,238.70267866242,16.1222138438478)) ;
#93645=CARTESIAN_POINT('Ctrl Pts',(81.7106181165948,238.626842360931,16.0969302608009)) ;
#93646=CARTESIAN_POINT('Ctrl Pts',(81.5461840821447,238.502579225023,16.0555134185675)) ;
#93647=CARTESIAN_POINT('Ctrl Pts',(82.1145102626716,238.735658579237,16.1332065366386)) ;
#93648=CARTESIAN_POINT('Ctrl Pts',(81.9057681233655,238.71938635235,16.1277824610098)) ;
#93649=CARTESIAN_POINT('Ctrl Pts',(81.7021582512993,238.641977009628,16.1019793467691)) ;
#93650=CARTESIAN_POINT('Ctrl Pts',(81.5353285026616,238.515462579386,16.0598078700218)) ;
#93651=CARTESIAN_POINT('',(81.5353285026616,238.515462579386,16.0598078700217)) ;
#93652=CARTESIAN_POINT('Origin',(81.5353285026616,238.483839802785,16.1546761998268)) ;
#93653=CARTESIAN_POINT('Origin',(82.2,237.638985654062,15.7676488949136)) ;
#93654=CARTESIAN_POINT('Ctrl Pts',(81.5957531842379,238.404160082301,16.1546761998268)) ;
#93655=CARTESIAN_POINT('Ctrl Pts',(81.5259305404763,238.351210461111,16.135261338724)) ;
#93656=CARTESIAN_POINT('Ctrl Pts',(81.4620702891285,238.288134589433,16.1213203435918)) ;
#93657=CARTESIAN_POINT('Ctrl Pts',(81.4075488173165,238.217298220807,16.1213203435596)) ;
#93658=CARTESIAN_POINT('Ctrl Pts',(81.5984884580875,238.40623436231,16.1376326562324)) ;
#93659=CARTESIAN_POINT('Ctrl Pts',(81.5278222659162,238.35302801714,16.1189375875305)) ;
#93660=CARTESIAN_POINT('Ctrl Pts',(81.462938591864,238.289258590766,16.1056627974852)) ;
#93661=CARTESIAN_POINT('Ctrl Pts',(81.4075488173195,238.217298220811,16.1063603785401)) ;
#93662=CARTESIAN_POINT('Ctrl Pts',(81.5983274323797,238.417772051001,16.1036566055189)) ;
#93663=CARTESIAN_POINT('Ctrl Pts',(81.5259047694456,238.362797284882,16.0863863691115)) ;
#93664=CARTESIAN_POINT('Ctrl Pts',(81.4591047090993,238.296564930755,16.0744149187042)) ;
#93665=CARTESIAN_POINT('Ctrl Pts',(81.4021235542092,238.22147394772,16.0764991597938)) ;
#93666=CARTESIAN_POINT('Ctrl Pts',(81.5785656655749,238.458467726493,16.0597468410921)) ;
#93667=CARTESIAN_POINT('Ctrl Pts',(81.503609725597,238.39738306884,16.0427856245866)) ;
#93668=CARTESIAN_POINT('Ctrl Pts',(81.4345131100941,238.324304784599,16.0313482653094)) ;
#93669=CARTESIAN_POINT('Ctrl Pts',(81.375611944421,238.241879454313,16.0344444600661)) ;
#93670=CARTESIAN_POINT('Ctrl Pts',(81.5516118718862,238.496137547842,16.0533661928403)) ;
#93671=CARTESIAN_POINT('Ctrl Pts',(81.4754838615336,238.430403938523,16.033529884074)) ;
#93672=CARTESIAN_POINT('Ctrl Pts',(81.405667898985,238.35229315755,16.0196569420612)) ;
#93673=CARTESIAN_POINT('Ctrl Pts',(81.346086262007,238.264604838082,16.021320343554)) ;
#93674=CARTESIAN_POINT('Ctrl Pts',(81.5353285026616,238.515462579386,16.0598078700217)) ;
#93675=CARTESIAN_POINT('Ctrl Pts',(81.4585235945239,238.448257290954,16.0374061072109)) ;
#93676=CARTESIAN_POINT('Ctrl Pts',(81.3882773180414,238.368199453823,16.0213203435967)) ;
#93677=CARTESIAN_POINT('Ctrl Pts',(81.3283036990481,238.278291755183,16.0213203435596)) ;
#93678=CARTESIAN_POINT('Origin',(81.3283036990481,238.278291755142,16.1213203435596)) ;
#93679=CARTESIAN_POINT('Ctrl Pts',(81.3283036990481,238.278291755183,16.0213203435596)) ;
#93680=CARTESIAN_POINT('Ctrl Pts',(81.3882773180414,238.368199453823,16.0213203435967)) ;
#93681=CARTESIAN_POINT('Ctrl Pts',(81.4585235945239,238.448257290954,16.0374061072109)) ;
#93682=CARTESIAN_POINT('Ctrl Pts',(81.5353285026616,238.515462579386,16.0598078700217)) ;
#93683=CARTESIAN_POINT('Origin',(82.2,237.60736287746,16.1213203435596)) ;
#93684=CARTESIAN_POINT('Origin',(81.1,237.60736287746,16.1213203435596)) ;
#93685=CARTESIAN_POINT('Origin',(81.1,234.318247777236,16.1213203435596)) ;
#93686=CARTESIAN_POINT('Origin',(81.1,226.002365511524,16.1213203435596)) ;
#93687=CARTESIAN_POINT('Origin',(80.5999999999999,226.002365511524,16.1213203435596)) ;
#93688=CARTESIAN_POINT('',(81.024264068712,225.578101442812,16.1213203435596)) ;
#93689=CARTESIAN_POINT('Origin',(80.9535533905933,225.648812120931,16.1213203435596)) ;
#93690=CARTESIAN_POINT('Origin',(80.5999999999999,226.002365511524,16.1213203435596)) ;
#93691=CARTESIAN_POINT('Origin',(79.3343678337509,224.029626564088,16.1213203435596)) ;
#93692=CARTESIAN_POINT('',(80.1757359312881,224.729573305388,16.1213203435596)) ;
#93693=CARTESIAN_POINT('Origin',(80.1050252531694,224.800283983507,16.1213203435596)) ;
#93694=CARTESIAN_POINT('',(79.4050785118696,223.95891588597,16.1213203435596)) ;
#93695=CARTESIAN_POINT('Origin',(80.6000000000002,224.305309236676,16.1213203435596)) ;
#93696=CARTESIAN_POINT('',(80.1316251501201,224.680309236676,16.1213203435596)) ;
#93697=CARTESIAN_POINT('Origin',(80.0535626751402,224.742809236676,16.1213203435596)) ;
#93698=CARTESIAN_POINT('Origin',(80.6000000000002,224.305309236676,16.1213203435596)) ;
#93699=CARTESIAN_POINT('Origin',(79.3510004003203,225.305309236676,16.1213203435596)) ;
#93700=CARTESIAN_POINT('',(79.3510004003203,224.305309236676,16.1213203435596)) ;
#93701=CARTESIAN_POINT('Origin',(79.3510004003203,224.405309236676,16.1213203435596)) ;
#93702=CARTESIAN_POINT('Origin',(79.3510004003203,225.305309236676,16.1213203435596)) ;
#93703=CARTESIAN_POINT('Origin',(75.046430535485,224.405309236676,16.1213203435596)) ;
#93704=CARTESIAN_POINT('Origin',(75.,224.405309236676,16.1213203435596)) ;
#93705=CARTESIAN_POINT('',(75.046430535485,224.305309236676,16.1213203435596)) ;
#93706=CARTESIAN_POINT('Origin',(74.9999999999998,220.305309236676,16.1213203435596)) ;
#93707=CARTESIAN_POINT('Origin',(70.8999999999999,220.305309236676,16.1213203435596)) ;
#93708=CARTESIAN_POINT('Origin',(70.9000000000001,225.16903572493,16.1213203435596)) ;
#93709=CARTESIAN_POINT('Origin',(70.8999999999998,217.165524426368,16.1213203435596)) ;
#93710=CARTESIAN_POINT('Origin',(69.4999999999997,217.165524426368,16.1213203435596)) ;
#93711=CARTESIAN_POINT('Origin',(69.4999999999997,217.165524426368,16.1213203435596)) ;
#93712=CARTESIAN_POINT('Origin',(69.4013544815242,215.668771587158,25.0213203435596)) ;
#93713=CARTESIAN_POINT('',(69.4013544815242,215.668771587158,23.2713203435596)) ;
#93714=CARTESIAN_POINT('',(69.4013544815242,215.668771587158,25.0213203435596)) ;
#93715=CARTESIAN_POINT('',(67.3755510624416,215.802284899022,23.2713203435596)) ;
#93716=CARTESIAN_POINT('Origin',(69.4999999999997,217.165524426368,25.0213203435596)) ;
#93717=CARTESIAN_POINT('Origin',(69.4999999999997,217.165524426368,23.2713203435596)) ;
#93718=CARTESIAN_POINT('Origin',(80.,224.305309236676,29.5213203435596)) ;
#93719=CARTESIAN_POINT('',(79.3510004003203,224.305309236676,29.5213203435596)) ;
#93720=CARTESIAN_POINT('Origin',(79.3510004003203,225.305309236676,29.5213203435596)) ;
#93721=CARTESIAN_POINT('',(80.1316251501201,224.680309236676,29.5213203435596)) ;
#93722=CARTESIAN_POINT('Origin',(80.6000000000002,224.305309236676,29.5213203435596)) ;
#93723=CARTESIAN_POINT('',(80.1757359312881,224.729573305388,29.5213203435596)) ;
#93724=CARTESIAN_POINT('Origin',(81.024264068712,225.578101442812,29.5213203435596)) ;
#93725=CARTESIAN_POINT('',(81.024264068712,225.578101442812,29.5213203435596)) ;
#93726=CARTESIAN_POINT('Origin',(80.5999999999999,226.002365511524,29.5213203435596)) ;
#93727=CARTESIAN_POINT('Origin',(55.2857703637053,245.2,18.1213203435596)) ;
#93728=CARTESIAN_POINT('',(26.8,245.2,18.0213203435596)) ;
#93729=CARTESIAN_POINT('Origin',(26.8,245.2,18.1213203435596)) ;
#93730=CARTESIAN_POINT('',(55.2857703637053,245.2,18.0213203435596)) ;
#93731=CARTESIAN_POINT('Origin',(47.7786796564403,245.2,19.3213203435596)) ;
#93732=CARTESIAN_POINT('Origin',(38.8,245.2,19.3213203435596)) ;
#93733=CARTESIAN_POINT('Origin',(41.6,246.4,19.3213203435596)) ;
#93734=CARTESIAN_POINT('',(41.7000000000001,242.9,19.3213203435596)) ;
#93735=CARTESIAN_POINT('',(41.7,246.4,19.3213203435596)) ;
#93736=CARTESIAN_POINT('Origin',(41.6000000000001,242.9,19.3213203435596)) ;
#93737=CARTESIAN_POINT('Origin',(40.2,242.9,19.3213203435596)) ;
#93738=CARTESIAN_POINT('',(38.7000000000001,242.9,19.3213203435596)) ;
#93739=CARTESIAN_POINT('Origin',(38.8,242.9,19.3213203435596)) ;
#93740=CARTESIAN_POINT('Origin',(40.2,242.9,19.3213203435596)) ;
#93741=CARTESIAN_POINT('Origin',(38.8,247.5,19.3213203435596)) ;
#93742=CARTESIAN_POINT('',(38.7,247.5,19.3213203435596)) ;
#93743=CARTESIAN_POINT('Origin',(26.8,245.6,18.1213203435596)) ;
#93744=CARTESIAN_POINT('',(26.4,245.6,18.0213203435596)) ;
#93745=CARTESIAN_POINT('Origin',(26.4,245.6,18.1213203435596)) ;
#93746=CARTESIAN_POINT('Origin',(26.8,245.6,18.0213203435596)) ;
#93747=CARTESIAN_POINT('Origin',(26.4,247.325,18.1213203435596)) ;
#93748=CARTESIAN_POINT('',(26.4,250.68933982822,18.0213203435596)) ;
#93749=CARTESIAN_POINT('Origin',(26.4,250.68933982822,18.1213203435596)) ;
#93750=CARTESIAN_POINT('',(26.4,247.325,18.0213203435596)) ;
#93751=CARTESIAN_POINT('Origin',(26.4,250.68933982822,18.7713203435596)) ;
#93752=CARTESIAN_POINT('Origin',(26.4,251.148959235991,18.3117009357884)) ;
#93753=CARTESIAN_POINT('Origin',(26.4,250.68933982822,18.7713203435596)) ;
#93754=CARTESIAN_POINT('Origin',(26.4,252.954289321881,20.1170310216783)) ;
#93755=CARTESIAN_POINT('Origin',(26.4,252.782842712475,19.9455844122715)) ;
#93756=CARTESIAN_POINT('Origin',(26.4,253.207106781187,19.5213203435596)) ;
#93757=CARTESIAN_POINT('Origin',(26.4,253.207106781187,20.1213203435596)) ;
#93758=CARTESIAN_POINT('Origin',(26.4,243.158305665508,20.1213203435596)) ;
#93759=CARTESIAN_POINT('',(26.4,261.559687576257,20.0213203435596)) ;
#93760=CARTESIAN_POINT('Origin',(26.4,261.559687576257,20.1213203435596)) ;
#93761=CARTESIAN_POINT('',(26.4,243.158305665508,20.0213203435596)) ;
#93762=CARTESIAN_POINT('Origin',(26.4,261.559687576257,20.5213203435596)) ;
#93763=CARTESIAN_POINT('',(26.4,261.950121980978,20.2089728197824)) ;
#93764=CARTESIAN_POINT('Origin',(26.4,261.872035100034,20.2714423245379)) ;
#93765=CARTESIAN_POINT('Origin',(26.4,261.559687576257,20.5213203435596)) ;
#93766=CARTESIAN_POINT('Origin',(26.4,261.378010680031,19.6539117995346)) ;
#93767=CARTESIAN_POINT('',(26.4,263.8,22.5213203435596)) ;
#93768=CARTESIAN_POINT('',(26.4,261.456097560976,19.5914422947791)) ;
#93769=CARTESIAN_POINT('Origin',(26.4,263.7,22.5563984494954)) ;
#93770=CARTESIAN_POINT('Origin',(34.,251.675,30.6213203435596)) ;
#93771=CARTESIAN_POINT('',(34.1,248.9,30.6213203435596)) ;
#93772=CARTESIAN_POINT('',(34.,248.9,30.7213203435596)) ;
#93773=CARTESIAN_POINT('Origin',(34.,248.9,30.6213203435596)) ;
#93774=CARTESIAN_POINT('',(34.,245.6,30.7213203435596)) ;
#93775=CARTESIAN_POINT('',(34.,251.675,30.7213203435596)) ;
#93776=CARTESIAN_POINT('',(34.1,245.6,30.6213203435596)) ;
#93777=CARTESIAN_POINT('Origin',(34.,245.6,30.6213203435596)) ;
#93778=CARTESIAN_POINT('',(34.1,251.675,30.6213203435596)) ;
#93779=CARTESIAN_POINT('Origin',(33.6,245.6,30.6213203435596)) ;
#93780=CARTESIAN_POINT('',(33.6,245.2,30.7213203435596)) ;
#93781=CARTESIAN_POINT('Origin',(33.6,245.2,30.6213203435596)) ;
#93782=CARTESIAN_POINT('Origin',(33.6,245.6,30.6213203435596)) ;
#93783=CARTESIAN_POINT('Origin',(33.6,245.6,30.7213203435596)) ;
#93784=CARTESIAN_POINT('Origin',(42.7786796564403,245.2,30.6213203435596)) ;
#93785=CARTESIAN_POINT('',(26.8,245.2,30.7213203435596)) ;
#93786=CARTESIAN_POINT('Origin',(26.8,245.2,30.6213203435596)) ;
#93787=CARTESIAN_POINT('',(42.7786796564403,245.2,30.7213203435596)) ;
#93788=CARTESIAN_POINT('Origin',(26.8,245.6,30.6213203435596)) ;
#93789=CARTESIAN_POINT('',(26.4,245.6,30.7213203435596)) ;
#93790=CARTESIAN_POINT('Origin',(26.4,245.6,30.6213203435596)) ;
#93791=CARTESIAN_POINT('Origin',(26.8,245.6,30.7213203435596)) ;
#93792=CARTESIAN_POINT('Origin',(26.4,250.025,30.6213203435596)) ;
#93793=CARTESIAN_POINT('',(26.4,263.4,30.7213203435596)) ;
#93794=CARTESIAN_POINT('Origin',(26.4,263.4,30.6213203435596)) ;
#93795=CARTESIAN_POINT('',(26.4,250.025,30.7213203435596)) ;
#93796=CARTESIAN_POINT('Origin',(26.4,263.4,30.3213203435596)) ;
#93797=CARTESIAN_POINT('',(26.4,263.8,30.3213203435596)) ;
#93798=CARTESIAN_POINT('Origin',(26.4,263.7,30.3213203435596)) ;
#93799=CARTESIAN_POINT('Origin',(26.4,263.4,30.3213203435596)) ;
#93800=CARTESIAN_POINT('Origin',(26.4,263.7,29.5213203435596)) ;
#93801=CARTESIAN_POINT('',(26.4,263.8,29.5213203435596)) ;
#93802=CARTESIAN_POINT('Origin',(45.7,244.9,18.0213203435596)) ;
#93803=CARTESIAN_POINT('Origin',(55.2141814145299,249.05,18.0213203435596)) ;
#93804=CARTESIAN_POINT('',(52.2356360608974,250.68933982822,18.0213203435596)) ;
#93805=CARTESIAN_POINT('Origin',(52.2356360608974,250.68933982822,18.7713203435596)) ;
#93806=CARTESIAN_POINT('Origin',(55.2141814145299,240.716611331017,20.0213203435596)) ;
#93807=CARTESIAN_POINT('',(46.6263598493593,261.559687576257,20.0213203435596)) ;
#93808=CARTESIAN_POINT('',(47.9856360608974,261.559687576257,20.0213203435596)) ;
#93809=CARTESIAN_POINT('',(46.6350889359327,261.466666666667,20.0213203435596)) ;
#93810=CARTESIAN_POINT('Origin',(46.1350889359327,261.466666666667,20.0213203435596)) ;
#93811=CARTESIAN_POINT('',(46.6350889359327,257.,20.0213203435596)) ;
#93812=CARTESIAN_POINT('',(46.6350889359327,252.258305665508,20.0213203435596)) ;
#93813=CARTESIAN_POINT('',(46.65,256.631336165532,20.0213203435596)) ;
#93814=CARTESIAN_POINT('Origin',(51.2,257.,20.0213203435596)) ;
#93815=CARTESIAN_POINT('',(46.65,255.5,20.0213203435596)) ;
#93816=CARTESIAN_POINT('',(46.65,248.108305665508,20.0213203435596)) ;
#93817=CARTESIAN_POINT('Origin',(51.2,255.5,20.0213203435596)) ;
#93818=CARTESIAN_POINT('',(30.7743961481358,257.164166814187,20.0213203435596)) ;
#93819=CARTESIAN_POINT('',(31.705490254513,258.090883136929,20.0213203435593)) ;
#93820=CARTESIAN_POINT('Ctrl Pts',(30.7743961481358,257.164166814187,20.0213203435596)) ;
#93821=CARTESIAN_POINT('Ctrl Pts',(30.8077000968365,257.162767488612,20.0213203435596)) ;
#93822=CARTESIAN_POINT('Ctrl Pts',(30.8410040455373,257.161368163036,20.0213203435596)) ;
#93823=CARTESIAN_POINT('Ctrl Pts',(30.9447220946478,257.157010261813,20.0213203435596)) ;
#93824=CARTESIAN_POINT('Ctrl Pts',(31.0509353958286,257.157783514541,20.0213203435571)) ;
#93825=CARTESIAN_POINT('Ctrl Pts',(31.1897565474607,257.182733549511,20.021320343557)) ;
#93826=CARTESIAN_POINT('Ctrl Pts',(31.2571806346872,257.213759459052,20.0213203435567)) ;
#93827=CARTESIAN_POINT('Ctrl Pts',(31.2858437484895,257.241279724063,20.0213203435566)) ;
#93828=CARTESIAN_POINT('Ctrl Pts',(31.2981495994694,257.253889722425,20.0213203435566)) ;
#93829=CARTESIAN_POINT('Ctrl Pts',(31.318498748845,257.279979678226,20.0213203435566)) ;
#93830=CARTESIAN_POINT('Ctrl Pts',(31.352487915175,257.336561723898,20.0213203435566)) ;
#93831=CARTESIAN_POINT('Ctrl Pts',(31.3833769551383,257.400055955828,20.0213203435566)) ;
#93832=CARTESIAN_POINT('Ctrl Pts',(31.4095784978925,257.455988292376,20.0213203435565)) ;
#93833=CARTESIAN_POINT('Ctrl Pts',(31.4215689681375,257.482038502719,20.0213203435565)) ;
#93834=CARTESIAN_POINT('Ctrl Pts',(31.4271002177055,257.494057204395,20.0213203435565)) ;
#93835=CARTESIAN_POINT('Ctrl Pts',(31.4298611935316,257.500068246514,20.0213203435565)) ;
#93836=CARTESIAN_POINT('Ctrl Pts',(31.4326210851137,257.506079046589,20.0213203435565)) ;
#93837=CARTESIAN_POINT('Ctrl Pts',(31.449163234782,257.542143350465,20.0213203435565)) ;
#93838=CARTESIAN_POINT('Ctrl Pts',(31.4940316374113,257.640298396679,20.0213203435568)) ;
#93839=CARTESIAN_POINT('Ctrl Pts',(31.567631288081,257.79951081352,20.0213203435576)) ;
#93840=CARTESIAN_POINT('Ctrl Pts',(31.6435315049203,257.960632026113,20.0213203435577)) ;
#93841=CARTESIAN_POINT('Ctrl Pts',(31.6896407086131,258.057612082693,20.0213203435588)) ;
#93842=CARTESIAN_POINT('Ctrl Pts',(31.7054902513284,258.090883129822,20.0213203435591)) ;
#93843=CARTESIAN_POINT('',(30.7492082877751,256.564695737578,20.0213203435596)) ;
#93844=CARTESIAN_POINT('',(30.4489043471128,249.417461949796,20.0213203435596)) ;
#93845=CARTESIAN_POINT('',(32.2494311094147,257.837238667481,20.0213203435596)) ;
#93846=CARTESIAN_POINT('Ctrl Pts',(32.2494305846701,257.837237537136,20.0213203435596)) ;
#93847=CARTESIAN_POINT('Ctrl Pts',(32.2079598075039,257.749584797189,20.0213203435596)) ;
#93848=CARTESIAN_POINT('Ctrl Pts',(32.1338192164731,257.591081166943,20.0213203435596)) ;
#93849=CARTESIAN_POINT('Ctrl Pts',(32.0151173093266,257.33883287554,20.0213203435596)) ;
#93850=CARTESIAN_POINT('Ctrl Pts',(31.9025505811396,257.076333688533,20.0213203435596)) ;
#93851=CARTESIAN_POINT('Ctrl Pts',(31.735897005124,256.808363024752,20.0213203435596)) ;
#93852=CARTESIAN_POINT('Ctrl Pts',(31.3799595822748,256.57233432435,20.0213203435596)) ;
#93853=CARTESIAN_POINT('Ctrl Pts',(31.0569053558616,256.55176728934,20.0213203435596)) ;
#93854=CARTESIAN_POINT('Ctrl Pts',(30.8158161851762,256.561897086427,20.0213203435597)) ;
#93855=CARTESIAN_POINT('Ctrl Pts',(30.7825122364757,256.563296412003,20.0213203435596)) ;
#93856=CARTESIAN_POINT('Ctrl Pts',(30.7492082877751,256.564695737578,20.0213203435596)) ;
#93857=CARTESIAN_POINT('',(32.7113239146176,257.621855202687,20.0213203435596)) ;
#93858=CARTESIAN_POINT('',(44.9147880370394,251.931286426383,20.0213203435596)) ;
#93859=CARTESIAN_POINT('',(32.8217003142836,259.81920153961,20.0213203435596)) ;
#93860=CARTESIAN_POINT('',(32.319849148055,249.82847140953,20.0213203435596)) ;
#93861=CARTESIAN_POINT('',(31.2093839453833,258.32222131243,20.0213203435596)) ;
#93862=CARTESIAN_POINT('',(33.9819120129541,260.896418149051,20.0213203435596)) ;
#93863=CARTESIAN_POINT('',(44.5070901774322,252.121399060531,20.0213203435596)) ;
#93864=CARTESIAN_POINT('',(28.594347661489,253.822145724429,20.0213203435596)) ;
#93865=CARTESIAN_POINT('',(28.704724061155,256.019492061351,20.0213203435596)) ;
#93866=CARTESIAN_POINT('',(28.3509795345864,248.977232647076,20.0213203435596)) ;
#93867=CARTESIAN_POINT('',(30.2066640303894,255.319125951608,20.0213203435596)) ;
#93868=CARTESIAN_POINT('',(32.5650931541241,257.50884617869,20.0213203435596)) ;
#93869=CARTESIAN_POINT('',(29.7113866401971,255.550077591566,20.0213203435596)) ;
#93870=CARTESIAN_POINT('',(43.2063774077619,249.25726004992,20.0213203435596)) ;
#93871=CARTESIAN_POINT('',(30.7304788580035,256.575626202204,20.0213203435596)) ;
#93872=CARTESIAN_POINT('Ctrl Pts',(30.7304788580035,256.575626202204,20.0213203435596)) ;
#93873=CARTESIAN_POINT('Ctrl Pts',(30.6975923919765,256.570186398587,20.0213203435596)) ;
#93874=CARTESIAN_POINT('Ctrl Pts',(30.6647059259495,256.564746594971,20.0213203435597)) ;
#93875=CARTESIAN_POINT('Ctrl Pts',(30.5574162678237,256.546999638827,20.0213203435596)) ;
#93876=CARTESIAN_POINT('Ctrl Pts',(30.4098121082759,256.517330456645,20.0213203435596)) ;
#93877=CARTESIAN_POINT('Ctrl Pts',(30.2468536416027,256.46621770294,20.0213203435596)) ;
#93878=CARTESIAN_POINT('Ctrl Pts',(30.1477680849333,256.411315348599,20.0213203435596)) ;
#93879=CARTESIAN_POINT('Ctrl Pts',(30.102845715951,256.376170629923,20.0213203435596)) ;
#93880=CARTESIAN_POINT('Ctrl Pts',(30.0697165858412,256.329790150052,20.0213203435596)) ;
#93881=CARTESIAN_POINT('Ctrl Pts',(30.0443195024724,256.279163360013,20.0213203435596)) ;
#93882=CARTESIAN_POINT('Ctrl Pts',(30.0210609313549,256.227379414746,20.0213203435596)) ;
#93883=CARTESIAN_POINT('Ctrl Pts',(29.9917240307883,256.158322827055,20.0213203435596)) ;
#93884=CARTESIAN_POINT('Ctrl Pts',(29.9116103717487,255.966894765232,20.0213203435596)) ;
#93885=CARTESIAN_POINT('Ctrl Pts',(29.8150167827562,255.758802051448,20.0213203435596)) ;
#93886=CARTESIAN_POINT('Ctrl Pts',(29.7297455839443,255.586884322961,20.0213203435596)) ;
#93887=CARTESIAN_POINT('Ctrl Pts',(29.7113866401971,255.550077591566,20.0213203435596)) ;
#93888=CARTESIAN_POINT('',(30.6325623929048,257.167582590684,20.0213203435596)) ;
#93889=CARTESIAN_POINT('',(32.3250488694829,246.935614134431,20.0213203435596)) ;
#93890=CARTESIAN_POINT('',(29.1672125989201,255.803831327378,20.0213203435596)) ;
#93891=CARTESIAN_POINT('Ctrl Pts',(29.1672135287853,255.803833319767,20.0213203435596)) ;
#93892=CARTESIAN_POINT('Ctrl Pts',(29.2098526575051,255.890075605729,20.0213203435596)) ;
#93893=CARTESIAN_POINT('Ctrl Pts',(29.2855162725872,256.046162959787,20.0213203435596)) ;
#93894=CARTESIAN_POINT('Ctrl Pts',(29.4018690227886,256.296948740307,20.0213203435596)) ;
#93895=CARTESIAN_POINT('Ctrl Pts',(29.5002329804407,256.562256782507,20.0213203435596)) ;
#93896=CARTESIAN_POINT('Ctrl Pts',(29.6710833447946,256.82479414277,20.0213203435596)) ;
#93897=CARTESIAN_POINT('Ctrl Pts',(30.0246139021395,257.050386605117,20.0213203435596)) ;
#93898=CARTESIAN_POINT('Ctrl Pts',(30.3309225628221,257.117687857779,20.0213203435596)) ;
#93899=CARTESIAN_POINT('Ctrl Pts',(30.5667894608518,257.156702983451,20.0213203435597)) ;
#93900=CARTESIAN_POINT('Ctrl Pts',(30.5996759268789,257.162142787068,20.0213203435597)) ;
#93901=CARTESIAN_POINT('Ctrl Pts',(30.6325623929059,257.167582590684,20.0213203435597)) ;
#93902=CARTESIAN_POINT('',(42.7981704029692,249.447610102367,20.0213203435596)) ;
#93903=CARTESIAN_POINT('Origin',(47.9856360608974,261.559687576257,20.5213203435596)) ;
#93904=CARTESIAN_POINT('',(46.6263598493593,261.950121980978,20.2089728197824)) ;
#93905=CARTESIAN_POINT('',(47.9856360608974,261.950121980978,20.2089728197824)) ;
#93906=CARTESIAN_POINT('Origin',(46.6263598493593,261.559687576257,20.5213203435596)) ;
#93907=CARTESIAN_POINT('Origin',(40.757090707265,262.8,21.2713203435596)) ;
#93908=CARTESIAN_POINT('',(45.3029147394738,263.8,22.5213203435596)) ;
#93909=CARTESIAN_POINT('',(40.757090707265,263.8,22.5213203435596)) ;
#93910=CARTESIAN_POINT('',(46.5350889359327,262.157101071388,20.4676966827949)) ;
#93911=CARTESIAN_POINT('',(44.3686862542563,265.04563798029,24.0783678189221)) ;
#93912=CARTESIAN_POINT('Origin',(46.1350889359327,261.857101071388,20.0926966827949)) ;
#93913=CARTESIAN_POINT('Origin',(26.3,263.8,29.5213203435596)) ;
#93914=CARTESIAN_POINT('',(26.7,263.8,30.3213203435596)) ;
#93915=CARTESIAN_POINT('',(28.25,263.8,30.3213203435596)) ;
#93916=CARTESIAN_POINT('',(26.7,263.8,30.7213203435596)) ;
#93917=CARTESIAN_POINT('',(45.6350889359327,263.8,22.9467108732387)) ;
#93918=CARTESIAN_POINT('',(45.6350889359327,263.8,29.5213203435596)) ;
#93919=CARTESIAN_POINT('Origin',(45.0100889359327,263.8,23.3217108732387)) ;
#93920=CARTESIAN_POINT('',(42.2,263.8,25.0213203435596)) ;
#93921=CARTESIAN_POINT('Origin',(40.2,263.8,25.0213203435596)) ;
#93922=CARTESIAN_POINT('Origin',(28.25,263.4,30.3213203435596)) ;
#93923=CARTESIAN_POINT('',(26.7,263.4,30.7213203435596)) ;
#93924=CARTESIAN_POINT('',(28.25,263.4,30.7213203435596)) ;
#93925=CARTESIAN_POINT('Origin',(26.7,263.4,30.3213203435596)) ;
#93926=CARTESIAN_POINT('Origin',(30.2,254.45,30.7213203435596)) ;
#93927=CARTESIAN_POINT('',(33.8,248.9,30.7213203435596)) ;
#93928=CARTESIAN_POINT('',(34.2,248.9,30.7213203435596)) ;
#93929=CARTESIAN_POINT('',(33.8,245.5,30.7213203435596)) ;
#93930=CARTESIAN_POINT('',(33.8,248.9,30.7213203435596)) ;
#93931=CARTESIAN_POINT('',(26.7,245.5,30.7213203435596)) ;
#93932=CARTESIAN_POINT('',(26.7,245.5,30.7213203435596)) ;
#93933=CARTESIAN_POINT('',(26.7,263.8,30.7213203435596)) ;
#93934=CARTESIAN_POINT('Origin',(33.8,248.9,30.7213203435596)) ;
#93935=CARTESIAN_POINT('',(34.1,248.9,30.7213203435596)) ;
#93936=CARTESIAN_POINT('',(33.8,248.9,30.7213203435596)) ;
#93937=CARTESIAN_POINT('Ctrl Pts',(65.5999303613899,241.999999985716,17.293483289198)) ;
#93938=CARTESIAN_POINT('Ctrl Pts',(65.6223872883743,241.999983684684,17.293472412949)) ;
#93939=CARTESIAN_POINT('Ctrl Pts',(65.6596675749485,242.013094396161,17.3022200416641)) ;
#93940=CARTESIAN_POINT('Ctrl Pts',(65.6931551015551,242.055168995966,17.330288781682)) ;
#93941=CARTESIAN_POINT('Ctrl Pts',(65.7000053564237,242.085052656273,17.3502211438567)) ;
#93942=CARTESIAN_POINT('Ctrl Pts',(65.7000000641616,242.100035052592,17.3602131913087)) ;
#93943=CARTESIAN_POINT('Ctrl Pts',(65.5999249277793,242.000021651293,17.2696626868496)) ;
#93944=CARTESIAN_POINT('Ctrl Pts',(65.6241340213892,242.000002492859,17.2696523403355)) ;
#93945=CARTESIAN_POINT('Ctrl Pts',(65.6644103131029,242.015411876757,17.2779740038621)) ;
#93946=CARTESIAN_POINT('Ctrl Pts',(65.6970732727148,242.062602858122,17.3042522328329)) ;
#93947=CARTESIAN_POINT('Ctrl Pts',(65.7014293655986,242.09429051932,17.3226735443473)) ;
#93948=CARTESIAN_POINT('Ctrl Pts',(65.6999581864955,242.109509455678,17.331789222077)) ;
#93949=CARTESIAN_POINT('Ctrl Pts',(65.5999043794225,241.984498189437,17.2281729676822)) ;
#93950=CARTESIAN_POINT('Ctrl Pts',(65.6307400247959,241.984473403835,17.2281636615388)) ;
#93951=CARTESIAN_POINT('Ctrl Pts',(65.6817645791198,242.004408765663,17.2356486243123)) ;
#93952=CARTESIAN_POINT('Ctrl Pts',(65.7227159874069,242.065586997243,17.2589885526196)) ;
#93953=CARTESIAN_POINT('Ctrl Pts',(65.7273533452622,242.106413945834,17.2748865541599)) ;
#93954=CARTESIAN_POINT('Ctrl Pts',(65.7250852524029,242.125921449753,17.2826065722531)) ;
#93955=CARTESIAN_POINT('Ctrl Pts',(65.599873772515,241.948550664554,17.2041705651312)) ;
#93956=CARTESIAN_POINT('Ctrl Pts',(65.6405794114654,241.948520314274,17.2041604139615)) ;
#93957=CARTESIAN_POINT('Ctrl Pts',(65.7080914959693,241.97293082834,17.2123249505645)) ;
#93958=CARTESIAN_POINT('Ctrl Pts',(65.7672744641676,242.050491491113,17.2381616472598)) ;
#93959=CARTESIAN_POINT('Ctrl Pts',(65.7782470503292,242.104798334671,17.2562659833551)) ;
#93960=CARTESIAN_POINT('Ctrl Pts',(65.7775568883756,242.131748070042,17.2652363069337)) ;
#93961=CARTESIAN_POINT('Ctrl Pts',(65.5998606830298,241.931622827182,17.1985279526202)) ;
#93962=CARTESIAN_POINT('Ctrl Pts',(65.6447873550492,241.93159020424,17.1985170783063)) ;
#93963=CARTESIAN_POINT('Ctrl Pts',(65.7193698426426,241.957828422043,17.2072631509073)) ;
#93964=CARTESIAN_POINT('Ctrl Pts',(65.7863389216959,242.042015023498,17.2353253513923)) ;
#93965=CARTESIAN_POINT('Ctrl Pts',(65.8000212346729,242.101795553135,17.2552521946044)) ;
#93966=CARTESIAN_POINT('Ctrl Pts',(65.7999999505254,242.131762093447,17.2652410413751)) ;
#93967=CARTESIAN_POINT('',(65.8,242.131622776602,17.2651946024269)) ;
#93968=CARTESIAN_POINT('',(65.6,241.931622776602,17.1985279357602)) ;
#93969=CARTESIAN_POINT('Origin',(65.6,242.131622776602,17.2651946024269)) ;
#93970=CARTESIAN_POINT('',(65.6,242.,17.2933962655652)) ;
#93971=CARTESIAN_POINT('Origin',(65.6,241.9,17.2933962655652)) ;
#93972=CARTESIAN_POINT('',(65.7,242.1,17.3600629322319)) ;
#93973=CARTESIAN_POINT('Origin',(65.6,242.1,17.3600629322319)) ;
#93974=CARTESIAN_POINT('Origin',(65.8,242.1,17.3600629322319)) ;
#93975=CARTESIAN_POINT('Ctrl Pts',(59.6999999358574,242.100035047439,17.3602131692166)) ;
#93976=CARTESIAN_POINT('Ctrl Pts',(59.6999946444109,242.08505265448,17.3502211245603)) ;
#93977=CARTESIAN_POINT('Ctrl Pts',(59.706844874529,242.055168958287,17.3302887398296)) ;
#93978=CARTESIAN_POINT('Ctrl Pts',(59.7403323865735,242.013094322282,17.3022199784523)) ;
#93979=CARTESIAN_POINT('Ctrl Pts',(59.777612703929,241.999983687182,17.2934724018186)) ;
#93980=CARTESIAN_POINT('Ctrl Pts',(59.8000696283755,241.99999998572,17.2934832764019)) ;
#93981=CARTESIAN_POINT('Ctrl Pts',(59.700041807277,242.109509448604,17.3317892058711)) ;
#93982=CARTESIAN_POINT('Ctrl Pts',(59.6985706299482,242.094290514752,17.3226735305565)) ;
#93983=CARTESIAN_POINT('Ctrl Pts',(59.7029267634591,242.06260272335,17.3042521582366)) ;
#93984=CARTESIAN_POINT('Ctrl Pts',(59.7355897453586,242.015411672362,17.2779738906251)) ;
#93985=CARTESIAN_POINT('Ctrl Pts',(59.7758659698318,242.000002492707,17.2696523335273)) ;
#93986=CARTESIAN_POINT('Ctrl Pts',(59.8000750611887,242.000021648067,17.2696626783861)) ;
#93987=CARTESIAN_POINT('Ctrl Pts',(59.6749147977919,242.125921458688,17.2826065001862)) ;
#93988=CARTESIAN_POINT('Ctrl Pts',(59.6726467078424,242.106413958098,17.2748864836143)) ;
#93989=CARTESIAN_POINT('Ctrl Pts',(59.6772839773079,242.06558697052,17.2589884854408)) ;
#93990=CARTESIAN_POINT('Ctrl Pts',(59.7182353474647,242.004408673025,17.235648539643)) ;
#93991=CARTESIAN_POINT('Ctrl Pts',(59.7692599649735,241.984473432376,17.2281636368172)) ;
#93992=CARTESIAN_POINT('Ctrl Pts',(59.8000956065233,241.984498214178,17.2281729415163)) ;
#93993=CARTESIAN_POINT('Ctrl Pts',(59.6224431111526,242.131748051622,17.2652363008027)) ;
#93994=CARTESIAN_POINT('Ctrl Pts',(59.6217529522638,242.104798322373,17.2562659792971)) ;
#93995=CARTESIAN_POINT('Ctrl Pts',(59.6327254809023,242.050491431942,17.2381616006781)) ;
#93996=CARTESIAN_POINT('Ctrl Pts',(59.69190841539,241.97293070804,17.212324871922)) ;
#93997=CARTESIAN_POINT('Ctrl Pts',(59.759420576324,241.948520318883,17.2041604155507)) ;
#93998=CARTESIAN_POINT('Ctrl Pts',(59.8001262089281,241.94855066454,17.2041705651264)) ;
#93999=CARTESIAN_POINT('Ctrl Pts',(59.60000004946,242.131762072965,17.265241034548)) ;
#94000=CARTESIAN_POINT('Ctrl Pts',(59.5999787685205,242.101795539627,17.2552521901018)) ;
#94001=CARTESIAN_POINT('Ctrl Pts',(59.6136610351411,242.042014939473,17.2353253233842)) ;
#94002=CARTESIAN_POINT('Ctrl Pts',(59.6806300862088,241.957828270871,17.2072631005166)) ;
#94003=CARTESIAN_POINT('Ctrl Pts',(59.755212631428,241.931590209221,17.1985170799667)) ;
#94004=CARTESIAN_POINT('Ctrl Pts',(59.8001392964891,241.931622827167,17.1985279526151)) ;
#94005=CARTESIAN_POINT('',(59.8,241.931622776602,17.1985279357602)) ;
#94006=CARTESIAN_POINT('',(59.6,242.131622776602,17.2651946024269)) ;
#94007=CARTESIAN_POINT('Origin',(59.8,242.131622776602,17.2651946024269)) ;
#94008=CARTESIAN_POINT('',(59.7,242.1,17.3600629322319)) ;
#94009=CARTESIAN_POINT('Origin',(59.6,242.1,17.3600629322319)) ;
#94010=CARTESIAN_POINT('',(59.8,242.,17.2933962655652)) ;
#94011=CARTESIAN_POINT('Origin',(59.8,242.1,17.3600629322319)) ;
#94012=CARTESIAN_POINT('Origin',(59.8,241.9,17.2933962655652)) ;
#94013=CARTESIAN_POINT('Origin',(59.5584606379469,244.3,18.0213203435596)) ;
#94014=CARTESIAN_POINT('',(59.6446141839292,244.350769740148,18.5618897586017)) ;
#94015=CARTESIAN_POINT('',(59.6446141839292,244.350769740148,18.0213203435596)) ;
#94016=CARTESIAN_POINT('',(59.5584606379469,244.4,18.5618897586017)) ;
#94017=CARTESIAN_POINT('Origin',(59.5584606379469,244.3,18.5618897586017)) ;
#94018=CARTESIAN_POINT('',(59.5584606379469,244.4,18.0213203435596)) ;
#94019=CARTESIAN_POINT('Ctrl Pts',(59.6449792856958,244.350205175131,18.5813019044811)) ;
#94020=CARTESIAN_POINT('Ctrl Pts',(59.6430156590439,244.353094663765,18.5096043208207)) ;
#94021=CARTESIAN_POINT('Ctrl Pts',(59.6643726514291,244.322762794723,18.3446198236948)) ;
#94022=CARTESIAN_POINT('Ctrl Pts',(59.7030495510182,244.213584940611,18.1990771050326)) ;
#94023=CARTESIAN_POINT('Ctrl Pts',(59.6996459812343,244.130500642109,18.129314888008)) ;
#94024=CARTESIAN_POINT('Ctrl Pts',(59.6349464633671,244.367348698933,18.58199169507)) ;
#94025=CARTESIAN_POINT('Ctrl Pts',(59.6329367571624,244.370044698671,18.5077410022612)) ;
#94026=CARTESIAN_POINT('Ctrl Pts',(59.6546927064743,244.341795048543,18.3370566394004)) ;
#94027=CARTESIAN_POINT('Ctrl Pts',(59.6991557712068,244.237488979578,18.1840665355433)) ;
#94028=CARTESIAN_POINT('Ctrl Pts',(59.700759507625,244.153316861886,18.1088960755437)) ;
#94029=CARTESIAN_POINT('Ctrl Pts',(59.6082389705581,244.391842293383,18.5831922626804)) ;
#94030=CARTESIAN_POINT('Ctrl Pts',(59.6063337160284,244.394263327123,18.5045025279965)) ;
#94031=CARTESIAN_POINT('Ctrl Pts',(59.6269047402143,244.368914661875,18.3237861932478)) ;
#94032=CARTESIAN_POINT('Ctrl Pts',(59.6716432201894,244.274302161456,18.1578059752604)) ;
#94033=CARTESIAN_POINT('Ctrl Pts',(59.6762070658786,244.193893615517,18.0736395593349)) ;
#94034=CARTESIAN_POINT('Ctrl Pts',(59.5735081239853,244.399670610509,18.5840368704358)) ;
#94035=CARTESIAN_POINT('Ctrl Pts',(59.5719051030305,244.402105264329,18.5022319176753)) ;
#94036=CARTESIAN_POINT('Ctrl Pts',(59.5892945812339,244.37657507066,18.3141889457068)) ;
#94037=CARTESIAN_POINT('Ctrl Pts',(59.6230383416314,244.283288012232,18.1450930356084)) ;
#94038=CARTESIAN_POINT('Ctrl Pts',(59.6226269787515,244.20916290406,18.0620326887834)) ;
#94039=CARTESIAN_POINT('Ctrl Pts',(59.5586579020403,244.399662026347,18.5842964723602)) ;
#94040=CARTESIAN_POINT('Ctrl Pts',(59.5571848337607,244.402160845737,18.501538570537)) ;
#94041=CARTESIAN_POINT('Ctrl Pts',(59.5732055894127,244.375930402281,18.3111050418282)) ;
#94042=CARTESIAN_POINT('Ctrl Pts',(59.6022571961834,244.281492408201,18.1430838566138)) ;
#94043=CARTESIAN_POINT('Ctrl Pts',(59.5997425774969,244.209583069344,18.062525619286)) ;
#94044=CARTESIAN_POINT('',(59.7,244.147690779557,18.1437942097801)) ;
#94045=CARTESIAN_POINT('',(59.6,244.224258591796,18.0794718176537)) ;
#94046=CARTESIAN_POINT('Origin',(59.6,244.147690779557,18.1437942097801)) ;
#94047=CARTESIAN_POINT('Ctrl Pts',(59.6,244.224258591796,18.0794718176537)) ;
#94048=CARTESIAN_POINT('Ctrl Pts',(59.6,244.288790166617,18.1562886358886)) ;
#94049=CARTESIAN_POINT('Ctrl Pts',(59.5736962854113,244.373361945941,18.311949011817)) ;
#94050=CARTESIAN_POINT('Ctrl Pts',(59.5584606379469,244.4,18.4866458512847)) ;
#94051=CARTESIAN_POINT('Ctrl Pts',(59.5584606379469,244.4,18.5618897586017)) ;
#94052=CARTESIAN_POINT('Ctrl Pts',(59.6446141839293,244.350769740148,18.5618897586017)) ;
#94053=CARTESIAN_POINT('Ctrl Pts',(59.6446141839293,244.350769740148,18.5439567476136)) ;
#94054=CARTESIAN_POINT('Ctrl Pts',(59.6452210304616,244.349749530056,18.5260482379517)) ;
#94055=CARTESIAN_POINT('Ctrl Pts',(59.6463723337907,244.347756284791,18.5082205111784)) ;
#94056=CARTESIAN_POINT('Ctrl Pts',(59.6475773410637,244.345670062176,18.4895611884093)) ;
#94057=CARTESIAN_POINT('Ctrl Pts',(59.6493785330647,244.342517330079,18.4709903607338)) ;
#94058=CARTESIAN_POINT('Ctrl Pts',(59.6516514055649,244.338324693025,18.4525725587764)) ;
#94059=CARTESIAN_POINT('Ctrl Pts',(59.6540993463895,244.333809117512,18.4327361230297)) ;
#94060=CARTESIAN_POINT('Ctrl Pts',(59.6570943867615,244.328086171057,18.4130771945381)) ;
#94061=CARTESIAN_POINT('Ctrl Pts',(59.6604228321352,244.321170986139,18.3936763934124)) ;
#94062=CARTESIAN_POINT('Ctrl Pts',(59.6617883780566,244.318333925139,18.3857169162767)) ;
#94063=CARTESIAN_POINT('Ctrl Pts',(59.663209403941,244.315296090927,18.3778008865419)) ;
#94064=CARTESIAN_POINT('Ctrl Pts',(59.6646686888534,244.312058499533,18.3699338714232)) ;
#94065=CARTESIAN_POINT('Ctrl Pts',(59.6682359483491,244.304144124111,18.3507027506552)) ;
#94066=CARTESIAN_POINT('Ctrl Pts',(59.6720043911007,244.295103438323,18.331764526822)) ;
#94067=CARTESIAN_POINT('Ctrl Pts',(59.675727045999,244.284910263978,18.3131841990656)) ;
#94068=CARTESIAN_POINT('Ctrl Pts',(59.6793120602611,244.275093969855,18.2952908563249)) ;
#94069=CARTESIAN_POINT('Ctrl Pts',(59.6828540129505,244.264207774873,18.2777294333825)) ;
#94070=CARTESIAN_POINT('Ctrl Pts',(59.6860916942254,244.252252740375,18.2605579828757)) ;
#94071=CARTESIAN_POINT('Ctrl Pts',(59.6892284705155,244.240670294304,18.2439216946671)) ;
#94072=CARTESIAN_POINT('Ctrl Pts',(59.6920789697902,244.228083726207,18.2276514500578)) ;
#94073=CARTESIAN_POINT('Ctrl Pts',(59.6943758946989,244.214531288834,18.2118000413148)) ;
#94074=CARTESIAN_POINT('Ctrl Pts',(59.6965663032281,244.201607325017,18.1966837174079)) ;
#94075=CARTESIAN_POINT('Ctrl Pts',(59.6982525026342,244.187804525414,18.1819482843279)) ;
#94076=CARTESIAN_POINT('Ctrl Pts',(59.6991857824465,244.173199818986,18.1676395251846)) ;
#94077=CARTESIAN_POINT('Ctrl Pts',(59.6997132846748,244.164945043641,18.1595520232023)) ;
#94078=CARTESIAN_POINT('Ctrl Pts',(59.7,244.156434931344,18.1516008291015)) ;
#94079=CARTESIAN_POINT('Ctrl Pts',(59.7,244.147690779557,18.1437942097801)) ;
#94080=CARTESIAN_POINT('Origin',(59.6,243.65,18.5618897586017)) ;
#94081=CARTESIAN_POINT('',(59.7,243.855548047911,17.9452456148689)) ;
#94082=CARTESIAN_POINT('',(59.6,243.887170824513,17.8503772850638)) ;
#94083=CARTESIAN_POINT('Origin',(59.6,243.855548047911,17.9452456148689)) ;
#94084=CARTESIAN_POINT('Origin',(59.6,243.65,18.5618897586017)) ;
#94085=CARTESIAN_POINT('Origin',(59.7,243.65,18.5618897586017)) ;
#94086=CARTESIAN_POINT('Origin',(59.6,242.688377223398,17.5561886733647)) ;
#94087=CARTESIAN_POINT('',(59.6,242.72,17.4613203435596)) ;
#94088=CARTESIAN_POINT('',(59.7,242.688377223398,17.5561886733647)) ;
#94089=CARTESIAN_POINT('Origin',(59.8,242.1,24.0213203435596)) ;
#94090=CARTESIAN_POINT('',(59.8,242.,24.0213203435596)) ;
#94091=CARTESIAN_POINT('',(59.7,242.1,24.0213203435596)) ;
#94092=CARTESIAN_POINT('Origin',(59.8,242.1,24.0213203435596)) ;
#94093=CARTESIAN_POINT('',(59.8,242.,24.0213203435596)) ;
#94094=CARTESIAN_POINT('',(59.7,242.1,24.0213203435596)) ;
#94095=CARTESIAN_POINT('Origin',(67.0732152677426,241.9,17.2933962655652)) ;
#94096=CARTESIAN_POINT('',(67.0732152677426,241.931622776602,17.1985279357602)) ;
#94097=CARTESIAN_POINT('',(67.0732152677426,242.,17.2933962655652)) ;
#94098=CARTESIAN_POINT('Origin',(65.6,242.1,24.0213203435596)) ;
#94099=CARTESIAN_POINT('',(65.7,242.1,24.0213203435596)) ;
#94100=CARTESIAN_POINT('',(65.6,242.,24.0213203435596)) ;
#94101=CARTESIAN_POINT('Origin',(65.6,242.1,24.0213203435596)) ;
#94102=CARTESIAN_POINT('',(65.7,242.1,24.0213203435596)) ;
#94103=CARTESIAN_POINT('',(65.6,242.,24.0213203435596)) ;
#94104=CARTESIAN_POINT('Origin',(65.8,243.768377223398,17.9161886733647)) ;
#94105=CARTESIAN_POINT('',(65.8,244.031622776602,17.8985279357602)) ;
#94106=CARTESIAN_POINT('Origin',(65.8,244.,17.9933962655652)) ;
#94107=CARTESIAN_POINT('',(65.8,243.8,17.8213203435596)) ;
#94108=CARTESIAN_POINT('',(65.7,243.768377223398,17.9161886733647)) ;
#94109=CARTESIAN_POINT('Ctrl Pts',(65.9404964381473,244.284865061027,17.9829450296875)) ;
#94110=CARTESIAN_POINT('Ctrl Pts',(65.8548709640911,244.23093375671,17.9649691455176)) ;
#94111=CARTESIAN_POINT('Ctrl Pts',(65.8002174113109,244.131095361456,17.9316866080974)) ;
#94112=CARTESIAN_POINT('Ctrl Pts',(65.8008983432499,244.029922223798,17.8979656321695)) ;
#94113=CARTESIAN_POINT('Ctrl Pts',(65.926661685959,244.304690467608,17.9893497096592)) ;
#94114=CARTESIAN_POINT('Ctrl Pts',(65.8331874853583,244.247141411488,17.9701164230807)) ;
#94115=CARTESIAN_POINT('Ctrl Pts',(65.7720145633604,244.1402530333,17.9345713375739)) ;
#94116=CARTESIAN_POINT('Ctrl Pts',(65.7706405073659,244.029858881983,17.8976377622117)) ;
#94117=CARTESIAN_POINT('Ctrl Pts',(65.9026183136662,244.33370948865,18.0167815320695)) ;
#94118=CARTESIAN_POINT('Ctrl Pts',(65.7955896720674,244.269304088194,17.9969915494265)) ;
#94119=CARTESIAN_POINT('Ctrl Pts',(65.7229721832936,244.149101928229,17.9601104641158)) ;
#94120=CARTESIAN_POINT('Ctrl Pts',(65.7183227383958,244.021629003268,17.9214387220682)) ;
#94121=CARTESIAN_POINT('Ctrl Pts',(65.889532984467,244.340167226494,18.0597208762946)) ;
#94122=CARTESIAN_POINT('Ctrl Pts',(65.7760178032742,244.270022860549,18.0411808238425)) ;
#94123=CARTESIAN_POINT('Ctrl Pts',(65.701573447933,244.139670349221,18.0067716316214)) ;
#94124=CARTESIAN_POINT('Ctrl Pts',(65.699966159831,244.004831770862,17.9715157748671)) ;
#94125=CARTESIAN_POINT('Ctrl Pts',(65.8867840653894,244.338435475849,18.0780051345276)) ;
#94126=CARTESIAN_POINT('Ctrl Pts',(65.7723078698088,244.266384553046,18.0599924038268)) ;
#94127=CARTESIAN_POINT('Ctrl Pts',(65.6991798482406,244.132988977868,18.0266435100323)) ;
#94128=CARTESIAN_POINT('Ctrl Pts',(65.700006943225,243.997728300858,17.9928283407797)) ;
#94129=CARTESIAN_POINT('',(65.9386488833497,244.284537420614,17.9828328170975)) ;
#94130=CARTESIAN_POINT('Origin',(65.9386488833497,244.252914644012,18.0777011469026)) ;
#94131=CARTESIAN_POINT('Origin',(66.1,244.031622776602,17.8985279357602)) ;
#94132=CARTESIAN_POINT('Ctrl Pts',(65.8848651777997,244.337219525349,18.0777011469026)) ;
#94133=CARTESIAN_POINT('Ctrl Pts',(65.9479936757444,244.377493403818,18.0877696165197)) ;
#94134=CARTESIAN_POINT('Ctrl Pts',(66.0239249506928,244.4,18.0918966374184)) ;
#94135=CARTESIAN_POINT('Ctrl Pts',(66.1,244.4,18.0918966374184)) ;
#94136=CARTESIAN_POINT('Ctrl Pts',(65.8885516400003,244.339571365413,18.0533102596963)) ;
#94137=CARTESIAN_POINT('Ctrl Pts',(65.9506433947663,244.378209794597,18.0630973328873)) ;
#94138=CARTESIAN_POINT('Ctrl Pts',(66.0251770337231,244.4,18.0670030923248)) ;
#94139=CARTESIAN_POINT('Ctrl Pts',(66.1,244.4,18.0670030923248)) ;
#94140=CARTESIAN_POINT('Ctrl Pts',(65.9040598961178,244.329415666601,18.0108507134782)) ;
#94141=CARTESIAN_POINT('Ctrl Pts',(65.9615840543736,244.363516408185,18.0201474104081)) ;
#94142=CARTESIAN_POINT('Ctrl Pts',(66.0306825545291,244.382934786786,18.0236727418492)) ;
#94143=CARTESIAN_POINT('Ctrl Pts',(66.1,244.382934786786,18.0236727418492)) ;
#94144=CARTESIAN_POINT('Ctrl Pts',(65.9282779384441,244.299168044213,17.9877096916306)) ;
#94145=CARTESIAN_POINT('Ctrl Pts',(65.9786741316863,244.32791510767,17.9966840244951)) ;
#94146=CARTESIAN_POINT('Ctrl Pts',(66.0392695942916,244.344107193227,18.0002280477271)) ;
#94147=CARTESIAN_POINT('Ctrl Pts',(66.1,244.344107193227,18.0002280477271)) ;
#94148=CARTESIAN_POINT('Ctrl Pts',(65.9386488833498,244.284537420614,17.9828328170975)) ;
#94149=CARTESIAN_POINT('Ctrl Pts',(65.9859952568083,244.311189251953,17.9917167608773)) ;
#94150=CARTESIAN_POINT('Ctrl Pts',(66.0429437130196,244.326083322956,17.9953582499056)) ;
#94151=CARTESIAN_POINT('Ctrl Pts',(66.1,244.326083322956,17.9953582499056)) ;
#94152=CARTESIAN_POINT('Ctrl Pts',(66.1,244.326083322956,17.9953582499056)) ;
#94153=CARTESIAN_POINT('Ctrl Pts',(66.0429437130196,244.326083322956,17.9953582499056)) ;
#94154=CARTESIAN_POINT('Ctrl Pts',(65.9859952568083,244.311189251953,17.9917167608773)) ;
#94155=CARTESIAN_POINT('Ctrl Pts',(65.9386488833498,244.284537420614,17.9828328170975)) ;
#94156=CARTESIAN_POINT('Origin',(59.3,244.147690779557,18.0213203435596)) ;
#94157=CARTESIAN_POINT('',(59.5361339486826,244.47055415357,24.0213203435596)) ;
#94158=CARTESIAN_POINT('',(59.5361339486826,244.47055415357,18.0213203435596)) ;
#94159=CARTESIAN_POINT('',(59.7,244.147690779557,24.0213203435596)) ;
#94160=CARTESIAN_POINT('Origin',(59.3,244.147690779557,24.0213203435596)) ;
#94161=CARTESIAN_POINT('',(59.7,244.147690779557,18.0213203435596)) ;
#94162=CARTESIAN_POINT('Origin',(59.7,244.4,24.0213203435596)) ;
#94163=CARTESIAN_POINT('',(64.0732152677426,244.4,18.5618897586017)) ;
#94164=CARTESIAN_POINT('Origin',(64.0732152677426,243.65,18.5618897586017)) ;
#94165=CARTESIAN_POINT('',(64.0732152677426,243.887170824513,17.8503772850638)) ;
#94166=CARTESIAN_POINT('Origin',(68.4464305354851,241.4,17.0213203435596)) ;
#94167=CARTESIAN_POINT('',(70.7915467797171,244.284537420614,17.9828328170975)) ;
#94168=CARTESIAN_POINT('',(61.8303059750075,244.284537420614,17.9828328170975)) ;
#94169=CARTESIAN_POINT('',(68.4423055214479,238.515462579386,16.0598078700218)) ;
#94170=CARTESIAN_POINT('Origin',(74.5283628290597,239.4,16.3546536768929)) ;
#94171=CARTESIAN_POINT('',(69.2696458032277,238.515462579386,16.0598078700217)) ;
#94172=CARTESIAN_POINT('Origin',(61.8303059750075,244.521708245126,17.2713203435596)) ;
#94173=CARTESIAN_POINT('',(68.3954399375726,244.400001501795,18.0113751658507)) ;
#94174=CARTESIAN_POINT('Origin',(68.7866534367343,244.532775091534,17.7025224033626)) ;
#94175=CARTESIAN_POINT('',(68.3828427124747,244.521708245126,18.0213203435596)) ;
#94176=CARTESIAN_POINT('Origin',(69.3328427124747,244.521708245126,17.2713203435596)) ;
#94177=CARTESIAN_POINT('',(71.1238651198807,244.521708245126,18.0213203435596)) ;
#94178=CARTESIAN_POINT('',(61.8303059750075,244.521708245126,18.0213203435596)) ;
#94179=CARTESIAN_POINT('Ctrl Pts',(71.1238651198807,244.521708245126,18.0213203435596)) ;
#94180=CARTESIAN_POINT('Ctrl Pts',(71.0892631962886,244.498707682821,18.0213203435596)) ;
#94181=CARTESIAN_POINT('Ctrl Pts',(71.0540815843477,244.474813864772,18.0202605768952)) ;
#94182=CARTESIAN_POINT('Ctrl Pts',(71.0186887369256,244.450216947004,18.0179052310927)) ;
#94183=CARTESIAN_POINT('Ctrl Pts',(70.983961512167,244.426082616089,18.0155941815721)) ;
#94184=CARTESIAN_POINT('Ctrl Pts',(70.9490309224995,244.401271595668,18.0120351354193)) ;
#94185=CARTESIAN_POINT('Ctrl Pts',(70.9142450211489,244.376005954662,18.0070314570774)) ;
#94186=CARTESIAN_POINT('Ctrl Pts',(70.88019684882,244.351276139836,18.0021338952536)) ;
#94187=CARTESIAN_POINT('Ctrl Pts',(70.8462872928706,244.326111176708,17.9958517649843)) ;
#94188=CARTESIAN_POINT('Ctrl Pts',(70.8128427286074,244.300755833278,17.9880350927442)) ;
#94189=CARTESIAN_POINT('Ctrl Pts',(70.8057219499922,244.295357353996,17.986370822518)) ;
#94190=CARTESIAN_POINT('Ctrl Pts',(70.7986222503317,244.289950365561,17.98463713208)) ;
#94191=CARTESIAN_POINT('Ctrl Pts',(70.7915467797171,244.284537420614,17.9828328170977)) ;
#94192=CARTESIAN_POINT('Origin',(66.9,250.2125,19.5627416997969)) ;
#94193=CARTESIAN_POINT('',(66.8,245.395181184141,19.562741699797)) ;
#94194=CARTESIAN_POINT('',(66.8,252.,19.5627416997969)) ;
#94195=CARTESIAN_POINT('',(66.8,250.2125,19.5627416997969)) ;
#94196=CARTESIAN_POINT('Origin',(66.9,251.9,19.5627416997969)) ;
#94197=CARTESIAN_POINT('Origin',(66.9,245.358578643763,19.5627416997969)) ;
#94198=CARTESIAN_POINT('Origin',(66.9651142374916,245.423692881254,19.4976274623054)) ;
#94199=CARTESIAN_POINT('',(65.7,244.229289321881,20.6213203435597)) ;
#94200=CARTESIAN_POINT('',(66.8944035593729,245.423692881254,19.4269167841868)) ;
#94201=CARTESIAN_POINT('',(65.7,244.3,20.6920310216783)) ;
#94202=CARTESIAN_POINT('Origin',(65.7,244.158578643763,20.762741699797)) ;
#94203=CARTESIAN_POINT('',(66.8,245.4,19.5920310216783)) ;
#94204=CARTESIAN_POINT('',(66.8944035593729,245.494403559373,19.4976274623054)) ;
#94205=CARTESIAN_POINT('Origin',(66.8,245.258578643763,19.6627416997969)) ;
#94206=CARTESIAN_POINT('Origin',(66.8,250.6,24.0213203435596)) ;
#94207=CARTESIAN_POINT('',(66.8,252.,24.0213203435596)) ;
#94208=CARTESIAN_POINT('',(66.8,245.4,24.0213203435596)) ;
#94209=CARTESIAN_POINT('',(66.8,245.4,24.0213203435596)) ;
#94210=CARTESIAN_POINT('',(66.8,252.,24.0213203435596)) ;
#94211=CARTESIAN_POINT('',(66.8000000000001,244.4,24.0213203435596)) ;
#94212=CARTESIAN_POINT('',(66.8,252.,23.0213203435596)) ;
#94213=CARTESIAN_POINT('',(66.8,252.,24.0213203435596)) ;
#94214=CARTESIAN_POINT('',(66.8,251.2,23.0213203435596)) ;
#94215=CARTESIAN_POINT('Origin',(66.3,244.9,24.0213203435596)) ;
#94216=CARTESIAN_POINT('',(65.7,244.3,24.0213203435596)) ;
#94217=CARTESIAN_POINT('',(65.7,244.3,24.0213203435596)) ;
#94218=CARTESIAN_POINT('',(66.0500000000001,244.65,24.0213203435596)) ;
#94219=CARTESIAN_POINT('Origin',(65.7,244.4,24.0213203435596)) ;
#94220=CARTESIAN_POINT('',(65.7,253.,24.0213203435596)) ;
#94221=CARTESIAN_POINT('',(65.7,247.1125,20.6213203435596)) ;
#94222=CARTESIAN_POINT('Ctrl Pts',(59.6215180227928,252.943103132053,20.0052643657055)) ;
#94223=CARTESIAN_POINT('Ctrl Pts',(59.4587725290195,252.824132060153,19.9903878946469)) ;
#94224=CARTESIAN_POINT('Ctrl Pts',(59.2951932514256,252.704225739539,19.9662044395718)) ;
#94225=CARTESIAN_POINT('Ctrl Pts',(59.1497059100836,252.591093317904,19.9188077169749)) ;
#94226=CARTESIAN_POINT('Ctrl Pts',(59.6134529174683,252.961577359466,19.9973173267384)) ;
#94227=CARTESIAN_POINT('Ctrl Pts',(59.4484449972835,252.850355285,19.975257967573)) ;
#94228=CARTESIAN_POINT('Ctrl Pts',(59.2832533401182,252.736942886568,19.9376027653372)) ;
#94229=CARTESIAN_POINT('Ctrl Pts',(59.1526056913556,252.627429846356,19.8774372154673)) ;
#94230=CARTESIAN_POINT('Ctrl Pts',(59.5953124915619,253.000455378881,19.9879673050628)) ;
#94231=CARTESIAN_POINT('Ctrl Pts',(59.4229785428761,252.907413224572,19.9572312235567)) ;
#94232=CARTESIAN_POINT('Ctrl Pts',(59.2498021909738,252.812198346872,19.9031169114175)) ;
#94233=CARTESIAN_POINT('Ctrl Pts',(59.127813604899,252.728969853432,19.818935866661)) ;
#94234=CARTESIAN_POINT('Ctrl Pts',(59.5750531169448,253.039128908801,19.9926485628779)) ;
#94235=CARTESIAN_POINT('Ctrl Pts',(59.392366555406,252.963955576352,19.9661862864617)) ;
#94236=CARTESIAN_POINT('Ctrl Pts',(59.2086840835645,252.888185966827,19.9217979904099)) ;
#94237=CARTESIAN_POINT('Ctrl Pts',(59.0586509200866,252.823325335416,19.8446456789754)) ;
#94238=CARTESIAN_POINT('Ctrl Pts',(59.5649218537582,253.057403741307,19.9983832323394)) ;
#94239=CARTESIAN_POINT('Ctrl Pts',(59.3770535644003,252.989679071533,19.9771311308272)) ;
#94240=CARTESIAN_POINT('Ctrl Pts',(59.1883855218148,252.921262994303,19.9425833378629)) ;
#94241=CARTESIAN_POINT('Ctrl Pts',(59.0238256449734,252.853553390593,19.8748737341529)) ;
#94242=CARTESIAN_POINT('',(59.1497059100836,252.591093317904,19.9188077169749)) ;
#94243=CARTESIAN_POINT('Ctrl Pts',(59.542455661465,252.885254883942,19.9972444447401)) ;
#94244=CARTESIAN_POINT('Ctrl Pts',(59.4062589370116,252.785468535468,19.9819452098712)) ;
#94245=CARTESIAN_POINT('Ctrl Pts',(59.2716294139949,252.685902262273,19.95852783585)) ;
#94246=CARTESIAN_POINT('Ctrl Pts',(59.1497059100836,252.591093317904,19.9188077169749)) ;
#94247=CARTESIAN_POINT('Origin',(59.0238256449734,252.712132034356,20.0162950903902)) ;
#94248=CARTESIAN_POINT('Origin',(57.5854307313793,251.289402981384,18.5935660374187)) ;
#94249=CARTESIAN_POINT('Origin',(58.508445556536,252.249338399547,19.5535014555817)) ;
#94250=CARTESIAN_POINT('Origin',(58.7659637180533,252.517157287525,19.8213203435596)) ;
#94251=CARTESIAN_POINT('Ctrl Pts',(58.7659637180532,252.658578643763,19.6798989873223)) ;
#94252=CARTESIAN_POINT('Ctrl Pts',(58.8312395983061,252.726465559226,19.7477859027853)) ;
#94253=CARTESIAN_POINT('Ctrl Pts',(58.9209234411789,252.794277371414,19.815597714974)) ;
#94254=CARTESIAN_POINT('Ctrl Pts',(59.0238256449735,252.853553390593,19.8748737341529)) ;
#94255=CARTESIAN_POINT('Ctrl Pts',(58.7987744253355,252.642804265262,19.6641246088212)) ;
#94256=CARTESIAN_POINT('Ctrl Pts',(58.8593200371507,252.709067270073,19.7304450892964)) ;
#94257=CARTESIAN_POINT('Ctrl Pts',(58.9447138592872,252.776719345374,19.7980061774175)) ;
#94258=CARTESIAN_POINT('Ctrl Pts',(59.043725802181,252.836280216206,19.8576005597657)) ;
#94259=CARTESIAN_POINT('Ctrl Pts',(58.8560072121908,252.600153838287,19.6517435099733)) ;
#94260=CARTESIAN_POINT('Ctrl Pts',(58.9083980147272,252.665691705911,19.7131626692118)) ;
#94261=CARTESIAN_POINT('Ctrl Pts',(58.9862562096281,252.734888009256,19.7784583013549)) ;
#94262=CARTESIAN_POINT('Ctrl Pts',(59.0785034559233,252.796663641143,19.8368436943977)) ;
#94263=CARTESIAN_POINT('Ctrl Pts',(58.9193709157606,252.511947666345,19.6790230438673)) ;
#94264=CARTESIAN_POINT('Ctrl Pts',(58.966096968321,252.57969046616,19.7287746196292)) ;
#94265=CARTESIAN_POINT('Ctrl Pts',(59.0374007547605,252.653426585229,19.7848110624398)) ;
#94266=CARTESIAN_POINT('Ctrl Pts',(59.1228031445117,252.720566563636,19.8360372340782)) ;
#94267=CARTESIAN_POINT('Ctrl Pts',(58.939090293356,252.431231488413,19.7407782818034)) ;
#94268=CARTESIAN_POINT('Ctrl Pts',(58.9902256027549,252.50112873637,19.7794810364602)) ;
#94269=CARTESIAN_POINT('Ctrl Pts',(59.063052354485,252.577729006518,19.8236599443425)) ;
#94270=CARTESIAN_POINT('Ctrl Pts',(59.1476646149207,252.648970096141,19.8644745938916)) ;
#94271=CARTESIAN_POINT('Ctrl Pts',(58.9221907728626,252.391078403777,19.7971809053757)) ;
#94272=CARTESIAN_POINT('Ctrl Pts',(58.9828221520423,252.460001328931,19.8317384222115)) ;
#94273=CARTESIAN_POINT('Ctrl Pts',(59.0623707400732,252.535288497676,19.8682866555266)) ;
#94274=CARTESIAN_POINT('Ctrl Pts',(59.1509486734859,252.606666115812,19.9010775020431)) ;
#94275=CARTESIAN_POINT('Ctrl Pts',(58.9101303310336,252.378535544275,19.8213203435596)) ;
#94276=CARTESIAN_POINT('Ctrl Pts',(58.9754062112864,252.446422459738,19.8552638012911)) ;
#94277=CARTESIAN_POINT('Ctrl Pts',(59.0587301003317,252.520349612145,19.8891697073854)) ;
#94278=CARTESIAN_POINT('Ctrl Pts',(59.1497059100837,252.591093317904,19.9188077169749)) ;
#94279=CARTESIAN_POINT('Origin',(59.3208772194954,252.517157287525,19.8213203435596)) ;
#94280=CARTESIAN_POINT('Ctrl Pts',(58.6541618099201,252.112319238985,19.5569044323066)) ;
#94281=CARTESIAN_POINT('Ctrl Pts',(58.6412166009376,252.099019648315,19.5315608669829)) ;
#94282=CARTESIAN_POINT('Ctrl Pts',(58.6089650298832,252.060786697827,19.4580880570343)) ;
#94283=CARTESIAN_POINT('Ctrl Pts',(58.5547081014922,252.00171431334,19.3867568112521)) ;
#94284=CARTESIAN_POINT('Ctrl Pts',(58.5216837989603,251.967622766116,19.3539222570156)) ;
#94285=CARTESIAN_POINT('Ctrl Pts',(58.6704529317958,252.128834613613,19.5244813361219)) ;
#94286=CARTESIAN_POINT('Ctrl Pts',(58.6563632481609,252.11721748364,19.5005676840661)) ;
#94287=CARTESIAN_POINT('Ctrl Pts',(58.6192697049124,252.081148152115,19.4296226050024)) ;
#94288=CARTESIAN_POINT('Ctrl Pts',(58.5632183786603,252.021835092628,19.3587907782628)) ;
#94289=CARTESIAN_POINT('Ctrl Pts',(58.5301886892986,251.987547381425,19.325699698679)) ;
#94290=CARTESIAN_POINT('Ctrl Pts',(58.6834103241829,252.172743456881,19.4679237313148)) ;
#94291=CARTESIAN_POINT('Ctrl Pts',(58.6670478349588,252.162202291369,19.4467076700389)) ;
#94292=CARTESIAN_POINT('Ctrl Pts',(58.6224726974963,252.126421961247,19.3816931047035)) ;
#94293=CARTESIAN_POINT('Ctrl Pts',(58.5644098772969,252.066679637707,19.3128450049597)) ;
#94294=CARTESIAN_POINT('Ctrl Pts',(58.5315660192152,252.032390152714,19.2795140331204)) ;
#94295=CARTESIAN_POINT('Ctrl Pts',(58.6559664334228,252.262045840093,19.4054163366162)) ;
#94296=CARTESIAN_POINT('Ctrl Pts',(58.636535671422,252.248751266018,19.3866086493998)) ;
#94297=CARTESIAN_POINT('Ctrl Pts',(58.5862516151643,252.206525568018,19.329729810431)) ;
#94298=CARTESIAN_POINT('Ctrl Pts',(58.5288429323904,252.146723044933,19.2656131002727)) ;
#94299=CARTESIAN_POINT('Ctrl Pts',(58.4967383304864,252.113266200792,19.232617788478)) ;
#94300=CARTESIAN_POINT('Ctrl Pts',(58.5932444721227,252.342557495049,19.3861425626071)) ;
#94301=CARTESIAN_POINT('Ctrl Pts',(58.5718821662184,252.324168403092,19.3666955691386)) ;
#94302=CARTESIAN_POINT('Ctrl Pts',(58.5221767212164,252.27324709964,19.3129859822417)) ;
#94303=CARTESIAN_POINT('Ctrl Pts',(58.4683968239059,252.214587012998,19.2535098455819)) ;
#94304=CARTESIAN_POINT('Ctrl Pts',(58.4372786347936,252.182442930322,19.2214525899989)) ;
#94305=CARTESIAN_POINT('Ctrl Pts',(58.5358524085125,252.381707064668,19.4030284834634)) ;
#94306=CARTESIAN_POINT('Ctrl Pts',(58.5135668240936,252.35975300744,19.3810656990374)) ;
#94307=CARTESIAN_POINT('Ctrl Pts',(58.466576100367,252.304160763346,19.3254641250641)) ;
#94308=CARTESIAN_POINT('Ctrl Pts',(58.4164010358533,252.2473691237,19.2686897384215)) ;
#94309=CARTESIAN_POINT('Ctrl Pts',(58.3860774651112,252.216264757314,19.2375851065789)) ;
#94310=CARTESIAN_POINT('Ctrl Pts',(58.5112912559021,252.39369690533,19.4150172488892)) ;
#94311=CARTESIAN_POINT('Ctrl Pts',(58.488596480636,252.370452373203,19.3917727167619)) ;
#94312=CARTESIAN_POINT('Ctrl Pts',(58.4427445299486,252.313461846912,19.334782190472)) ;
#94313=CARTESIAN_POINT('Ctrl Pts',(58.3941384948706,252.257638852692,19.2789591962518)) ;
#94314=CARTESIAN_POINT('Ctrl Pts',(58.3641533318596,252.226959669971,19.2482800135306)) ;
#94315=CARTESIAN_POINT('',(58.5249792341639,251.971066018137,19.3570204704755)) ;
#94316=CARTESIAN_POINT('Origin',(58.3670916964374,252.088555764606,19.3927188206398)) ;
#94317=CARTESIAN_POINT('Ctrl Pts',(58.6524986843825,252.11059862929,19.5535233690183)) ;
#94318=CARTESIAN_POINT('Ctrl Pts',(58.6490777400388,252.107038472653,19.5466722663875)) ;
#94319=CARTESIAN_POINT('Ctrl Pts',(58.6456004439748,252.103274227079,19.5393615524109)) ;
#94320=CARTESIAN_POINT('Ctrl Pts',(58.6419741682487,252.099258925526,19.5317637793487)) ;
#94321=CARTESIAN_POINT('Ctrl Pts',(58.6384200614618,252.095323535175,19.5243172146512)) ;
#94322=CARTESIAN_POINT('Ctrl Pts',(58.6347225086479,252.091146337458,19.5165945586219)) ;
#94323=CARTESIAN_POINT('Ctrl Pts',(58.630821440443,252.086704458926,19.5087232340329)) ;
#94324=CARTESIAN_POINT('Ctrl Pts',(58.6269702679149,252.082319393175,19.5009525857324)) ;
#94325=CARTESIAN_POINT('Ctrl Pts',(58.6229207512004,252.077676015761,19.4930368668497)) ;
#94326=CARTESIAN_POINT('Ctrl Pts',(58.6186441018831,252.072780693303,19.4850679359159)) ;
#94327=CARTESIAN_POINT('Ctrl Pts',(58.6156853025889,252.069393865074,19.4795546320481)) ;
#94328=CARTESIAN_POINT('Ctrl Pts',(58.6126184029932,252.065887060929,19.4740152306126)) ;
#94329=CARTESIAN_POINT('Ctrl Pts',(58.60944188193,252.062271443542,19.4684719115025)) ;
#94330=CARTESIAN_POINT('Ctrl Pts',(58.6043334334077,252.056456844825,19.4595572026895)) ;
#94331=CARTESIAN_POINT('Ctrl Pts',(58.5989562698347,252.050376860908,19.450675029644)) ;
#94332=CARTESIAN_POINT('Ctrl Pts',(58.5932897765977,252.04404070345,19.4418943388873)) ;
#94333=CARTESIAN_POINT('Ctrl Pts',(58.5875867409455,252.037663685006,19.4330570226952)) ;
#94334=CARTESIAN_POINT('Ctrl Pts',(58.5815906397197,252.031027137424,19.4243225888452)) ;
#94335=CARTESIAN_POINT('Ctrl Pts',(58.5753214413841,252.024174076536,19.4157649379888)) ;
#94336=CARTESIAN_POINT('Ctrl Pts',(58.5689961570257,252.017259706225,19.4071307279657)) ;
#94337=CARTESIAN_POINT('Ctrl Pts',(58.5623928420313,252.010125071074,19.3986767325429)) ;
#94338=CARTESIAN_POINT('Ctrl Pts',(58.5555738544669,252.002847655641,19.3904798460872)) ;
#94339=CARTESIAN_POINT('Ctrl Pts',(58.5485973256502,251.99540210775,19.3820935843401)) ;
#94340=CARTESIAN_POINT('Ctrl Pts',(58.5413950213182,251.987807285818,19.3739767810072)) ;
#94341=CARTESIAN_POINT('Ctrl Pts',(58.5340779798077,251.980178469763,19.366208203947)) ;
#94342=CARTESIAN_POINT('Ctrl Pts',(58.5311233572343,251.977097952577,19.3630712512438)) ;
#94343=CARTESIAN_POINT('Ctrl Pts',(58.5281505221452,251.974012237786,19.3599910098373)) ;
#94344=CARTESIAN_POINT('Ctrl Pts',(58.5251687296973,251.970930243872,19.3569723289424)) ;
#94345=CARTESIAN_POINT('Ctrl Pts',(58.524967204456,251.971078582415,19.3570195820997)) ;
#94346=CARTESIAN_POINT('Ctrl Pts',(58.1932634960872,251.627647614635,19.0202451972619)) ;
#94347=CARTESIAN_POINT('Ctrl Pts',(57.8654129205822,251.287968355625,18.6871483232392)) ;
#94348=CARTESIAN_POINT('Ctrl Pts',(57.5423066932673,250.95296417531,18.3586344366773)) ;
#94349=CARTESIAN_POINT('Ctrl Pts',(58.5334325604522,251.991006744364,19.328878031335)) ;
#94350=CARTESIAN_POINT('Ctrl Pts',(58.202537180283,251.647324552634,18.9915783013781)) ;
#94351=CARTESIAN_POINT('Ctrl Pts',(57.8754995261934,251.307368901923,18.6579788187517)) ;
#94352=CARTESIAN_POINT('Ctrl Pts',(57.5532400350036,250.972037111679,18.328983776375)) ;
#94353=CARTESIAN_POINT('Ctrl Pts',(58.5347701387631,252.035810849651,19.2827761601016)) ;
#94354=CARTESIAN_POINT('Ctrl Pts',(58.205003850642,251.692198114189,18.9443126242704)) ;
#94355=CARTESIAN_POINT('Ctrl Pts',(57.8791543584745,251.352251162712,18.6095560812731)) ;
#94356=CARTESIAN_POINT('Ctrl Pts',(57.5581161076161,251.016886757035,18.279416657513)) ;
#94357=CARTESIAN_POINT('Ctrl Pts',(58.4998940599975,252.116554687307,19.2358703317831)) ;
#94358=CARTESIAN_POINT('Ctrl Pts',(58.1707506410098,251.773947691982,18.8957653654841)) ;
#94359=CARTESIAN_POINT('Ctrl Pts',(57.8455821936292,251.434982083835,18.5593363592066)) ;
#94360=CARTESIAN_POINT('Ctrl Pts',(57.525280969944,251.100564766762,18.227505789981)) ;
#94361=CARTESIAN_POINT('Ctrl Pts',(58.4403340595383,252.185604669324,19.2246075759389)) ;
#94362=CARTESIAN_POINT('Ctrl Pts',(58.1107466473917,251.844202743674,18.8836747590476)) ;
#94363=CARTESIAN_POINT('Ctrl Pts',(57.7851546063529,251.506441300288,18.5463966965541)) ;
#94364=CARTESIAN_POINT('Ctrl Pts',(57.4644511534692,251.173238980184,18.2136828428116)) ;
#94365=CARTESIAN_POINT('Ctrl Pts',(58.3890508349148,252.219324353113,19.2406446966726)) ;
#94366=CARTESIAN_POINT('Ctrl Pts',(58.0587653814927,251.878470792537,18.899794609743)) ;
#94367=CARTESIAN_POINT('Ctrl Pts',(57.7324871267912,251.541263118157,18.5625797539281)) ;
#94368=CARTESIAN_POINT('Ctrl Pts',(57.4110825009508,251.208617131752,18.2299374753112)) ;
#94369=CARTESIAN_POINT('Ctrl Pts',(58.3670916964373,252.229977120843,19.2512974644025)) ;
#94370=CARTESIAN_POINT('Ctrl Pts',(58.0365134267979,251.889257498265,18.9105778418249)) ;
#94371=CARTESIAN_POINT('Ctrl Pts',(57.7099315251708,251.552182999603,18.5735033431626)) ;
#94372=CARTESIAN_POINT('Ctrl Pts',(57.3882337581722,251.21966991411,18.2409902576697)) ;
#94373=CARTESIAN_POINT('',(57.5423066932673,250.95296417531,18.3586344366773)) ;
#94374=CARTESIAN_POINT('Origin',(57.3882337581722,251.078248557873,18.382411613907)) ;
#94375=CARTESIAN_POINT('Origin',(62.771739895016,256.106054470067,23.4102175261011)) ;
#94376=CARTESIAN_POINT('Ctrl Pts',(57.08796902046,250.694045291555,18.0213351046284)) ;
#94377=CARTESIAN_POINT('Ctrl Pts',(57.1258423453833,250.802045427011,18.0220127055346)) ;
#94378=CARTESIAN_POINT('Ctrl Pts',(57.2314306338671,250.992507784516,18.066477901939)) ;
#94379=CARTESIAN_POINT('Ctrl Pts',(57.3390787831373,251.150386903953,18.1717072475128)) ;
#94380=CARTESIAN_POINT('Ctrl Pts',(57.3882337581722,251.21966991411,18.2409902576698)) ;
#94381=CARTESIAN_POINT('Ctrl Pts',(57.107641411712,250.684638364735,18.0212760848678)) ;
#94382=CARTESIAN_POINT('Ctrl Pts',(57.1469906807295,250.788268335791,18.0205613562701)) ;
#94383=CARTESIAN_POINT('Ctrl Pts',(57.255633922619,250.973466511641,18.0590773371353)) ;
#94384=CARTESIAN_POINT('Ctrl Pts',(57.3675725762443,251.133340840632,18.1585412492811)) ;
#94385=CARTESIAN_POINT('Ctrl Pts',(57.4186987485437,251.204932870965,18.2262532145251)) ;
#94386=CARTESIAN_POINT('Ctrl Pts',(57.1420566838705,250.668142088394,18.027486377803)) ;
#94387=CARTESIAN_POINT('Ctrl Pts',(57.183976115983,250.763206632424,18.0262403194019)) ;
#94388=CARTESIAN_POINT('Ctrl Pts',(57.2979617793206,250.935859716831,18.0586106436234)) ;
#94389=CARTESIAN_POINT('Ctrl Pts',(57.4173496108119,251.093267835686,18.1493153206436)) ;
#94390=CARTESIAN_POINT('Ctrl Pts',(57.4718803430079,251.166163965728,18.2135703095001)) ;
#94391=CARTESIAN_POINT('Ctrl Pts',(57.1911537271729,250.64450016656,18.0535964453211)) ;
#94392=CARTESIAN_POINT('Ctrl Pts',(57.235290594596,250.72552619711,18.0564256989547)) ;
#94393=CARTESIAN_POINT('Ctrl Pts',(57.3527071216605,250.875068403139,18.0913312692755)) ;
#94394=CARTESIAN_POINT('Ctrl Pts',(57.4769453332363,251.017240971583,18.1755695140533)) ;
#94395=CARTESIAN_POINT('Ctrl Pts',(57.533955734056,251.085548454793,18.2341294931593)) ;
#94396=CARTESIAN_POINT('Ctrl Pts',(57.2280967504656,250.626602169704,18.0905610922877)) ;
#94397=CARTESIAN_POINT('Ctrl Pts',(57.2715143002045,250.695684375206,18.1008339037926)) ;
#94398=CARTESIAN_POINT('Ctrl Pts',(57.3847356823201,250.825549532579,18.1472995157663)) ;
#94399=CARTESIAN_POINT('Ctrl Pts',(57.5038966823451,250.949199444535,18.2321302434064)) ;
#94400=CARTESIAN_POINT('Ctrl Pts',(57.5592426011106,251.009151616513,18.2860619448616)) ;
#94401=CARTESIAN_POINT('Ctrl Pts',(57.2461791971729,250.61774963895,18.1233215980465)) ;
#94402=CARTESIAN_POINT('Ctrl Pts',(57.2865158711383,250.680159607724,18.1402603227317)) ;
#94403=CARTESIAN_POINT('Ctrl Pts',(57.3904321283034,250.800687273232,18.1978577670584)) ;
#94404=CARTESIAN_POINT('Ctrl Pts',(57.4991294772935,250.913640261489,18.2851184067917)) ;
#94405=CARTESIAN_POINT('Ctrl Pts',(57.5505066995696,250.967268877587,18.3363964414506)) ;
#94406=CARTESIAN_POINT('Ctrl Pts',(57.2522759660783,250.614740854374,18.1381958555625)) ;
#94407=CARTESIAN_POINT('Ctrl Pts',(57.2908028309611,250.674714714559,18.1580345116492)) ;
#94408=CARTESIAN_POINT('Ctrl Pts',(57.3895885689374,250.792382169794,18.220330010732)) ;
#94409=CARTESIAN_POINT('Ctrl Pts',(57.492936507439,250.901775998676,18.3084379679755)) ;
#94410=CARTESIAN_POINT('Ctrl Pts',(57.5423066932674,250.95296417531,18.3586344366773)) ;
#94411=CARTESIAN_POINT('',(57.2522842181377,250.614754130417,18.1381996970991)) ;
#94412=CARTESIAN_POINT('Ctrl Pts',(57.2522759660783,250.614740854374,18.1381958555625)) ;
#94413=CARTESIAN_POINT('Ctrl Pts',(57.2452365621931,250.625532166615,18.1141521490421)) ;
#94414=CARTESIAN_POINT('Ctrl Pts',(57.2350607949463,250.640021825605,18.0928712338379)) ;
#94415=CARTESIAN_POINT('Ctrl Pts',(57.2097486588519,250.673406188019,18.058304224436)) ;
#94416=CARTESIAN_POINT('Ctrl Pts',(57.1947896709115,250.692061496643,18.0451005266235)) ;
#94417=CARTESIAN_POINT('Ctrl Pts',(57.1694020380105,250.721784873435,18.0321296306987)) ;
#94418=CARTESIAN_POINT('Ctrl Pts',(57.1602559849713,250.732185523338,18.0289839177341)) ;
#94419=CARTESIAN_POINT('Ctrl Pts',(57.1411635563705,250.753269492834,18.025401410602)) ;
#94420=CARTESIAN_POINT('Ctrl Pts',(57.1312497748175,250.76390267473,18.0250400908081)) ;
#94421=CARTESIAN_POINT('Ctrl Pts',(57.1209450813301,250.774641221836,18.0261880479281)) ;
#94422=CARTESIAN_POINT('Ctrl Pts',(57.120652398181,250.77494597076,18.0262219055369)) ;
#94423=CARTESIAN_POINT('Ctrl Pts',(57.1203596587326,250.775250521649,18.0262570222543)) ;
#94424=CARTESIAN_POINT('Ctrl Pts',(57.5423066932674,250.95296417531,18.3586344366773)) ;
#94425=CARTESIAN_POINT('Ctrl Pts',(57.492936507439,250.901775998676,18.3084379679755)) ;
#94426=CARTESIAN_POINT('Ctrl Pts',(57.3896168747837,250.792412131542,18.2203541425176)) ;
#94427=CARTESIAN_POINT('Ctrl Pts',(57.2908569439244,250.674779169542,18.1580686376687)) ;
#94428=CARTESIAN_POINT('Ctrl Pts',(57.2523392883266,250.614839410371,18.1382284672602)) ;
#94429=CARTESIAN_POINT('Origin',(60.4427446298904,253.683899394336,19.8213203435596)) ;
#94430=CARTESIAN_POINT('',(60.4427446298904,253.683899394336,20.0213203435596)) ;
#94431=CARTESIAN_POINT('Origin',(52.2356360608974,253.207106781187,19.5213203435596)) ;
#94432=CARTESIAN_POINT('',(55.1300306216516,253.207106781187,20.0213203435596)) ;
#94433=CARTESIAN_POINT('Ctrl Pts',(55.1300306216516,253.207106781187,20.0213203435596)) ;
#94434=CARTESIAN_POINT('Ctrl Pts',(54.9727816340446,253.072343999508,20.0213203435596)) ;
#94435=CARTESIAN_POINT('Ctrl Pts',(54.7853404806882,252.94731363725,19.9686339808095)) ;
#94436=CARTESIAN_POINT('Ctrl Pts',(54.6208916966195,252.853553390593,19.8748737341529)) ;
#94437=CARTESIAN_POINT('',(69.2699693783484,253.207106781187,20.0213203435596)) ;
#94438=CARTESIAN_POINT('',(52.2356360608974,253.207106781187,20.0213203435596)) ;
#94439=CARTESIAN_POINT('',(69.7791083033806,252.853553390593,19.8748737341529)) ;
#94440=CARTESIAN_POINT('Ctrl Pts',(69.7791083033805,252.853553390593,19.8748737341529)) ;
#94441=CARTESIAN_POINT('Ctrl Pts',(69.6146576393448,252.947314709111,19.9686350526701)) ;
#94442=CARTESIAN_POINT('Ctrl Pts',(69.4272201636148,253.072342458909,20.0213203435596)) ;
#94443=CARTESIAN_POINT('Ctrl Pts',(69.2699693783484,253.207106781187,20.0213203435596)) ;
#94444=CARTESIAN_POINT('',(66.3707106781187,252.853553390593,19.8748737341529)) ;
#94445=CARTESIAN_POINT('',(52.2356360608974,252.853553390593,19.8748737341529)) ;
#94446=CARTESIAN_POINT('',(65.8856854219273,253.19999999981,20.021269638343)) ;
#94447=CARTESIAN_POINT('Origin',(65.8757359312881,253.207106781187,19.5213203435596)) ;
#94448=CARTESIAN_POINT('',(52.2356360608974,253.2,20.0212698346696)) ;
#94449=CARTESIAN_POINT('Ctrl Pts',(65.881623518379,253.202901361836,20.0213026576949)) ;
#94450=CARTESIAN_POINT('Ctrl Pts',(66.0629141248793,253.073408071479,20.0202134719904)) ;
#94451=CARTESIAN_POINT('Ctrl Pts',(66.2425143263702,252.945122213271,19.9664425568304)) ;
#94452=CARTESIAN_POINT('Ctrl Pts',(66.3707106781187,252.853553390593,19.8748737341529)) ;
#94453=CARTESIAN_POINT('Ctrl Pts',(65.8603864536687,253.181665799482,20.0211240424873)) ;
#94454=CARTESIAN_POINT('Ctrl Pts',(66.0391798872376,253.049783724924,20.0144847987807)) ;
#94455=CARTESIAN_POINT('Ctrl Pts',(66.2151031676496,252.922902350671,19.9527372340496)) ;
#94456=CARTESIAN_POINT('Ctrl Pts',(66.3381379840193,252.837267043544,19.8585873871032)) ;
#94457=CARTESIAN_POINT('Ctrl Pts',(65.8232639540795,253.144444214368,20.0329043207371)) ;
#94458=CARTESIAN_POINT('Ctrl Pts',(65.9977280232127,253.005226836627,20.0194760945433)) ;
#94459=CARTESIAN_POINT('Ctrl Pts',(66.167186464512,252.875203335031,19.9457924120113)) ;
#94460=CARTESIAN_POINT('Ctrl Pts',(66.2813241360136,252.793554120498,19.8454864621427)) ;
#94461=CARTESIAN_POINT('Ctrl Pts',(65.7749943263166,253.095769049503,20.0811186276069)) ;
#94462=CARTESIAN_POINT('Ctrl Pts',(65.9461044669602,252.940725734752,20.0657729104122)) ;
#94463=CARTESIAN_POINT('Ctrl Pts',(66.1107270602757,252.795106259162,19.9834237274542)) ;
#94464=CARTESIAN_POINT('Ctrl Pts',(66.2187011364029,252.7039244006,19.8724931824299)) ;
#94465=CARTESIAN_POINT('Ctrl Pts',(65.7461964320231,253.066423830258,20.1461900919877)) ;
#94466=CARTESIAN_POINT('Ctrl Pts',(65.9191932009661,252.896367685805,20.136008428504)) ;
#94467=CARTESIAN_POINT('Ctrl Pts',(66.0869160227462,252.732236492732,20.0547507894586)) ;
#94468=CARTESIAN_POINT('Ctrl Pts',(66.1997216851912,252.622654654284,19.9347834775349)) ;
#94469=CARTESIAN_POINT('Ctrl Pts',(65.7401074337726,253.059892566227,20.1987710714045)) ;
#94470=CARTESIAN_POINT('Ctrl Pts',(65.9184828909875,252.881535564304,20.1946701420602)) ;
#94471=CARTESIAN_POINT('Ctrl Pts',(66.0939250192433,252.706049839441,20.1175725763353)) ;
#94472=CARTESIAN_POINT('Ctrl Pts',(66.2170745615941,252.582925438406,19.9918655698157)) ;
#94473=CARTESIAN_POINT('Ctrl Pts',(65.7402021621417,253.059797837858,20.221295583349)) ;
#94474=CARTESIAN_POINT('Ctrl Pts',(65.921492768642,252.878507231358,20.2197707233628)) ;
#94475=CARTESIAN_POINT('Ctrl Pts',(66.1010929701329,252.698907029867,20.1444914421387)) ;
#94476=CARTESIAN_POINT('Ctrl Pts',(66.2292893218814,252.570710678119,20.0162950903902)) ;
#94477=CARTESIAN_POINT('Origin',(65.8734821123455,253.2,20.0921424382039)) ;
#94478=CARTESIAN_POINT('',(66.2292893218814,252.570710678119,20.0162950903902)) ;
#94479=CARTESIAN_POINT('Origin',(66.3707106781187,252.712132034356,20.0162950903902)) ;
#94480=CARTESIAN_POINT('Origin',(65.7343145750508,253.065685424949,19.5213203435596)) ;
#94481=CARTESIAN_POINT('Origin',(63.3756911636855,255.707151548789,23.0113146048234)) ;
#94482=CARTESIAN_POINT('',(68.0045941546019,251.21966991411,18.2409902576697)) ;
#94483=CARTESIAN_POINT('',(67.8631727983646,250.936827201635,18.382411613907)) ;
#94484=CARTESIAN_POINT('Origin',(68.0045941546019,251.078248557873,18.382411613907)) ;
#94485=CARTESIAN_POINT('',(63.2342698074482,255.565730192552,23.0113146048234)) ;
#94486=CARTESIAN_POINT('',(63.3756911636855,255.848572905027,22.8698932485861)) ;
#94487=CARTESIAN_POINT('Ctrl Pts',(68.0685234977135,250.731476513624,18.2529125788923)) ;
#94488=CARTESIAN_POINT('Ctrl Pts',(67.9915773915309,250.808422669384,18.2801593165379)) ;
#94489=CARTESIAN_POINT('Ctrl Pts',(67.9208460458532,250.879153909218,18.3247963104889)) ;
#94490=CARTESIAN_POINT('Ctrl Pts',(67.863139102423,250.93686091303,18.3825247079237)) ;
#94491=CARTESIAN_POINT('Ctrl Pts',(68.0625957834865,250.7373902321,18.2194680319063)) ;
#94492=CARTESIAN_POINT('Ctrl Pts',(67.9826680670271,250.81728663264,18.2457549454805)) ;
#94493=CARTESIAN_POINT('Ctrl Pts',(67.908459192823,250.891559782816,18.29032024332)) ;
#94494=CARTESIAN_POINT('Ctrl Pts',(67.8468303112623,250.953150707556,18.3499362264217)) ;
#94495=CARTESIAN_POINT('Ctrl Pts',(68.0635796741313,250.759053528145,18.1610618496374)) ;
#94496=CARTESIAN_POINT('Ctrl Pts',(67.9798052466115,250.845433836891,18.1857150875349)) ;
#94497=CARTESIAN_POINT('Ctrl Pts',(67.9007979465452,250.927216465425,18.230154819357)) ;
#94498=CARTESIAN_POINT('Ctrl Pts',(67.8337102502296,250.996881438386,18.2931030142913)) ;
#94499=CARTESIAN_POINT('Ctrl Pts',(68.0955315081987,250.816176850352,18.0899683881281)) ;
#94500=CARTESIAN_POINT('Ctrl Pts',(68.0105392122114,250.913117794014,18.1148812713429)) ;
#94501=CARTESIAN_POINT('Ctrl Pts',(67.9298874864649,251.006131356308,18.1617654797125)) ;
#94502=CARTESIAN_POINT('Ctrl Pts',(67.8607201289279,251.086540013528,18.2304736893628)) ;
#94503=CARTESIAN_POINT('Ctrl Pts',(68.1472211618773,250.880004775357,18.055685461842)) ;
#94504=CARTESIAN_POINT('Ctrl Pts',(68.0651794996633,250.984185012154,18.0846738399297)) ;
#94505=CARTESIAN_POINT('Ctrl Pts',(67.9881198107097,251.08329094827,18.137196304556)) ;
#94506=CARTESIAN_POINT('Ctrl Pts',(67.9230204305914,251.167821577733,18.2114983154127)) ;
#94507=CARTESIAN_POINT('Ctrl Pts',(68.191141483228,250.92296018793,18.0584107582352)) ;
#94508=CARTESIAN_POINT('Ctrl Pts',(68.1126799325993,251.028292595487,18.0929309831573)) ;
#94509=CARTESIAN_POINT('Ctrl Pts',(68.0400154676919,251.126346778526,18.1512287876413)) ;
#94510=CARTESIAN_POINT('Ctrl Pts',(67.9801172777256,251.207550315327,18.2288610080907)) ;
#94511=CARTESIAN_POINT('Ctrl Pts',(68.2099526347344,250.939674811849,18.0643320877577)) ;
#94512=CARTESIAN_POINT('Ctrl Pts',(68.1330030864753,251.04460755176,18.1014870418244)) ;
#94513=CARTESIAN_POINT('Ctrl Pts',(68.0622678793746,251.141065609732,18.1623578912056)) ;
#94514=CARTESIAN_POINT('Ctrl Pts',(68.0045565913183,251.219763261572,18.2410836242414)) ;
#94515=CARTESIAN_POINT('',(68.20985501736,250.939768737622,18.0643653511196)) ;
#94516=CARTESIAN_POINT('Origin',(68.20985501736,250.872987695115,18.2528866824369)) ;
#94517=CARTESIAN_POINT('Origin',(68.2520815280172,250.547918471983,18.7713203435596)) ;
#94518=CARTESIAN_POINT('Origin',(68.3935028842545,250.68933982822,18.7713203435596)) ;
#94519=CARTESIAN_POINT('Ctrl Pts',(68.20985501736,250.939768737622,18.0643653511195)) ;
#94520=CARTESIAN_POINT('Ctrl Pts',(68.2640374140654,250.865883651205,18.0381925935746)) ;
#94521=CARTESIAN_POINT('Ctrl Pts',(68.3212444282195,250.78787408645,18.0237007750708)) ;
#94522=CARTESIAN_POINT('Ctrl Pts',(68.3787050687238,250.70951866758,18.021591849742)) ;
#94523=CARTESIAN_POINT('Ctrl Pts',(68.1659721653548,250.900778502873,18.0505536062847)) ;
#94524=CARTESIAN_POINT('Ctrl Pts',(68.2226923077703,250.826137853427,18.0288422946047)) ;
#94525=CARTESIAN_POINT('Ctrl Pts',(68.2819524792602,250.748870082081,18.0186430165262)) ;
#94526=CARTESIAN_POINT('Ctrl Pts',(68.3412258152467,250.672066544789,18.0205838310049)) ;
#94527=CARTESIAN_POINT('Ctrl Pts',(68.0789578599896,250.803901913784,18.0783946040854)) ;
#94528=CARTESIAN_POINT('Ctrl Pts',(68.1404418139846,250.735363554207,18.0624840627055)) ;
#94529=CARTESIAN_POINT('Ctrl Pts',(68.2039059525548,250.665266954687,18.0576296401064)) ;
#94530=CARTESIAN_POINT('Ctrl Pts',(68.2666372217533,250.596333931781,18.0630889529167)) ;
#94531=CARTESIAN_POINT('Ctrl Pts',(68.0580726283796,250.74192737162,18.1943887730536)) ;
#94532=CARTESIAN_POINT('Ctrl Pts',(68.1160062559218,250.684163270981,18.1764052639078)) ;
#94533=CARTESIAN_POINT('Ctrl Pts',(68.1762425132091,250.623639667933,18.1676682325686)) ;
#94534=CARTESIAN_POINT('Ctrl Pts',(68.2365706774774,250.563429322523,18.1685349672834)) ;
#94535=CARTESIAN_POINT('Ctrl Pts',(68.0684336611227,250.731566338877,18.2528866824369)) ;
#94536=CARTESIAN_POINT('Ctrl Pts',(68.1226160578281,250.677383942172,18.233693326904)) ;
#94537=CARTESIAN_POINT('Ctrl Pts',(68.1798230719822,250.620176928018,18.2230659933345)) ;
#94538=CARTESIAN_POINT('Ctrl Pts',(68.2372837124865,250.562716287513,18.2215194480934)) ;
#94539=CARTESIAN_POINT('',(68.357584866715,250.738305523749,18.0229216337057)) ;
#94540=CARTESIAN_POINT('Origin',(68.3935028842545,250.68933982822,18.7713203435596)) ;
#94541=CARTESIAN_POINT('Ctrl Pts',(68.2414080333741,250.64489209549,18.0799123114407)) ;
#94542=CARTESIAN_POINT('Ctrl Pts',(68.2546291643386,250.650461761277,18.0666886890814)) ;
#94543=CARTESIAN_POINT('Ctrl Pts',(68.2694566046645,250.656926759755,18.0555657574139)) ;
#94544=CARTESIAN_POINT('Ctrl Pts',(68.3010063111761,250.670467574526,18.0379499729927)) ;
#94545=CARTESIAN_POINT('Ctrl Pts',(68.317760304708,250.677503134716,18.0313727702642)) ;
#94546=CARTESIAN_POINT('Ctrl Pts',(68.3507682624113,250.691144831296,18.0232435116254)) ;
#94547=CARTESIAN_POINT('Ctrl Pts',(68.3633682258265,250.695971216193,18.0222098102947)) ;
#94548=CARTESIAN_POINT('Ctrl Pts',(68.3691979799543,250.70106845124,18.0217842131582)) ;
#94549=CARTESIAN_POINT('Ctrl Pts',(68.3698685266312,250.70187026372,18.0217410723846)) ;
#94550=CARTESIAN_POINT('Ctrl Pts',(68.3706966899262,250.703387313299,18.0216891631644)) ;
#94551=CARTESIAN_POINT('Ctrl Pts',(68.3709338331895,250.704088059953,18.0216751736344)) ;
#94552=CARTESIAN_POINT('Ctrl Pts',(68.3712313275294,250.705902215846,18.021657612549)) ;
#94553=CARTESIAN_POINT('Ctrl Pts',(68.3711853396952,250.707102221528,18.0216601799892)) ;
#94554=CARTESIAN_POINT('Ctrl Pts',(68.3704253757421,250.711057343193,18.0217055973424)) ;
#94555=CARTESIAN_POINT('Ctrl Pts',(68.3691918827918,250.714442050838,18.0217732060915)) ;
#94556=CARTESIAN_POINT('Ctrl Pts',(68.3642229304804,250.725329533552,18.022171205809)) ;
#94557=CARTESIAN_POINT('Ctrl Pts',(68.360737041717,250.732154691993,18.0225201305636)) ;
#94558=CARTESIAN_POINT('Ctrl Pts',(68.3575711698691,250.738297080151,18.0229233951598)) ;
#94559=CARTESIAN_POINT('Origin',(55.2141814145299,249.05,18.0213203435596)) ;
#94560=CARTESIAN_POINT('',(77.9328605382387,244.521708245126,18.0213203435596)) ;
#94561=CARTESIAN_POINT('',(61.8303059750075,244.521708245126,18.0213203435596)) ;
#94562=CARTESIAN_POINT('',(75.4283628290596,245.483789937202,18.0213203435596)) ;
#94563=CARTESIAN_POINT('Origin',(74.5283628290597,239.4,18.0213203435596)) ;
#94564=CARTESIAN_POINT('',(75.4283628290596,246.,18.0213203435596)) ;
#94565=CARTESIAN_POINT('',(75.4283628290596,247.266894968601,18.0213203435596)) ;
#94566=CARTESIAN_POINT('',(73.6283628290596,246.,18.0213203435596)) ;
#94567=CARTESIAN_POINT('',(65.3212721217947,246.,18.0213203435596)) ;
#94568=CARTESIAN_POINT('',(73.6283628290596,245.483789937202,18.0213203435596)) ;
#94569=CARTESIAN_POINT('',(73.6283628290596,247.525,18.0213203435596)) ;
#94570=CARTESIAN_POINT('Origin',(74.5283628290597,239.4,18.0213203435596)) ;
#94571=CARTESIAN_POINT('',(68.3828427124746,250.68933982822,18.0213203435596)) ;
#94572=CARTESIAN_POINT('',(68.3828427124746,249.4375,18.0213203435596)) ;
#94573=CARTESIAN_POINT('',(52.2356360608974,250.68933982822,18.0213203435596)) ;
#94574=CARTESIAN_POINT('',(72.0133921147013,247.214089774802,18.0213203435596)) ;
#94575=CARTESIAN_POINT('',(72.0133921147013,248.124963207434,18.0213203435596)) ;
#94576=CARTESIAN_POINT('',(72.0133921147013,248.637481603717,18.0213203435596)) ;
#94577=CARTESIAN_POINT('',(73.2395171459957,246.537024447301,18.0213203435596)) ;
#94578=CARTESIAN_POINT('Origin',(72.8133921147013,247.214089774802,18.0213203435596)) ;
#94579=CARTESIAN_POINT('',(74.19803042292,247.140284551659,18.0213203435596)) ;
#94580=CARTESIAN_POINT('',(67.3503775087141,242.830572927334,18.0213203435596)) ;
#94581=CARTESIAN_POINT('',(73.8784366494491,247.648083547285,18.0213203435596)) ;
#94582=CARTESIAN_POINT('',(71.0478693800126,252.145540430945,18.0213203435596)) ;
#94583=CARTESIAN_POINT('',(72.9199233725249,247.044823442927,18.0213203435596)) ;
#94584=CARTESIAN_POINT('',(67.4677237907363,243.613369160683,18.0213203435596)) ;
#94585=CARTESIAN_POINT('',(72.6133921147013,247.214089774802,18.0213203435596)) ;
#94586=CARTESIAN_POINT('Origin',(72.8133921147013,247.214089774802,18.0213203435596)) ;
#94587=CARTESIAN_POINT('',(72.6133921147013,248.124963207434,18.0213203435596)) ;
#94588=CARTESIAN_POINT('',(72.6133921147013,248.132044887401,18.0213203435596)) ;
#94589=CARTESIAN_POINT('',(73.1273459706961,248.124963207434,18.0213203435596)) ;
#94590=CARTESIAN_POINT('',(63.8637867646156,248.124963207434,18.0213203435596)) ;
#94591=CARTESIAN_POINT('',(72.2987422718658,250.163082385568,18.0213203435596)) ;
#94592=CARTESIAN_POINT('',(71.6675838322311,251.715544825786,18.0213203435596)) ;
#94593=CARTESIAN_POINT('',(71.4701385730357,248.124963207434,18.0213203435596)) ;
#94594=CARTESIAN_POINT('',(70.8466068278818,246.591260172113,18.0213203435596)) ;
#94595=CARTESIAN_POINT('',(63.416461843198,248.124963207434,18.0213203435596)) ;
#94596=CARTESIAN_POINT('',(74.9348607567984,249.429895468622,18.0213203435596)) ;
#94597=CARTESIAN_POINT('',(75.2544545302692,248.922096472997,18.0213203435596)) ;
#94598=CARTESIAN_POINT('',(72.2495203324155,253.696603031808,18.0213203435596)) ;
#94599=CARTESIAN_POINT('',(76.1283346412558,249.472090948443,18.0213203435596)) ;
#94600=CARTESIAN_POINT('',(68.1060880979734,244.423124592531,18.0213203435596)) ;
#94601=CARTESIAN_POINT('',(76.4348658990794,249.302824616567,18.0213203435596)) ;
#94602=CARTESIAN_POINT('Origin',(76.2348658990794,249.302824616567,18.0213203435596)) ;
#94603=CARTESIAN_POINT('',(76.4348658990794,248.391951183936,18.0213203435596)) ;
#94604=CARTESIAN_POINT('',(76.4348658990794,249.176412308284,18.0213203435596)) ;
#94605=CARTESIAN_POINT('',(75.9209120430846,248.391951183936,18.0213203435596)) ;
#94606=CARTESIAN_POINT('',(65.8745236568046,248.391951183936,18.0213203435596)) ;
#94607=CARTESIAN_POINT('',(76.7495157419148,246.353832005802,18.0213203435596)) ;
#94608=CARTESIAN_POINT('',(74.3655697550003,252.217631603154,18.0213203435596)) ;
#94609=CARTESIAN_POINT('',(77.578119440745,248.391951183936,18.0213203435596)) ;
#94610=CARTESIAN_POINT('',(75.7388649854292,243.867931095515,18.0213203435596)) ;
#94611=CARTESIAN_POINT('',(77.0348658990794,248.391951183936,18.0213203435596)) ;
#94612=CARTESIAN_POINT('',(66.3218485782223,248.391951183936,18.0213203435596)) ;
#94613=CARTESIAN_POINT('',(77.0348658990794,249.302824616567,18.0213203435596)) ;
#94614=CARTESIAN_POINT('',(77.0348658990794,248.670975591968,18.0213203435596)) ;
#94615=CARTESIAN_POINT('',(75.8087408677849,249.979889944069,18.0213203435596)) ;
#94616=CARTESIAN_POINT('Origin',(76.2348658990794,249.302824616567,18.0213203435596)) ;
#94617=CARTESIAN_POINT('',(68.223434379996,245.20592082588,18.0213203435596)) ;
#94618=CARTESIAN_POINT('',(74.2283628290596,249.52834685842,18.0213203435596)) ;
#94619=CARTESIAN_POINT('',(74.8283628290596,249.52834685842,18.0213203435596)) ;
#94620=CARTESIAN_POINT('',(64.9712721217948,249.52834685842,18.0213203435596)) ;
#94621=CARTESIAN_POINT('',(74.2283628290596,246.82834685842,18.0213203435596)) ;
#94622=CARTESIAN_POINT('',(74.2283628290596,249.23917342921,18.0213203435596)) ;
#94623=CARTESIAN_POINT('',(74.8283628290596,246.82834685842,18.0213203435596)) ;
#94624=CARTESIAN_POINT('',(64.7712721217948,246.82834685842,18.0213203435596)) ;
#94625=CARTESIAN_POINT('',(74.8283628290596,247.98917342921,18.0213203435596)) ;
#94626=CARTESIAN_POINT('Origin',(52.2356360608974,250.68933982822,18.7713203435596)) ;
#94627=CARTESIAN_POINT('Origin',(68.3985118238593,250.691109216673,18.5008448049847)) ;
#94628=CARTESIAN_POINT('',(52.2356360608974,251.21966991411,18.2409902576697)) ;
#94629=CARTESIAN_POINT('Origin',(49.257090707265,252.,19.0213203435596)) ;
#94630=CARTESIAN_POINT('',(76.6208916966195,252.853553390593,19.8748737341529)) ;
#94631=CARTESIAN_POINT('Origin',(73.2,255.853553390593,22.8748737341529)) ;
#94632=CARTESIAN_POINT('',(52.2356360608974,252.853553390593,19.8748737341529)) ;
#94633=CARTESIAN_POINT('Origin',(68.3828427124746,249.4375,18.2213203435596)) ;
#94634=CARTESIAN_POINT('Origin',(68.3828427124747,244.521708245126,18.2213203435596)) ;
#94635=CARTESIAN_POINT('Ctrl Pts',(68.274306674866,244.273916677043,18.0470136686937)) ;
#94636=CARTESIAN_POINT('Ctrl Pts',(68.2525104982572,244.35458767695,18.0688098453025)) ;
#94637=CARTESIAN_POINT('Ctrl Pts',(68.2414213562374,244.438144595489,18.0798989873223)) ;
#94638=CARTESIAN_POINT('Ctrl Pts',(68.2414213562374,244.521708245126,18.0798989873223)) ;
#94639=CARTESIAN_POINT('Ctrl Pts',(68.310391048944,244.293415664068,18.0109292946157)) ;
#94640=CARTESIAN_POINT('Ctrl Pts',(68.2892363653393,244.367600584991,18.0321209883094)) ;
#94641=CARTESIAN_POINT('Ctrl Pts',(68.278445380722,244.444667068531,18.0428749628377)) ;
#94642=CARTESIAN_POINT('Ctrl Pts',(68.278445380722,244.521708245126,18.0428749628377)) ;
#94643=CARTESIAN_POINT('Ctrl Pts',(68.362867182144,244.312772739493,17.9917619163006)) ;
#94644=CARTESIAN_POINT('Ctrl Pts',(68.3414167382309,244.380543003792,18.0113579653632)) ;
#94645=CARTESIAN_POINT('Ctrl Pts',(68.3304828349148,244.451143558849,18.0213203435596)) ;
#94646=CARTESIAN_POINT('Ctrl Pts',(68.3304828349148,244.521708245126,18.0213203435596)) ;
#94647=CARTESIAN_POINT('Ctrl Pts',(68.4157280311033,244.326083322955,17.9953582499055)) ;
#94648=CARTESIAN_POINT('Ctrl Pts',(68.3939318544945,244.389770954461,18.0125657577545)) ;
#94649=CARTESIAN_POINT('Ctrl Pts',(68.3828427124747,244.455736942781,18.0213203435596)) ;
#94650=CARTESIAN_POINT('Ctrl Pts',(68.3828427124747,244.521708245126,18.0213203435596)) ;
#94651=CARTESIAN_POINT('Ctrl Pts',(58.6558325375659,252.114065839068,19.604968115859)) ;
#94652=CARTESIAN_POINT('Ctrl Pts',(58.6560546890527,252.114296876615,19.499708534422)) ;
#94653=CARTESIAN_POINT('Ctrl Pts',(58.6126930842203,252.069200807589,19.3950243599491)) ;
#94654=CARTESIAN_POINT('Ctrl Pts',(58.5381062355785,251.991630485002,19.3207516809529)) ;
#94655=CARTESIAN_POINT('Ctrl Pts',(58.6203761977389,252.077191235786,19.6048193809459)) ;
#94656=CARTESIAN_POINT('Ctrl Pts',(58.6205836533543,252.077409571898,19.519006774521)) ;
#94657=CARTESIAN_POINT('Ctrl Pts',(58.5800900326603,252.034790418159,19.4335598510852)) ;
#94658=CARTESIAN_POINT('Ctrl Pts',(58.5108234404051,251.963260236624,19.3777695274782)) ;
#94659=CARTESIAN_POINT('Ctrl Pts',(58.599917094062,252.026292564171,19.6046716026803)) ;
#94660=CARTESIAN_POINT('Ctrl Pts',(58.6000890621805,252.026517346894,19.5381801383464)) ;
#94661=CARTESIAN_POINT('Ctrl Pts',(58.5665185027056,251.982640513062,19.4721422791318)) ;
#94662=CARTESIAN_POINT('Ctrl Pts',(58.5120777999854,251.908453143741,19.4337397059719)) ;
#94663=CARTESIAN_POINT('Ctrl Pts',(58.5999998252129,251.97513584248,19.6045649427454)) ;
#94664=CARTESIAN_POINT('Ctrl Pts',(58.6001105321248,251.975366917946,19.5520192504951)) ;
#94665=CARTESIAN_POINT('Ctrl Pts',(58.5785017471512,251.930263457254,19.4997602590865)) ;
#94666=CARTESIAN_POINT('Ctrl Pts',(58.5413122444863,251.852672635479,19.4626317919105)) ;
#94667=CARTESIAN_POINT('',(58.5414213562373,251.853601400224,19.4627416997969)) ;
#94668=CARTESIAN_POINT('Origin',(58.4,251.55944497925,19.6041630560343)) ;
#94669=CARTESIAN_POINT('Origin',(58.6828427124746,251.853601400224,19.3213203435596)) ;
#94670=CARTESIAN_POINT('Origin',(58.3256944230447,251.482167179217,18.9641720541297)) ;
#94671=CARTESIAN_POINT('',(57.3360353944838,250.6,18.2573557380434)) ;
#94672=CARTESIAN_POINT('',(58.1842730668074,251.482167179217,19.105593410367)) ;
#94673=CARTESIAN_POINT('Ctrl Pts',(57.3360353944838,250.6,18.2573557380434)) ;
#94674=CARTESIAN_POINT('Ctrl Pts',(57.3181896909239,250.6,18.2395100344835)) ;
#94675=CARTESIAN_POINT('Ctrl Pts',(57.3005245771568,250.599676577703,18.2194780649264)) ;
#94676=CARTESIAN_POINT('Ctrl Pts',(57.2777853264116,250.601948658739,18.1885691056682)) ;
#94677=CARTESIAN_POINT('Ctrl Pts',(57.2699676956912,250.603347306435,18.1767561178791)) ;
#94678=CARTESIAN_POINT('Ctrl Pts',(57.2610778226503,250.60716749495,18.1601317033773)) ;
#94679=CARTESIAN_POINT('Ctrl Pts',(57.2586681750948,250.608544938818,18.1551388788019)) ;
#94680=CARTESIAN_POINT('Ctrl Pts',(57.2549670712099,250.611595514249,18.1461752289758)) ;
#94681=CARTESIAN_POINT('Ctrl Pts',(57.2535461821065,250.613147135549,18.142207243288)) ;
#94682=CARTESIAN_POINT('Ctrl Pts',(57.2524006549569,250.6149414558,18.1382539013022)) ;
#94683=CARTESIAN_POINT('Origin',(58.4,245.5625,19.6041630560343)) ;
#94684=CARTESIAN_POINT('',(58.5414213562374,245.458578643763,19.4627416997969)) ;
#94685=CARTESIAN_POINT('Origin',(58.4,245.6,19.6041630560343)) ;
#94686=CARTESIAN_POINT('',(58.5414213562374,245.5625,19.4627416997969)) ;
#94687=CARTESIAN_POINT('Origin',(66.25,251.8,20.0213203435596)) ;
#94688=CARTESIAN_POINT('Ctrl Pts',(57.3360353944838,250.6,18.2573557380434)) ;
#94689=CARTESIAN_POINT('Ctrl Pts',(57.3340473556883,250.6,18.255367699248)) ;
#94690=CARTESIAN_POINT('Ctrl Pts',(57.3300486483845,250.6,18.2513689919442)) ;
#94691=CARTESIAN_POINT('Ctrl Pts',(57.3219725324425,250.6,18.2432928760022)) ;
#94692=CARTESIAN_POINT('Ctrl Pts',(57.2953493638287,250.6,18.2166697073883)) ;
#94693=CARTESIAN_POINT('Ctrl Pts',(57.2571236188557,250.6,18.1784439624154)) ;
#94694=CARTESIAN_POINT('Ctrl Pts',(57.207773891194,250.6,18.1290942347537)) ;
#94695=CARTESIAN_POINT('Ctrl Pts',(57.1830512714168,250.6,18.1043716149764)) ;
#94696=CARTESIAN_POINT('Ctrl Pts',(57.1734725423205,250.6,18.0947928858801)) ;
#94697=CARTESIAN_POINT('Ctrl Pts',(57.3333527411373,250.592253069194,18.194783093941)) ;
#94698=CARTESIAN_POINT('Ctrl Pts',(57.3316948915604,250.59291821646,18.1930083348525)) ;
#94699=CARTESIAN_POINT('Ctrl Pts',(57.3283033876591,250.594238062535,18.1894701538716)) ;
#94700=CARTESIAN_POINT('Ctrl Pts',(57.3212436334276,250.596857460934,18.1824465273365)) ;
#94701=CARTESIAN_POINT('Ctrl Pts',(57.2969689913209,250.605207915463,18.1598768130777)) ;
#94702=CARTESIAN_POINT('Ctrl Pts',(57.2569809892506,250.614379141446,18.1302403683433)) ;
#94703=CARTESIAN_POINT('Ctrl Pts',(57.2003714037071,250.618567551195,18.0947534362098)) ;
#94704=CARTESIAN_POINT('Ctrl Pts',(57.170211619543,250.615028729546,18.078006465602)) ;
#94705=CARTESIAN_POINT('Ctrl Pts',(57.1582126167144,250.61077488758,18.0719249151656)) ;
#94706=CARTESIAN_POINT('Ctrl Pts',(57.3362613117172,250.64045272393,18.0627210228977)) ;
#94707=CARTESIAN_POINT('Ctrl Pts',(57.3344481626957,250.641874746874,18.0621160423691)) ;
#94708=CARTESIAN_POINT('Ctrl Pts',(57.3306964101622,250.644659791177,18.0609462582947)) ;
#94709=CARTESIAN_POINT('Ctrl Pts',(57.3227262302857,250.64994988976,18.0587275800888)) ;
#94710=CARTESIAN_POINT('Ctrl Pts',(57.294574348591,250.665713573551,18.052155533589)) ;
#94711=CARTESIAN_POINT('Ctrl Pts',(57.2451381515996,250.678074698665,18.0454508927218)) ;
#94712=CARTESIAN_POINT('Ctrl Pts',(57.1735021273919,250.671463165854,18.0378317708818)) ;
#94713=CARTESIAN_POINT('Ctrl Pts',(57.1349950092079,250.654089939879,18.0348746164525)) ;
#94714=CARTESIAN_POINT('Ctrl Pts',(57.1192875831677,250.63825948163,18.0346271738767)) ;
#94715=CARTESIAN_POINT('Ctrl Pts',(57.3530175024253,250.774455018098,18.0235461286619)) ;
#94716=CARTESIAN_POINT('Ctrl Pts',(57.3497024752754,250.775415195087,18.0236910929475)) ;
#94717=CARTESIAN_POINT('Ctrl Pts',(57.3430153907722,250.777175758591,18.0239599227483)) ;
#94718=CARTESIAN_POINT('Ctrl Pts',(57.3294481719789,250.780101722395,18.0244426251914)) ;
#94719=CARTESIAN_POINT('Ctrl Pts',(57.2843980090737,250.78649635771,18.0257611907679)) ;
#94720=CARTESIAN_POINT('Ctrl Pts',(57.2185876893421,250.779765247521,18.02518066019)) ;
#94721=CARTESIAN_POINT('Ctrl Pts',(57.1328468261104,250.741672390444,18.0222725008139)) ;
#94722=CARTESIAN_POINT('Ctrl Pts',(57.0890785776611,250.702463609168,18.0204629952553)) ;
#94723=CARTESIAN_POINT('Ctrl Pts',(57.0710662135815,250.672308129681,18.0213203435596)) ;
#94724=CARTESIAN_POINT('Ctrl Pts',(57.3614836315263,250.835788185648,18.0357573764341)) ;
#94725=CARTESIAN_POINT('Ctrl Pts',(57.3573995943998,250.836527612015,18.0359045939827)) ;
#94726=CARTESIAN_POINT('Ctrl Pts',(57.3492123791771,250.837811031858,18.0361634130032)) ;
#94727=CARTESIAN_POINT('Ctrl Pts',(57.3327905714109,250.839665322753,18.0365310164789)) ;
#94728=CARTESIAN_POINT('Ctrl Pts',(57.2791569903834,250.841940496107,18.0370590762059)) ;
#94729=CARTESIAN_POINT('Ctrl Pts',(57.2051851586706,250.827317494238,18.0336777240699)) ;
#94730=CARTESIAN_POINT('Ctrl Pts',(57.112442265655,250.775538088749,18.0255551391046)) ;
#94731=CARTESIAN_POINT('Ctrl Pts',(57.0661025428336,250.726337647705,18.0213203435596)) ;
#94732=CARTESIAN_POINT('Ctrl Pts',(57.046945084641,250.68933982822,18.0213203435596)) ;
#94733=CARTESIAN_POINT('',(57.1734725423205,250.6,18.0947928858801)) ;
#94734=CARTESIAN_POINT('',(59.35,250.6,20.2713203435596)) ;
#94735=CARTESIAN_POINT('Origin',(57.046945084641,250.68933982822,18.2213203435596)) ;
#94736=CARTESIAN_POINT('Ctrl Pts',(57.1734725423205,250.6,18.0947928858801)) ;
#94737=CARTESIAN_POINT('Ctrl Pts',(57.1731461743363,250.6,18.0944665178959)) ;
#94738=CARTESIAN_POINT('Ctrl Pts',(57.1725010996802,250.6,18.0938214432399)) ;
#94739=CARTESIAN_POINT('Ctrl Pts',(57.1712430810202,250.6,18.0925634245799)) ;
#94740=CARTESIAN_POINT('Ctrl Pts',(57.1691302969587,250.6,18.0904506405183)) ;
#94741=CARTESIAN_POINT('Ctrl Pts',(57.1669367401687,250.6,18.0882570837283)) ;
#94742=CARTESIAN_POINT('Ctrl Pts',(57.1649991631621,250.6,18.0863195067217)) ;
#94743=CARTESIAN_POINT('Ctrl Pts',(57.1604293063194,250.6,18.0817496498791)) ;
#94744=CARTESIAN_POINT('Ctrl Pts',(57.1584079275307,250.6,18.0797282710903)) ;
#94745=CARTESIAN_POINT('Ctrl Pts',(57.1585946892593,250.599997334071,18.0799134496435)) ;
#94746=CARTESIAN_POINT('Ctrl Pts',(57.1429446492179,250.621555453462,18.0490448931659)) ;
#94747=CARTESIAN_POINT('Ctrl Pts',(57.1424797946325,250.621375921649,18.0489088621478)) ;
#94748=CARTESIAN_POINT('Ctrl Pts',(57.1415607216988,250.621008706217,18.0486394209038)) ;
#94749=CARTESIAN_POINT('Ctrl Pts',(57.1397653075042,250.620246901795,18.0481166236226)) ;
#94750=CARTESIAN_POINT('Ctrl Pts',(57.1367454202683,250.61883616044,18.0472382453025)) ;
#94751=CARTESIAN_POINT('Ctrl Pts',(57.1335982829151,250.617060962106,18.0463315951316)) ;
#94752=CARTESIAN_POINT('Ctrl Pts',(57.1308083691544,250.615146586166,18.045539816041)) ;
#94753=CARTESIAN_POINT('Ctrl Pts',(57.1242109639996,250.609962299049,18.0436867512443)) ;
#94754=CARTESIAN_POINT('Ctrl Pts',(57.1212989029449,250.60431006208,18.0427897179726)) ;
#94755=CARTESIAN_POINT('Ctrl Pts',(57.1215631814552,250.5993051408,18.0428708220856)) ;
#94756=CARTESIAN_POINT('Ctrl Pts',(57.0951621692686,250.655294205737,18.0213057277848)) ;
#94757=CARTESIAN_POINT('Ctrl Pts',(57.094601304706,250.654745987511,18.0213088809629)) ;
#94758=CARTESIAN_POINT('Ctrl Pts',(57.0934927123476,250.653637902561,18.0213139894636)) ;
#94759=CARTESIAN_POINT('Ctrl Pts',(57.0913291481799,250.651379993583,18.0213249675951)) ;
#94760=CARTESIAN_POINT('Ctrl Pts',(57.0876937748347,250.647315907814,18.0213383959865)) ;
#94761=CARTESIAN_POINT('Ctrl Pts',(57.0839139948312,250.642433992342,18.0213487187058)) ;
#94762=CARTESIAN_POINT('Ctrl Pts',(57.0805700602664,250.637351731764,18.0213615345955)) ;
#94763=CARTESIAN_POINT('Ctrl Pts',(57.0726744213749,250.62385451521,18.0213962624513)) ;
#94764=CARTESIAN_POINT('Ctrl Pts',(57.0691959132974,250.610399542745,18.0213013549948)) ;
#94765=CARTESIAN_POINT('Ctrl Pts',(57.069511625002,250.598324499523,18.0213095441839)) ;
#94766=CARTESIAN_POINT('Ctrl Pts',(57.0469069494654,250.689366755103,18.0213203493371)) ;
#94767=CARTESIAN_POINT('Ctrl Pts',(57.0462541408344,250.688442020775,18.0213203468729)) ;
#94768=CARTESIAN_POINT('Ctrl Pts',(57.0449638479257,250.686578176133,18.0213203428908)) ;
#94769=CARTESIAN_POINT('Ctrl Pts',(57.0424475318287,250.682795217849,18.0213203343216)) ;
#94770=CARTESIAN_POINT('Ctrl Pts',(57.0382214969108,250.676032304701,18.0213203238896)) ;
#94771=CARTESIAN_POINT('Ctrl Pts',(57.0338339029805,250.66799976973,18.0213203159184)) ;
#94772=CARTESIAN_POINT('Ctrl Pts',(57.029958328817,250.659709674647,18.0213203059525)) ;
#94773=CARTESIAN_POINT('Ctrl Pts',(57.020817631172,250.637802853616,18.0213202788865)) ;
#94774=CARTESIAN_POINT('Ctrl Pts',(57.0167744273248,250.616535402224,18.0213203540969)) ;
#94775=CARTESIAN_POINT('Ctrl Pts',(57.0171413288756,250.597336706409,18.0213203476065)) ;
#94776=CARTESIAN_POINT('',(57.1585786437627,250.6,18.0798989873223)) ;
#94777=CARTESIAN_POINT('Origin',(57.0171572875254,250.6,18.2213203435596)) ;
#94778=CARTESIAN_POINT('',(59.35,250.6,20.2713203435596)) ;
#94779=CARTESIAN_POINT('Origin',(57.0171572875254,247.8875,18.2213203435596)) ;
#94780=CARTESIAN_POINT('',(57.1585786437627,247.8875,18.0798989873223)) ;
#94781=CARTESIAN_POINT('Origin',(57.85,246.725,18.7713203435596)) ;
#94782=CARTESIAN_POINT('',(59.4894251848905,244.51057481511,20.4107455284501)) ;
#94783=CARTESIAN_POINT('',(59.0458333333334,244.954166666667,19.967153676893)) ;
#94784=CARTESIAN_POINT('Origin',(59.7722678973651,244.793417527584,20.6935882409247)) ;
#94785=CARTESIAN_POINT('Origin',(59.7,253.2,24.0213203435596)) ;
#94786=CARTESIAN_POINT('',(59.7,253.2,24.0213203435596)) ;
#94787=CARTESIAN_POINT('',(61.2,253.2,24.0213203435596)) ;
#94788=CARTESIAN_POINT('',(59.7,253.2,24.0213203435596)) ;
#94789=CARTESIAN_POINT('Origin',(66.95,251.85,24.0213203435596)) ;
#94790=CARTESIAN_POINT('',(66.7875,252.0125,23.0213203435596)) ;
#94791=CARTESIAN_POINT('',(66.975,251.825,24.0213203435596)) ;
#94792=CARTESIAN_POINT('Origin',(69.2696458032277,238.278291754874,16.7713203435596)) ;
#94793=CARTESIAN_POINT('',(80.6144201366714,238.515462579386,16.0598078700218)) ;
#94794=CARTESIAN_POINT('Ctrl Pts',(80.5752025501715,238.278291754874,16.0213203435596)) ;
#94795=CARTESIAN_POINT('Ctrl Pts',(80.5895127461922,238.355434329238,16.0213203435596)) ;
#94796=CARTESIAN_POINT('Ctrl Pts',(80.6030553487399,238.437267187051,16.0337427392433)) ;
#94797=CARTESIAN_POINT('Ctrl Pts',(80.6144201366714,238.515462579386,16.0598078700215)) ;
#94798=CARTESIAN_POINT('',(69.2696458032277,238.515462579386,16.0598078700217)) ;
#94799=CARTESIAN_POINT('Origin',(74.5283628290597,239.4,16.0213203435596)) ;
#94800=CARTESIAN_POINT('Ctrl Pts',(68.442305521448,238.515462579386,16.0598078700215)) ;
#94801=CARTESIAN_POINT('Ctrl Pts',(68.4536700072495,238.437269265856,16.0337434321782)) ;
#94802=CARTESIAN_POINT('Ctrl Pts',(68.4672116831744,238.355440953127,16.0213203435596)) ;
#94803=CARTESIAN_POINT('Ctrl Pts',(68.4815231079478,238.278291754874,16.0213203435596)) ;
#94804=CARTESIAN_POINT('',(73.6283628290596,245.483789937202,18.5213203435596)) ;
#94805=CARTESIAN_POINT('',(73.6283628290596,245.483789937202,16.0213203435596)) ;
#94806=CARTESIAN_POINT('',(75.4283628290596,245.483789937202,18.5213203435596)) ;
#94807=CARTESIAN_POINT('Origin',(74.5283628290597,239.4,18.5213203435596)) ;
#94808=CARTESIAN_POINT('',(75.4283628290596,245.483789937202,16.0213203435596)) ;
#94809=CARTESIAN_POINT('',(78.2651788784023,244.284537420614,17.9828328170975)) ;
#94810=CARTESIAN_POINT('Ctrl Pts',(78.2651788784023,244.284537420614,17.9828328170977)) ;
#94811=CARTESIAN_POINT('Ctrl Pts',(78.2318038761366,244.310070287572,17.9913437727504)) ;
#94812=CARTESIAN_POINT('Ctrl Pts',(78.1978897752054,244.335468004199,17.9982799362105)) ;
#94813=CARTESIAN_POINT('Ctrl Pts',(78.1637671894526,244.360475493408,18.0037846770076)) ;
#94814=CARTESIAN_POINT('Ctrl Pts',(78.1291333505218,244.385857665779,18.0093718944449)) ;
#94815=CARTESIAN_POINT('Ctrl Pts',(78.0942847325789,244.410837421656,18.013485084683)) ;
#94816=CARTESIAN_POINT('Ctrl Pts',(78.059567033835,244.43518585183,18.0163128773869)) ;
#94817=CARTESIAN_POINT('Ctrl Pts',(78.0239386127422,244.460172995408,18.0192148493742)) ;
#94818=CARTESIAN_POINT('Ctrl Pts',(77.9884480695404,244.484494937463,18.0207637869309)) ;
#94819=CARTESIAN_POINT('Ctrl Pts',(77.9534690276318,244.507949572025,18.0211941322164)) ;
#94820=CARTESIAN_POINT('Ctrl Pts',(77.9465787317034,244.512569749257,18.0212789031594)) ;
#94821=CARTESIAN_POINT('Ctrl Pts',(77.9397082833141,244.517156417629,18.0213203435596)) ;
#94822=CARTESIAN_POINT('Ctrl Pts',(77.9328605382387,244.521708245126,18.0213203435596)) ;
#94823=CARTESIAN_POINT('Origin',(74.5283628290597,239.4,16.3546536768929)) ;
#94824=CARTESIAN_POINT('Origin',(66.95,251.85,24.0213203435596)) ;
#94825=CARTESIAN_POINT('Origin',(61.8303059750075,244.521708245126,17.2713203435596)) ;
#94826=CARTESIAN_POINT('',(61.8303059750075,244.284537420614,17.9828328170975)) ;
#94827=CARTESIAN_POINT('Origin',(59.7,242.,24.0213203435596)) ;
#94828=CARTESIAN_POINT('',(59.7,242.,24.0213203435596)) ;
#94829=CARTESIAN_POINT('Origin',(69.2696458032277,238.278291754874,16.7713203435596)) ;
#94830=CARTESIAN_POINT('Origin',(60.5916108526749,220.645409008718,23.3713203435596)) ;
#94831=CARTESIAN_POINT('',(60.5916108526749,219.647053884905,30.7213203435596)) ;
#94832=CARTESIAN_POINT('',(60.5916108526749,220.125049696322,30.7213203435596)) ;
#94833=CARTESIAN_POINT('',(60.5916108526749,227.303573749953,30.7213203435596)) ;
#94834=CARTESIAN_POINT('',(60.5916108526749,219.647053884905,23.3713203435596)) ;
#94835=CARTESIAN_POINT('',(60.5916108526749,219.647053884905,23.3713203435596)) ;
#94836=CARTESIAN_POINT('',(60.5916108526749,220.645409008718,23.3713203435596)) ;
#94837=CARTESIAN_POINT('',(60.5916108526749,220.645409008718,23.3713203435596)) ;
#94838=CARTESIAN_POINT('',(60.5916108526749,220.645409008718,23.3713203435596)) ;
#94839=CARTESIAN_POINT('',(60.5916108526749,220.125049696322,27.0463203435596)) ;
#94840=CARTESIAN_POINT('Origin',(64.1568347953872,220.146231446812,23.3713203435596)) ;
#94841=CARTESIAN_POINT('',(63.1200364144528,223.593701405679,23.3713203435596)) ;
#94842=CARTESIAN_POINT('Origin',(64.1568347953872,220.146231446812,23.3713203435596)) ;
#94843=CARTESIAN_POINT('',(63.1200364144528,223.593701405679,23.3713203435596)) ;
#94844=CARTESIAN_POINT('Origin',(70.3850625789433,219.622496965577,23.3713203435596)) ;
#94845=CARTESIAN_POINT('',(67.2791272966079,221.938238572027,23.3713203435596)) ;
#94846=CARTESIAN_POINT('',(67.2791272966079,221.938238572027,23.3713203435596)) ;
#94847=CARTESIAN_POINT('',(70.3850625789433,219.622496965577,23.3713203435596)) ;
#94848=CARTESIAN_POINT('',(64.9830939940346,223.650128668,23.3713203435596)) ;
#94849=CARTESIAN_POINT('',(70.3850625789433,219.622496965577,23.3713203435596)) ;
#94850=CARTESIAN_POINT('Ctrl Pts',(84.4412221473412,189.289539758744,23.1313203435596)) ;
#94851=CARTESIAN_POINT('Ctrl Pts',(84.4412221473412,189.289539758744,30.7993203435596)) ;
#94852=CARTESIAN_POINT('Ctrl Pts',(83.8416464716194,189.870585945118,23.1313203435596)) ;
#94853=CARTESIAN_POINT('Ctrl Pts',(83.8416464716194,189.870585945118,30.7993203435596)) ;
#94854=CARTESIAN_POINT('Ctrl Pts',(82.6693997344123,191.034842241154,23.1313203435596)) ;
#94855=CARTESIAN_POINT('Ctrl Pts',(82.6693997344123,191.034842241154,30.7993203435596)) ;
#94856=CARTESIAN_POINT('Ctrl Pts',(80.9917381958488,192.787718030768,23.1313203435596)) ;
#94857=CARTESIAN_POINT('Ctrl Pts',(80.9917381958488,192.787718030768,30.7993203435596)) ;
#94858=CARTESIAN_POINT('Ctrl Pts',(78.9189744912756,195.138085698398,23.1313203435596)) ;
#94859=CARTESIAN_POINT('Ctrl Pts',(78.9189744912756,195.138085698398,30.7993203435596)) ;
#94860=CARTESIAN_POINT('Ctrl Pts',(76.6209129092212,198.099602509355,23.1313203435596)) ;
#94861=CARTESIAN_POINT('Ctrl Pts',(76.6209129092212,198.099602509355,30.7993203435596)) ;
#94862=CARTESIAN_POINT('Ctrl Pts',(74.6447403893034,201.087008680127,23.1313203435596)) ;
#94863=CARTESIAN_POINT('Ctrl Pts',(74.6447403893034,201.087008680127,30.7993203435596)) ;
#94864=CARTESIAN_POINT('Ctrl Pts',(73.0215367693529,204.102803944955,23.1313203435596)) ;
#94865=CARTESIAN_POINT('Ctrl Pts',(73.0215367693529,204.102803944955,30.7993203435596)) ;
#94866=CARTESIAN_POINT('Ctrl Pts',(71.775922405272,207.148968505506,23.1313203435596)) ;
#94867=CARTESIAN_POINT('Ctrl Pts',(71.775922405272,207.148968505506,30.7993203435596)) ;
#94868=CARTESIAN_POINT('Ctrl Pts',(70.9055309357216,210.225312036653,23.1313203435596)) ;
#94869=CARTESIAN_POINT('Ctrl Pts',(70.9055309357216,210.225312036653,30.7993203435596)) ;
#94870=CARTESIAN_POINT('Ctrl Pts',(70.3872265023368,213.329973734064,23.1313203435596)) ;
#94871=CARTESIAN_POINT('Ctrl Pts',(70.3872265023368,213.329973734064,30.7993203435596)) ;
#94872=CARTESIAN_POINT('Ctrl Pts',(70.2337598673437,215.834709407061,23.1313203435596)) ;
#94873=CARTESIAN_POINT('Ctrl Pts',(70.2337598673437,215.834709407061,30.7993203435596)) ;
#94874=CARTESIAN_POINT('Ctrl Pts',(70.2566219573908,217.724357374766,23.1313203435596)) ;
#94875=CARTESIAN_POINT('Ctrl Pts',(70.2566219573908,217.724357374766,30.7993203435596)) ;
#94876=CARTESIAN_POINT('Ctrl Pts',(70.3321941673992,218.988975060904,23.1313203435596)) ;
#94877=CARTESIAN_POINT('Ctrl Pts',(70.3321941673992,218.988975060904,30.7993203435596)) ;
#94878=CARTESIAN_POINT('Ctrl Pts',(70.3850625789433,219.622496965577,23.1313203435596)) ;
#94879=CARTESIAN_POINT('Ctrl Pts',(70.3850625789433,219.622496965577,30.7993203435596)) ;
#94880=CARTESIAN_POINT('Ctrl Pts',(70.3850625789433,219.622496965577,23.3713203435596)) ;
#94881=CARTESIAN_POINT('Ctrl Pts',(70.3511634134941,219.216283439675,23.3713203435596)) ;
#94882=CARTESIAN_POINT('Ctrl Pts',(70.3247009237789,218.810668041503,23.3713203435596)) ;
#94883=CARTESIAN_POINT('Ctrl Pts',(70.3057017675343,218.40565291513,23.3713203435596)) ;
#94884=CARTESIAN_POINT('Ctrl Pts',(70.3024116855331,218.335516485894,23.3713203435596)) ;
#94885=CARTESIAN_POINT('Ctrl Pts',(70.2993455385549,218.265398067628,23.3713203435596)) ;
#94886=CARTESIAN_POINT('Ctrl Pts',(70.2965036217263,218.19529768407,23.3713203435596)) ;
#94887=CARTESIAN_POINT('Origin',(64.1568347953872,220.146231446812,23.3713203435596)) ;
#94888=CARTESIAN_POINT('',(60.6037668263229,219.566828299419,30.7213203435596)) ;
#94889=CARTESIAN_POINT('Origin',(64.1568347953872,220.146231446812,30.7213203435596)) ;
#94890=CARTESIAN_POINT('',(60.6037668263229,219.566828299419,23.3713203435596)) ;
#94891=CARTESIAN_POINT('',(60.6037668263229,219.566828299419,23.3713203435596)) ;
#94892=CARTESIAN_POINT('Origin',(64.1568347953872,220.146231446812,23.3713203435596)) ;
#94893=CARTESIAN_POINT('Origin',(64.1568347953872,220.146231446812,23.3713203435596)) ;
#94894=CARTESIAN_POINT('',(64.9830939940346,223.650128668,23.3713203435596)) ;
#94895=CARTESIAN_POINT('',(64.9830939940346,223.650128668,23.3713203435596)) ;
#94896=CARTESIAN_POINT('Origin',(64.1568347953872,220.146231446812,23.3713203435596)) ;
#94897=CARTESIAN_POINT('Origin',(57.4999031800138,224.540465846463,30.7213203435596)) ;
#94898=CARTESIAN_POINT('',(57.4999031800138,224.540465846463,30.7213203435596)) ;
#94899=CARTESIAN_POINT('',(57.4999031800138,224.540465846463,30.7213203435596)) ;
#94900=CARTESIAN_POINT('',(57.4999031800138,224.540465846463,30.7213203435596)) ;
#94901=CARTESIAN_POINT('Origin',(70.9999999999998,217.633222662033,29.5213203435596)) ;
#94902=CARTESIAN_POINT('',(63.8582048387328,224.775017823302,23.3713203435596)) ;
#94903=CARTESIAN_POINT('',(63.8582048387328,224.775017823302,29.5213203435596)) ;
#94904=CARTESIAN_POINT('',(69.0112682894225,219.621954372611,23.3713203435596)) ;
#94905=CARTESIAN_POINT('Origin',(63.8582048387328,224.775017823302,29.5213203435596)) ;
#94906=CARTESIAN_POINT('',(63.0838307469447,223.535760225819,23.3713203435596)) ;
#94907=CARTESIAN_POINT('Origin',(65.632121620491,220.220271124835,23.3713203435596)) ;
#94908=CARTESIAN_POINT('',(60.321811570171,219.115605567354,23.3713203435596)) ;
#94909=CARTESIAN_POINT('',(63.0838307469447,223.535760225819,23.3713203435596)) ;
#94910=CARTESIAN_POINT('',(61.3703326482681,217.618162279643,23.3713203435596)) ;
#94911=CARTESIAN_POINT('',(60.9479927510422,218.221326162033,23.3713203435596)) ;
#94912=CARTESIAN_POINT('',(63.3614933659283,216.167053742856,23.3713203435596)) ;
#94913=CARTESIAN_POINT('Origin',(64.4831104165663,219.797752737776,23.3713203435596)) ;
#94914=CARTESIAN_POINT('',(69.4079308494226,215.768555109772,23.3713203435596)) ;
#94915=CARTESIAN_POINT('',(67.38212743034,215.902068421636,23.3713203435596)) ;
#94916=CARTESIAN_POINT('Origin',(69.4999999999997,217.165524426368,23.3713203435596)) ;
#94917=CARTESIAN_POINT('',(62.9568347953872,216.946231446812,23.3713203435596)) ;
#94918=CARTESIAN_POINT('',(65.4944782079391,216.946231446812,23.3713203435596)) ;
#94919=CARTESIAN_POINT('',(62.9568347953872,218.583251285823,23.3713203435596)) ;
#94920=CARTESIAN_POINT('Origin',(64.4831104165663,219.797752737776,23.2713203435596)) ;
#94921=CARTESIAN_POINT('Origin',(61.3703326482681,217.618162279643,23.2713203435596)) ;
#94922=CARTESIAN_POINT('Origin',(63.3615337725872,216.167062621809,23.271302987489)) ;
#94923=CARTESIAN_POINT('Origin',(67.38212743034,215.902068421636,23.2713203435596)) ;
#94924=CARTESIAN_POINT('Origin',(69.4079308494226,215.768555109772,23.2713203435596)) ;
#94925=CARTESIAN_POINT('Origin',(69.4999999999997,217.165524426368,23.2713203435596)) ;
#94926=CARTESIAN_POINT('Origin',(60.9479927510422,218.221326162033,23.2713203435596)) ;
#94927=CARTESIAN_POINT('Origin',(60.321811570171,219.115605567354,23.2713203435596)) ;
#94928=CARTESIAN_POINT('Origin',(63.8582048387328,224.775017823302,29.5213203435596)) ;
#94929=CARTESIAN_POINT('',(60.2066749117936,218.931348397394,30.7213203435596)) ;
#94930=CARTESIAN_POINT('Origin',(28.3,247.7,21.7213203435596)) ;
#94931=CARTESIAN_POINT('',(31.,247.7,26.7213203435596)) ;
#94932=CARTESIAN_POINT('',(27.3,247.7,26.7213203435596)) ;
#94933=CARTESIAN_POINT('',(31.,247.7,21.7213203435596)) ;
#94934=CARTESIAN_POINT('',(31.,247.7,21.7213203435596)) ;
#94935=CARTESIAN_POINT('',(27.3,247.7,21.7213203435596)) ;
#94936=CARTESIAN_POINT('Origin',(28.3,245.7,26.7213203435596)) ;
#94937=CARTESIAN_POINT('',(31.,245.7,21.7213203435596)) ;
#94938=CARTESIAN_POINT('',(27.3,245.7,21.7213203435596)) ;
#94939=CARTESIAN_POINT('',(31.,245.7,26.7213203435596)) ;
#94940=CARTESIAN_POINT('',(31.,245.7,26.7213203435596)) ;
#94941=CARTESIAN_POINT('',(27.3,245.7,26.7213203435596)) ;
#94942=CARTESIAN_POINT('Origin',(31.,246.7,24.2213203435596)) ;
#94943=CARTESIAN_POINT('',(31.,249.25,26.7213203435596)) ;
#94944=CARTESIAN_POINT('',(31.,245.9,21.7213203435596)) ;
#94945=CARTESIAN_POINT('Origin',(26.3,251.8,26.7213203435596)) ;
#94946=CARTESIAN_POINT('',(31.8,251.8,26.7213203435596)) ;
#94947=CARTESIAN_POINT('Origin',(26.3,251.8,21.7213203435596)) ;
#94948=CARTESIAN_POINT('',(31.8,251.8,21.7213203435596)) ;
#94949=CARTESIAN_POINT('Origin',(26.3,245.1,21.7213203435596)) ;
#94950=CARTESIAN_POINT('',(31.8,245.1,21.7213203435596)) ;
#94951=CARTESIAN_POINT('Origin',(31.8,248.45,24.2213203435596)) ;
#94952=CARTESIAN_POINT('Origin',(31.6354870749573,258.344201743738,20.2213203435596)) ;
#94953=CARTESIAN_POINT('',(31.5632689765959,258.377877596062,20.3213203435596)) ;
#94954=CARTESIAN_POINT('',(31.9729281400346,258.186850390917,20.3213203435596)) ;
#94955=CARTESIAN_POINT('',(31.6354870749573,258.344201743738,20.3213203435596)) ;
#94956=CARTESIAN_POINT('',(31.8391836130389,258.138878696195,20.2213203435596)) ;
#94957=CARTESIAN_POINT('Ctrl Pts',(31.9729281400345,258.186850390917,20.3213203435596)) ;
#94958=CARTESIAN_POINT('Ctrl Pts',(31.9726024539967,258.186730118955,20.3213203435596)) ;
#94959=CARTESIAN_POINT('Ctrl Pts',(31.9722767429558,258.186609910221,20.3213194310587)) ;
#94960=CARTESIAN_POINT('Ctrl Pts',(31.9566232186436,258.18083617139,20.3212317767765)) ;
#94961=CARTESIAN_POINT('Ctrl Pts',(31.9410876688426,258.175272220085,20.3191272439651)) ;
#94962=CARTESIAN_POINT('Ctrl Pts',(31.9123178937877,258.165043736205,20.3111145572994)) ;
#94963=CARTESIAN_POINT('Ctrl Pts',(31.8985908679471,258.160195813954,20.3053444921507)) ;
#94964=CARTESIAN_POINT('Ctrl Pts',(31.8733668278068,258.151021378108,20.2891795517339)) ;
#94965=CARTESIAN_POINT('Ctrl Pts',(31.8626456130347,258.147058717567,20.2790419175932)) ;
#94966=CARTESIAN_POINT('Ctrl Pts',(31.8498697583427,258.142470666398,20.260741297088)) ;
#94967=CARTESIAN_POINT('Ctrl Pts',(31.8459410167225,258.14109113882,20.2532165079448)) ;
#94968=CARTESIAN_POINT('Ctrl Pts',(31.8406780156682,258.139281704229,20.2374755979539)) ;
#94969=CARTESIAN_POINT('Ctrl Pts',(31.8392887152522,258.138829692159,20.2294674434764)) ;
#94970=CARTESIAN_POINT('Ctrl Pts',(31.8392904312326,258.138828886053,20.2213204095382)) ;
#94971=CARTESIAN_POINT('',(31.3863264609896,258.350049454246,20.2213203435596)) ;
#94972=CARTESIAN_POINT('',(31.5932252487832,258.253570965035,20.2213203435596)) ;
#94973=CARTESIAN_POINT('Origin',(31.5632689765959,258.377877596062,20.2213203435596)) ;
#94974=CARTESIAN_POINT('Ctrl Pts',(31.8826961677427,258.229957132574,20.2213203435596)) ;
#94975=CARTESIAN_POINT('Ctrl Pts',(31.8082406667398,258.074105253142,20.2213203435596)) ;
#94976=CARTESIAN_POINT('Ctrl Pts',(31.6975075374418,257.838597906516,20.2213203435596)) ;
#94977=CARTESIAN_POINT('Ctrl Pts',(31.5516420000274,257.525488877785,20.2213203435596)) ;
#94978=CARTESIAN_POINT('Ctrl Pts',(31.4640838198982,257.326016007648,20.2213203435596)) ;
#94979=CARTESIAN_POINT('Ctrl Pts',(31.3867201416434,257.194870160616,20.2213203435596)) ;
#94980=CARTESIAN_POINT('Ctrl Pts',(31.318862957822,257.131020174664,20.2213203435596)) ;
#94981=CARTESIAN_POINT('Ctrl Pts',(31.1611331373571,257.060468743905,20.2213203435597)) ;
#94982=CARTESIAN_POINT('Ctrl Pts',(30.993693898815,257.054864391304,20.2213203435596)) ;
#94983=CARTESIAN_POINT('Ctrl Pts',(30.8701100175112,257.060056991359,20.2213203435596)) ;
#94984=CARTESIAN_POINT('Ctrl Pts',(31.8826961677427,258.229957132574,20.2512402735938)) ;
#94985=CARTESIAN_POINT('Ctrl Pts',(31.8082407435551,258.074105413933,20.2512402735938)) ;
#94986=CARTESIAN_POINT('Ctrl Pts',(31.6973456699681,257.838498509911,20.2512402735938)) ;
#94987=CARTESIAN_POINT('Ctrl Pts',(31.5514897050399,257.525395035868,20.2512402735938)) ;
#94988=CARTESIAN_POINT('Ctrl Pts',(31.4638702756497,257.325881332878,20.2512402735938)) ;
#94989=CARTESIAN_POINT('Ctrl Pts',(31.3865371441645,257.194796533992,20.2512402735938)) ;
#94990=CARTESIAN_POINT('Ctrl Pts',(31.3187416910112,257.131018868321,20.2512402735938)) ;
#94991=CARTESIAN_POINT('Ctrl Pts',(31.1611435563971,257.060513922087,20.2512402735938)) ;
#94992=CARTESIAN_POINT('Ctrl Pts',(30.9936750861112,257.054865181754,20.2512402735938)) ;
#94993=CARTESIAN_POINT('Ctrl Pts',(30.8701100175112,257.060056991359,20.2512402735938)) ;
#94994=CARTESIAN_POINT('Ctrl Pts',(31.905373394501,258.219123485359,20.3030172712892)) ;
#94995=CARTESIAN_POINT('Ctrl Pts',(31.8309118350413,258.063258924232,20.3030172712892)) ;
#94996=CARTESIAN_POINT('Ctrl Pts',(31.7201990688088,257.827925373884,20.3030172712892)) ;
#94997=CARTESIAN_POINT('Ctrl Pts',(31.5743763641736,257.514858199604,20.3030172712892)) ;
#94998=CARTESIAN_POINT('Ctrl Pts',(31.4869575684128,257.315781063247,20.3030172712892)) ;
#94999=CARTESIAN_POINT('Ctrl Pts',(31.4072395052171,257.179852665022,20.3030172712892)) ;
#95000=CARTESIAN_POINT('Ctrl Pts',(31.3325657749029,257.109128082676,20.3030172712892)) ;
#95001=CARTESIAN_POINT('Ctrl Pts',(31.1638934400229,257.034573409644,20.3030172712892)) ;
#95002=CARTESIAN_POINT('Ctrl Pts',(30.9941226236966,257.029692061861,20.3030172712892)) ;
#95003=CARTESIAN_POINT('Ctrl Pts',(30.8690549760692,257.034947005039,20.3030172712892)) ;
#95004=CARTESIAN_POINT('Ctrl Pts',(31.952680132801,258.196523521125,20.3213203435596)) ;
#95005=CARTESIAN_POINT('Ctrl Pts',(31.8782059784266,258.040632596048,20.3213203435596)) ;
#95006=CARTESIAN_POINT('Ctrl Pts',(31.7674438315788,257.805605128362,20.3213203435597)) ;
#95007=CARTESIAN_POINT('Ctrl Pts',(31.6217159097903,257.492628417029,20.3213203435597)) ;
#95008=CARTESIAN_POINT('Ctrl Pts',(31.5345531399074,257.294353655337,20.3213203435597)) ;
#95009=CARTESIAN_POINT('Ctrl Pts',(31.4499409446598,257.148483052797,20.3213203435597)) ;
#95010=CARTESIAN_POINT('Ctrl Pts',(31.361082299714,257.063458465252,20.3213203435597)) ;
#95011=CARTESIAN_POINT('Ctrl Pts',(31.1696575900964,256.980579035594,20.3213203435597)) ;
#95012=CARTESIAN_POINT('Ctrl Pts',(30.9950063112822,256.977180762913,20.3213203435596)) ;
#95013=CARTESIAN_POINT('Ctrl Pts',(30.866854064559,256.982565311094,20.3213203435596)) ;
#95014=CARTESIAN_POINT('Ctrl Pts',(31.9729281400347,258.186850390917,20.3213203435596)) ;
#95015=CARTESIAN_POINT('Ctrl Pts',(31.8984486030264,258.030948198793,20.3213203435596)) ;
#95016=CARTESIAN_POINT('Ctrl Pts',(31.7876480706037,257.796041134552,20.3213203435597)) ;
#95017=CARTESIAN_POINT('Ctrl Pts',(31.6419617369609,257.483103734415,20.3213203435597)) ;
#95018=CARTESIAN_POINT('Ctrl Pts',(31.5549020259439,257.28516805193,20.3213203435597)) ;
#95019=CARTESIAN_POINT('Ctrl Pts',(31.4681983211233,257.135048536644,20.3213203435597)) ;
#95020=CARTESIAN_POINT('Ctrl Pts',(31.373274891254,257.043911031634,20.3213203435597)) ;
#95021=CARTESIAN_POINT('Ctrl Pts',(31.1721258442632,256.957473430288,20.3213203435597)) ;
#95022=CARTESIAN_POINT('Ctrl Pts',(30.995382539195,256.954705208349,20.3213203435596)) ;
#95023=CARTESIAN_POINT('Ctrl Pts',(30.8659120407843,256.960145145257,20.3213203435596)) ;
#95024=CARTESIAN_POINT('',(30.965916234277,256.957946490344,20.3213203435596)) ;
#95025=CARTESIAN_POINT('Ctrl Pts',(31.9729281400347,258.186850390917,20.3213203435596)) ;
#95026=CARTESIAN_POINT('Ctrl Pts',(31.8984486030264,258.030948198793,20.3213203435596)) ;
#95027=CARTESIAN_POINT('Ctrl Pts',(31.7876480706037,257.796041134552,20.3213203435597)) ;
#95028=CARTESIAN_POINT('Ctrl Pts',(31.6419617369609,257.483103734415,20.3213203435597)) ;
#95029=CARTESIAN_POINT('Ctrl Pts',(31.5549020259439,257.28516805193,20.3213203435597)) ;
#95030=CARTESIAN_POINT('Ctrl Pts',(31.4681983211233,257.135048536644,20.3213203435597)) ;
#95031=CARTESIAN_POINT('Ctrl Pts',(31.373274891254,257.043911031634,20.3213203435597)) ;
#95032=CARTESIAN_POINT('Ctrl Pts',(31.2030784552785,256.970774360576,20.3213203435597)) ;
#95033=CARTESIAN_POINT('Ctrl Pts',(31.06278978041,256.958226134581,20.3213203435597)) ;
#95034=CARTESIAN_POINT('Ctrl Pts',(30.9659328929364,256.957945874245,20.3213203435597)) ;
#95035=CARTESIAN_POINT('',(30.8701100175112,257.060056991359,20.2213203435596)) ;
#95036=CARTESIAN_POINT('Ctrl Pts',(30.9659078630823,256.957945802006,20.3213203435596)) ;
#95037=CARTESIAN_POINT('Ctrl Pts',(30.965671039864,256.958187990349,20.3213203435596)) ;
#95038=CARTESIAN_POINT('Ctrl Pts',(30.9654342887815,256.958430251337,20.3213194300433)) ;
#95039=CARTESIAN_POINT('Ctrl Pts',(30.9538716458124,256.970269071732,20.3212302458049)) ;
#95040=CARTESIAN_POINT('Ctrl Pts',(30.9426060928688,256.982148587136,20.3190544364554)) ;
#95041=CARTESIAN_POINT('Ctrl Pts',(30.9218631652494,257.004280924155,20.31084455494)) ;
#95042=CARTESIAN_POINT('Ctrl Pts',(30.9120149894988,257.01490568464,20.3049218660286)) ;
#95043=CARTESIAN_POINT('Ctrl Pts',(30.8938674792948,257.034213340876,20.2884844231793)) ;
#95044=CARTESIAN_POINT('Ctrl Pts',(30.8861826729993,257.042373958168,20.2782727116012)) ;
#95045=CARTESIAN_POINT('Ctrl Pts',(30.8772600100429,257.052056353529,20.2600246370711)) ;
#95046=CARTESIAN_POINT('Ctrl Pts',(30.8745807988497,257.055014131683,20.2526227319016)) ;
#95047=CARTESIAN_POINT('Ctrl Pts',(30.8710246291092,257.05899573171,20.2371678111417)) ;
#95048=CARTESIAN_POINT('Ctrl Pts',(30.8701100175114,257.060056991359,20.2293097304074)) ;
#95049=CARTESIAN_POINT('Ctrl Pts',(30.8701100175114,257.060056991359,20.2213203435596)) ;
#95050=CARTESIAN_POINT('Ctrl Pts',(30.8701100175112,257.060056991359,20.2213203435596)) ;
#95051=CARTESIAN_POINT('Ctrl Pts',(30.8881460152925,257.059299176326,20.2213203435596)) ;
#95052=CARTESIAN_POINT('Ctrl Pts',(30.9060122530829,257.058797146371,20.2213203435596)) ;
#95053=CARTESIAN_POINT('Ctrl Pts',(30.9237874982588,257.058573241475,20.2213203435596)) ;
#95054=CARTESIAN_POINT('Ctrl Pts',(30.9414214994052,257.058351115751,20.2213203435596)) ;
#95055=CARTESIAN_POINT('Ctrl Pts',(30.958966057566,257.058402889749,20.2213203435596)) ;
#95056=CARTESIAN_POINT('Ctrl Pts',(30.9764494613066,257.058765569003,20.2213203435596)) ;
#95057=CARTESIAN_POINT('Ctrl Pts',(30.9937966530257,257.059125422647,20.2213203435596)) ;
#95058=CARTESIAN_POINT('Ctrl Pts',(31.0110837583664,257.059791597926,20.2213203435596)) ;
#95059=CARTESIAN_POINT('Ctrl Pts',(31.0282886130343,257.060812188465,20.2213203435596)) ;
#95060=CARTESIAN_POINT('Ctrl Pts',(31.0453745456915,257.06182572456,20.2213203435596)) ;
#95061=CARTESIAN_POINT('Ctrl Pts',(31.0623794450239,257.063189146832,20.2213203435596)) ;
#95062=CARTESIAN_POINT('Ctrl Pts',(31.0792307306913,257.064957006289,20.2213203435596)) ;
#95063=CARTESIAN_POINT('Ctrl Pts',(31.0960542072034,257.066721948302,20.2213203435596)) ;
#95064=CARTESIAN_POINT('Ctrl Pts',(31.1127246102277,257.068890521463,20.2213203435597)) ;
#95065=CARTESIAN_POINT('Ctrl Pts',(31.1291178321619,257.071517944538,20.2213203435597)) ;
#95066=CARTESIAN_POINT('Ctrl Pts',(31.1454306602944,257.074132482499,20.2213203435597)) ;
#95067=CARTESIAN_POINT('Ctrl Pts',(31.1614688636718,257.077202150573,20.2213203435597)) ;
#95068=CARTESIAN_POINT('Ctrl Pts',(31.1770596212641,257.080772665844,20.2213203435597)) ;
#95069=CARTESIAN_POINT('Ctrl Pts',(31.1923295505933,257.084269706673,20.2213203435597)) ;
#95070=CARTESIAN_POINT('Ctrl Pts',(31.2071697772336,257.088248157638,20.2213203435597)) ;
#95071=CARTESIAN_POINT('Ctrl Pts',(31.2213742220269,257.092729903584,20.2213203435597)) ;
#95072=CARTESIAN_POINT('Ctrl Pts',(31.2305286847959,257.095618293592,20.2213203435596)) ;
#95073=CARTESIAN_POINT('Ctrl Pts',(31.2396247906868,257.098783024267,20.2213203435596)) ;
#95074=CARTESIAN_POINT('Ctrl Pts',(31.2484400659356,257.102196823945,20.2213203435596)) ;
#95075=CARTESIAN_POINT('Ctrl Pts',(31.2564036162801,257.105280785005,20.2213203435596)) ;
#95076=CARTESIAN_POINT('Ctrl Pts',(31.2641382578939,257.108567681928,20.2213203435596)) ;
#95077=CARTESIAN_POINT('Ctrl Pts',(31.2715131924955,257.112021656713,20.2213203435596)) ;
#95078=CARTESIAN_POINT('Ctrl Pts',(31.2805359440217,257.11624736961,20.2213203435596)) ;
#95079=CARTESIAN_POINT('Ctrl Pts',(31.289364636101,257.120737569893,20.2213203435596)) ;
#95080=CARTESIAN_POINT('Ctrl Pts',(31.2978878243988,257.125497027665,20.2213203435596)) ;
#95081=CARTESIAN_POINT('Ctrl Pts',(31.3034204922576,257.12858654043,20.2213203435596)) ;
#95082=CARTESIAN_POINT('Ctrl Pts',(31.3088255627919,257.131789527954,20.2213203435596)) ;
#95083=CARTESIAN_POINT('Ctrl Pts',(31.3140842359417,257.135106517862,20.2213203435596)) ;
#95084=CARTESIAN_POINT('Ctrl Pts',(31.3251260171775,257.142071293174,20.2213203435596)) ;
#95085=CARTESIAN_POINT('Ctrl Pts',(31.335568121659,257.149562438639,20.2213203435596)) ;
#95086=CARTESIAN_POINT('Ctrl Pts',(31.3455081907556,257.157763710087,20.2213203435596)) ;
#95087=CARTESIAN_POINT('Ctrl Pts',(31.3542057512151,257.164939822604,20.2213203435596)) ;
#95088=CARTESIAN_POINT('Ctrl Pts',(31.3625183834661,257.172659779784,20.2213203435596)) ;
#95089=CARTESIAN_POINT('Ctrl Pts',(31.3705318439148,257.181079707773,20.2213203435596)) ;
#95090=CARTESIAN_POINT('Ctrl Pts',(31.3745857184255,257.185339207359,20.2213203435596)) ;
#95091=CARTESIAN_POINT('Ctrl Pts',(31.3785634161927,257.189778383009,20.2213203435596)) ;
#95092=CARTESIAN_POINT('Ctrl Pts',(31.3824791104723,257.194421183466,20.2213203435596)) ;
#95093=CARTESIAN_POINT('Ctrl Pts',(31.3856937678516,257.198232771319,20.2213203435596)) ;
#95094=CARTESIAN_POINT('Ctrl Pts',(31.3888701589267,257.202186788496,20.2213203435596)) ;
#95095=CARTESIAN_POINT('Ctrl Pts',(31.3919927963429,257.206263925275,20.2213203435596)) ;
#95096=CARTESIAN_POINT('Ctrl Pts',(31.3982423422826,257.214423775492,20.2213203435596)) ;
#95097=CARTESIAN_POINT('Ctrl Pts',(31.404285482801,257.223091327263,20.2213203435596)) ;
#95098=CARTESIAN_POINT('Ctrl Pts',(31.4101412935664,257.232211050084,20.2213203435596)) ;
#95099=CARTESIAN_POINT('Ctrl Pts',(31.4158483968946,257.241099178911,20.2213203435596)) ;
#95100=CARTESIAN_POINT('Ctrl Pts',(31.421379377071,257.250417334289,20.2213203435596)) ;
#95101=CARTESIAN_POINT('Ctrl Pts',(31.4267676789623,257.260069003584,20.2213203435596)) ;
#95102=CARTESIAN_POINT('Ctrl Pts',(31.4313169879582,257.268217846546,20.2213203435596)) ;
#95103=CARTESIAN_POINT('Ctrl Pts',(31.4357653406137,257.276603779098,20.2213203435596)) ;
#95104=CARTESIAN_POINT('Ctrl Pts',(31.4401282884918,257.285139319864,20.2213203435596)) ;
#95105=CARTESIAN_POINT('Ctrl Pts',(31.4425442454129,257.289865825741,20.2213203435596)) ;
#95106=CARTESIAN_POINT('Ctrl Pts',(31.4449324432114,257.294634794624,20.2213203435596)) ;
#95107=CARTESIAN_POINT('Ctrl Pts',(31.4472990616257,257.299438290958,20.2213203435596)) ;
#95108=CARTESIAN_POINT('Ctrl Pts',(31.453697048331,257.312424206006,20.2213203435596)) ;
#95109=CARTESIAN_POINT('Ctrl Pts',(31.459951086791,257.325681772639,20.2213203435596)) ;
#95110=CARTESIAN_POINT('Ctrl Pts',(31.4661895021085,257.339150167048,20.2213203435596)) ;
#95111=CARTESIAN_POINT('Ctrl Pts',(31.4728199784414,257.353464999555,20.2213203435596)) ;
#95112=CARTESIAN_POINT('Ctrl Pts',(31.479432120829,257.368017614714,20.2213203435596)) ;
#95113=CARTESIAN_POINT('Ctrl Pts',(31.4861192778588,257.382734893759,20.2213203435596)) ;
#95114=CARTESIAN_POINT('Ctrl Pts',(31.4934700853774,257.398912753046,20.2213203435596)) ;
#95115=CARTESIAN_POINT('Ctrl Pts',(31.5009109032352,257.415289051434,20.2213203435596)) ;
#95116=CARTESIAN_POINT('Ctrl Pts',(31.5085049435486,257.431774039478,20.2213203435596)) ;
#95117=CARTESIAN_POINT('Ctrl Pts',(31.5089271055015,257.432690460047,20.2213203435596)) ;
#95118=CARTESIAN_POINT('Ctrl Pts',(31.5093497283266,257.43360721947,20.2213203435596)) ;
#95119=CARTESIAN_POINT('Ctrl Pts',(31.509772818656,257.434524303432,20.2213203435596)) ;
#95120=CARTESIAN_POINT('Ctrl Pts',(31.5165025689967,257.449111604719,20.2213203435596)) ;
#95121=CARTESIAN_POINT('Ctrl Pts',(31.5233210366753,257.463886724714,20.2213203435596)) ;
#95122=CARTESIAN_POINT('Ctrl Pts',(31.5301544632509,257.478686862547,20.2213203435596)) ;
#95123=CARTESIAN_POINT('Ctrl Pts',(31.5365608006656,257.492561991765,20.2213203435596)) ;
#95124=CARTESIAN_POINT('Ctrl Pts',(31.5429807467931,257.506460149131,20.2213203435596)) ;
#95125=CARTESIAN_POINT('Ctrl Pts',(31.5493714042548,257.520287040577,20.2213203435596)) ;
#95126=CARTESIAN_POINT('Ctrl Pts',(31.5513920368639,257.52465890183,20.2213203435596)) ;
#95127=CARTESIAN_POINT('Ctrl Pts',(31.5534094887509,257.529023100625,20.2213203435596)) ;
#95128=CARTESIAN_POINT('Ctrl Pts',(31.5554299324024,257.533392951736,20.2213203435596)) ;
#95129=CARTESIAN_POINT('Ctrl Pts',(31.5633310508952,257.550481629959,20.2213203435596)) ;
#95130=CARTESIAN_POINT('Ctrl Pts',(31.5712513069425,257.567599094905,20.2213203435596)) ;
#95131=CARTESIAN_POINT('Ctrl Pts',(31.5791650505042,257.584687939887,20.2213203435596)) ;
#95132=CARTESIAN_POINT('Ctrl Pts',(31.587614982311,257.602934623473,20.2213203435596)) ;
#95133=CARTESIAN_POINT('Ctrl Pts',(31.5960576753152,257.621149119168,20.2213203435596)) ;
#95134=CARTESIAN_POINT('Ctrl Pts',(31.6044872091412,257.639316861752,20.2213203435596)) ;
#95135=CARTESIAN_POINT('Ctrl Pts',(31.6135924929299,257.658941013625,20.2213203435596)) ;
#95136=CARTESIAN_POINT('Ctrl Pts',(31.6226826149776,257.678511082707,20.2213203435596)) ;
#95137=CARTESIAN_POINT('Ctrl Pts',(31.6317756665799,257.698063905933,20.2213203435596)) ;
#95138=CARTESIAN_POINT('Ctrl Pts',(31.6403047005873,257.716403919992,20.2213203435596)) ;
#95139=CARTESIAN_POINT('Ctrl Pts',(31.6488368372567,257.734729927809,20.2213203435596)) ;
#95140=CARTESIAN_POINT('Ctrl Pts',(31.6574024333342,257.753105040464,20.2213203435596)) ;
#95141=CARTESIAN_POINT('Ctrl Pts',(31.6619174230045,257.762790699591,20.2213203435596)) ;
#95142=CARTESIAN_POINT('Ctrl Pts',(31.6664420477939,257.772490706991,20.2213203435596)) ;
#95143=CARTESIAN_POINT('Ctrl Pts',(31.6709701075337,257.782191437883,20.2213203435596)) ;
#95144=CARTESIAN_POINT('Ctrl Pts',(31.6842270030051,257.810592471177,20.2213203435596)) ;
#95145=CARTESIAN_POINT('Ctrl Pts',(31.6975227286466,257.839019902207,20.2213203435596)) ;
#95146=CARTESIAN_POINT('Ctrl Pts',(31.7108387516935,257.867425705876,20.2213203435596)) ;
#95147=CARTESIAN_POINT('Ctrl Pts',(31.7269899500257,257.901879518941,20.2213203435596)) ;
#95148=CARTESIAN_POINT('Ctrl Pts',(31.7431711953078,257.936302176977,20.2213203435596)) ;
#95149=CARTESIAN_POINT('Ctrl Pts',(31.7593838316716,257.970678860503,20.2213203435596)) ;
#95150=CARTESIAN_POINT('Ctrl Pts',(31.7845303488226,258.023998619393,20.2213203435596)) ;
#95151=CARTESIAN_POINT('Ctrl Pts',(31.8097554620621,258.077217498546,20.2213203435596)) ;
#95152=CARTESIAN_POINT('Ctrl Pts',(31.8351282490926,258.130384143046,20.2213203435596)) ;
#95153=CARTESIAN_POINT('Ctrl Pts',(31.836479618475,258.133215829429,20.2213203435596)) ;
#95154=CARTESIAN_POINT('Ctrl Pts',(31.8378314038708,258.136047348203,20.2213203435596)) ;
#95155=CARTESIAN_POINT('Ctrl Pts',(31.8391836130389,258.138878696195,20.2213203435596)) ;
#95156=CARTESIAN_POINT('Origin',(30.9927777216053,257.597448434855,20.2213203435596)) ;
#95157=CARTESIAN_POINT('',(30.9575197581061,256.75826900652,20.3213203435596)) ;
#95158=CARTESIAN_POINT('',(30.9927777216053,257.597448434855,20.3213203435596)) ;
#95159=CARTESIAN_POINT('',(30.8533181106036,256.660409606953,20.2213203435596)) ;
#95160=CARTESIAN_POINT('Ctrl Pts',(30.9575180778337,256.758268913088,20.3213203435596)) ;
#95161=CARTESIAN_POINT('Ctrl Pts',(30.9572608740877,256.758025782119,20.3213203435596)) ;
#95162=CARTESIAN_POINT('Ctrl Pts',(30.9570036902145,256.757782627797,20.321319430125)) ;
#95163=CARTESIAN_POINT('Ctrl Pts',(30.9447772812169,256.74622121684,20.3212325950421)) ;
#95164=CARTESIAN_POINT('Ctrl Pts',(30.9327366006538,256.734738416808,20.3191690170698)) ;
#95165=CARTESIAN_POINT('Ctrl Pts',(30.9104851869289,256.713579232422,20.3112355499301)) ;
#95166=CARTESIAN_POINT('Ctrl Pts',(30.8998969464719,256.703542376543,20.3055366838106)) ;
#95167=CARTESIAN_POINT('Ctrl Pts',(30.8801360641889,256.685251674835,20.2894998523043)) ;
#95168=CARTESIAN_POINT('Ctrl Pts',(30.8716480508847,256.677535742468,20.2794186430539)) ;
#95169=CARTESIAN_POINT('Ctrl Pts',(30.861575957675,256.66822888513,20.2611063637428)) ;
#95170=CARTESIAN_POINT('Ctrl Pts',(30.8584846426284,256.665338066437,20.2535176474882)) ;
#95171=CARTESIAN_POINT('Ctrl Pts',(30.8543790138895,256.661448508963,20.2376314832746)) ;
#95172=CARTESIAN_POINT('Ctrl Pts',(30.8533181106036,256.660409606953,20.22954590721)) ;
#95173=CARTESIAN_POINT('Ctrl Pts',(30.8533181106036,256.660409606953,20.2213203435596)) ;
#95174=CARTESIAN_POINT('',(30.8928658755038,257.601646411582,20.2213203435596)) ;
#95175=CARTESIAN_POINT('Ctrl Pts',(30.8533181106035,256.660409606953,20.2213203435596)) ;
#95176=CARTESIAN_POINT('Ctrl Pts',(30.9548849732834,256.656142091714,20.2213203435596)) ;
#95177=CARTESIAN_POINT('Ctrl Pts',(31.1603957461103,256.65842875267,20.2213203435596)) ;
#95178=CARTESIAN_POINT('Ctrl Pts',(31.4294296466895,256.727933237041,20.2213203435596)) ;
#95179=CARTESIAN_POINT('Ctrl Pts',(31.620729986201,256.8593293761,20.2213203435596)) ;
#95180=CARTESIAN_POINT('Ctrl Pts',(31.7681817196131,257.035881970398,20.2213203435596)) ;
#95181=CARTESIAN_POINT('Ctrl Pts',(31.8730100005906,257.26858199656,20.2213203435596)) ;
#95182=CARTESIAN_POINT('Ctrl Pts',(31.9737678628349,257.486117355144,20.2213203435596)) ;
#95183=CARTESIAN_POINT('Ctrl Pts',(32.0972269406744,257.751397872113,20.2213203435596)) ;
#95184=CARTESIAN_POINT('Ctrl Pts',(32.1813080297677,257.927086809909,20.2213203435596)) ;
#95185=CARTESIAN_POINT('Ctrl Pts',(32.2444298429768,258.059216868221,20.2213203435596)) ;
#95186=CARTESIAN_POINT('Ctrl Pts',(30.8533181106035,256.660409606953,20.2512402735938)) ;
#95187=CARTESIAN_POINT('Ctrl Pts',(30.9548979600485,256.656141546052,20.2512402735938)) ;
#95188=CARTESIAN_POINT('Ctrl Pts',(31.1604023801564,256.658404182352,20.2512402735938)) ;
#95189=CARTESIAN_POINT('Ctrl Pts',(31.4294987777394,256.727910448283,20.2512402735938)) ;
#95190=CARTESIAN_POINT('Ctrl Pts',(31.6208848030502,256.859363688134,20.2512402735938)) ;
#95191=CARTESIAN_POINT('Ctrl Pts',(31.7683753766291,257.03598413956,20.2512402735938)) ;
#95192=CARTESIAN_POINT('Ctrl Pts',(31.8732029711292,257.268708585883,20.2512402735938)) ;
#95193=CARTESIAN_POINT('Ctrl Pts',(31.9738911236935,257.486192550919,20.2512402735938)) ;
#95194=CARTESIAN_POINT('Ctrl Pts',(32.0973472479167,257.751471757306,20.2512402735938)) ;
#95195=CARTESIAN_POINT('Ctrl Pts',(32.1813079612835,257.927086666554,20.2512402735938)) ;
#95196=CARTESIAN_POINT('Ctrl Pts',(32.2444298429768,258.059216868221,20.2512402735938)) ;
#95197=CARTESIAN_POINT('Ctrl Pts',(30.8543731520913,256.685519594361,20.3030172699825)) ;
#95198=CARTESIAN_POINT('Ctrl Pts',(30.9549157428196,256.681295115759,20.3030172699825)) ;
#95199=CARTESIAN_POINT('Ctrl Pts',(31.1578746686145,256.6836549958,20.3030172699825)) ;
#95200=CARTESIAN_POINT('Ctrl Pts',(31.4195632325522,256.751572357658,20.3030172699825)) ;
#95201=CARTESIAN_POINT('Ctrl Pts',(31.6035540679525,256.878134439093,20.3030172699825)) ;
#95202=CARTESIAN_POINT('Ctrl Pts',(31.7458235525455,257.048058386227,20.3030172699825)) ;
#95203=CARTESIAN_POINT('Ctrl Pts',(31.8499630479459,257.278384117763,20.3030172699825)) ;
#95204=CARTESIAN_POINT('Ctrl Pts',(31.9509466435699,257.496794195582,20.3030172699825)) ;
#95205=CARTESIAN_POINT('Ctrl Pts',(32.0744757842965,257.762079759478,20.3030172699825)) ;
#95206=CARTESIAN_POINT('Ctrl Pts',(32.1586361363901,257.937931623778,20.3030172699825)) ;
#95207=CARTESIAN_POINT('Ctrl Pts',(32.221752548216,258.070050375617,20.3030172699825)) ;
#95208=CARTESIAN_POINT('Ctrl Pts',(30.8565740635558,256.737901287217,20.3213203435596)) ;
#95209=CARTESIAN_POINT('Ctrl Pts',(30.9549872971979,256.7337662774,20.3213203435596)) ;
#95210=CARTESIAN_POINT('Ctrl Pts',(31.1526192371051,256.736265271766,20.3213203435596)) ;
#95211=CARTESIAN_POINT('Ctrl Pts',(31.3990202175279,256.800872763809,20.3213203435596)) ;
#95212=CARTESIAN_POINT('Ctrl Pts',(31.567811372452,256.917382954853,20.3213203435596)) ;
#95213=CARTESIAN_POINT('Ctrl Pts',(31.6992922506992,257.073517437575,20.3213203435596)) ;
#95214=CARTESIAN_POINT('Ctrl Pts',(31.8019944880323,257.298904028522,20.3213203435596)) ;
#95215=CARTESIAN_POINT('Ctrl Pts',(31.9034094430465,257.519109697895,20.3213203435596)) ;
#95216=CARTESIAN_POINT('Ctrl Pts',(32.0270830659073,257.784405046748,20.3213203435596)) ;
#95217=CARTESIAN_POINT('Ctrl Pts',(32.1113404881888,257.960554799894,20.3213203435596)) ;
#95218=CARTESIAN_POINT('Ctrl Pts',(32.174445671089,258.092650046726,20.3213203435596)) ;
#95219=CARTESIAN_POINT('Ctrl Pts',(30.8575160873304,256.760321453054,20.3213203435596)) ;
#95220=CARTESIAN_POINT('Ctrl Pts',(30.9550193069044,256.756224679123,20.3213203435596)) ;
#95221=CARTESIAN_POINT('Ctrl Pts',(31.1503705386778,256.758780657464,20.3213203435596)) ;
#95222=CARTESIAN_POINT('Ctrl Pts',(31.3902348566204,256.821971664364,20.3213203435596)) ;
#95223=CARTESIAN_POINT('Ctrl Pts',(31.5525294429582,256.934185574877,20.3213203435596)) ;
#95224=CARTESIAN_POINT('Ctrl Pts',(31.6793967698716,257.084425183967,20.3213203435596)) ;
#95225=CARTESIAN_POINT('Ctrl Pts',(31.781483765643,257.307700348399,20.3213203435596)) ;
#95226=CARTESIAN_POINT('Ctrl Pts',(31.8830759236654,257.528669084034,20.3213203435596)) ;
#95227=CARTESIAN_POINT('Ctrl Pts',(32.0068110724735,257.793968481396,20.3213203435596)) ;
#95228=CARTESIAN_POINT('Ctrl Pts',(32.0910972199716,257.970237850073,20.3213203435596)) ;
#95229=CARTESIAN_POINT('Ctrl Pts',(32.1541976040146,258.102323051673,20.3213203435596)) ;
#95230=CARTESIAN_POINT('',(32.2017228806822,257.969823855374,20.2213203435596)) ;
#95231=CARTESIAN_POINT('Ctrl Pts',(32.2017235795172,257.969823517693,20.2213203435596)) ;
#95232=CARTESIAN_POINT('Ctrl Pts',(32.1529021533786,257.867592660009,20.2213203435596)) ;
#95233=CARTESIAN_POINT('Ctrl Pts',(32.0832989624708,257.721470374493,20.2213203435596)) ;
#95234=CARTESIAN_POINT('Ctrl Pts',(31.9737678628349,257.486117355144,20.2213203435596)) ;
#95235=CARTESIAN_POINT('Ctrl Pts',(31.8730100005906,257.26858199656,20.2213203435596)) ;
#95236=CARTESIAN_POINT('Ctrl Pts',(31.7681817196131,257.035881970398,20.2213203435596)) ;
#95237=CARTESIAN_POINT('Ctrl Pts',(31.620729986201,256.8593293761,20.2213203435596)) ;
#95238=CARTESIAN_POINT('Ctrl Pts',(31.4294296466895,256.727933237041,20.2213203435596)) ;
#95239=CARTESIAN_POINT('Ctrl Pts',(31.1603957461103,256.65842875267,20.2213203435596)) ;
#95240=CARTESIAN_POINT('Ctrl Pts',(30.9548849732834,256.656142091714,20.2213203435596)) ;
#95241=CARTESIAN_POINT('Ctrl Pts',(30.8533181106035,256.660409606953,20.2213203435596)) ;
#95242=CARTESIAN_POINT('',(32.1541976040147,258.102323051673,20.3213203435596)) ;
#95243=CARTESIAN_POINT('Ctrl Pts',(30.957523107636,256.758268931228,20.3213203435596)) ;
#95244=CARTESIAN_POINT('Ctrl Pts',(31.0216947820032,256.75850044908,20.3213203435596)) ;
#95245=CARTESIAN_POINT('Ctrl Pts',(31.1831674844922,256.767420842244,20.3213203435596)) ;
#95246=CARTESIAN_POINT('Ctrl Pts',(31.3902348566204,256.821971664364,20.3213203435596)) ;
#95247=CARTESIAN_POINT('Ctrl Pts',(31.5525294429582,256.934185574877,20.3213203435596)) ;
#95248=CARTESIAN_POINT('Ctrl Pts',(31.6793967698716,257.084425183967,20.3213203435596)) ;
#95249=CARTESIAN_POINT('Ctrl Pts',(31.781483765643,257.307700348399,20.3213203435596)) ;
#95250=CARTESIAN_POINT('Ctrl Pts',(31.8830759236654,257.528669084034,20.3213203435596)) ;
#95251=CARTESIAN_POINT('Ctrl Pts',(32.0068110724735,257.793968481396,20.3213203435596)) ;
#95252=CARTESIAN_POINT('Ctrl Pts',(32.0910972199716,257.970237850073,20.3213203435596)) ;
#95253=CARTESIAN_POINT('Ctrl Pts',(32.1541976040146,258.102323051673,20.3213203435596)) ;
#95254=CARTESIAN_POINT('Ctrl Pts',(32.1541976040147,258.102323051673,20.3213203435596)) ;
#95255=CARTESIAN_POINT('Ctrl Pts',(32.154310750693,258.101997885783,20.3213203435596)) ;
#95256=CARTESIAN_POINT('Ctrl Pts',(32.1544239638944,258.10167274146,20.321319429295)) ;
#95257=CARTESIAN_POINT('Ctrl Pts',(32.1598800150608,258.086013269478,20.32123140759)) ;
#95258=CARTESIAN_POINT('Ctrl Pts',(32.1654271588702,258.070582281274,20.3191133347114)) ;
#95259=CARTESIAN_POINT('Ctrl Pts',(32.1757628035262,258.042057844251,20.3110552232775)) ;
#95260=CARTESIAN_POINT('Ctrl Pts',(32.1807182443946,258.028478240893,20.3052525405995)) ;
#95261=CARTESIAN_POINT('Ctrl Pts',(32.1895979729969,258.003419474963,20.2890377823574)) ;
#95262=CARTESIAN_POINT('Ctrl Pts',(32.1933219350999,257.992745598067,20.2788893171814)) ;
#95263=CARTESIAN_POINT('Ctrl Pts',(32.1978571834542,257.980133965385,20.2605941621586)) ;
#95264=CARTESIAN_POINT('Ctrl Pts',(32.1992720778467,257.976288165441,20.2530925159503)) ;
#95265=CARTESIAN_POINT('Ctrl Pts',(32.2011977766946,257.971159193015,20.2374109489562)) ;
#95266=CARTESIAN_POINT('Ctrl Pts',(32.2017254632468,257.969822655041,20.2294326270796)) ;
#95267=CARTESIAN_POINT('Ctrl Pts',(32.2017235856673,257.969823530571,20.2213203435596)) ;
#95268=CARTESIAN_POINT('Origin',(32.0431849345645,258.15408910959,20.2213203435596)) ;
#95269=CARTESIAN_POINT('',(32.6189050513595,257.775288618279,20.2213203435596)) ;
#95270=CARTESIAN_POINT('',(32.0009231083904,258.063458330887,20.2213203435596)) ;
#95271=CARTESIAN_POINT('',(32.5264861881013,257.92872203387,20.3213203435596)) ;
#95272=CARTESIAN_POINT('',(32.0431849345645,258.15408910959,20.3213203435596)) ;
#95273=CARTESIAN_POINT('Origin',(32.5264861881013,257.92872203387,20.2213203435596)) ;
#95274=CARTESIAN_POINT('Origin',(32.5262827782143,257.924672599648,20.2213203435596)) ;
#95275=CARTESIAN_POINT('',(32.7094862928853,259.578557794143,20.2213203435596)) ;
#95276=CARTESIAN_POINT('',(32.6261568553752,257.91965575689,20.2213203435596)) ;
#95277=CARTESIAN_POINT('',(32.5972722714868,259.337914048676,20.3213203435596)) ;
#95278=CARTESIAN_POINT('',(32.5262827782143,257.924672599648,20.3213203435596)) ;
#95279=CARTESIAN_POINT('Origin',(32.5972722714868,259.337914048676,20.2213203435596)) ;
#95280=CARTESIAN_POINT('Origin',(32.1602128107536,258.932119389861,20.2213203435596)) ;
#95281=CARTESIAN_POINT('',(32.092171866909,259.005402607317,20.2213203435596)) ;
#95282=CARTESIAN_POINT('',(32.1602128107536,258.932119389861,20.3213203435596)) ;
#95283=CARTESIAN_POINT('Origin',(32.2017221802041,257.969824185949,20.0213203435596)) ;
#95284=CARTESIAN_POINT('',(32.6189050513595,257.775288618279,20.1213203435596)) ;
#95285=CARTESIAN_POINT('',(32.6189050513595,257.775288618279,20.0213203435596)) ;
#95286=CARTESIAN_POINT('',(32.2017221802041,257.969824185949,20.1213203435596)) ;
#95287=CARTESIAN_POINT('',(44.9570498632135,252.021917205086,20.1213203435596)) ;
#95288=CARTESIAN_POINT('',(32.2017221802041,257.969824185949,20.0213203435596)) ;
#95289=CARTESIAN_POINT('Origin',(32.6189050513595,257.775288618279,20.0213203435596)) ;
#95290=CARTESIAN_POINT('',(32.7094862928853,259.578557794143,20.1213203435596)) ;
#95291=CARTESIAN_POINT('',(32.7094862928853,259.578557794143,20.0213203435596)) ;
#95292=CARTESIAN_POINT('',(32.2199750708941,249.833488252288,20.1213203435596)) ;
#95293=CARTESIAN_POINT('Origin',(32.7094862928853,259.578557794143,20.0213203435596)) ;
#95294=CARTESIAN_POINT('',(31.3863264609896,258.350049454246,20.1213203435596)) ;
#95295=CARTESIAN_POINT('',(31.3863264609896,258.350049454246,20.0213203435596)) ;
#95296=CARTESIAN_POINT('',(34.0499529567987,260.823134931594,20.1213203435596)) ;
#95297=CARTESIAN_POINT('Origin',(31.3863264609896,258.350049454246,20.0213203435596)) ;
#95298=CARTESIAN_POINT('',(31.839183613039,258.138878696195,20.1213203435596)) ;
#95299=CARTESIAN_POINT('',(31.839183613039,258.138878696195,20.0213203435596)) ;
#95300=CARTESIAN_POINT('',(44.5493520036063,252.212029839235,20.1213203435596)) ;
#95301=CARTESIAN_POINT('Origin',(31.7767899168982,258.107052294689,20.3213203435596)) ;
#95302=CARTESIAN_POINT('Ctrl Pts',(30.5502224056744,257.052603781754,20.2213203435596)) ;
#95303=CARTESIAN_POINT('Ctrl Pts',(30.4504373470295,257.036098173567,20.2213203435596)) ;
#95304=CARTESIAN_POINT('Ctrl Pts',(30.2507744072825,256.993547832196,20.2213203435598)) ;
#95305=CARTESIAN_POINT('Ctrl Pts',(29.9535859505325,256.89665014184,20.2213203435598)) ;
#95306=CARTESIAN_POINT('Ctrl Pts',(29.6697087711132,256.680511270254,20.2213203435599)) ;
#95307=CARTESIAN_POINT('Ctrl Pts',(29.5798204552179,256.467740611946,20.22132034356)) ;
#95308=CARTESIAN_POINT('Ctrl Pts',(29.5387593890436,256.371007899967,20.22132034356)) ;
#95309=CARTESIAN_POINT('Ctrl Pts',(29.5339221017733,256.359561959438,20.22132034356)) ;
#95310=CARTESIAN_POINT('Ctrl Pts',(29.5255243701777,256.339659474417,20.22132034356)) ;
#95311=CARTESIAN_POINT('Ctrl Pts',(29.5088379386217,256.300040213624,20.22132034356)) ;
#95312=CARTESIAN_POINT('Ctrl Pts',(29.4850272312111,256.243996783598,20.22132034356)) ;
#95313=CARTESIAN_POINT('Ctrl Pts',(29.4607697687769,256.188324327745,20.22132034356)) ;
#95314=CARTESIAN_POINT('Ctrl Pts',(29.4410231456084,256.143964729335,20.22132034356)) ;
#95315=CARTESIAN_POINT('Ctrl Pts',(29.3511457605012,255.944690099184,20.22132034356)) ;
#95316=CARTESIAN_POINT('Ctrl Pts',(29.2580498043477,255.761710546012,20.2213203435596)) ;
#95317=CARTESIAN_POINT('Ctrl Pts',(29.1697396985386,255.584956164831,20.2213203435596)) ;
#95318=CARTESIAN_POINT('Ctrl Pts',(30.5502224056744,257.052603781754,20.2512402735938)) ;
#95319=CARTESIAN_POINT('Ctrl Pts',(30.4504290994671,257.036096809325,20.2512402735938)) ;
#95320=CARTESIAN_POINT('Ctrl Pts',(30.250787991272,256.993571390254,20.251240273594)) ;
#95321=CARTESIAN_POINT('Ctrl Pts',(29.953570539349,256.896684290815,20.251240273594)) ;
#95322=CARTESIAN_POINT('Ctrl Pts',(29.6695953979979,256.680469695693,20.2512402735941)) ;
#95323=CARTESIAN_POINT('Ctrl Pts',(29.5796974644403,256.467635740865,20.2512402735942)) ;
#95324=CARTESIAN_POINT('Ctrl Pts',(29.5386402549432,256.370904573759,20.2512402735942)) ;
#95325=CARTESIAN_POINT('Ctrl Pts',(29.5338026904391,256.359458201952,20.2512402735942)) ;
#95326=CARTESIAN_POINT('Ctrl Pts',(29.5254052731515,256.339555807343,20.2512402735942)) ;
#95327=CARTESIAN_POINT('Ctrl Pts',(29.5087194815055,256.299937206453,20.2512402735942)) ;
#95328=CARTESIAN_POINT('Ctrl Pts',(29.4849117359914,256.243897323674,20.2512402735942)) ;
#95329=CARTESIAN_POINT('Ctrl Pts',(29.4606563257843,256.188228104397,20.2512402735942)) ;
#95330=CARTESIAN_POINT('Ctrl Pts',(29.4409117402036,256.143871399368,20.2512402735942)) ;
#95331=CARTESIAN_POINT('Ctrl Pts',(29.3510404818838,255.944607280785,20.2512402735942)) ;
#95332=CARTESIAN_POINT('Ctrl Pts',(29.2580505786398,255.761712095772,20.2512402735938)) ;
#95333=CARTESIAN_POINT('Ctrl Pts',(29.1697396985386,255.584956164831,20.2512402735938)) ;
#95334=CARTESIAN_POINT('Ctrl Pts',(30.5543238187055,257.027808588799,20.3030173033455)) ;
#95335=CARTESIAN_POINT('Ctrl Pts',(30.4551892489819,257.011410579038,20.3030173033455)) ;
#95336=CARTESIAN_POINT('Ctrl Pts',(30.2572087756548,256.969401492031,20.3030173033456)) ;
#95337=CARTESIAN_POINT('Ctrl Pts',(29.9641223307203,256.873009951542,20.3030173033457)) ;
#95338=CARTESIAN_POINT('Ctrl Pts',(29.6908334963393,256.664955954783,20.3030173033458)) ;
#95339=CARTESIAN_POINT('Ctrl Pts',(29.6030899043467,256.458207136188,20.3030173033459)) ;
#95340=CARTESIAN_POINT('Ctrl Pts',(29.562095221275,256.361626988556,20.3030173033459)) ;
#95341=CARTESIAN_POINT('Ctrl Pts',(29.5572688117543,256.350206925962,20.3030173033459)) ;
#95342=CARTESIAN_POINT('Ctrl Pts',(29.5488779342165,256.330320721087,20.3030173033459)) ;
#95343=CARTESIAN_POINT('Ctrl Pts',(29.5321823528865,256.290679973573,20.3030173033459)) ;
#95344=CARTESIAN_POINT('Ctrl Pts',(29.5083052653683,256.234480293537,20.3030173033459)) ;
#95345=CARTESIAN_POINT('Ctrl Pts',(29.4839605385045,256.178607635609,20.3030173033459)) ;
#95346=CARTESIAN_POINT('Ctrl Pts',(29.4641412177491,256.134084748371,20.3030173033459)) ;
#95347=CARTESIAN_POINT('Ctrl Pts',(29.3739437406398,255.934101429851,20.3030173033459)) ;
#95348=CARTESIAN_POINT('Ctrl Pts',(29.2804709943218,255.750355719183,20.3030173033455)) ;
#95349=CARTESIAN_POINT('Ctrl Pts',(29.1922219572742,255.573723568307,20.3030173033455)) ;
#95350=CARTESIAN_POINT('Ctrl Pts',(30.5628797492928,256.976083500832,20.3213203435596)) ;
#95351=CARTESIAN_POINT('Ctrl Pts',(30.4650974797975,256.959909177243,20.3213203435596)) ;
#95352=CARTESIAN_POINT('Ctrl Pts',(30.2706391777167,256.919043340531,20.3213203435598)) ;
#95353=CARTESIAN_POINT('Ctrl Pts',(29.9860934580288,256.823713686167,20.3213203435598)) ;
#95354=CARTESIAN_POINT('Ctrl Pts',(29.7348373077925,256.632482520968,20.3213203435599)) ;
#95355=CARTESIAN_POINT('Ctrl Pts',(29.6515623522189,256.438259902233,20.32132034356)) ;
#95356=CARTESIAN_POINT('Ctrl Pts',(29.6107083391225,256.341998894775,20.32132034356)) ;
#95357=CARTESIAN_POINT('Ctrl Pts',(29.6059044642761,256.330632571226,20.32132034356)) ;
#95358=CARTESIAN_POINT('Ctrl Pts',(29.5975280633095,256.310780379563,20.32132034356)) ;
#95359=CARTESIAN_POINT('Ctrl Pts',(29.5808137578388,256.27109518323,20.32132034356)) ;
#95360=CARTESIAN_POINT('Ctrl Pts',(29.5567998760631,256.214571564109,20.32132034356)) ;
#95361=CARTESIAN_POINT('Ctrl Pts',(29.5322742720676,256.158283102678,20.32132034356)) ;
#95362=CARTESIAN_POINT('Ctrl Pts',(29.5123044536673,256.113421221662,20.32132034356)) ;
#95363=CARTESIAN_POINT('Ctrl Pts',(29.4214427116386,255.911965478229,20.32132034356)) ;
#95364=CARTESIAN_POINT('Ctrl Pts',(29.3272441297798,255.726669369536,20.3213203435596)) ;
#95365=CARTESIAN_POINT('Ctrl Pts',(29.2391220484686,255.550291323017,20.3213203435596)) ;
#95366=CARTESIAN_POINT('Ctrl Pts',(30.566541816524,256.953944383674,20.3213203435596)) ;
#95367=CARTESIAN_POINT('Ctrl Pts',(30.4693374736902,256.93786565587,20.3213203435596)) ;
#95368=CARTESIAN_POINT('Ctrl Pts',(30.2763890386465,256.897491801285,20.3213203435598)) ;
#95369=CARTESIAN_POINT('Ctrl Pts',(29.9954957906156,256.802617777926,20.3213203435598)) ;
#95370=CARTESIAN_POINT('Ctrl Pts',(29.7536595300643,256.618578974978,20.3213203435599)) ;
#95371=CARTESIAN_POINT('Ctrl Pts',(29.672296194115,256.429711018626,20.32132034356)) ;
#95372=CARTESIAN_POINT('Ctrl Pts',(29.6315028005541,256.333586772474,20.32132034356)) ;
#95373=CARTESIAN_POINT('Ctrl Pts',(29.6267085413676,256.322243404122,20.32132034356)) ;
#95374=CARTESIAN_POINT('Ctrl Pts',(29.6183383700597,256.302405780253,20.32132034356)) ;
#95375=CARTESIAN_POINT('Ctrl Pts',(29.6016161185133,256.262701629424,20.32132034356)) ;
#95376=CARTESIAN_POINT('Ctrl Pts',(29.5775440021221,256.20603973721,20.32132034356)) ;
#95377=CARTESIAN_POINT('Ctrl Pts',(29.5529411985134,256.14957365025,20.32132034356)) ;
#95378=CARTESIAN_POINT('Ctrl Pts',(29.532907181819,256.104566982881,20.32132034356)) ;
#95379=CARTESIAN_POINT('Ctrl Pts',(29.4417617767858,255.902482138686,20.32132034356)) ;
#95380=CARTESIAN_POINT('Ctrl Pts',(29.3472638190854,255.71653141995,20.3213203435596)) ;
#95381=CARTESIAN_POINT('Ctrl Pts',(29.2591959942947,255.540261968904,20.3213203435596)) ;
#95382=CARTESIAN_POINT('',(30.4681271505274,256.936145439019,20.3213203435596)) ;
#95383=CARTESIAN_POINT('',(29.2591959942946,255.540261968904,20.3213203435596)) ;
#95384=CARTESIAN_POINT('Ctrl Pts',(30.4681271505274,256.936145439019,20.3213203435596)) ;
#95385=CARTESIAN_POINT('Ctrl Pts',(30.404199598279,256.923546655539,20.3213203435597)) ;
#95386=CARTESIAN_POINT('Ctrl Pts',(30.2447009077672,256.88678887236,20.3213203435598)) ;
#95387=CARTESIAN_POINT('Ctrl Pts',(29.9954957906156,256.802617777926,20.3213203435598)) ;
#95388=CARTESIAN_POINT('Ctrl Pts',(29.7536595300643,256.618578974978,20.3213203435599)) ;
#95389=CARTESIAN_POINT('Ctrl Pts',(29.672296194115,256.429711018626,20.32132034356)) ;
#95390=CARTESIAN_POINT('Ctrl Pts',(29.6315028005541,256.333586772474,20.32132034356)) ;
#95391=CARTESIAN_POINT('Ctrl Pts',(29.6267085413676,256.322243404122,20.32132034356)) ;
#95392=CARTESIAN_POINT('Ctrl Pts',(29.6183383700597,256.302405780253,20.32132034356)) ;
#95393=CARTESIAN_POINT('Ctrl Pts',(29.6016161185133,256.262701629424,20.32132034356)) ;
#95394=CARTESIAN_POINT('Ctrl Pts',(29.5775440021221,256.20603973721,20.32132034356)) ;
#95395=CARTESIAN_POINT('Ctrl Pts',(29.5529411985134,256.14957365025,20.32132034356)) ;
#95396=CARTESIAN_POINT('Ctrl Pts',(29.532907181819,256.104566982881,20.32132034356)) ;
#95397=CARTESIAN_POINT('Ctrl Pts',(29.4417617767858,255.902482138686,20.32132034356)) ;
#95398=CARTESIAN_POINT('Ctrl Pts',(29.3472638190854,255.71653141995,20.3213203435596)) ;
#95399=CARTESIAN_POINT('Ctrl Pts',(29.2591959942947,255.540261968904,20.3213203435596)) ;
#95400=CARTESIAN_POINT('',(29.213306918992,255.671998198108,20.2213203435596)) ;
#95401=CARTESIAN_POINT('Ctrl Pts',(29.2591959942946,255.540261968904,20.3213203435596)) ;
#95402=CARTESIAN_POINT('Ctrl Pts',(29.2590867165055,255.540585371864,20.3213203435596)) ;
#95403=CARTESIAN_POINT('Ctrl Pts',(29.2589773726705,255.54090875402,20.3213194290187)) ;
#95404=CARTESIAN_POINT('Ctrl Pts',(29.2536958381592,255.556518479706,20.321231181363)) ;
#95405=CARTESIAN_POINT('Ctrl Pts',(29.2483227014057,255.57189823562,20.3191028849279)) ;
#95406=CARTESIAN_POINT('Ctrl Pts',(29.2383131514629,255.600324941419,20.3110059033691)) ;
#95407=CARTESIAN_POINT('Ctrl Pts',(29.2335189659059,255.613847174906,20.3051753495665)) ;
#95408=CARTESIAN_POINT('Ctrl Pts',(29.2249637172964,255.638735334461,20.2889211055947)) ;
#95409=CARTESIAN_POINT('Ctrl Pts',(29.2213832985399,255.649320365818,20.2787669436689)) ;
#95410=CARTESIAN_POINT('Ctrl Pts',(29.2170223683631,255.661812395744,20.2604759078399)) ;
#95411=CARTESIAN_POINT('Ctrl Pts',(29.215664386302,255.665610853218,20.2529927710902)) ;
#95412=CARTESIAN_POINT('Ctrl Pts',(29.213813498395,255.670679065537,20.237359488709)) ;
#95413=CARTESIAN_POINT('Ctrl Pts',(29.2133053651598,255.671998912603,20.2294043743899)) ;
#95414=CARTESIAN_POINT('Ctrl Pts',(29.2133063229928,255.671998465958,20.2213203435596)) ;
#95415=CARTESIAN_POINT('',(30.5502224056744,257.052603781754,20.2213203435596)) ;
#95416=CARTESIAN_POINT('Ctrl Pts',(29.2133075051976,255.671997914687,20.2213203435597)) ;
#95417=CARTESIAN_POINT('Ctrl Pts',(29.2307530417186,255.706837709317,20.2213203435597)) ;
#95418=CARTESIAN_POINT('Ctrl Pts',(29.2480451874319,255.741544522718,20.2213203435597)) ;
#95419=CARTESIAN_POINT('Ctrl Pts',(29.2651899065699,255.776196982818,20.2213203435597)) ;
#95420=CARTESIAN_POINT('Ctrl Pts',(29.2836186893254,255.813444758883,20.2213203435598)) ;
#95421=CARTESIAN_POINT('Ctrl Pts',(29.3018805490242,255.850634869259,20.2213203435598)) ;
#95422=CARTESIAN_POINT('Ctrl Pts',(29.3199861498403,255.887894741683,20.2213203435598)) ;
#95423=CARTESIAN_POINT('Ctrl Pts',(29.3342424835541,255.917233131545,20.2213203435599)) ;
#95424=CARTESIAN_POINT('Ctrl Pts',(29.3484027162989,255.946616480248,20.2213203435599)) ;
#95425=CARTESIAN_POINT('Ctrl Pts',(29.3624503738921,255.976083989101,20.2213203435599)) ;
#95426=CARTESIAN_POINT('Ctrl Pts',(29.3744610562137,256.001278572988,20.2213203435599)) ;
#95427=CARTESIAN_POINT('Ctrl Pts',(29.3863896118145,256.026535087145,20.22132034356)) ;
#95428=CARTESIAN_POINT('Ctrl Pts',(29.3982031370694,256.051848366021,20.22132034356)) ;
#95429=CARTESIAN_POINT('Ctrl Pts',(29.4073911676691,256.071535900087,20.22132034356)) ;
#95430=CARTESIAN_POINT('Ctrl Pts',(29.4165093180901,256.091257405863,20.22132034356)) ;
#95431=CARTESIAN_POINT('Ctrl Pts',(29.425529160593,256.110992495285,20.22132034356)) ;
#95432=CARTESIAN_POINT('Ctrl Pts',(29.4305752194442,256.122033089689,20.22132034356)) ;
#95433=CARTESIAN_POINT('Ctrl Pts',(29.4355961225057,256.13309037525,20.22132034356)) ;
#95434=CARTESIAN_POINT('Ctrl Pts',(29.4405850973892,256.144158974749,20.22132034356)) ;
#95435=CARTESIAN_POINT('Ctrl Pts',(29.4455894877222,256.155261775149,20.22132034356)) ;
#95436=CARTESIAN_POINT('Ctrl Pts',(29.4505617588215,256.166375877005,20.22132034356)) ;
#95437=CARTESIAN_POINT('Ctrl Pts',(29.4554995354655,256.177507784875,20.22132034356)) ;
#95438=CARTESIAN_POINT('Ctrl Pts',(29.4589254454287,256.1852312841,20.22132034356)) ;
#95439=CARTESIAN_POINT('Ctrl Pts',(29.4623367397909,256.192967969647,20.22132034356)) ;
#95440=CARTESIAN_POINT('Ctrl Pts',(29.4657236710055,256.200700387666,20.22132034356)) ;
#95441=CARTESIAN_POINT('Ctrl Pts',(29.4710997144517,256.212973980657,20.22132034356)) ;
#95442=CARTESIAN_POINT('Ctrl Pts',(29.476410769658,256.22531618242,20.22132034356)) ;
#95443=CARTESIAN_POINT('Ctrl Pts',(29.4816615232414,256.237682350978,20.22132034356)) ;
#95444=CARTESIAN_POINT('Ctrl Pts',(29.4863645891097,256.248758647807,20.22132034356)) ;
#95445=CARTESIAN_POINT('Ctrl Pts',(29.491019360315,256.259853814514,20.22132034356)) ;
#95446=CARTESIAN_POINT('Ctrl Pts',(29.4956515405211,256.270981218767,20.22132034356)) ;
#95447=CARTESIAN_POINT('Ctrl Pts',(29.5035602780298,256.289979555507,20.22132034356)) ;
#95448=CARTESIAN_POINT('Ctrl Pts',(29.511399561512,256.309067225097,20.22132034356)) ;
#95449=CARTESIAN_POINT('Ctrl Pts',(29.5192933563511,256.32825717138,20.22132034356)) ;
#95450=CARTESIAN_POINT('Ctrl Pts',(29.5225268702631,256.336117897373,20.22132034356)) ;
#95451=CARTESIAN_POINT('Ctrl Pts',(29.5257686806131,256.343992960907,20.22132034356)) ;
#95452=CARTESIAN_POINT('Ctrl Pts',(29.529030465216,256.351887406121,20.22132034356)) ;
#95453=CARTESIAN_POINT('Ctrl Pts',(29.5307511106271,256.356051856747,20.22132034356)) ;
#95454=CARTESIAN_POINT('Ctrl Pts',(29.5324781961111,256.360223805101,20.22132034356)) ;
#95455=CARTESIAN_POINT('Ctrl Pts',(29.5342149642331,256.36440733422,20.22132034356)) ;
#95456=CARTESIAN_POINT('Ctrl Pts',(29.535495630112,256.367492203713,20.22132034356)) ;
#95457=CARTESIAN_POINT('Ctrl Pts',(29.5367799677669,256.370579502307,20.22132034356)) ;
#95458=CARTESIAN_POINT('Ctrl Pts',(29.5380635719759,256.373657193282,20.22132034356)) ;
#95459=CARTESIAN_POINT('Ctrl Pts',(29.5394513950042,256.376984769164,20.22132034356)) ;
#95460=CARTESIAN_POINT('Ctrl Pts',(29.5408419684465,256.380309842844,20.22132034356)) ;
#95461=CARTESIAN_POINT('Ctrl Pts',(29.5422463762053,256.383656789344,20.22132034356)) ;
#95462=CARTESIAN_POINT('Ctrl Pts',(29.5500527870912,256.402260816147,20.22132034356)) ;
#95463=CARTESIAN_POINT('Ctrl Pts',(29.5582185870785,256.421386647834,20.22132034356)) ;
#95464=CARTESIAN_POINT('Ctrl Pts',(29.5668254892807,256.440765383713,20.22132034356)) ;
#95465=CARTESIAN_POINT('Ctrl Pts',(29.5764165175254,256.462359913173,20.22132034356)) ;
#95466=CARTESIAN_POINT('Ctrl Pts',(29.5865567090972,256.48426749885,20.22132034356)) ;
#95467=CARTESIAN_POINT('Ctrl Pts',(29.597423005008,256.506146707171,20.22132034356)) ;
#95468=CARTESIAN_POINT('Ctrl Pts',(29.6089408564768,256.529337817902,20.22132034356)) ;
#95469=CARTESIAN_POINT('Ctrl Pts',(29.6212791896667,256.55249607905,20.22132034356)) ;
#95470=CARTESIAN_POINT('Ctrl Pts',(29.6346677671494,256.575263247164,20.2213203435599)) ;
#95471=CARTESIAN_POINT('Ctrl Pts',(29.6447092002614,256.592338623249,20.2213203435599)) ;
#95472=CARTESIAN_POINT('Ctrl Pts',(29.6553424455427,256.609195022114,20.2213203435599)) ;
#95473=CARTESIAN_POINT('Ctrl Pts',(29.6666432561968,256.625702023723,20.2213203435599)) ;
#95474=CARTESIAN_POINT('Ctrl Pts',(29.6730261077246,256.635025402698,20.2213203435599)) ;
#95475=CARTESIAN_POINT('Ctrl Pts',(29.6796214358638,256.644237651328,20.2213203435599)) ;
#95476=CARTESIAN_POINT('Ctrl Pts',(29.6864374605946,256.653317913181,20.2213203435599)) ;
#95477=CARTESIAN_POINT('Ctrl Pts',(29.6920155866947,256.660749054885,20.2213203435599)) ;
#95478=CARTESIAN_POINT('Ctrl Pts',(29.6977426583487,256.668093123778,20.2213203435599)) ;
#95479=CARTESIAN_POINT('Ctrl Pts',(29.7036113206688,256.675328820148,20.2213203435599)) ;
#95480=CARTESIAN_POINT('Ctrl Pts',(29.7192328828822,256.694589236719,20.2213203435599)) ;
#95481=CARTESIAN_POINT('Ctrl Pts',(29.7358819982484,256.713110580123,20.2213203435599)) ;
#95482=CARTESIAN_POINT('Ctrl Pts',(29.7536800879331,256.730900674017,20.2213203435599)) ;
#95483=CARTESIAN_POINT('Ctrl Pts',(29.7644212276756,256.741636988304,20.2213203435599)) ;
#95484=CARTESIAN_POINT('Ctrl Pts',(29.7755798595812,256.752107073421,20.2213203435599)) ;
#95485=CARTESIAN_POINT('Ctrl Pts',(29.7871734949583,256.762313540024,20.2213203435599)) ;
#95486=CARTESIAN_POINT('Ctrl Pts',(29.8155501675463,256.787294967475,20.2213203435599)) ;
#95487=CARTESIAN_POINT('Ctrl Pts',(29.8451075130733,256.809701403991,20.2213203435598)) ;
#95488=CARTESIAN_POINT('Ctrl Pts',(29.8755296737893,256.829949043671,20.2213203435598)) ;
#95489=CARTESIAN_POINT('Ctrl Pts',(29.8888393691026,256.838807386031,20.2213203435598)) ;
#95490=CARTESIAN_POINT('Ctrl Pts',(29.9023141156151,256.847252072064,20.2213203435598)) ;
#95491=CARTESIAN_POINT('Ctrl Pts',(29.9159253289018,256.855315666829,20.2213203435598)) ;
#95492=CARTESIAN_POINT('Ctrl Pts',(29.9277267736438,256.862307113222,20.2213203435598)) ;
#95493=CARTESIAN_POINT('Ctrl Pts',(29.939630786004,256.869012052383,20.2213203435598)) ;
#95494=CARTESIAN_POINT('Ctrl Pts',(29.9516180101726,256.875450759323,20.2213203435598)) ;
#95495=CARTESIAN_POINT('Ctrl Pts',(29.9566614722954,256.878159758013,20.2213203435598)) ;
#95496=CARTESIAN_POINT('Ctrl Pts',(29.9617179154655,256.880820619487,20.2213203435598)) ;
#95497=CARTESIAN_POINT('Ctrl Pts',(29.9667766228262,256.883430336315,20.2213203435598)) ;
#95498=CARTESIAN_POINT('Ctrl Pts',(29.9906424899446,256.895742405505,20.2213203435598)) ;
#95499=CARTESIAN_POINT('Ctrl Pts',(30.0146186463981,256.906953970521,20.2213203435598)) ;
#95500=CARTESIAN_POINT('Ctrl Pts',(30.0386586200925,256.917289953597,20.2213203435598)) ;
#95501=CARTESIAN_POINT('Ctrl Pts',(30.0634818792387,256.927962710135,20.2213203435598)) ;
#95502=CARTESIAN_POINT('Ctrl Pts',(30.0883731914004,256.937701390127,20.2213203435598)) ;
#95503=CARTESIAN_POINT('Ctrl Pts',(30.1133144111727,256.946703407878,20.2213203435598)) ;
#95504=CARTESIAN_POINT('Ctrl Pts',(30.1392690558496,256.9560712004,20.2213203435598)) ;
#95505=CARTESIAN_POINT('Ctrl Pts',(30.165277713297,256.96464080163,20.2213203435598)) ;
#95506=CARTESIAN_POINT('Ctrl Pts',(30.1913553599989,256.97258858843,20.2213203435598)) ;
#95507=CARTESIAN_POINT('Ctrl Pts',(30.2107444937283,256.978497890863,20.2213203435598)) ;
#95508=CARTESIAN_POINT('Ctrl Pts',(30.2301725212875,256.984062442463,20.2213203435598)) ;
#95509=CARTESIAN_POINT('Ctrl Pts',(30.249657583769,256.989341417562,20.2213203435597)) ;
#95510=CARTESIAN_POINT('Ctrl Pts',(30.262842937433,256.992913649046,20.2213203435597)) ;
#95511=CARTESIAN_POINT('Ctrl Pts',(30.2760454316719,256.996352315282,20.2213203435597)) ;
#95512=CARTESIAN_POINT('Ctrl Pts',(30.2892583034633,256.999670387357,20.2213203435597)) ;
#95513=CARTESIAN_POINT('Ctrl Pts',(30.322651117236,257.008056131547,20.2213203435597)) ;
#95514=CARTESIAN_POINT('Ctrl Pts',(30.3561115692332,257.015675648504,20.2213203435597)) ;
#95515=CARTESIAN_POINT('Ctrl Pts',(30.3895792904966,257.02271246259,20.2213203435597)) ;
#95516=CARTESIAN_POINT('Ctrl Pts',(30.4248514059428,257.030128662721,20.2213203435596)) ;
#95517=CARTESIAN_POINT('Ctrl Pts',(30.460131466338,257.036897256708,20.2213203435596)) ;
#95518=CARTESIAN_POINT('Ctrl Pts',(30.4953842467288,257.043186416176,20.2213203435596)) ;
#95519=CARTESIAN_POINT('Ctrl Pts',(30.5136708291516,257.046448775392,20.2213203435596)) ;
#95520=CARTESIAN_POINT('Ctrl Pts',(30.5319506504597,257.049581421127,20.2213203435596)) ;
#95521=CARTESIAN_POINT('Ctrl Pts',(30.5502224056744,257.052603781754,20.2213203435596)) ;
#95522=CARTESIAN_POINT('Ctrl Pts',(30.4681271505273,256.936145439019,20.3213203435596)) ;
#95523=CARTESIAN_POINT('Ctrl Pts',(30.4683299268523,256.936432008588,20.3213203435596)) ;
#95524=CARTESIAN_POINT('Ctrl Pts',(30.4685326646057,256.936718607507,20.3213194297254)) ;
#95525=CARTESIAN_POINT('Ctrl Pts',(30.4782179507238,256.950414093123,20.3212321344664)) ;
#95526=CARTESIAN_POINT('Ctrl Pts',(30.4877061821935,256.964022936168,20.3191476657588)) ;
#95527=CARTESIAN_POINT('Ctrl Pts',(30.5052277006315,256.989161753491,20.3111707686004)) ;
#95528=CARTESIAN_POINT('Ctrl Pts',(30.5135659702218,257.001123783895,20.3054349322803)) ;
#95529=CARTESIAN_POINT('Ctrl Pts',(30.5291730023403,257.022992686367,20.2893352101867)) ;
#95530=CARTESIAN_POINT('Ctrl Pts',(30.5358844390855,257.032244721745,20.2792373192504)) ;
#95531=CARTESIAN_POINT('Ctrl Pts',(30.5437948938036,257.043343479936,20.2609382270818)) ;
#95532=CARTESIAN_POINT('Ctrl Pts',(30.5462083785189,257.04677470554,20.253378482991)) ;
#95533=CARTESIAN_POINT('Ctrl Pts',(30.5494038052607,257.051380924324,20.2375590756384)) ;
#95534=CARTESIAN_POINT('Ctrl Pts',(30.5502224056744,257.052603781754,20.2295089201093)) ;
#95535=CARTESIAN_POINT('Ctrl Pts',(30.5502224056744,257.052603781754,20.2213203435596)) ;
#95536=CARTESIAN_POINT('Origin',(29.3774646884419,255.485112371103,20.2213203435596)) ;
#95537=CARTESIAN_POINT('',(28.8895617876714,255.712625230168,20.3213203435596)) ;
#95538=CARTESIAN_POINT('',(29.3774646884419,255.485112371103,20.3213203435596)) ;
#95539=CARTESIAN_POINT('',(28.7971429244132,255.86605864576,20.2213203435596)) ;
#95540=CARTESIAN_POINT('Origin',(28.8895617876714,255.712625230168,20.2213203435596)) ;
#95541=CARTESIAN_POINT('',(29.419726514616,255.575743149807,20.2213203435596)) ;
#95542=CARTESIAN_POINT('Origin',(28.890502822535,255.731359121804,20.2213203435596)) ;
#95543=CARTESIAN_POINT('',(28.8187757042858,254.303433215363,20.3213203435596)) ;
#95544=CARTESIAN_POINT('',(28.890502822535,255.731359121804,20.3213203435596)) ;
#95545=CARTESIAN_POINT('',(28.7065616828874,254.062789469896,20.2213203435596)) ;
#95546=CARTESIAN_POINT('Origin',(28.8187757042858,254.303433215363,20.2213203435596)) ;
#95547=CARTESIAN_POINT('',(28.7906287453741,255.736375964562,20.2213203435596)) ;
#95548=CARTESIAN_POINT('Origin',(29.2697227541073,254.722122022416,20.2213203435596)) ;
#95549=CARTESIAN_POINT('',(30.029721514783,255.291297809793,20.2213203435596)) ;
#95550=CARTESIAN_POINT('',(29.3377636979518,254.64883880496,20.2213203435596)) ;
#95551=CARTESIAN_POINT('',(29.8527789991768,255.263469667977,20.3213203435596)) ;
#95552=CARTESIAN_POINT('',(29.2697227541073,254.722122022416,20.3213203435596)) ;
#95553=CARTESIAN_POINT('Origin',(29.8527789991768,255.263469667977,20.2213203435596)) ;
#95554=CARTESIAN_POINT('Origin',(29.7856716932347,255.294762318656,20.2213203435596)) ;
#95555=CARTESIAN_POINT('',(29.5759716504483,255.502885786844,20.2213203435596)) ;
#95556=CARTESIAN_POINT('',(29.8279335194087,255.385393097359,20.2213203435596)) ;
#95557=CARTESIAN_POINT('',(29.4405240550635,255.455707305529,20.3213203435596)) ;
#95558=CARTESIAN_POINT('',(29.7856716932347,255.294762318656,20.3213203435596)) ;
#95559=CARTESIAN_POINT('Ctrl Pts',(29.4405240550636,255.455707305529,20.3213203435596)) ;
#95560=CARTESIAN_POINT('Ctrl Pts',(29.4408538386378,255.455825702211,20.3213203435596)) ;
#95561=CARTESIAN_POINT('Ctrl Pts',(29.4411836478927,255.455944032111,20.3213194308211)) ;
#95562=CARTESIAN_POINT('Ctrl Pts',(29.4569924888621,255.461612375186,20.3212319872543)) ;
#95563=CARTESIAN_POINT('Ctrl Pts',(29.4726867912404,255.46706644739,20.3191381135824)) ;
#95564=CARTESIAN_POINT('Ctrl Pts',(29.5017651669459,255.477084800126,20.3111718218544)) ;
#95565=CARTESIAN_POINT('Ctrl Pts',(29.51565798919,255.48183265499,20.3054342440869)) ;
#95566=CARTESIAN_POINT('Ctrl Pts',(29.5412810399391,255.490845015337,20.2893159232801)) ;
#95567=CARTESIAN_POINT('Ctrl Pts',(29.5521970843937,255.494745565626,20.2791809771031)) ;
#95568=CARTESIAN_POINT('Ctrl Pts',(29.5652171491802,255.499264264589,20.260871828191)) ;
#95569=CARTESIAN_POINT('Ctrl Pts',(29.5692328543724,255.500626571788,20.2533267661999)) ;
#95570=CARTESIAN_POINT('Ctrl Pts',(29.574609399851,255.502411678272,20.2375324969203)) ;
#95571=CARTESIAN_POINT('Ctrl Pts',(29.5760300223821,255.502857627139,20.2294989756937)) ;
#95572=CARTESIAN_POINT('Ctrl Pts',(29.5760287878866,255.502858202794,20.2213203435596)) ;
#95573=CARTESIAN_POINT('Ctrl Pts',(29.5299739324064,255.41100026533,20.2213203435596)) ;
#95574=CARTESIAN_POINT('Ctrl Pts',(29.6096016195701,255.57031939758,20.2213203435596)) ;
#95575=CARTESIAN_POINT('Ctrl Pts',(29.7125884839771,255.771554438639,20.2213203435596)) ;
#95576=CARTESIAN_POINT('Ctrl Pts',(29.8151211010034,255.998133968456,20.2213203435596)) ;
#95577=CARTESIAN_POINT('Ctrl Pts',(29.8513771953728,256.081187321587,20.2213203435596)) ;
#95578=CARTESIAN_POINT('Ctrl Pts',(29.8781139616688,256.143488201183,20.2213203435596)) ;
#95579=CARTESIAN_POINT('Ctrl Pts',(29.8995554831711,256.195063929691,20.2213203435596)) ;
#95580=CARTESIAN_POINT('Ctrl Pts',(29.9348455746236,256.276402827328,20.2213203435596)) ;
#95581=CARTESIAN_POINT('Ctrl Pts',(29.9896815685447,256.4130504425,20.2213203435596)) ;
#95582=CARTESIAN_POINT('Ctrl Pts',(30.1179835005034,256.525685163548,20.2213203435596)) ;
#95583=CARTESIAN_POINT('Ctrl Pts',(30.3645779003689,256.610912055866,20.2213203435596)) ;
#95584=CARTESIAN_POINT('Ctrl Pts',(30.5298821415626,256.643803992665,20.2213203435596)) ;
#95585=CARTESIAN_POINT('Ctrl Pts',(30.6155000490728,256.657966189434,20.2213203435596)) ;
#95586=CARTESIAN_POINT('Ctrl Pts',(29.5299739324064,255.41100026533,20.2512402735938)) ;
#95587=CARTESIAN_POINT('Ctrl Pts',(29.6096009693679,255.570318096655,20.2512402735938)) ;
#95588=CARTESIAN_POINT('Ctrl Pts',(29.712707938933,255.771649641491,20.2512402735938)) ;
#95589=CARTESIAN_POINT('Ctrl Pts',(29.8152362132554,255.998232225974,20.2512402735938)) ;
#95590=CARTESIAN_POINT('Ctrl Pts',(29.8515002767356,256.081293849312,20.2512402735938)) ;
#95591=CARTESIAN_POINT('Ctrl Pts',(29.8782395213483,256.143598800648,20.2512402735938)) ;
#95592=CARTESIAN_POINT('Ctrl Pts',(29.8996858196018,256.195177190556,20.2512402735938)) ;
#95593=CARTESIAN_POINT('Ctrl Pts',(29.934976344848,256.276518880556,20.2512402735938)) ;
#95594=CARTESIAN_POINT('Ctrl Pts',(29.9898180967585,256.413130044856,20.2512402735938)) ;
#95595=CARTESIAN_POINT('Ctrl Pts',(30.1179763379782,256.525623320505,20.2512402735938)) ;
#95596=CARTESIAN_POINT('Ctrl Pts',(30.3645571335651,256.610892638431,20.2512402735938)) ;
#95597=CARTESIAN_POINT('Ctrl Pts',(30.5298900347182,256.643805298284,20.2512402735938)) ;
#95598=CARTESIAN_POINT('Ctrl Pts',(30.6155000490728,256.657966189434,20.2512402735938)) ;
#95599=CARTESIAN_POINT('Ctrl Pts',(29.5074932885477,255.422236088995,20.3030173057519)) ;
#95600=CARTESIAN_POINT('Ctrl Pts',(29.5871722574481,255.58165782578,20.3030173057519)) ;
#95601=CARTESIAN_POINT('Ctrl Pts',(29.6898117905486,255.782015377311,20.3030173057519)) ;
#95602=CARTESIAN_POINT('Ctrl Pts',(29.7920157725665,256.007858969755,20.3030173057519)) ;
#95603=CARTESIAN_POINT('Ctrl Pts',(29.8281359664057,256.090623692282,20.3030173057519)) ;
#95604=CARTESIAN_POINT('Ctrl Pts',(29.8548106554516,256.152702041668,20.3030173057519)) ;
#95605=CARTESIAN_POINT('Ctrl Pts',(29.8762058240841,256.204312000057,20.3030173057519)) ;
#95606=CARTESIAN_POINT('Ctrl Pts',(29.9116403677314,256.285562615183,20.3030173057519)) ;
#95607=CARTESIAN_POINT('Ctrl Pts',(29.9666803048971,256.425572767907,20.3030173057519)) ;
#95608=CARTESIAN_POINT('Ctrl Pts',(30.1078757132933,256.55051479079,20.3030173057519)) ;
#95609=CARTESIAN_POINT('Ctrl Pts',(30.357955853848,256.634175797297,20.3030173057519)) ;
#95610=CARTESIAN_POINT('Ctrl Pts',(30.5251581921543,256.668496208837,20.3030173057519)) ;
#95611=CARTESIAN_POINT('Ctrl Pts',(30.611398636369,256.682761380411,20.3030173057519)) ;
#95612=CARTESIAN_POINT('Ctrl Pts',(29.4605965606009,255.445675069168,20.3213203435596)) ;
#95613=CARTESIAN_POINT('Ctrl Pts',(29.5403821390099,255.605310110332,20.3213203435596)) ;
#95614=CARTESIAN_POINT('Ctrl Pts',(29.6423652672512,255.803891903317,20.3213203435596)) ;
#95615=CARTESIAN_POINT('Ctrl Pts',(29.7438812213478,256.028201995047,20.3213203435596)) ;
#95616=CARTESIAN_POINT('Ctrl Pts',(29.7797224364993,256.110369300527,20.3213203435596)) ;
#95617=CARTESIAN_POINT('Ctrl Pts',(29.8062690330564,256.171985741807,20.3213203435596)) ;
#95618=CARTESIAN_POINT('Ctrl Pts',(29.8275702161123,256.223668617304,20.3213203435596)) ;
#95619=CARTESIAN_POINT('Ctrl Pts',(29.8633063467445,256.304736651538,20.3213203435596)) ;
#95620=CARTESIAN_POINT('Ctrl Pts',(29.9187749963249,256.451740686228,20.3213203435596)) ;
#95621=CARTESIAN_POINT('Ctrl Pts',(30.0867858579854,256.602276621519,20.3213203435596)) ;
#95622=CARTESIAN_POINT('Ctrl Pts',(30.3441298594353,256.682695120528,20.3213203435596)) ;
#95623=CARTESIAN_POINT('Ctrl Pts',(30.5153080708237,256.720007224649,20.3213203435596)) ;
#95624=CARTESIAN_POINT('Ctrl Pts',(30.6028427054544,256.734486470356,20.3213203435596)) ;
#95625=CARTESIAN_POINT('Ctrl Pts',(29.4405240550634,255.455707305529,20.3213203435596)) ;
#95626=CARTESIAN_POINT('Ctrl Pts',(29.5203551947139,255.615433505657,20.3213203435596)) ;
#95627=CARTESIAN_POINT('Ctrl Pts',(29.6220701604893,255.813265522892,20.3213203435596)) ;
#95628=CARTESIAN_POINT('Ctrl Pts',(29.7232911658707,256.03691957849,20.3213203435596)) ;
#95629=CARTESIAN_POINT('Ctrl Pts',(29.7590138224883,256.118832061085,20.3213203435596)) ;
#95630=CARTESIAN_POINT('Ctrl Pts',(29.785505857421,256.180251232298,20.3213203435596)) ;
#95631=CARTESIAN_POINT('Ctrl Pts',(29.8067673218597,256.231965600798,20.3213203435596)) ;
#95632=CARTESIAN_POINT('Ctrl Pts',(29.8426325824515,256.31295578499,20.3213203435596)) ;
#95633=CARTESIAN_POINT('Ctrl Pts',(29.8982853405048,256.462949425189,20.3213203435596)) ;
#95634=CARTESIAN_POINT('Ctrl Pts',(30.0777583197704,256.624424879292,20.3213203435596)) ;
#95635=CARTESIAN_POINT('Ctrl Pts',(30.3382099144606,256.703460053722,20.3213203435596)) ;
#95636=CARTESIAN_POINT('Ctrl Pts',(30.5110929110685,256.742054853877,20.3213203435596)) ;
#95637=CARTESIAN_POINT('Ctrl Pts',(30.5991806382232,256.756625587514,20.3213203435596)) ;
#95638=CARTESIAN_POINT('',(30.6155000490728,256.657966189434,20.2213203435596)) ;
#95639=CARTESIAN_POINT('Ctrl Pts',(30.6155000490728,256.657966189434,20.2213203435596)) ;
#95640=CARTESIAN_POINT('Ctrl Pts',(30.5934162583261,256.654313273834,20.2213203435596)) ;
#95641=CARTESIAN_POINT('Ctrl Pts',(30.5716039157812,256.650478363725,20.2213203435596)) ;
#95642=CARTESIAN_POINT('Ctrl Pts',(30.5499306316617,256.646421331829,20.2213203435596)) ;
#95643=CARTESIAN_POINT('Ctrl Pts',(30.5289501530439,256.642493986509,20.2213203435596)) ;
#95644=CARTESIAN_POINT('Ctrl Pts',(30.5080997796798,256.638358378979,20.2213203435596)) ;
#95645=CARTESIAN_POINT('Ctrl Pts',(30.4873064930217,256.633971075942,20.2213203435596)) ;
#95646=CARTESIAN_POINT('Ctrl Pts',(30.4672536265848,256.629739998706,20.2213203435596)) ;
#95647=CARTESIAN_POINT('Ctrl Pts',(30.4472536147319,256.625274726044,20.2213203435596)) ;
#95648=CARTESIAN_POINT('Ctrl Pts',(30.4272886443642,256.620531223793,20.2213203435596)) ;
#95649=CARTESIAN_POINT('Ctrl Pts',(30.4142897652556,256.617442803866,20.2213203435596)) ;
#95650=CARTESIAN_POINT('Ctrl Pts',(30.4013066983077,256.614236338128,20.2213203435596)) ;
#95651=CARTESIAN_POINT('Ctrl Pts',(30.388346948028,256.6108987856,20.2213203435596)) ;
#95652=CARTESIAN_POINT('Ctrl Pts',(30.3819900047351,256.609261668241,20.2213203435596)) ;
#95653=CARTESIAN_POINT('Ctrl Pts',(30.3756388304382,256.607593001585,20.2213203435596)) ;
#95654=CARTESIAN_POINT('Ctrl Pts',(30.3692952787652,256.605891200963,20.2213203435596)) ;
#95655=CARTESIAN_POINT('Ctrl Pts',(30.3643550423544,256.604565871268,20.2213203435596)) ;
#95656=CARTESIAN_POINT('Ctrl Pts',(30.3594204422208,256.603220681278,20.2213203435596)) ;
#95657=CARTESIAN_POINT('Ctrl Pts',(30.3545032359515,256.601857933052,20.2213203435596)) ;
#95658=CARTESIAN_POINT('Ctrl Pts',(30.3380407124697,256.597295530452,20.2213203435596)) ;
#95659=CARTESIAN_POINT('Ctrl Pts',(30.3217321675932,256.592526619223,20.2213203435596)) ;
#95660=CARTESIAN_POINT('Ctrl Pts',(30.3055753847063,256.587509301036,20.2213203435596)) ;
#95661=CARTESIAN_POINT('Ctrl Pts',(30.2899301860841,256.582650849936,20.2213203435596)) ;
#95662=CARTESIAN_POINT('Ctrl Pts',(30.2744270028255,256.577559375667,20.2213203435596)) ;
#95663=CARTESIAN_POINT('Ctrl Pts',(30.259111696462,256.572195013264,20.2213203435596)) ;
#95664=CARTESIAN_POINT('Ctrl Pts',(30.2445222032144,256.567084875263,20.2213203435596)) ;
#95665=CARTESIAN_POINT('Ctrl Pts',(30.2301030378545,256.561727000506,20.2213203435596)) ;
#95666=CARTESIAN_POINT('Ctrl Pts',(30.2159410139053,256.556086667428,20.2213203435596)) ;
#95667=CARTESIAN_POINT('Ctrl Pts',(30.2097149645829,256.553607008302,20.2213203435596)) ;
#95668=CARTESIAN_POINT('Ctrl Pts',(30.203539260331,256.551072762465,20.2213203435596)) ;
#95669=CARTESIAN_POINT('Ctrl Pts',(30.1974245258637,256.548481045224,20.2213203435596)) ;
#95670=CARTESIAN_POINT('Ctrl Pts',(30.1828338390648,256.542296813556,20.2213203435596)) ;
#95671=CARTESIAN_POINT('Ctrl Pts',(30.1687288435062,256.536122143351,20.2213203435596)) ;
#95672=CARTESIAN_POINT('Ctrl Pts',(30.1551584931796,256.529847245861,20.2213203435596)) ;
#95673=CARTESIAN_POINT('Ctrl Pts',(30.1514273273943,256.528121963738,20.2213203435596)) ;
#95674=CARTESIAN_POINT('Ctrl Pts',(30.1477365791022,256.526388810279,20.2213203435596)) ;
#95675=CARTESIAN_POINT('Ctrl Pts',(30.1440871984713,256.524644752035,20.2213203435596)) ;
#95676=CARTESIAN_POINT('Ctrl Pts',(30.1411815402234,256.523256122639,20.2213203435596)) ;
#95677=CARTESIAN_POINT('Ctrl Pts',(30.138302106203,256.521860573952,20.2213203435596)) ;
#95678=CARTESIAN_POINT('Ctrl Pts',(30.135449332951,256.520456391843,20.2213203435596)) ;
#95679=CARTESIAN_POINT('Ctrl Pts',(30.1335861372718,256.519539296158,20.2213203435596)) ;
#95680=CARTESIAN_POINT('Ctrl Pts',(30.1317325967933,256.518617702671,20.2213203435596)) ;
#95681=CARTESIAN_POINT('Ctrl Pts',(30.1298799116381,256.517686461576,20.2213203435596)) ;
#95682=CARTESIAN_POINT('Ctrl Pts',(30.1218807340664,256.513665722888,20.2213203435596)) ;
#95683=CARTESIAN_POINT('Ctrl Pts',(30.1139562040359,256.509493804869,20.2213203435596)) ;
#95684=CARTESIAN_POINT('Ctrl Pts',(30.1062297261487,256.505164397409,20.2213203435596)) ;
#95685=CARTESIAN_POINT('Ctrl Pts',(30.0983390998272,256.500743012018,20.2213203435596)) ;
#95686=CARTESIAN_POINT('Ctrl Pts',(30.0906551333939,256.496157031995,20.2213203435596)) ;
#95687=CARTESIAN_POINT('Ctrl Pts',(30.0832576762508,256.491379023066,20.2213203435596)) ;
#95688=CARTESIAN_POINT('Ctrl Pts',(30.0755133796667,256.486376990948,20.2213203435596)) ;
#95689=CARTESIAN_POINT('Ctrl Pts',(30.0680830047494,256.481163853088,20.2213203435596)) ;
#95690=CARTESIAN_POINT('Ctrl Pts',(30.0610015763669,256.475693171023,20.2213203435596)) ;
#95691=CARTESIAN_POINT('Ctrl Pts',(30.0534085353477,256.469827248065,20.2213203435596)) ;
#95692=CARTESIAN_POINT('Ctrl Pts',(30.0462162092421,256.463663963291,20.2213203435596)) ;
#95693=CARTESIAN_POINT('Ctrl Pts',(30.0394079239686,256.457144203383,20.2213203435596)) ;
#95694=CARTESIAN_POINT('Ctrl Pts',(30.0323252760618,256.450361707937,20.2213203435596)) ;
#95695=CARTESIAN_POINT('Ctrl Pts',(30.0256567171885,256.443191537756,20.2213203435596)) ;
#95696=CARTESIAN_POINT('Ctrl Pts',(30.0193370543812,256.435590226317,20.2213203435596)) ;
#95697=CARTESIAN_POINT('Ctrl Pts',(30.0134514152341,256.42851095998,20.2213203435596)) ;
#95698=CARTESIAN_POINT('Ctrl Pts',(30.0078666198455,256.421056878535,20.2213203435596)) ;
#95699=CARTESIAN_POINT('Ctrl Pts',(30.0025158682114,256.41323156183,20.2213203435596)) ;
#95700=CARTESIAN_POINT('Ctrl Pts',(29.9974204876885,256.405779717855,20.2213203435596)) ;
#95701=CARTESIAN_POINT('Ctrl Pts',(29.9925362825257,256.397990818504,20.2213203435596)) ;
#95702=CARTESIAN_POINT('Ctrl Pts',(29.9878117975722,256.389913149835,20.2213203435596)) ;
#95703=CARTESIAN_POINT('Ctrl Pts',(29.9850035581777,256.385111774109,20.2213203435596)) ;
#95704=CARTESIAN_POINT('Ctrl Pts',(29.9822527683305,256.380210786577,20.2213203435596)) ;
#95705=CARTESIAN_POINT('Ctrl Pts',(29.9795492395846,256.375224378147,20.2213203435596)) ;
#95706=CARTESIAN_POINT('Ctrl Pts',(29.973935966022,256.36487121484,20.2213203435596)) ;
#95707=CARTESIAN_POINT('Ctrl Pts',(29.9685037596898,256.354113134005,20.2213203435596)) ;
#95708=CARTESIAN_POINT('Ctrl Pts',(29.9631379985744,256.342986062281,20.2213203435596)) ;
#95709=CARTESIAN_POINT('Ctrl Pts',(29.9575091150603,256.331313349083,20.2213203435596)) ;
#95710=CARTESIAN_POINT('Ctrl Pts',(29.951953721328,256.319234967557,20.2213203435596)) ;
#95711=CARTESIAN_POINT('Ctrl Pts',(29.9463917654129,256.306822917892,20.2213203435596)) ;
#95712=CARTESIAN_POINT('Ctrl Pts',(29.940330026839,256.293295554248,20.2213203435596)) ;
#95713=CARTESIAN_POINT('Ctrl Pts',(29.9342606912573,256.279372250169,20.2213203435596)) ;
#95714=CARTESIAN_POINT('Ctrl Pts',(29.9281366213413,256.265175509829,20.2213203435596)) ;
#95715=CARTESIAN_POINT('Ctrl Pts',(29.9250495282719,256.258019050266,20.2213203435596)) ;
#95716=CARTESIAN_POINT('Ctrl Pts',(29.9219493584908,256.250793510573,20.2213203435596)) ;
#95717=CARTESIAN_POINT('Ctrl Pts',(29.9188345104747,256.243516527177,20.2213203435596)) ;
#95718=CARTESIAN_POINT('Ctrl Pts',(29.917799703434,256.241098985899,20.2213203435596)) ;
#95719=CARTESIAN_POINT('Ctrl Pts',(29.9167633738339,256.238680704014,20.2213203435596)) ;
#95720=CARTESIAN_POINT('Ctrl Pts',(29.9157260475512,256.236262805576,20.2213203435596)) ;
#95721=CARTESIAN_POINT('Ctrl Pts',(29.9114086798316,256.226199475615,20.2213203435596)) ;
#95722=CARTESIAN_POINT('Ctrl Pts',(29.9070371070764,256.216056684626,20.2213203435596)) ;
#95723=CARTESIAN_POINT('Ctrl Pts',(29.9026389079555,256.20589382332,20.2213203435596)) ;
#95724=CARTESIAN_POINT('Ctrl Pts',(29.8967419008071,256.192267685866,20.2213203435596)) ;
#95725=CARTESIAN_POINT('Ctrl Pts',(29.8907954352119,256.178601428562,20.2213203435596)) ;
#95726=CARTESIAN_POINT('Ctrl Pts',(29.8848059534797,256.164901729482,20.2213203435596)) ;
#95727=CARTESIAN_POINT('Ctrl Pts',(29.8803666705202,256.154747789058,20.2213203435596)) ;
#95728=CARTESIAN_POINT('Ctrl Pts',(29.8759018339445,256.144571176857,20.2213203435596)) ;
#95729=CARTESIAN_POINT('Ctrl Pts',(29.8714117082223,256.13437046548,20.2213203435596)) ;
#95730=CARTESIAN_POINT('Ctrl Pts',(29.8630996041311,256.115486946395,20.2213203435596)) ;
#95731=CARTESIAN_POINT('Ctrl Pts',(29.8547089250513,256.096539146837,20.2213203435596)) ;
#95732=CARTESIAN_POINT('Ctrl Pts',(29.8462711252824,256.077589395044,20.2213203435596)) ;
#95733=CARTESIAN_POINT('Ctrl Pts',(29.8377907984774,256.058544135322,20.2213203435596)) ;
#95734=CARTESIAN_POINT('Ctrl Pts',(29.82926345751,256.039498220475,20.2213203435596)) ;
#95735=CARTESIAN_POINT('Ctrl Pts',(29.820704336771,256.020480351935,20.2213203435596)) ;
#95736=CARTESIAN_POINT('Ctrl Pts',(29.8109891323347,255.998893732649,20.2213203435596)) ;
#95737=CARTESIAN_POINT('Ctrl Pts',(29.8012292399256,255.977334867106,20.2213203435596)) ;
#95738=CARTESIAN_POINT('Ctrl Pts',(29.791431425698,255.955815501484,20.2213203435596)) ;
#95739=CARTESIAN_POINT('Ctrl Pts',(29.7810056880256,255.932917000284,20.2213203435596)) ;
#95740=CARTESIAN_POINT('Ctrl Pts',(29.7705369433913,255.910062911148,20.2213203435596)) ;
#95741=CARTESIAN_POINT('Ctrl Pts',(29.7600080208177,255.887217116999,20.2213203435596)) ;
#95742=CARTESIAN_POINT('Ctrl Pts',(29.7465625544269,255.858042967863,20.2213203435596)) ;
#95743=CARTESIAN_POINT('Ctrl Pts',(29.7330220922707,255.82888937671,20.2213203435596)) ;
#95744=CARTESIAN_POINT('Ctrl Pts',(29.7194047389056,255.799807444113,20.2213203435596)) ;
#95745=CARTESIAN_POINT('Ctrl Pts',(29.7026300227241,255.763982482224,20.2213203435596)) ;
#95746=CARTESIAN_POINT('Ctrl Pts',(29.6857384416576,255.728264855005,20.2213203435596)) ;
#95747=CARTESIAN_POINT('Ctrl Pts',(29.6687236887841,255.692681924167,20.2213203435596)) ;
#95748=CARTESIAN_POINT('Ctrl Pts',(29.651375474443,255.656401625791,20.2213203435596)) ;
#95749=CARTESIAN_POINT('Ctrl Pts',(29.6338974093498,255.620256710442,20.2213203435596)) ;
#95750=CARTESIAN_POINT('Ctrl Pts',(29.6162632186691,255.584264740826,20.2213203435596)) ;
#95751=CARTESIAN_POINT('Ctrl Pts',(29.60292557718,255.557042170994,20.2213203435596)) ;
#95752=CARTESIAN_POINT('Ctrl Pts',(29.5894980112796,255.52990631417,20.2213203435596)) ;
#95753=CARTESIAN_POINT('Ctrl Pts',(29.5759716504483,255.502885786844,20.2213203435596)) ;
#95754=CARTESIAN_POINT('',(30.5008469122091,256.738337318211,20.3213203435596)) ;
#95755=CARTESIAN_POINT('Ctrl Pts',(29.4405240550634,255.455707305529,20.3213203435596)) ;
#95756=CARTESIAN_POINT('Ctrl Pts',(29.5203551947139,255.615433505657,20.3213203435596)) ;
#95757=CARTESIAN_POINT('Ctrl Pts',(29.6220701604893,255.813265522892,20.3213203435596)) ;
#95758=CARTESIAN_POINT('Ctrl Pts',(29.7232911658707,256.03691957849,20.3213203435596)) ;
#95759=CARTESIAN_POINT('Ctrl Pts',(29.7590138224883,256.118832061085,20.3213203435596)) ;
#95760=CARTESIAN_POINT('Ctrl Pts',(29.785505857421,256.180251232298,20.3213203435596)) ;
#95761=CARTESIAN_POINT('Ctrl Pts',(29.8067673218597,256.231965600798,20.3213203435596)) ;
#95762=CARTESIAN_POINT('Ctrl Pts',(29.8426325824515,256.31295578499,20.3213203435596)) ;
#95763=CARTESIAN_POINT('Ctrl Pts',(29.8982853405048,256.462949425189,20.3213203435596)) ;
#95764=CARTESIAN_POINT('Ctrl Pts',(30.0777583197704,256.624424879292,20.3213203435596)) ;
#95765=CARTESIAN_POINT('Ctrl Pts',(30.3057090045425,256.693597510598,20.3213203435596)) ;
#95766=CARTESIAN_POINT('Ctrl Pts',(30.446346059137,256.727112644825,20.3213203435596)) ;
#95767=CARTESIAN_POINT('Ctrl Pts',(30.5008469122103,256.738337318211,20.3213203435596)) ;
#95768=CARTESIAN_POINT('Ctrl Pts',(30.5008469122093,256.73833731821,20.3213203435596)) ;
#95769=CARTESIAN_POINT('Ctrl Pts',(30.5011281297113,256.738149508513,20.3213203435596)) ;
#95770=CARTESIAN_POINT('Ctrl Pts',(30.5014092894833,256.737961609899,20.3213194299206)) ;
#95771=CARTESIAN_POINT('Ctrl Pts',(30.5150875989089,256.728814269044,20.3212305906335)) ;
#95772=CARTESIAN_POINT('Ctrl Pts',(30.5284725288954,256.719563247393,20.3190721427316)) ;
#95773=CARTESIAN_POINT('Ctrl Pts',(30.5531946098367,256.70222613735,20.3109405228244)) ;
#95774=CARTESIAN_POINT('Ctrl Pts',(30.5649646262603,256.693857183022,20.3050698997908)) ;
#95775=CARTESIAN_POINT('Ctrl Pts',(30.5866919680773,256.678623368935,20.2887421025002)) ;
#95776=CARTESIAN_POINT('Ctrl Pts',(30.5959391028663,256.672153993788,20.2785447738736)) ;
#95777=CARTESIAN_POINT('Ctrl Pts',(30.6067555479079,256.66441843623,20.2602592440806)) ;
#95778=CARTESIAN_POINT('Ctrl Pts',(30.6100239931557,256.662039953674,20.2528168931027)) ;
#95779=CARTESIAN_POINT('Ctrl Pts',(30.6143734110351,256.658828819451,20.2372682660181)) ;
#95780=CARTESIAN_POINT('Ctrl Pts',(30.6155000490728,256.657966189434,20.2293609459321)) ;
#95781=CARTESIAN_POINT('Ctrl Pts',(30.6155000490728,256.657966189434,20.2213203435596)) ;
#95782=CARTESIAN_POINT('Origin',(30.5923736638261,256.185010099112,20.2213203435596)) ;
#95783=CARTESIAN_POINT('',(30.6910330619062,256.201329509961,20.2213203435596)) ;
#95784=CARTESIAN_POINT('',(30.5923736638261,256.185010099112,20.3213203435596)) ;
#95785=CARTESIAN_POINT('Origin',(30.029721514783,255.291297809793,20.0213203435596)) ;
#95786=CARTESIAN_POINT('',(29.5759712687712,255.502885024399,20.1213203435596)) ;
#95787=CARTESIAN_POINT('',(29.5759712687709,255.502885024398,20.0213203435596)) ;
#95788=CARTESIAN_POINT('',(30.029721514783,255.291297809793,20.1213203435596)) ;
#95789=CARTESIAN_POINT('',(43.1641155815879,249.166629271216,20.1213203435596)) ;
#95790=CARTESIAN_POINT('',(30.029721514783,255.291297809793,20.0213203435596)) ;
#95791=CARTESIAN_POINT('Ctrl Pts',(29.5759712687716,255.502885024399,20.0213203435596)) ;
#95792=CARTESIAN_POINT('Ctrl Pts',(29.5759712687716,255.502885024399,20.3813203435596)) ;
#95793=CARTESIAN_POINT('Ctrl Pts',(29.7060244888525,255.762681865726,20.0213203435596)) ;
#95794=CARTESIAN_POINT('Ctrl Pts',(29.7060244888525,255.762681865726,20.3813203435596)) ;
#95795=CARTESIAN_POINT('Ctrl Pts',(29.8400217958637,256.05939235397,20.0213203435596)) ;
#95796=CARTESIAN_POINT('Ctrl Pts',(29.8400217958637,256.05939235397,20.3813203435596)) ;
#95797=CARTESIAN_POINT('Ctrl Pts',(29.9188345104747,256.243516527177,20.0213203435596)) ;
#95798=CARTESIAN_POINT('Ctrl Pts',(29.9188345104747,256.243516527177,20.3813203435596)) ;
#95799=CARTESIAN_POINT('Ctrl Pts',(30.0015982144022,256.436871097342,20.0213203435596)) ;
#95800=CARTESIAN_POINT('Ctrl Pts',(30.0015982144022,256.436871097342,20.3813203435596)) ;
#95801=CARTESIAN_POINT('Ctrl Pts',(30.0230446934974,256.474570522956,20.0213203435596)) ;
#95802=CARTESIAN_POINT('Ctrl Pts',(30.0230446934974,256.474570522956,20.3813203435596)) ;
#95803=CARTESIAN_POINT('Ctrl Pts',(30.1974245258637,256.548481045224,20.0213203435596)) ;
#95804=CARTESIAN_POINT('Ctrl Pts',(30.1974245258637,256.548481045224,20.3813203435596)) ;
#95805=CARTESIAN_POINT('Ctrl Pts',(30.2961501724434,256.590325701232,20.0213203435596)) ;
#95806=CARTESIAN_POINT('Ctrl Pts',(30.2961501724434,256.590325701232,20.3813203435596)) ;
#95807=CARTESIAN_POINT('Ctrl Pts',(30.4375870001386,256.628537303818,20.0213203435596)) ;
#95808=CARTESIAN_POINT('Ctrl Pts',(30.4375870001386,256.628537303818,20.3813203435596)) ;
#95809=CARTESIAN_POINT('Ctrl Pts',(30.6155000490728,256.657966189434,20.0213203435596)) ;
#95810=CARTESIAN_POINT('Ctrl Pts',(30.6155000490728,256.657966189434,20.3813203435596)) ;
#95811=CARTESIAN_POINT('',(30.6155000490728,256.657966189434,20.1213203435596)) ;
#95812=CARTESIAN_POINT('',(30.6155000490728,256.657966189434,20.0213203435596)) ;
#95813=CARTESIAN_POINT('Ctrl Pts',(29.5759712687716,255.502885024399,20.1213203435596)) ;
#95814=CARTESIAN_POINT('Ctrl Pts',(29.5913953099987,255.533696389076,20.1213203435596)) ;
#95815=CARTESIAN_POINT('Ctrl Pts',(29.606657599885,255.564590752194,20.1213203435596)) ;
#95816=CARTESIAN_POINT('Ctrl Pts',(29.6217610079184,255.595501219028,20.1213203435596)) ;
#95817=CARTESIAN_POINT('Ctrl Pts',(29.6375733914914,255.627862667312,20.1213203435596)) ;
#95818=CARTESIAN_POINT('Ctrl Pts',(29.6532125375535,255.660243957624,20.1213203435596)) ;
#95819=CARTESIAN_POINT('Ctrl Pts',(29.6686892717481,255.692609948402,20.1213203435596)) ;
#95820=CARTESIAN_POINT('Ctrl Pts',(29.672942829729,255.701505275843,20.1213203435596)) ;
#95821=CARTESIAN_POINT('Ctrl Pts',(29.6771854330678,255.71040235893,20.1213203435596)) ;
#95822=CARTESIAN_POINT('Ctrl Pts',(29.6814079996186,255.719281115549,20.1213203435596)) ;
#95823=CARTESIAN_POINT('Ctrl Pts',(29.6963375495941,255.75067335983,20.1213203435596)) ;
#95824=CARTESIAN_POINT('Ctrl Pts',(29.7110459269022,255.781895244612,20.1213203435596)) ;
#95825=CARTESIAN_POINT('Ctrl Pts',(29.7256409125464,255.813142245774,20.1213203435596)) ;
#95826=CARTESIAN_POINT('Ctrl Pts',(29.737497273023,255.838526012405,20.1213203435596)) ;
#95827=CARTESIAN_POINT('Ctrl Pts',(29.7492789979749,255.863927567679,20.1213203435596)) ;
#95828=CARTESIAN_POINT('Ctrl Pts',(29.7610245812382,255.889423296196,20.1213203435596)) ;
#95829=CARTESIAN_POINT('Ctrl Pts',(29.7715454768417,255.912260637863,20.1213203435596)) ;
#95830=CARTESIAN_POINT('Ctrl Pts',(29.7820375533546,255.93517417614,20.1213203435596)) ;
#95831=CARTESIAN_POINT('Ctrl Pts',(29.7925088651715,255.958182425098,20.1213203435596)) ;
#95832=CARTESIAN_POINT('Ctrl Pts',(29.8021506276027,255.979367934068,20.1213203435596)) ;
#95833=CARTESIAN_POINT('Ctrl Pts',(29.8117749431216,256.000634221753,20.1213203435596)) ;
#95834=CARTESIAN_POINT('Ctrl Pts',(29.8213682132304,256.021955645211,20.1213203435596)) ;
#95835=CARTESIAN_POINT('Ctrl Pts',(29.8296255852217,256.040307982096,20.1213203435596)) ;
#95836=CARTESIAN_POINT('Ctrl Pts',(29.8378598391904,256.058700999499,20.1213203435596)) ;
#95837=CARTESIAN_POINT('Ctrl Pts',(29.8460471694367,256.077086455705,20.1213203435596)) ;
#95838=CARTESIAN_POINT('Ctrl Pts',(29.8503425417667,256.086732137202,20.1213203435596)) ;
#95839=CARTESIAN_POINT('Ctrl Pts',(29.8546247428343,256.096375192364,20.1213203435596)) ;
#95840=CARTESIAN_POINT('Ctrl Pts',(29.8588884181389,256.106004515113,20.1213203435596)) ;
#95841=CARTESIAN_POINT('Ctrl Pts',(29.8628290229948,256.114904197494,20.1213203435596)) ;
#95842=CARTESIAN_POINT('Ctrl Pts',(29.8667535356127,256.123791473506,20.1213203435596)) ;
#95843=CARTESIAN_POINT('Ctrl Pts',(29.8706737970368,256.132694372067,20.1213203435596)) ;
#95844=CARTESIAN_POINT('Ctrl Pts',(29.8765711738735,256.146087292099,20.1213203435596)) ;
#95845=CARTESIAN_POINT('Ctrl Pts',(29.8824574550096,256.159512078262,20.1213203435596)) ;
#95846=CARTESIAN_POINT('Ctrl Pts',(29.8883430841851,256.172999840968,20.1213203435596)) ;
#95847=CARTESIAN_POINT('Ctrl Pts',(29.8934307149093,256.184658875864,20.1213203435596)) ;
#95848=CARTESIAN_POINT('Ctrl Pts',(29.898517743333,256.196364776907,20.1213203435596)) ;
#95849=CARTESIAN_POINT('Ctrl Pts',(29.9035963493755,256.208106827721,20.1213203435596)) ;
#95850=CARTESIAN_POINT('Ctrl Pts',(29.905695121645,256.212959318824,20.1213203435596)) ;
#95851=CARTESIAN_POINT('Ctrl Pts',(29.9077913676636,256.217815491281,20.1213203435596)) ;
#95852=CARTESIAN_POINT('Ctrl Pts',(29.9098864190254,256.222679100839,20.1213203435596)) ;
#95853=CARTESIAN_POINT('Ctrl Pts',(29.912860969859,256.229584446516,20.1213203435596)) ;
#95854=CARTESIAN_POINT('Ctrl Pts',(29.9158371382348,256.236513993535,20.1213203435596)) ;
#95855=CARTESIAN_POINT('Ctrl Pts',(29.9188345104747,256.243516527177,20.1213203435596)) ;
#95856=CARTESIAN_POINT('Ctrl Pts',(29.9220123338014,256.250940635019,20.1213203435596)) ;
#95857=CARTESIAN_POINT('Ctrl Pts',(29.925212850827,256.258400497147,20.1213203435596)) ;
#95858=CARTESIAN_POINT('Ctrl Pts',(29.928467485032,256.265942362595,20.1213203435596)) ;
#95859=CARTESIAN_POINT('Ctrl Pts',(29.9334713297245,256.277537620624,20.1213203435596)) ;
#95860=CARTESIAN_POINT('Ctrl Pts',(29.9385989767258,256.289323440153,20.1213203435596)) ;
#95861=CARTESIAN_POINT('Ctrl Pts',(29.9439045097073,256.30125136341,20.1213203435596)) ;
#95862=CARTESIAN_POINT('Ctrl Pts',(29.9465408387867,256.307178370375,20.1213203435596)) ;
#95863=CARTESIAN_POINT('Ctrl Pts',(29.9492214566145,256.313139672616,20.1213203435596)) ;
#95864=CARTESIAN_POINT('Ctrl Pts',(29.951956258577,256.319123975837,20.1213203435596)) ;
#95865=CARTESIAN_POINT('Ctrl Pts',(29.9533078440368,256.322081519868,20.1213203435596)) ;
#95866=CARTESIAN_POINT('Ctrl Pts',(29.9546721053878,256.325043308408,20.1213203435596)) ;
#95867=CARTESIAN_POINT('Ctrl Pts',(29.956050766892,256.328008190301,20.1213203435596)) ;
#95868=CARTESIAN_POINT('Ctrl Pts',(29.9589666164282,256.334278873472,20.1213203435596)) ;
#95869=CARTESIAN_POINT('Ctrl Pts',(29.9619550897243,256.340585078762,20.1213203435596)) ;
#95870=CARTESIAN_POINT('Ctrl Pts',(29.9651070813677,256.347046007774,20.1213203435596)) ;
#95871=CARTESIAN_POINT('Ctrl Pts',(29.9681841792228,256.353353420057,20.1213203435596)) ;
#95872=CARTESIAN_POINT('Ctrl Pts',(29.9714161991448,256.35980818082,20.1213203435596)) ;
#95873=CARTESIAN_POINT('Ctrl Pts',(29.9748955028022,256.366473500977,20.1213203435596)) ;
#95874=CARTESIAN_POINT('Ctrl Pts',(29.9764839882022,256.36951657074,20.1213203435596)) ;
#95875=CARTESIAN_POINT('Ctrl Pts',(29.9781242063225,256.372602871453,20.1213203435596)) ;
#95876=CARTESIAN_POINT('Ctrl Pts',(29.9798264965544,256.375735147287,20.1213203435596)) ;
#95877=CARTESIAN_POINT('Ctrl Pts',(29.9815832708521,256.378967675781,20.1213203435596)) ;
#95878=CARTESIAN_POINT('Ctrl Pts',(29.9834033211469,256.382244469693,20.1213203435596)) ;
#95879=CARTESIAN_POINT('Ctrl Pts',(29.9853133457605,256.385589444858,20.1213203435596)) ;
#95880=CARTESIAN_POINT('Ctrl Pts',(29.9886267348614,256.391392094821,20.1213203435596)) ;
#95881=CARTESIAN_POINT('Ctrl Pts',(29.9921970041105,256.397371990751,20.1213203435596)) ;
#95882=CARTESIAN_POINT('Ctrl Pts',(29.9960076069629,256.403360144144,20.1213203435596)) ;
#95883=CARTESIAN_POINT('Ctrl Pts',(29.9998805570769,256.40944627284,20.1213203435596)) ;
#95884=CARTESIAN_POINT('Ctrl Pts',(30.0040023918854,256.415540642767,20.1213203435596)) ;
#95885=CARTESIAN_POINT('Ctrl Pts',(30.0083734751479,256.421518111582,20.1213203435596)) ;
#95886=CARTESIAN_POINT('Ctrl Pts',(30.0129328358726,256.427753050362,20.1213203435596)) ;
#95887=CARTESIAN_POINT('Ctrl Pts',(30.0177646044409,256.433860953415,20.1213203435596)) ;
#95888=CARTESIAN_POINT('Ctrl Pts',(30.0228741686605,256.439757844301,20.1213203435596)) ;
#95889=CARTESIAN_POINT('Ctrl Pts',(30.0246611862642,256.441820221319,20.1213203435596)) ;
#95890=CARTESIAN_POINT('Ctrl Pts',(30.0264821328035,256.443857271186,20.1213203435596)) ;
#95891=CARTESIAN_POINT('Ctrl Pts',(30.0283368868403,256.445866834091,20.1213203435596)) ;
#95892=CARTESIAN_POINT('Ctrl Pts',(30.0298862112431,256.447545474377,20.1213203435596)) ;
#95893=CARTESIAN_POINT('Ctrl Pts',(30.0314569037599,256.449202440719,20.1213203435596)) ;
#95894=CARTESIAN_POINT('Ctrl Pts',(30.033042872478,256.450831503359,20.1213203435596)) ;
#95895=CARTESIAN_POINT('Ctrl Pts',(30.0386707717201,256.456612323806,20.1213203435596)) ;
#95896=CARTESIAN_POINT('Ctrl Pts',(30.0445161457859,256.462064166021,20.1213203435596)) ;
#95897=CARTESIAN_POINT('Ctrl Pts',(30.0505343605665,256.467198645817,20.1213203435596)) ;
#95898=CARTESIAN_POINT('Ctrl Pts',(30.0562706995585,256.472092641418,20.1213203435596)) ;
#95899=CARTESIAN_POINT('Ctrl Pts',(30.0621643768898,256.476699356839,20.1213203435596)) ;
#95900=CARTESIAN_POINT('Ctrl Pts',(30.0681284991347,256.481029630627,20.1213203435596)) ;
#95901=CARTESIAN_POINT('Ctrl Pts',(30.0737341056397,256.485099602689,20.1213203435596)) ;
#95902=CARTESIAN_POINT('Ctrl Pts',(30.0794015874553,256.488925833284,20.1213203435596)) ;
#95903=CARTESIAN_POINT('Ctrl Pts',(30.0850160332146,256.492507744526,20.1213203435596)) ;
#95904=CARTESIAN_POINT('Ctrl Pts',(30.0872502332293,256.493933122292,20.1213203435596)) ;
#95905=CARTESIAN_POINT('Ctrl Pts',(30.0894737911333,256.495318583433,20.1213203435596)) ;
#95906=CARTESIAN_POINT('Ctrl Pts',(30.091683401717,256.49666693007,20.1213203435596)) ;
#95907=CARTESIAN_POINT('Ctrl Pts',(30.0990683870628,256.501173389365,20.1213203435596)) ;
#95908=CARTESIAN_POINT('Ctrl Pts',(30.1063559904706,256.505305915035,20.1213203435596)) ;
#95909=CARTESIAN_POINT('Ctrl Pts',(30.113544973547,256.509186721459,20.1213203435596)) ;
#95910=CARTESIAN_POINT('Ctrl Pts',(30.1206692308092,256.513032587147,20.1213203435596)) ;
#95911=CARTESIAN_POINT('Ctrl Pts',(30.1276961540222,256.516629737619,20.1213203435596)) ;
#95912=CARTESIAN_POINT('Ctrl Pts',(30.1346612641855,256.520067935113,20.1213203435596)) ;
#95913=CARTESIAN_POINT('Ctrl Pts',(30.1389827717456,256.522201167196,20.1213203435596)) ;
#95914=CARTESIAN_POINT('Ctrl Pts',(30.1432812579292,256.524272756909,20.1213203435596)) ;
#95915=CARTESIAN_POINT('Ctrl Pts',(30.1475731986693,256.526301573969,20.1213203435596)) ;
#95916=CARTESIAN_POINT('Ctrl Pts',(30.1508165612268,256.527834724049,20.1213203435596)) ;
#95917=CARTESIAN_POINT('Ctrl Pts',(30.1540561636965,256.529343370907,20.1213203435596)) ;
#95918=CARTESIAN_POINT('Ctrl Pts',(30.1573093625281,256.530838892824,20.1213203435596)) ;
#95919=CARTESIAN_POINT('Ctrl Pts',(30.1694617945698,256.536425464502,20.1213203435596)) ;
#95920=CARTESIAN_POINT('Ctrl Pts',(30.1817428975319,256.541804089539,20.1213203435596)) ;
#95921=CARTESIAN_POINT('Ctrl Pts',(30.1940635106411,256.547052875707,20.1213203435596)) ;
#95922=CARTESIAN_POINT('Ctrl Pts',(30.1951835168917,256.547530017004,20.1213203435596)) ;
#95923=CARTESIAN_POINT('Ctrl Pts',(30.1963038727072,256.548006058759,20.1213203435596)) ;
#95924=CARTESIAN_POINT('Ctrl Pts',(30.1974245258637,256.548481045224,20.1213203435596)) ;
#95925=CARTESIAN_POINT('Ctrl Pts',(30.208594161561,256.553215271635,20.1213203435596)) ;
#95926=CARTESIAN_POINT('Ctrl Pts',(30.2197078755529,256.557649623137,20.1213203435596)) ;
#95927=CARTESIAN_POINT('Ctrl Pts',(30.2307049675344,256.561831588478,20.1213203435596)) ;
#95928=CARTESIAN_POINT('Ctrl Pts',(30.2422487637936,256.566221454084,20.1213203435596)) ;
#95929=CARTESIAN_POINT('Ctrl Pts',(30.2536644123742,256.570333309343,20.1213203435596)) ;
#95930=CARTESIAN_POINT('Ctrl Pts',(30.2649410294572,256.574220554478,20.1213203435596)) ;
#95931=CARTESIAN_POINT('Ctrl Pts',(30.2767770287943,256.578300628361,20.1213203435596)) ;
#95932=CARTESIAN_POINT('Ctrl Pts',(30.2884602178804,256.582133338675,20.1213203435596)) ;
#95933=CARTESIAN_POINT('Ctrl Pts',(30.3000360626451,256.585777382226,20.1213203435596)) ;
#95934=CARTESIAN_POINT('Ctrl Pts',(30.3121484715133,256.589590334656,20.1213203435596)) ;
#95935=CARTESIAN_POINT('Ctrl Pts',(30.3241436827804,256.593196802209,20.1213203435596)) ;
#95936=CARTESIAN_POINT('Ctrl Pts',(30.3361302501676,256.596659505367,20.1213203435596)) ;
#95937=CARTESIAN_POINT('Ctrl Pts',(30.3476017541364,256.599973415991,20.1213203435596)) ;
#95938=CARTESIAN_POINT('Ctrl Pts',(30.3590660993346,256.603155652241,20.1213203435596)) ;
#95939=CARTESIAN_POINT('Ctrl Pts',(30.3706597165934,256.606256700273,20.1213203435596)) ;
#95940=CARTESIAN_POINT('Ctrl Pts',(30.3745723985987,256.607303260165,20.1213203435596)) ;
#95941=CARTESIAN_POINT('Ctrl Pts',(30.3785001170307,256.608340533834,20.1213203435596)) ;
#95942=CARTESIAN_POINT('Ctrl Pts',(30.38244904473,256.609370338222,20.1213203435596)) ;
#95943=CARTESIAN_POINT('Ctrl Pts',(30.3852902557076,256.610111271395,20.1213203435596)) ;
#95944=CARTESIAN_POINT('Ctrl Pts',(30.388142904833,256.610848427449,20.1213203435596)) ;
#95945=CARTESIAN_POINT('Ctrl Pts',(30.3909923573432,256.611578161377,20.1213203435596)) ;
#95946=CARTESIAN_POINT('Ctrl Pts',(30.4116121950221,256.616858823221,20.1213203435596)) ;
#95947=CARTESIAN_POINT('Ctrl Pts',(30.4322462282601,256.621799850728,20.1213203435596)) ;
#95948=CARTESIAN_POINT('Ctrl Pts',(30.4528279178749,256.626445919744,20.1213203435596)) ;
#95949=CARTESIAN_POINT('Ctrl Pts',(30.4740982133567,256.631247433257,20.1213203435596)) ;
#95950=CARTESIAN_POINT('Ctrl Pts',(30.4953129743173,256.6357340405,20.1213203435596)) ;
#95951=CARTESIAN_POINT('Ctrl Pts',(30.5164561522723,256.639951891567,20.1213203435596)) ;
#95952=CARTESIAN_POINT('Ctrl Pts',(30.5330282715866,256.64325786247,20.1213203435596)) ;
#95953=CARTESIAN_POINT('Ctrl Pts',(30.5495576412942,256.646398667391,20.1213203435596)) ;
#95954=CARTESIAN_POINT('Ctrl Pts',(30.5660577288476,256.649394609518,20.1213203435596)) ;
#95955=CARTESIAN_POINT('Ctrl Pts',(30.5743106576067,256.650893104412,20.1213203435596)) ;
#95956=CARTESIAN_POINT('Ctrl Pts',(30.5825565323396,256.652355329413,20.1213203435596)) ;
#95957=CARTESIAN_POINT('Ctrl Pts',(30.5907985781165,256.653783641014,20.1213203435596)) ;
#95958=CARTESIAN_POINT('Ctrl Pts',(30.5966484079928,256.654797391738,20.1213203435596)) ;
#95959=CARTESIAN_POINT('Ctrl Pts',(30.6024963300507,256.655794055932,20.1213203435596)) ;
#95960=CARTESIAN_POINT('Ctrl Pts',(30.6083437875869,256.656774435841,20.1213203435596)) ;
#95961=CARTESIAN_POINT('Ctrl Pts',(30.6107292733287,256.657174384413,20.1213203435596)) ;
#95962=CARTESIAN_POINT('Ctrl Pts',(30.6131151734722,256.657571703298,20.1213203435596)) ;
#95963=CARTESIAN_POINT('Ctrl Pts',(30.6155000490728,256.657966189434,20.1213203435596)) ;
#95964=CARTESIAN_POINT('Origin',(30.6155000490728,256.657966189434,20.0213203435596)) ;
#95965=CARTESIAN_POINT('',(30.5502224098271,257.05260375666,20.1213203435596)) ;
#95966=CARTESIAN_POINT('',(30.5502224056744,257.052603781754,20.0213203435596)) ;
#95967=CARTESIAN_POINT('',(32.2263894714028,246.919294723581,20.1213203435596)) ;
#95968=CARTESIAN_POINT('Ctrl Pts',(30.5502224056744,257.052603781754,20.0213203435596)) ;
#95969=CARTESIAN_POINT('Ctrl Pts',(30.5502224056744,257.052603781754,20.3813203435596)) ;
#95970=CARTESIAN_POINT('Ctrl Pts',(30.2175036768426,256.997568237865,20.0213203435596)) ;
#95971=CARTESIAN_POINT('Ctrl Pts',(30.2175036768426,256.997568237865,20.3813203435596)) ;
#95972=CARTESIAN_POINT('Ctrl Pts',(29.9660260593743,256.919766544724,20.0213203435596)) ;
#95973=CARTESIAN_POINT('Ctrl Pts',(29.9660260593743,256.919766544724,20.3813203435596)) ;
#95974=CARTESIAN_POINT('Ctrl Pts',(29.7871734949583,256.762313540024,20.0213203435596)) ;
#95975=CARTESIAN_POINT('Ctrl Pts',(29.7871734949583,256.762313540024,20.3813203435596)) ;
#95976=CARTESIAN_POINT('Ctrl Pts',(29.6146430046735,256.610426178574,20.0213203435596)) ;
#95977=CARTESIAN_POINT('Ctrl Pts',(29.6146430046735,256.610426178574,20.3813203435596)) ;
#95978=CARTESIAN_POINT('Ctrl Pts',(29.5623693529378,256.421344022006,20.0213203435596)) ;
#95979=CARTESIAN_POINT('Ctrl Pts',(29.5623693529378,256.421344022006,20.3813203435596)) ;
#95980=CARTESIAN_POINT('Ctrl Pts',(29.4657236710055,256.200700387666,20.0213203435596)) ;
#95981=CARTESIAN_POINT('Ctrl Pts',(29.4657236710055,256.200700387666,20.3813203435596)) ;
#95982=CARTESIAN_POINT('Ctrl Pts',(29.3957391712889,256.040924657844,20.0213203435596)) ;
#95983=CARTESIAN_POINT('Ctrl Pts',(29.3957391712889,256.040924657844,20.3813203435596)) ;
#95984=CARTESIAN_POINT('Ctrl Pts',(29.303002575605,255.851124410942,20.0213203435596)) ;
#95985=CARTESIAN_POINT('Ctrl Pts',(29.303002575605,255.851124410942,20.3813203435596)) ;
#95986=CARTESIAN_POINT('Ctrl Pts',(29.2133075051976,255.671997914687,20.0213203435596)) ;
#95987=CARTESIAN_POINT('Ctrl Pts',(29.2133075051976,255.671997914687,20.3813203435596)) ;
#95988=CARTESIAN_POINT('',(29.2133075051975,255.671997914687,20.1213203435596)) ;
#95989=CARTESIAN_POINT('',(29.2133075051975,255.671997914687,20.0213203435596)) ;
#95990=CARTESIAN_POINT('Ctrl Pts',(30.5502224021797,257.052603781176,20.1213203435596)) ;
#95991=CARTESIAN_POINT('Ctrl Pts',(30.5065121505456,257.045373597616,20.1213203435596)) ;
#95992=CARTESIAN_POINT('Ctrl Pts',(30.4628107310559,257.037524057822,20.1213203435596)) ;
#95993=CARTESIAN_POINT('Ctrl Pts',(30.419433748458,257.028837962877,20.1213203435596)) ;
#95994=CARTESIAN_POINT('Ctrl Pts',(30.3764380403507,257.020228216866,20.1213203435596)) ;
#95995=CARTESIAN_POINT('Ctrl Pts',(30.3337612777691,257.010796594269,20.1213203435596)) ;
#95996=CARTESIAN_POINT('Ctrl Pts',(30.2916991266286,257.000281937884,20.1213203435596)) ;
#95997=CARTESIAN_POINT('Ctrl Pts',(30.2498339205488,256.989816513638,20.1213203435596)) ;
#95998=CARTESIAN_POINT('Ctrl Pts',(30.2085777501619,256.978278169064,20.1213203435596)) ;
#95999=CARTESIAN_POINT('Ctrl Pts',(30.1682078765978,256.965359723244,20.1213203435596)) ;
#96000=CARTESIAN_POINT('Ctrl Pts',(30.132392671999,256.953898781227,20.1213203435596)) ;
#96001=CARTESIAN_POINT('Ctrl Pts',(30.0972749265278,256.941350869345,20.1213203435596)) ;
#96002=CARTESIAN_POINT('Ctrl Pts',(30.063037275111,256.927468848656,20.1213203435596)) ;
#96003=CARTESIAN_POINT('Ctrl Pts',(30.0369143514349,256.91687703082,20.1213203435596)) ;
#96004=CARTESIAN_POINT('Ctrl Pts',(30.011303572708,256.905507926888,20.1213203435596)) ;
#96005=CARTESIAN_POINT('Ctrl Pts',(29.9862815616792,256.893239962228,20.1213203435596)) ;
#96006=CARTESIAN_POINT('Ctrl Pts',(29.9808065317204,256.890555626666,20.1213203435596)) ;
#96007=CARTESIAN_POINT('Ctrl Pts',(29.9753662544494,256.887831397022,20.1213203435596)) ;
#96008=CARTESIAN_POINT('Ctrl Pts',(29.9699674807984,256.885069553557,20.1213203435596)) ;
#96009=CARTESIAN_POINT('Ctrl Pts',(29.9339427287467,256.866640419009,20.1213203435596)) ;
#96010=CARTESIAN_POINT('Ctrl Pts',(29.8996687771619,256.846493324965,20.1213203435596)) ;
#96011=CARTESIAN_POINT('Ctrl Pts',(29.8671268712235,256.824286093635,20.1213203435596)) ;
#96012=CARTESIAN_POINT('Ctrl Pts',(29.8391989590962,256.805227541676,20.1213203435596)) ;
#96013=CARTESIAN_POINT('Ctrl Pts',(29.812547151782,256.784651260035,20.1213203435596)) ;
#96014=CARTESIAN_POINT('Ctrl Pts',(29.7871734949583,256.762313540024,20.1213203435596)) ;
#96015=CARTESIAN_POINT('Ctrl Pts',(29.7798631632135,256.755877883357,20.1213203435596)) ;
#96016=CARTESIAN_POINT('Ctrl Pts',(29.7727535941871,256.749362117533,20.1213203435596)) ;
#96017=CARTESIAN_POINT('Ctrl Pts',(29.7658341604035,256.742765184829,20.1213203435596)) ;
#96018=CARTESIAN_POINT('Ctrl Pts',(29.7629186498988,256.739985560484,20.1213203435596)) ;
#96019=CARTESIAN_POINT('Ctrl Pts',(29.760038549478,256.737193161988,20.1213203435596)) ;
#96020=CARTESIAN_POINT('Ctrl Pts',(29.7571877188389,256.734382633857,20.1213203435596)) ;
#96021=CARTESIAN_POINT('Ctrl Pts',(29.7414155814302,256.718833468903,20.1213203435596)) ;
#96022=CARTESIAN_POINT('Ctrl Pts',(29.7264026361634,256.70258812366,20.1213203435596)) ;
#96023=CARTESIAN_POINT('Ctrl Pts',(29.7121305617268,256.685637834918,20.1213203435596)) ;
#96024=CARTESIAN_POINT('Ctrl Pts',(29.6976717683343,256.668465788628,20.1213203435596)) ;
#96025=CARTESIAN_POINT('Ctrl Pts',(29.6839733667144,256.650570190372,20.1213203435596)) ;
#96026=CARTESIAN_POINT('Ctrl Pts',(29.6709626703656,256.631947663274,20.1213203435596)) ;
#96027=CARTESIAN_POINT('Ctrl Pts',(29.6577459536387,256.613030254183,20.1213203435596)) ;
#96028=CARTESIAN_POINT('Ctrl Pts',(29.6452388100344,256.593362670542,20.1213203435596)) ;
#96029=CARTESIAN_POINT('Ctrl Pts',(29.6333105692318,256.572947902923,20.1213203435596)) ;
#96030=CARTESIAN_POINT('Ctrl Pts',(29.6250306407882,256.558777094514,20.1213203435596)) ;
#96031=CARTESIAN_POINT('Ctrl Pts',(29.6170284895913,256.544246402727,20.1213203435596)) ;
#96032=CARTESIAN_POINT('Ctrl Pts',(29.6092459213769,256.529358778693,20.1213203435596)) ;
#96033=CARTESIAN_POINT('Ctrl Pts',(29.6022331469033,256.515943727656,20.1213203435596)) ;
#96034=CARTESIAN_POINT('Ctrl Pts',(29.595395074189,256.502230920785,20.1213203435596)) ;
#96035=CARTESIAN_POINT('Ctrl Pts',(29.5887073572941,256.488280078175,20.1213203435596)) ;
#96036=CARTESIAN_POINT('Ctrl Pts',(29.5770550838555,256.46397297377,20.1213203435596)) ;
#96037=CARTESIAN_POINT('Ctrl Pts',(29.5658526158538,256.438926685936,20.1213203435596)) ;
#96038=CARTESIAN_POINT('Ctrl Pts',(29.5548544878541,256.413358282385,20.1213203435596)) ;
#96039=CARTESIAN_POINT('Ctrl Pts',(29.5436688986819,256.387354069856,20.1213203435596)) ;
#96040=CARTESIAN_POINT('Ctrl Pts',(29.5326904502648,256.360809843577,20.1213203435596)) ;
#96041=CARTESIAN_POINT('Ctrl Pts',(29.5216537891901,256.333994033072,20.1213203435596)) ;
#96042=CARTESIAN_POINT('Ctrl Pts',(29.5119415174706,256.310396095593,20.1213203435596)) ;
#96043=CARTESIAN_POINT('Ctrl Pts',(29.502182328794,256.28658856044,20.1213203435596)) ;
#96044=CARTESIAN_POINT('Ctrl Pts',(29.4922299276695,256.262778202882,20.1213203435596)) ;
#96045=CARTESIAN_POINT('Ctrl Pts',(29.4888317484153,256.254648319241,20.1213203435596)) ;
#96046=CARTESIAN_POINT('Ctrl Pts',(29.4854114762981,256.246518287048,20.1213203435596)) ;
#96047=CARTESIAN_POINT('Ctrl Pts',(29.4819648387099,256.238396879059,20.1213203435596)) ;
#96048=CARTESIAN_POINT('Ctrl Pts',(29.4793643985126,256.232269389512,20.1213203435596)) ;
#96049=CARTESIAN_POINT('Ctrl Pts',(29.4767502042541,256.226149754618,20.1213203435596)) ;
#96050=CARTESIAN_POINT('Ctrl Pts',(29.4741225626305,256.220045764497,20.1213203435596)) ;
#96051=CARTESIAN_POINT('Ctrl Pts',(29.4713402639055,256.213582507187,20.1213203435596)) ;
#96052=CARTESIAN_POINT('Ctrl Pts',(29.4685417765459,256.207134167592,20.1213203435596)) ;
#96053=CARTESIAN_POINT('Ctrl Pts',(29.4657236710055,256.200700387666,20.1213203435596)) ;
#96054=CARTESIAN_POINT('Ctrl Pts',(29.4555593833296,256.177495156678,20.1213203435596)) ;
#96055=CARTESIAN_POINT('Ctrl Pts',(29.4451538317021,256.154199155577,20.1213203435596)) ;
#96056=CARTESIAN_POINT('Ctrl Pts',(29.4346031772323,256.130925997744,20.1213203435596)) ;
#96057=CARTESIAN_POINT('Ctrl Pts',(29.4257673000282,256.111435380803,20.1213203435596)) ;
#96058=CARTESIAN_POINT('Ctrl Pts',(29.4168288645707,256.091959615128,20.1213203435596)) ;
#96059=CARTESIAN_POINT('Ctrl Pts',(29.4078284012213,256.072542223159,20.1213203435596)) ;
#96060=CARTESIAN_POINT('Ctrl Pts',(29.3998947826689,256.05542641754,20.1213203435596)) ;
#96061=CARTESIAN_POINT('Ctrl Pts',(29.3919126877309,256.038355551961,20.1213203435596)) ;
#96062=CARTESIAN_POINT('Ctrl Pts',(29.3839024014031,256.021348711648,20.1213203435596)) ;
#96063=CARTESIAN_POINT('Ctrl Pts',(29.3795273962477,256.012060028197,20.1213203435596)) ;
#96064=CARTESIAN_POINT('Ctrl Pts',(29.3751396619238,256.002781349386,20.1213203435596)) ;
#96065=CARTESIAN_POINT('Ctrl Pts',(29.3707407195716,255.993512741724,20.1213203435596)) ;
#96066=CARTESIAN_POINT('Ctrl Pts',(29.3568245289963,255.964191213894,20.1213203435596)) ;
#96067=CARTESIAN_POINT('Ctrl Pts',(29.3428004323725,255.934977549532,20.1213203435596)) ;
#96068=CARTESIAN_POINT('Ctrl Pts',(29.3287093952518,255.905877638673,20.1213203435596)) ;
#96069=CARTESIAN_POINT('Ctrl Pts',(29.3106871743266,255.86865929783,20.1213203435596)) ;
#96070=CARTESIAN_POINT('Ctrl Pts',(29.2925549661882,255.831625614527,20.1213203435596)) ;
#96071=CARTESIAN_POINT('Ctrl Pts',(29.2743437474354,255.794722208492,20.1213203435596)) ;
#96072=CARTESIAN_POINT('Ctrl Pts',(29.2540926156927,255.753685101227,20.1213203435596)) ;
#96073=CARTESIAN_POINT('Ctrl Pts',(29.2337394567466,255.712801761275,20.1213203435596)) ;
#96074=CARTESIAN_POINT('Ctrl Pts',(29.2133075051976,255.671997914687,20.1213203435596)) ;
#96075=CARTESIAN_POINT('Origin',(29.6648327135485,255.562453330574,20.3213203435596)) ;
#96076=CARTESIAN_POINT('Origin',(65.0184058153773,255.92214694455,20.2213203435596)) ;
#96077=CARTESIAN_POINT('',(65.0184058153773,255.92214694455,20.3213203435596)) ;
#96078=CARTESIAN_POINT('',(65.0184058153773,255.49075064338,20.3213203435596)) ;
#96079=CARTESIAN_POINT('',(65.0184058153773,255.92214694455,20.3213203435596)) ;
#96080=CARTESIAN_POINT('',(64.9184058153773,255.34214694455,20.2213203435596)) ;
#96081=CARTESIAN_POINT('Origin',(65.0184058153773,255.49075064338,20.2213203435596)) ;
#96082=CARTESIAN_POINT('',(64.9184058153773,255.82214694455,20.2213203435596)) ;
#96083=CARTESIAN_POINT('',(64.9184058153773,255.92214694455,20.2213203435596)) ;
#96084=CARTESIAN_POINT('Origin',(65.0184058153773,255.92214694455,20.2213203435596)) ;
#96085=CARTESIAN_POINT('Origin',(65.0133528506462,255.488696344833,20.2213203435596)) ;
#96086=CARTESIAN_POINT('',(66.3254830033414,256.02214694455,20.3213203435596)) ;
#96087=CARTESIAN_POINT('',(65.0133528506462,255.488696344833,20.3213203435596)) ;
#96088=CARTESIAN_POINT('',(66.5910039984262,256.02214694455,20.2213203435596)) ;
#96089=CARTESIAN_POINT('Origin',(66.3254830033414,256.02214694455,20.2213203435596)) ;
#96090=CARTESIAN_POINT('',(65.0510146558711,255.396059481613,20.2213203435596)) ;
#96091=CARTESIAN_POINT('Origin',(65.8496519421707,256.215597544267,20.2213203435596)) ;
#96092=CARTESIAN_POINT('',(65.0184058153773,256.55354324572,20.3213203435596)) ;
#96093=CARTESIAN_POINT('',(65.8496519421707,256.215597544267,20.3213203435596)) ;
#96094=CARTESIAN_POINT('',(64.9184058153773,256.70214694455,20.2213203435596)) ;
#96095=CARTESIAN_POINT('Origin',(65.0184058153773,256.55354324572,20.2213203435596)) ;
#96096=CARTESIAN_POINT('',(65.8873137473955,256.308234407487,20.2213203435596)) ;
#96097=CARTESIAN_POINT('Origin',(65.0184058153773,256.36214694455,20.2213203435596)) ;
#96098=CARTESIAN_POINT('',(64.9184058153773,256.22214694455,20.2213203435596)) ;
#96099=CARTESIAN_POINT('',(64.9184058153773,256.36214694455,20.2213203435596)) ;
#96100=CARTESIAN_POINT('',(65.0184058153773,256.12214694455,20.3213203435596)) ;
#96101=CARTESIAN_POINT('',(65.0184058153773,256.36214694455,20.3213203435596)) ;
#96102=CARTESIAN_POINT('Origin',(65.0184058153773,256.12214694455,20.2213203435596)) ;
#96103=CARTESIAN_POINT('Origin',(64.9347049069018,256.12214694455,20.2213203435596)) ;
#96104=CARTESIAN_POINT('',(63.3110039984262,256.22214694455,20.2213203435596)) ;
#96105=CARTESIAN_POINT('',(64.9347049069018,256.22214694455,20.2213203435596)) ;
#96106=CARTESIAN_POINT('',(63.4110039984262,256.12214694455,20.3213203435596)) ;
#96107=CARTESIAN_POINT('',(64.9347049069018,256.12214694455,20.3213203435596)) ;
#96108=CARTESIAN_POINT('Origin',(63.4110039984262,256.12214694455,20.2213203435596)) ;
#96109=CARTESIAN_POINT('Origin',(63.4110039984262,256.12214694455,20.2213203435596)) ;
#96110=CARTESIAN_POINT('',(63.3110039984262,255.82214694455,20.2213203435596)) ;
#96111=CARTESIAN_POINT('',(63.3110039984262,256.12214694455,20.2213203435596)) ;
#96112=CARTESIAN_POINT('',(63.4110039984262,255.92214694455,20.3213203435596)) ;
#96113=CARTESIAN_POINT('',(63.4110039984262,256.12214694455,20.3213203435596)) ;
#96114=CARTESIAN_POINT('Origin',(63.4110039984262,255.92214694455,20.2213203435596)) ;
#96115=CARTESIAN_POINT('Origin',(64.1310039984262,255.92214694455,20.2213203435596)) ;
#96116=CARTESIAN_POINT('',(64.1310039984262,255.82214694455,20.2213203435596)) ;
#96117=CARTESIAN_POINT('',(64.1310039984262,255.92214694455,20.3213203435596)) ;
#96118=CARTESIAN_POINT('Origin',(64.9184058153773,256.22214694455,20.0213203435596)) ;
#96119=CARTESIAN_POINT('',(63.3110039984262,256.22214694455,20.1213203435596)) ;
#96120=CARTESIAN_POINT('',(63.3110039984262,256.22214694455,20.0213203435596)) ;
#96121=CARTESIAN_POINT('',(64.9184058153773,256.22214694455,20.1213203435596)) ;
#96122=CARTESIAN_POINT('',(60.0662936149535,256.22214694455,20.1213203435596)) ;
#96123=CARTESIAN_POINT('',(64.9184058153773,256.22214694455,20.0213203435596)) ;
#96124=CARTESIAN_POINT('Origin',(63.3110039984262,256.22214694455,20.0213203435596)) ;
#96125=CARTESIAN_POINT('',(63.3110039984262,255.82214694455,20.1213203435596)) ;
#96126=CARTESIAN_POINT('',(63.3110039984262,255.82214694455,20.0213203435596)) ;
#96127=CARTESIAN_POINT('',(63.3110039984262,248.469379137783,20.1213203435596)) ;
#96128=CARTESIAN_POINT('Origin',(63.3110039984262,255.82214694455,20.0213203435596)) ;
#96129=CARTESIAN_POINT('',(64.9184058153773,255.82214694455,20.1213203435596)) ;
#96130=CARTESIAN_POINT('',(64.9184058153773,255.82214694455,20.0213203435596)) ;
#96131=CARTESIAN_POINT('',(59.2625927064781,255.82214694455,20.1213203435596)) ;
#96132=CARTESIAN_POINT('Origin',(64.9184058153773,255.82214694455,20.0213203435596)) ;
#96133=CARTESIAN_POINT('',(64.9184058153773,255.34214694455,20.1213203435596)) ;
#96134=CARTESIAN_POINT('',(64.9184058153773,255.34214694455,20.0213203435596)) ;
#96135=CARTESIAN_POINT('',(64.9184058153773,248.269379137783,20.1213203435596)) ;
#96136=CARTESIAN_POINT('Origin',(64.9510039984262,256.02214694455,20.3213203435596)) ;
#96137=CARTESIAN_POINT('Origin',(62.6000000000001,255.12214694455,20.2213203435596)) ;
#96138=CARTESIAN_POINT('',(62.6,255.12214694455,20.3213203435596)) ;
#96139=CARTESIAN_POINT('',(62.8,255.12214694455,20.3213203435596)) ;
#96140=CARTESIAN_POINT('',(62.6000000000001,255.12214694455,20.3213203435596)) ;
#96141=CARTESIAN_POINT('',(62.9,255.02214694455,20.2213203435596)) ;
#96142=CARTESIAN_POINT('Origin',(62.8,255.12214694455,20.2213203435596)) ;
#96143=CARTESIAN_POINT('',(62.5,255.02214694455,20.2213203435596)) ;
#96144=CARTESIAN_POINT('',(62.6000000000001,255.02214694455,20.2213203435596)) ;
#96145=CARTESIAN_POINT('Origin',(62.6,255.12214694455,20.2213203435596)) ;
#96146=CARTESIAN_POINT('Origin',(62.8,255.52214694455,20.2213203435596)) ;
#96147=CARTESIAN_POINT('',(62.9,257.02214694455,20.2213203435596)) ;
#96148=CARTESIAN_POINT('',(62.9,255.52214694455,20.2213203435596)) ;
#96149=CARTESIAN_POINT('',(62.8,256.92214694455,20.3213203435596)) ;
#96150=CARTESIAN_POINT('',(62.8,255.52214694455,20.3213203435596)) ;
#96151=CARTESIAN_POINT('Origin',(62.8,256.92214694455,20.2213203435596)) ;
#96152=CARTESIAN_POINT('Origin',(62.8,256.92214694455,20.2213203435596)) ;
#96153=CARTESIAN_POINT('',(62.5,257.02214694455,20.2213203435596)) ;
#96154=CARTESIAN_POINT('',(62.8,257.02214694455,20.2213203435596)) ;
#96155=CARTESIAN_POINT('',(62.6,256.92214694455,20.3213203435596)) ;
#96156=CARTESIAN_POINT('',(62.8,256.92214694455,20.3213203435596)) ;
#96157=CARTESIAN_POINT('Origin',(62.6,256.92214694455,20.2213203435596)) ;
#96158=CARTESIAN_POINT('Origin',(62.6,256.52214694455,20.2213203435596)) ;
#96159=CARTESIAN_POINT('',(62.5,256.52214694455,20.2213203435596)) ;
#96160=CARTESIAN_POINT('',(62.6,256.52214694455,20.3213203435596)) ;
#96161=CARTESIAN_POINT('Origin',(62.5,257.02214694455,20.0213203435596)) ;
#96162=CARTESIAN_POINT('',(62.5,255.02214694455,20.1213203435596)) ;
#96163=CARTESIAN_POINT('',(62.5,255.02214694455,20.0213203435596)) ;
#96164=CARTESIAN_POINT('',(62.5,257.02214694455,20.1213203435596)) ;
#96165=CARTESIAN_POINT('',(62.5,248.869379137783,20.1213203435596)) ;
#96166=CARTESIAN_POINT('',(62.5,257.02214694455,20.0213203435596)) ;
#96167=CARTESIAN_POINT('Origin',(62.5,255.02214694455,20.0213203435596)) ;
#96168=CARTESIAN_POINT('',(62.9,255.02214694455,20.1213203435596)) ;
#96169=CARTESIAN_POINT('',(62.9,255.02214694455,20.0213203435596)) ;
#96170=CARTESIAN_POINT('',(58.8570907072643,255.02214694455,20.1213203435596)) ;
#96171=CARTESIAN_POINT('Origin',(62.7,256.02214694455,20.3213203435596)) ;
#96172=CARTESIAN_POINT('Origin',(60.3815941846227,255.68214694455,20.2213203435596)) ;
#96173=CARTESIAN_POINT('',(60.3815941846227,255.49075064338,20.3213203435596)) ;
#96174=CARTESIAN_POINT('',(60.3815941846227,255.92214694455,20.3213203435596)) ;
#96175=CARTESIAN_POINT('',(60.3815941846227,255.68214694455,20.3213203435596)) ;
#96176=CARTESIAN_POINT('',(60.4815941846227,255.82214694455,20.2213203435596)) ;
#96177=CARTESIAN_POINT('Origin',(60.3815941846227,255.92214694455,20.2213203435596)) ;
#96178=CARTESIAN_POINT('',(60.4815941846227,255.34214694455,20.2213203435596)) ;
#96179=CARTESIAN_POINT('',(60.4815941846227,255.68214694455,20.2213203435596)) ;
#96180=CARTESIAN_POINT('Origin',(60.3815941846227,255.49075064338,20.2213203435596)) ;
#96181=CARTESIAN_POINT('Origin',(60.4652950930983,255.92214694455,20.2213203435596)) ;
#96182=CARTESIAN_POINT('',(61.9889960015738,255.92214694455,20.3213203435596)) ;
#96183=CARTESIAN_POINT('',(60.4652950930983,255.92214694455,20.3213203435596)) ;
#96184=CARTESIAN_POINT('',(62.0889960015738,255.82214694455,20.2213203435596)) ;
#96185=CARTESIAN_POINT('Origin',(61.9889960015738,255.92214694455,20.2213203435596)) ;
#96186=CARTESIAN_POINT('',(60.4652950930983,255.82214694455,20.2213203435596)) ;
#96187=CARTESIAN_POINT('Origin',(61.9889960015738,255.92214694455,20.2213203435596)) ;
#96188=CARTESIAN_POINT('',(61.9889960015738,256.12214694455,20.3213203435596)) ;
#96189=CARTESIAN_POINT('',(61.9889960015738,255.92214694455,20.3213203435596)) ;
#96190=CARTESIAN_POINT('',(62.0889960015738,256.22214694455,20.2213203435596)) ;
#96191=CARTESIAN_POINT('Origin',(61.9889960015738,256.12214694455,20.2213203435596)) ;
#96192=CARTESIAN_POINT('',(62.0889960015738,255.92214694455,20.2213203435596)) ;
#96193=CARTESIAN_POINT('Origin',(61.2689960015738,256.12214694455,20.2213203435596)) ;
#96194=CARTESIAN_POINT('',(60.4815941846227,256.22214694455,20.2213203435596)) ;
#96195=CARTESIAN_POINT('',(61.2689960015738,256.22214694455,20.2213203435596)) ;
#96196=CARTESIAN_POINT('',(60.3815941846227,256.12214694455,20.3213203435596)) ;
#96197=CARTESIAN_POINT('',(61.2689960015738,256.12214694455,20.3213203435596)) ;
#96198=CARTESIAN_POINT('Origin',(60.3815941846227,256.12214694455,20.2213203435596)) ;
#96199=CARTESIAN_POINT('Origin',(60.3815941846227,256.12214694455,20.2213203435596)) ;
#96200=CARTESIAN_POINT('',(60.4815941846227,256.70214694455,20.2213203435596)) ;
#96201=CARTESIAN_POINT('',(60.4815941846227,256.12214694455,20.2213203435596)) ;
#96202=CARTESIAN_POINT('',(60.3815941846227,256.55354324572,20.3213203435596)) ;
#96203=CARTESIAN_POINT('',(60.3815941846227,256.12214694455,20.3213203435596)) ;
#96204=CARTESIAN_POINT('Origin',(60.3815941846227,256.55354324572,20.2213203435596)) ;
#96205=CARTESIAN_POINT('Origin',(60.3866471493538,256.555597544267,20.2213203435596)) ;
#96206=CARTESIAN_POINT('',(58.8089960015738,256.02214694455,20.2213203435596)) ;
#96207=CARTESIAN_POINT('',(60.348985344129,256.648234407487,20.2213203435596)) ;
#96208=CARTESIAN_POINT('',(59.0745169966587,256.02214694455,20.3213203435596)) ;
#96209=CARTESIAN_POINT('',(60.3866471493538,256.555597544267,20.3213203435596)) ;
#96210=CARTESIAN_POINT('Origin',(59.0745169966587,256.02214694455,20.2213203435596)) ;
#96211=CARTESIAN_POINT('Origin',(59.5503480578294,255.828696344833,20.2213203435596)) ;
#96212=CARTESIAN_POINT('',(59.5126862526045,255.736059481613,20.2213203435596)) ;
#96213=CARTESIAN_POINT('',(59.5503480578294,255.828696344833,20.3213203435596)) ;
#96214=CARTESIAN_POINT('Origin',(60.4815941846227,256.22214694455,20.0213203435596)) ;
#96215=CARTESIAN_POINT('',(60.4815941846227,256.70214694455,20.1213203435596)) ;
#96216=CARTESIAN_POINT('',(60.4815941846227,256.70214694455,20.0213203435596)) ;
#96217=CARTESIAN_POINT('',(60.4815941846227,256.22214694455,20.1213203435596)) ;
#96218=CARTESIAN_POINT('',(60.4815941846227,248.469379137783,20.1213203435596)) ;
#96219=CARTESIAN_POINT('',(60.4815941846227,256.22214694455,20.0213203435596)) ;
#96220=CARTESIAN_POINT('Origin',(60.4815941846227,256.70214694455,20.0213203435596)) ;
#96221=CARTESIAN_POINT('',(58.8089960015738,256.02214694455,20.1213203435596)) ;
#96222=CARTESIAN_POINT('',(58.8089960015738,256.02214694455,20.0213203435596)) ;
#96223=CARTESIAN_POINT('',(55.4328817810691,254.649577194559,20.1213203435596)) ;
#96224=CARTESIAN_POINT('Origin',(58.8089960015738,256.02214694455,20.0213203435596)) ;
#96225=CARTESIAN_POINT('',(60.4815941846227,255.34214694455,20.1213203435596)) ;
#96226=CARTESIAN_POINT('',(60.4815941846227,255.34214694455,20.0213203435596)) ;
#96227=CARTESIAN_POINT('',(59.9364873877912,255.563761810333,20.1213203435596)) ;
#96228=CARTESIAN_POINT('Origin',(60.4815941846227,255.34214694455,20.0213203435596)) ;
#96229=CARTESIAN_POINT('',(60.4815941846227,255.82214694455,20.1213203435596)) ;
#96230=CARTESIAN_POINT('',(60.4815941846227,255.82214694455,20.0213203435596)) ;
#96231=CARTESIAN_POINT('',(60.4815941846227,248.029379137783,20.1213203435596)) ;
#96232=CARTESIAN_POINT('Origin',(60.4489960015738,256.02214694455,20.3213203435596)) ;
#96233=CARTESIAN_POINT('Origin',(74.4283628290596,248.80334685842,18.2213203435596)) ;
#96234=CARTESIAN_POINT('',(74.4283628290596,249.32834685842,18.3213203435596)) ;
#96235=CARTESIAN_POINT('',(74.4283628290596,247.02834685842,18.3213203435596)) ;
#96236=CARTESIAN_POINT('',(74.4283628290596,248.80334685842,18.3213203435596)) ;
#96237=CARTESIAN_POINT('',(74.3283628290596,246.92834685842,18.2213203435596)) ;
#96238=CARTESIAN_POINT('Origin',(74.4283628290596,247.02834685842,18.2213203435596)) ;
#96239=CARTESIAN_POINT('',(74.3283628290596,249.42834685842,18.2213203435596)) ;
#96240=CARTESIAN_POINT('',(74.3283628290596,248.80334685842,18.2213203435596)) ;
#96241=CARTESIAN_POINT('Origin',(74.4283628290596,249.32834685842,18.2213203435596)) ;
#96242=CARTESIAN_POINT('Origin',(74.4283628290596,247.02834685842,18.2213203435596)) ;
#96243=CARTESIAN_POINT('',(74.7283628290596,246.92834685842,18.2213203435596)) ;
#96244=CARTESIAN_POINT('',(74.4283628290596,246.92834685842,18.2213203435596)) ;
#96245=CARTESIAN_POINT('',(74.6283628290596,247.02834685842,18.3213203435596)) ;
#96246=CARTESIAN_POINT('',(74.4283628290596,247.02834685842,18.3213203435596)) ;
#96247=CARTESIAN_POINT('Origin',(74.6283628290596,247.02834685842,18.2213203435596)) ;
#96248=CARTESIAN_POINT('Origin',(74.6283628290596,247.55334685842,18.2213203435596)) ;
#96249=CARTESIAN_POINT('',(74.7283628290596,249.42834685842,18.2213203435596)) ;
#96250=CARTESIAN_POINT('',(74.7283628290596,247.55334685842,18.2213203435596)) ;
#96251=CARTESIAN_POINT('',(74.6283628290596,249.32834685842,18.3213203435596)) ;
#96252=CARTESIAN_POINT('',(74.6283628290596,247.55334685842,18.3213203435596)) ;
#96253=CARTESIAN_POINT('Origin',(74.6283628290596,249.32834685842,18.2213203435596)) ;
#96254=CARTESIAN_POINT('Origin',(74.6283628290596,249.32834685842,18.2213203435596)) ;
#96255=CARTESIAN_POINT('',(74.6283628290596,249.42834685842,18.2213203435596)) ;
#96256=CARTESIAN_POINT('',(74.6283628290596,249.32834685842,18.3213203435596)) ;
#96257=CARTESIAN_POINT('Origin',(74.7283628290596,249.42834685842,18.0213203435596)) ;
#96258=CARTESIAN_POINT('',(74.3283628290596,249.42834685842,18.1213203435596)) ;
#96259=CARTESIAN_POINT('',(74.3283628290596,249.42834685842,18.0213203435596)) ;
#96260=CARTESIAN_POINT('',(74.7283628290596,249.42834685842,18.1213203435596)) ;
#96261=CARTESIAN_POINT('',(64.9712721217948,249.42834685842,18.1213203435596)) ;
#96262=CARTESIAN_POINT('',(74.7283628290596,249.42834685842,18.0213203435596)) ;
#96263=CARTESIAN_POINT('Origin',(74.3283628290596,249.42834685842,18.0213203435596)) ;
#96264=CARTESIAN_POINT('',(74.3283628290596,246.92834685842,18.1213203435596)) ;
#96265=CARTESIAN_POINT('',(74.3283628290596,246.92834685842,18.0213203435596)) ;
#96266=CARTESIAN_POINT('',(74.3283628290596,249.23917342921,18.1213203435596)) ;
#96267=CARTESIAN_POINT('Origin',(74.5283628290596,248.17834685842,18.3213203435596)) ;
#96268=CARTESIAN_POINT('Origin',(76.9136449414663,247.288583115023,18.2213203435596)) ;
#96269=CARTESIAN_POINT('',(76.7495157419148,246.884873995972,18.3213203435596)) ;
#96270=CARTESIAN_POINT('',(77.2809120430846,248.191951183936,18.3213203435596)) ;
#96271=CARTESIAN_POINT('',(76.9136449414663,247.288583115023,18.3213203435596)) ;
#96272=CARTESIAN_POINT('',(77.4295157419147,248.291951183936,18.2213203435596)) ;
#96273=CARTESIAN_POINT('Origin',(77.2809120430846,248.191951183936,18.2213203435596)) ;
#96274=CARTESIAN_POINT('',(76.7495157419148,246.619353000887,18.2213203435596)) ;
#96275=CARTESIAN_POINT('',(77.0062818046861,247.250921309799,18.2213203435596)) ;
#96276=CARTESIAN_POINT('Origin',(76.7495157419148,246.884873995972,18.2213203435596)) ;
#96277=CARTESIAN_POINT('Origin',(76.8191684028636,248.191951183936,18.2213203435596)) ;
#96278=CARTESIAN_POINT('',(76.8348658990794,248.191951183936,18.3213203435596)) ;
#96279=CARTESIAN_POINT('',(76.8191684028636,248.191951183936,18.3213203435596)) ;
#96280=CARTESIAN_POINT('',(76.9348658990794,248.291951183936,18.2213203435596)) ;
#96281=CARTESIAN_POINT('Origin',(76.8348658990794,248.191951183936,18.2213203435596)) ;
#96282=CARTESIAN_POINT('',(76.8191684028636,248.291951183936,18.2213203435596)) ;
#96283=CARTESIAN_POINT('Origin',(76.8348658990794,248.301519996331,18.2213203435596)) ;
#96284=CARTESIAN_POINT('',(76.8348658990794,249.302824616567,18.3213203435596)) ;
#96285=CARTESIAN_POINT('',(76.8348658990794,248.301519996331,18.3213203435596)) ;
#96286=CARTESIAN_POINT('',(76.9348658990794,249.302824616567,18.2213203435596)) ;
#96287=CARTESIAN_POINT('Origin',(76.8348658990794,249.302824616567,18.2213203435596)) ;
#96288=CARTESIAN_POINT('',(76.9348658990794,248.301519996331,18.2213203435596)) ;
#96289=CARTESIAN_POINT('Origin',(76.2348658990794,249.302824616567,18.2213203435596)) ;
#96290=CARTESIAN_POINT('',(75.9152721256086,249.810623612193,18.3213203435596)) ;
#96291=CARTESIAN_POINT('',(75.8620064966968,249.895256778131,18.2213203435596)) ;
#96292=CARTESIAN_POINT('Origin',(75.9152721256086,249.810623612193,18.2213203435596)) ;
#96293=CARTESIAN_POINT('Origin',(76.2348658990794,249.302824616567,18.2213203435596)) ;
#96294=CARTESIAN_POINT('Origin',(76.2348658990794,249.302824616567,18.3213203435596)) ;
#96295=CARTESIAN_POINT('Origin',(75.6824052881838,249.664064064164,18.2213203435596)) ;
#96296=CARTESIAN_POINT('',(74.9881263857102,249.345262302685,18.2213203435596)) ;
#96297=CARTESIAN_POINT('',(75.629139659272,249.748697230101,18.2213203435596)) ;
#96298=CARTESIAN_POINT('',(75.1260251805597,249.313894765659,18.3213203435596)) ;
#96299=CARTESIAN_POINT('',(75.6824052881838,249.664064064164,18.3213203435596)) ;
#96300=CARTESIAN_POINT('Origin',(75.1260251805597,249.313894765659,18.2213203435596)) ;
#96301=CARTESIAN_POINT('Origin',(75.4790336726305,248.753003494924,18.2213203435596)) ;
#96302=CARTESIAN_POINT('',(75.2011889013574,249.006729638934,18.2213203435596)) ;
#96303=CARTESIAN_POINT('',(75.3944005066928,248.699737866012,18.2213203435596)) ;
#96304=CARTESIAN_POINT('',(75.2325564383833,249.144628433784,18.3213203435596)) ;
#96305=CARTESIAN_POINT('',(75.4790336726305,248.753003494924,18.3213203435596)) ;
#96306=CARTESIAN_POINT('Origin',(75.2325564383833,249.144628433784,18.2213203435596)) ;
#96307=CARTESIAN_POINT('Origin',(75.3519964905142,249.219800494565,18.2213203435596)) ;
#96308=CARTESIAN_POINT('',(76.0218033834322,249.641357280318,18.3213203435596)) ;
#96309=CARTESIAN_POINT('',(75.3519964905142,249.219800494565,18.3213203435596)) ;
#96310=CARTESIAN_POINT('',(76.075069012344,249.55672411438,18.2213203435596)) ;
#96311=CARTESIAN_POINT('Origin',(76.0218033834322,249.641357280318,18.2213203435596)) ;
#96312=CARTESIAN_POINT('',(75.405262119426,249.135167328628,18.2213203435596)) ;
#96313=CARTESIAN_POINT('Origin',(76.2348658990794,249.302824616567,18.2213203435596)) ;
#96314=CARTESIAN_POINT('',(76.6348658990794,249.302824616567,18.3213203435596)) ;
#96315=CARTESIAN_POINT('',(76.5348658990794,249.302824616567,18.2213203435596)) ;
#96316=CARTESIAN_POINT('Origin',(76.6348658990794,249.302824616567,18.2213203435596)) ;
#96317=CARTESIAN_POINT('Origin',(76.2348658990794,249.302824616567,18.2213203435596)) ;
#96318=CARTESIAN_POINT('Origin',(76.2348658990794,249.302824616567,18.3213203435596)) ;
#96319=CARTESIAN_POINT('Origin',(76.6348658990794,248.806956712647,18.2213203435596)) ;
#96320=CARTESIAN_POINT('',(76.5348658990794,248.291951183936,18.2213203435596)) ;
#96321=CARTESIAN_POINT('',(76.5348658990794,248.806956712647,18.2213203435596)) ;
#96322=CARTESIAN_POINT('',(76.6348658990794,248.191951183936,18.3213203435596)) ;
#96323=CARTESIAN_POINT('',(76.6348658990794,248.806956712647,18.3213203435596)) ;
#96324=CARTESIAN_POINT('Origin',(76.6348658990794,248.191951183936,18.2213203435596)) ;
#96325=CARTESIAN_POINT('Origin',(76.3718434814459,248.191951183936,18.2213203435596)) ;
#96326=CARTESIAN_POINT('',(76.0695157419148,248.291951183936,18.2213203435596)) ;
#96327=CARTESIAN_POINT('',(76.3718434814459,248.291951183936,18.2213203435596)) ;
#96328=CARTESIAN_POINT('',(76.218119440745,248.191951183936,18.3213203435596)) ;
#96329=CARTESIAN_POINT('',(76.3718434814459,248.191951183936,18.3213203435596)) ;
#96330=CARTESIAN_POINT('Origin',(76.218119440745,248.191951183936,18.2213203435596)) ;
#96331=CARTESIAN_POINT('Origin',(76.1686937834863,248.313523631769,18.2213203435596)) ;
#96332=CARTESIAN_POINT('',(76.0760569202665,248.275861826544,18.2213203435596)) ;
#96333=CARTESIAN_POINT('',(76.1686937834863,248.313523631769,18.3213203435596)) ;
#96334=CARTESIAN_POINT('Origin',(75.2011889013574,249.006729638934,18.0213203435596)) ;
#96335=CARTESIAN_POINT('',(76.075069012344,249.55672411438,18.1213203435596)) ;
#96336=CARTESIAN_POINT('',(76.075069012344,249.55672411438,18.0213203435596)) ;
#96337=CARTESIAN_POINT('',(75.2011889013574,249.006729638934,18.1213203435596)) ;
#96338=CARTESIAN_POINT('',(68.0528224690616,244.507757758468,18.1213203435596)) ;
#96339=CARTESIAN_POINT('',(75.2011889013574,249.006729638934,18.0213203435596)) ;
#96340=CARTESIAN_POINT('Origin',(76.2348658990794,249.302824616567,18.0213203435596)) ;
#96341=CARTESIAN_POINT('',(76.5348658990794,249.302824616567,18.1213203435596)) ;
#96342=CARTESIAN_POINT('',(76.5348658990794,249.302824616567,18.0213203435596)) ;
#96343=CARTESIAN_POINT('Origin',(76.2348658990794,249.302824616567,18.1213203435596)) ;
#96344=CARTESIAN_POINT('Origin',(76.5348658990794,249.302824616567,18.0213203435596)) ;
#96345=CARTESIAN_POINT('',(76.5348658990794,248.291951183936,18.1213203435596)) ;
#96346=CARTESIAN_POINT('',(76.5348658990794,248.291951183936,18.0213203435596)) ;
#96347=CARTESIAN_POINT('',(76.5348658990794,249.176412308284,18.1213203435596)) ;
#96348=CARTESIAN_POINT('Origin',(76.5348658990794,248.291951183936,18.0213203435596)) ;
#96349=CARTESIAN_POINT('',(76.0695157419148,248.291951183936,18.1213203435596)) ;
#96350=CARTESIAN_POINT('',(76.0695157419148,248.291951183936,18.0213203435596)) ;
#96351=CARTESIAN_POINT('',(65.8745236568046,248.291951183936,18.1213203435596)) ;
#96352=CARTESIAN_POINT('Origin',(76.0695157419148,248.291951183936,18.0213203435596)) ;
#96353=CARTESIAN_POINT('',(76.7495157419148,246.619353000887,18.1213203435596)) ;
#96354=CARTESIAN_POINT('',(76.7495157419148,246.619353000887,18.0213203435596)) ;
#96355=CARTESIAN_POINT('',(74.4582066182201,252.255293408379,18.1213203435596)) ;
#96356=CARTESIAN_POINT('Origin',(76.7495157419148,246.619353000887,18.0213203435596)) ;
#96357=CARTESIAN_POINT('',(77.4295157419147,248.291951183936,18.1213203435596)) ;
#96358=CARTESIAN_POINT('',(77.4295157419147,248.291951183936,18.0213203435596)) ;
#96359=CARTESIAN_POINT('',(75.6462281222094,243.90559290074,18.1213203435596)) ;
#96360=CARTESIAN_POINT('Origin',(76.2088210638125,248.311088808727,18.3213203435596)) ;
#96361=CARTESIAN_POINT('Origin',(72.2290896109171,248.324963207434,18.2213203435596)) ;
#96362=CARTESIAN_POINT('',(71.7673459706961,248.324963207434,18.3213203435596)) ;
#96363=CARTESIAN_POINT('',(72.2133921147013,248.324963207434,18.3213203435596)) ;
#96364=CARTESIAN_POINT('',(72.2290896109171,248.324963207434,18.3213203435596)) ;
#96365=CARTESIAN_POINT('',(72.1133921147013,248.224963207434,18.2213203435596)) ;
#96366=CARTESIAN_POINT('Origin',(72.2133921147013,248.324963207434,18.2213203435596)) ;
#96367=CARTESIAN_POINT('',(71.618742271866,248.224963207434,18.2213203435596)) ;
#96368=CARTESIAN_POINT('',(72.2290896109171,248.224963207434,18.2213203435596)) ;
#96369=CARTESIAN_POINT('Origin',(71.7673459706961,248.324963207434,18.2213203435596)) ;
#96370=CARTESIAN_POINT('Origin',(72.2133921147013,248.215394395038,18.2213203435596)) ;
#96371=CARTESIAN_POINT('',(72.2133921147013,247.214089774802,18.3213203435596)) ;
#96372=CARTESIAN_POINT('',(72.2133921147013,248.215394395038,18.3213203435596)) ;
#96373=CARTESIAN_POINT('',(72.1133921147013,247.214089774802,18.2213203435596)) ;
#96374=CARTESIAN_POINT('Origin',(72.2133921147013,247.214089774802,18.2213203435596)) ;
#96375=CARTESIAN_POINT('',(72.1133921147013,248.215394395038,18.2213203435596)) ;
#96376=CARTESIAN_POINT('Origin',(72.8133921147013,247.214089774802,18.2213203435596)) ;
#96377=CARTESIAN_POINT('',(73.1329858881721,246.706290779176,18.3213203435596)) ;
#96378=CARTESIAN_POINT('',(73.1862515170839,246.621657613239,18.2213203435596)) ;
#96379=CARTESIAN_POINT('Origin',(73.1329858881721,246.706290779176,18.2213203435596)) ;
#96380=CARTESIAN_POINT('Origin',(72.8133921147013,247.214089774802,18.2213203435596)) ;
#96381=CARTESIAN_POINT('Origin',(72.8133921147013,247.214089774802,18.3213203435596)) ;
#96382=CARTESIAN_POINT('Origin',(73.3658527255969,246.852850327206,18.2213203435596)) ;
#96383=CARTESIAN_POINT('',(74.0601316280705,247.171652088685,18.2213203435596)) ;
#96384=CARTESIAN_POINT('',(73.4191183545087,246.768217161268,18.2213203435596)) ;
#96385=CARTESIAN_POINT('',(73.922232833221,247.203019625711,18.3213203435596)) ;
#96386=CARTESIAN_POINT('',(73.3658527255969,246.852850327206,18.3213203435596)) ;
#96387=CARTESIAN_POINT('Origin',(73.922232833221,247.203019625711,18.2213203435596)) ;
#96388=CARTESIAN_POINT('Origin',(73.5692243411502,247.763910896445,18.2213203435596)) ;
#96389=CARTESIAN_POINT('',(73.8157015753974,247.372285957586,18.3213203435596)) ;
#96390=CARTESIAN_POINT('',(73.5692243411502,247.763910896445,18.3213203435596)) ;
#96391=CARTESIAN_POINT('',(73.8470691124233,247.510184752435,18.2213203435596)) ;
#96392=CARTESIAN_POINT('Origin',(73.8157015753974,247.372285957586,18.2213203435596)) ;
#96393=CARTESIAN_POINT('',(73.6538575070879,247.817176525357,18.2213203435596)) ;
#96394=CARTESIAN_POINT('Origin',(73.6962615232665,247.297113896804,18.2213203435596)) ;
#96395=CARTESIAN_POINT('',(73.0264546303485,246.875557111052,18.3213203435596)) ;
#96396=CARTESIAN_POINT('',(73.6962615232665,247.297113896804,18.3213203435596)) ;
#96397=CARTESIAN_POINT('',(72.9731890014367,246.960190276989,18.2213203435596)) ;
#96398=CARTESIAN_POINT('Origin',(73.0264546303485,246.875557111052,18.2213203435596)) ;
#96399=CARTESIAN_POINT('',(73.6429958943547,247.381747062742,18.2213203435596)) ;
#96400=CARTESIAN_POINT('Origin',(72.8133921147013,247.214089774802,18.2213203435596)) ;
#96401=CARTESIAN_POINT('',(72.4133921147013,247.214089774802,18.3213203435596)) ;
#96402=CARTESIAN_POINT('',(72.5133921147013,247.214089774802,18.2213203435596)) ;
#96403=CARTESIAN_POINT('Origin',(72.4133921147013,247.214089774802,18.2213203435596)) ;
#96404=CARTESIAN_POINT('Origin',(72.8133921147013,247.214089774802,18.2213203435596)) ;
#96405=CARTESIAN_POINT('Origin',(72.8133921147013,247.214089774802,18.3213203435596)) ;
#96406=CARTESIAN_POINT('Origin',(72.4133921147013,247.709957678722,18.2213203435596)) ;
#96407=CARTESIAN_POINT('',(72.5133921147013,248.224963207434,18.2213203435596)) ;
#96408=CARTESIAN_POINT('',(72.5133921147013,247.709957678722,18.2213203435596)) ;
#96409=CARTESIAN_POINT('',(72.4133921147013,248.324963207434,18.3213203435596)) ;
#96410=CARTESIAN_POINT('',(72.4133921147013,247.709957678722,18.3213203435596)) ;
#96411=CARTESIAN_POINT('Origin',(72.4133921147013,248.324963207434,18.2213203435596)) ;
#96412=CARTESIAN_POINT('Origin',(72.6764145323348,248.324963207434,18.2213203435596)) ;
#96413=CARTESIAN_POINT('',(72.9787422718659,248.224963207434,18.2213203435596)) ;
#96414=CARTESIAN_POINT('',(72.6764145323348,248.224963207434,18.2213203435596)) ;
#96415=CARTESIAN_POINT('',(72.8301385730357,248.324963207434,18.3213203435596)) ;
#96416=CARTESIAN_POINT('',(72.6764145323348,248.324963207434,18.3213203435596)) ;
#96417=CARTESIAN_POINT('Origin',(72.8301385730357,248.324963207434,18.2213203435596)) ;
#96418=CARTESIAN_POINT('Origin',(72.8795642302944,248.2033907596,18.2213203435596)) ;
#96419=CARTESIAN_POINT('',(72.2987422718658,249.897561390483,18.2213203435596)) ;
#96420=CARTESIAN_POINT('',(72.9722010935142,248.241052564825,18.2213203435596)) ;
#96421=CARTESIAN_POINT('',(72.2987422718659,249.632040395398,18.3213203435596)) ;
#96422=CARTESIAN_POINT('',(72.8795642302944,248.2033907596,18.3213203435596)) ;
#96423=CARTESIAN_POINT('Origin',(72.2987422718659,249.632040395398,18.2213203435596)) ;
#96424=CARTESIAN_POINT('Origin',(72.1346130723144,249.228331276346,18.2213203435596)) ;
#96425=CARTESIAN_POINT('',(72.0419762090946,249.265993081571,18.2213203435596)) ;
#96426=CARTESIAN_POINT('',(72.1346130723144,249.228331276346,18.3213203435596)) ;
#96427=CARTESIAN_POINT('Origin',(72.8133921147013,247.214089774802,18.0213203435596)) ;
#96428=CARTESIAN_POINT('',(72.5133921147013,247.214089774802,18.1213203435596)) ;
#96429=CARTESIAN_POINT('',(72.5133921147013,247.214089774802,18.0213203435596)) ;
#96430=CARTESIAN_POINT('',(72.9731890014367,246.960190276989,18.1213203435596)) ;
#96431=CARTESIAN_POINT('Origin',(72.8133921147013,247.214089774802,18.1213203435596)) ;
#96432=CARTESIAN_POINT('',(72.9731890014367,246.960190276989,18.0213203435596)) ;
#96433=CARTESIAN_POINT('Origin',(72.5133921147013,247.214089774802,18.0213203435596)) ;
#96434=CARTESIAN_POINT('',(72.5133921147013,248.224963207434,18.1213203435596)) ;
#96435=CARTESIAN_POINT('',(72.5133921147013,248.224963207434,18.0213203435596)) ;
#96436=CARTESIAN_POINT('',(72.5133921147013,248.132044887401,18.1213203435596)) ;
#96437=CARTESIAN_POINT('Origin',(72.5133921147013,248.224963207434,18.0213203435596)) ;
#96438=CARTESIAN_POINT('',(72.9787422718659,248.224963207434,18.1213203435596)) ;
#96439=CARTESIAN_POINT('',(72.9787422718659,248.224963207434,18.0213203435596)) ;
#96440=CARTESIAN_POINT('',(63.8637867646156,248.224963207434,18.1213203435596)) ;
#96441=CARTESIAN_POINT('Origin',(72.9787422718659,248.224963207434,18.0213203435596)) ;
#96442=CARTESIAN_POINT('',(72.2987422718658,249.897561390483,18.1213203435596)) ;
#96443=CARTESIAN_POINT('',(72.2987422718658,249.897561390483,18.0213203435596)) ;
#96444=CARTESIAN_POINT('',(71.5749469690114,251.677883020562,18.1213203435596)) ;
#96445=CARTESIAN_POINT('Origin',(72.2987422718659,249.897561390483,18.0213203435596)) ;
#96446=CARTESIAN_POINT('',(71.618742271866,248.224963207434,18.1213203435596)) ;
#96447=CARTESIAN_POINT('',(71.618742271866,248.224963207434,18.0213203435596)) ;
#96448=CARTESIAN_POINT('',(70.9392436911016,246.553598366889,18.1213203435596)) ;
#96449=CARTESIAN_POINT('Origin',(71.618742271866,248.224963207434,18.0213203435596)) ;
#96450=CARTESIAN_POINT('',(72.1133921147013,248.224963207434,18.1213203435596)) ;
#96451=CARTESIAN_POINT('',(72.1133921147013,248.224963207434,18.0213203435596)) ;
#96452=CARTESIAN_POINT('',(63.416461843198,248.224963207434,18.1213203435596)) ;
#96453=CARTESIAN_POINT('Origin',(72.8394369499682,248.205825582643,18.3213203435596)) ;
#96454=CARTESIAN_POINT('Ctrl Pts',(31.8391836130391,258.138878696195,20.1213203435596)) ;
#96455=CARTESIAN_POINT('Ctrl Pts',(31.8088277838837,258.075317586011,20.1213203435596)) ;
#96456=CARTESIAN_POINT('Ctrl Pts',(31.7480710314216,257.948103917433,20.1213203435577)) ;
#96457=CARTESIAN_POINT('Ctrl Pts',(31.65807074167,257.757060544542,20.1213203435576)) ;
#96458=CARTESIAN_POINT('Ctrl Pts',(31.5846672172411,257.598364328898,20.1213203435568)) ;
#96459=CARTESIAN_POINT('Ctrl Pts',(31.5398429295626,257.500340825891,20.1213203435565)) ;
#96460=CARTESIAN_POINT('Ctrl Pts',(31.5232414331806,257.464149039576,20.1213203435565)) ;
#96461=CARTESIAN_POINT('Ctrl Pts',(31.5204692836011,257.458111769045,20.1213203435565)) ;
#96462=CARTESIAN_POINT('Ctrl Pts',(31.5176945388745,257.45207046735,20.1213203435565)) ;
#96463=CARTESIAN_POINT('Ctrl Pts',(31.5121271696917,257.43997576795,20.1213203435565)) ;
#96464=CARTESIAN_POINT('Ctrl Pts',(31.5000486151333,257.413723558212,20.1213203435565)) ;
#96465=CARTESIAN_POINT('Ctrl Pts',(31.4733366583784,257.356758147137,20.1213203435566)) ;
#96466=CARTESIAN_POINT('Ctrl Pts',(31.4411791361222,257.290450232183,20.1213203435566)) ;
#96467=CARTESIAN_POINT('Ctrl Pts',(31.4018882564612,257.224550414268,20.1213203435566)) ;
#96468=CARTESIAN_POINT('Ctrl Pts',(31.3743956554151,257.188936944183,20.1213203435566)) ;
#96469=CARTESIAN_POINT('Ctrl Pts',(31.3560237927364,257.170047934177,20.1213203435566)) ;
#96470=CARTESIAN_POINT('Ctrl Pts',(31.311584729612,257.127602179568,20.1213203435567)) ;
#96471=CARTESIAN_POINT('Ctrl Pts',(31.2152044538023,257.0849023214,20.121320343557)) ;
#96472=CARTESIAN_POINT('Ctrl Pts',(31.0594322135369,257.058857932597,20.1213203435571)) ;
#96473=CARTESIAN_POINT('Ctrl Pts',(30.9440458722358,257.056950442841,20.1213203435596)) ;
#96474=CARTESIAN_POINT('Ctrl Pts',(30.8368060688104,257.061456316934,20.1213203435596)) ;
#96475=CARTESIAN_POINT('Ctrl Pts',(30.8035021201096,257.06285564251,20.1213203435596)) ;
#96476=CARTESIAN_POINT('Ctrl Pts',(30.7701981714089,257.064254968086,20.1213203435596)) ;
#96477=CARTESIAN_POINT('Ctrl Pts',(31.8391836130391,258.138878696195,20.1063603785425)) ;
#96478=CARTESIAN_POINT('Ctrl Pts',(31.8088277838837,258.075317586011,20.1063603785425)) ;
#96479=CARTESIAN_POINT('Ctrl Pts',(31.7480710314216,257.948103917433,20.1063603785406)) ;
#96480=CARTESIAN_POINT('Ctrl Pts',(31.65807074167,257.757060544542,20.1063603785405)) ;
#96481=CARTESIAN_POINT('Ctrl Pts',(31.5846672172411,257.598364328898,20.1063603785397)) ;
#96482=CARTESIAN_POINT('Ctrl Pts',(31.5398429295626,257.500340825891,20.1063603785394)) ;
#96483=CARTESIAN_POINT('Ctrl Pts',(31.5232414331806,257.464149039576,20.1063603785394)) ;
#96484=CARTESIAN_POINT('Ctrl Pts',(31.5204692836011,257.458111769045,20.1063603785394)) ;
#96485=CARTESIAN_POINT('Ctrl Pts',(31.5176945388745,257.45207046735,20.1063603785394)) ;
#96486=CARTESIAN_POINT('Ctrl Pts',(31.5121271696917,257.43997576795,20.1063603785394)) ;
#96487=CARTESIAN_POINT('Ctrl Pts',(31.5000486151333,257.413723558212,20.1063603785394)) ;
#96488=CARTESIAN_POINT('Ctrl Pts',(31.4733366583784,257.356758147137,20.1063603785395)) ;
#96489=CARTESIAN_POINT('Ctrl Pts',(31.4411791361222,257.290450232183,20.1063603785395)) ;
#96490=CARTESIAN_POINT('Ctrl Pts',(31.4018882564612,257.224550414268,20.1063603785395)) ;
#96491=CARTESIAN_POINT('Ctrl Pts',(31.3743956554151,257.188936944183,20.1063603785395)) ;
#96492=CARTESIAN_POINT('Ctrl Pts',(31.3560237927364,257.170047934177,20.1063603785395)) ;
#96493=CARTESIAN_POINT('Ctrl Pts',(31.311584729612,257.127602179568,20.1063603785396)) ;
#96494=CARTESIAN_POINT('Ctrl Pts',(31.2152044538023,257.0849023214,20.1063603785399)) ;
#96495=CARTESIAN_POINT('Ctrl Pts',(31.0594322135369,257.058857932597,20.10636037854)) ;
#96496=CARTESIAN_POINT('Ctrl Pts',(30.9440458722358,257.056950442841,20.1063603785425)) ;
#96497=CARTESIAN_POINT('Ctrl Pts',(30.8368060688104,257.061456316934,20.1063603785425)) ;
#96498=CARTESIAN_POINT('Ctrl Pts',(30.8035021201096,257.06285564251,20.1063603785425)) ;
#96499=CARTESIAN_POINT('Ctrl Pts',(30.7701981714089,257.064254968086,20.1063603785425)) ;
#96500=CARTESIAN_POINT('Ctrl Pts',(31.8330058570152,258.141829099451,20.0764990828381)) ;
#96501=CARTESIAN_POINT('Ctrl Pts',(31.8026486089796,258.07826500619,20.0764990828381)) ;
#96502=CARTESIAN_POINT('Ctrl Pts',(31.7419443110348,257.951087199869,20.0764990828362)) ;
#96503=CARTESIAN_POINT('Ctrl Pts',(31.6519283830522,257.760006830989,20.0764990828361)) ;
#96504=CARTESIAN_POINT('Ctrl Pts',(31.5785318221264,257.601292622869,20.0764990828353)) ;
#96505=CARTESIAN_POINT('Ctrl Pts',(31.5337121585615,257.503266786335,20.076499082835)) ;
#96506=CARTESIAN_POINT('Ctrl Pts',(31.5171153568792,257.467084414751,20.076499082835)) ;
#96507=CARTESIAN_POINT('Ctrl Pts',(31.5143435056701,257.461047860026,20.076499082835)) ;
#96508=CARTESIAN_POINT('Ctrl Pts',(31.5115709052337,257.455011047666,20.076499082835)) ;
#96509=CARTESIAN_POINT('Ctrl Pts',(31.5060037126059,257.442916481506,20.076499082835)) ;
#96510=CARTESIAN_POINT('Ctrl Pts',(31.4939343137359,257.416686125584,20.076499082835)) ;
#96511=CARTESIAN_POINT('Ctrl Pts',(31.4672601801766,257.359787112992,20.0764990828351)) ;
#96512=CARTESIAN_POINT('Ctrl Pts',(31.4351804253194,257.293668828372,20.0764990828351)) ;
#96513=CARTESIAN_POINT('Ctrl Pts',(31.396265321692,257.228410794591,20.0764990828351)) ;
#96514=CARTESIAN_POINT('Ctrl Pts',(31.3692366359014,257.193442400304,20.0764990828351)) ;
#96515=CARTESIAN_POINT('Ctrl Pts',(31.3513485240157,257.175019065014,20.0764990828351)) ;
#96516=CARTESIAN_POINT('Ctrl Pts',(31.3072749058674,257.133136091133,20.0764990828352)) ;
#96517=CARTESIAN_POINT('Ctrl Pts',(31.213617844106,257.091685982779,20.0764990828355)) ;
#96518=CARTESIAN_POINT('Ctrl Pts',(31.0583683718114,257.065331495388,20.0764990828356)) ;
#96519=CARTESIAN_POINT('Ctrl Pts',(30.9439706532423,257.063749482234,20.0764990828381)) ;
#96520=CARTESIAN_POINT('Ctrl Pts',(30.8370934679167,257.068296415663,20.0764990828381)) ;
#96521=CARTESIAN_POINT('Ctrl Pts',(30.8037895192159,257.069695741239,20.0764990828381)) ;
#96522=CARTESIAN_POINT('Ctrl Pts',(30.7704855705151,257.071095066814,20.0764990828381)) ;
#96523=CARTESIAN_POINT('Ctrl Pts',(31.8028168586867,258.156246910483,20.0344443101957)) ;
#96524=CARTESIAN_POINT('Ctrl Pts',(31.7724543635431,258.09267184256,20.0344443101957)) ;
#96525=CARTESIAN_POINT('Ctrl Pts',(31.7117274582361,257.965437861777,20.0344443101938)) ;
#96526=CARTESIAN_POINT('Ctrl Pts',(31.6216226089589,257.774168684096,20.0344443101937)) ;
#96527=CARTESIAN_POINT('Ctrl Pts',(31.5481401064261,257.61526448649,20.0344443101928)) ;
#96528=CARTESIAN_POINT('Ctrl Pts',(31.5032980635907,257.517187990573,20.0344443101925)) ;
#96529=CARTESIAN_POINT('Ctrl Pts',(31.4867204866751,257.481047583487,20.0344443101925)) ;
#96530=CARTESIAN_POINT('Ctrl Pts',(31.4839532755492,257.475020977491,20.0344443101925)) ;
#96531=CARTESIAN_POINT('Ctrl Pts',(31.481184083603,257.468991878312,20.0344443101925)) ;
#96532=CARTESIAN_POINT('Ctrl Pts',(31.4756312639653,257.456927791243,20.0344443101925)) ;
#96533=CARTESIAN_POINT('Ctrl Pts',(31.4635882182489,257.430757014838,20.0344443101926)) ;
#96534=CARTESIAN_POINT('Ctrl Pts',(31.4370819739745,257.374207932902,20.0344443101926)) ;
#96535=CARTESIAN_POINT('Ctrl Pts',(31.4054356385254,257.309033959787,20.0344443101926)) ;
#96536=CARTESIAN_POINT('Ctrl Pts',(31.3682814586617,257.246889338311,20.0344443101927)) ;
#96537=CARTESIAN_POINT('Ctrl Pts',(31.3436676842271,257.215113947874,20.0344443101927)) ;
#96538=CARTESIAN_POINT('Ctrl Pts',(31.3277407164849,257.198755573123,20.0344443101927)) ;
#96539=CARTESIAN_POINT('Ctrl Pts',(31.2896573479193,257.162323560542,20.0344443101927)) ;
#96540=CARTESIAN_POINT('Ctrl Pts',(31.2049490971881,257.124329856327,20.034444310193)) ;
#96541=CARTESIAN_POINT('Ctrl Pts',(31.0560063868325,257.098725310413,20.0344443101932)) ;
#96542=CARTESIAN_POINT('Ctrl Pts',(30.944318021254,257.097275702916,20.0344443101957)) ;
#96543=CARTESIAN_POINT('Ctrl Pts',(30.838497908478,257.101722101022,20.0344443101957)) ;
#96544=CARTESIAN_POINT('Ctrl Pts',(30.8051939597772,257.103121426598,20.0344443101956)) ;
#96545=CARTESIAN_POINT('Ctrl Pts',(30.7718900110764,257.104520752174,20.0344443101956)) ;
#96546=CARTESIAN_POINT('Ctrl Pts',(31.7691956328132,258.17230390171,20.0213203435596)) ;
#96547=CARTESIAN_POINT('Ctrl Pts',(31.7388267566149,258.108715463427,20.0213203435596)) ;
#96548=CARTESIAN_POINT('Ctrl Pts',(31.6781635524218,257.981492660641,20.0213203435577)) ;
#96549=CARTESIAN_POINT('Ctrl Pts',(31.5879636556681,257.790015763526,20.0213203435576)) ;
#96550=CARTESIAN_POINT('Ctrl Pts',(31.5144236671445,257.630932497549,20.0213203435568)) ;
#96551=CARTESIAN_POINT('Ctrl Pts',(31.4695710315332,257.532812090972,20.0213203435565)) ;
#96552=CARTESIAN_POINT('Ctrl Pts',(31.4530160494117,257.496719707522,20.0213203435565)) ;
#96553=CARTESIAN_POINT('Ctrl Pts',(31.4502529920088,257.490702125912,20.0213203435565)) ;
#96554=CARTESIAN_POINT('Ctrl Pts',(31.4474898488209,257.484686149371,20.0213203435565)) ;
#96555=CARTESIAN_POINT('Ctrl Pts',(31.4419487314663,257.47264650244,20.0213203435565)) ;
#96556=CARTESIAN_POINT('Ctrl Pts',(31.4299408940992,257.446557123162,20.0213203435565)) ;
#96557=CARTESIAN_POINT('Ctrl Pts',(31.4036270250294,257.390389643748,20.0213203435566)) ;
#96558=CARTESIAN_POINT('Ctrl Pts',(31.3724463727691,257.326261721467,20.0213203435566)) ;
#96559=CARTESIAN_POINT('Ctrl Pts',(31.3372773403256,257.267591748504,20.0213203435566)) ;
#96560=CARTESIAN_POINT('Ctrl Pts',(31.3153059108559,257.239359411903,20.0213203435566)) ;
#96561=CARTESIAN_POINT('Ctrl Pts',(31.3016914016871,257.225367890183,20.0213203435566)) ;
#96562=CARTESIAN_POINT('Ctrl Pts',(31.2689396577891,257.194146001655,20.0213203435567)) ;
#96563=CARTESIAN_POINT('Ctrl Pts',(31.1955864715343,257.160846289167,20.021320343557)) ;
#96564=CARTESIAN_POINT('Ctrl Pts',(31.0524719945826,257.135355146069,20.0213203435571)) ;
#96565=CARTESIAN_POINT('Ctrl Pts',(30.9444770781476,257.134517598386,20.0213203435596)) ;
#96566=CARTESIAN_POINT('Ctrl Pts',(30.8400620217627,257.138947997199,20.0213203435596)) ;
#96567=CARTESIAN_POINT('Ctrl Pts',(30.8067580730619,257.140347322774,20.0213203435596)) ;
#96568=CARTESIAN_POINT('Ctrl Pts',(30.7734541243611,257.14174664835,20.0213203435596)) ;
#96569=CARTESIAN_POINT('Ctrl Pts',(31.7489464638971,258.181974599884,20.0213203435596)) ;
#96570=CARTESIAN_POINT('Ctrl Pts',(31.7185740965757,258.118378860957,20.0213203435596)) ;
#96571=CARTESIAN_POINT('Ctrl Pts',(31.6578910386864,257.991114488338,20.0213203435577)) ;
#96572=CARTESIAN_POINT('Ctrl Pts',(31.567631288081,257.79951081352,20.0213203435576)) ;
#96573=CARTESIAN_POINT('Ctrl Pts',(31.4940316374113,257.640298396679,20.0213203435568)) ;
#96574=CARTESIAN_POINT('Ctrl Pts',(31.449163234782,257.542143350465,20.0213203435565)) ;
#96575=CARTESIAN_POINT('Ctrl Pts',(31.4326210851137,257.506079046589,20.0213203435565)) ;
#96576=CARTESIAN_POINT('Ctrl Pts',(31.4298611935316,257.500068246514,20.0213203435565)) ;
#96577=CARTESIAN_POINT('Ctrl Pts',(31.4271002177055,257.494057204395,20.0213203435565)) ;
#96578=CARTESIAN_POINT('Ctrl Pts',(31.4215689681375,257.482038502719,20.0213203435565)) ;
#96579=CARTESIAN_POINT('Ctrl Pts',(31.4095784978925,257.455988292376,20.0213203435565)) ;
#96580=CARTESIAN_POINT('Ctrl Pts',(31.3833769551383,257.400055955828,20.0213203435566)) ;
#96581=CARTESIAN_POINT('Ctrl Pts',(31.352487915175,257.336561723898,20.0213203435566)) ;
#96582=CARTESIAN_POINT('Ctrl Pts',(31.318498748845,257.279979678226,20.0213203435566)) ;
#96583=CARTESIAN_POINT('Ctrl Pts',(31.2981495994694,257.253889722425,20.0213203435566)) ;
#96584=CARTESIAN_POINT('Ctrl Pts',(31.2858437484895,257.241279724063,20.0213203435566)) ;
#96585=CARTESIAN_POINT('Ctrl Pts',(31.2571806346872,257.213759459052,20.0213203435567)) ;
#96586=CARTESIAN_POINT('Ctrl Pts',(31.1897565474607,257.182733549511,20.021320343557)) ;
#96587=CARTESIAN_POINT('Ctrl Pts',(31.0509353958286,257.157783514541,20.0213203435571)) ;
#96588=CARTESIAN_POINT('Ctrl Pts',(30.9447220946478,257.157010261813,20.0213203435596)) ;
#96589=CARTESIAN_POINT('Ctrl Pts',(30.8410040455373,257.161368163036,20.0213203435596)) ;
#96590=CARTESIAN_POINT('Ctrl Pts',(30.8077000968365,257.162767488612,20.0213203435596)) ;
#96591=CARTESIAN_POINT('Ctrl Pts',(30.7743961481358,257.164166814187,20.0213203435596)) ;
#96592=CARTESIAN_POINT('Ctrl Pts',(31.7054902563519,258.090883140368,20.0213203435591)) ;
#96593=CARTESIAN_POINT('Ctrl Pts',(31.7058154780415,258.091003801209,20.0213203435591)) ;
#96594=CARTESIAN_POINT('Ctrl Pts',(31.7061407247937,258.091124403856,20.021321257223)) ;
#96595=CARTESIAN_POINT('Ctrl Pts',(31.7217810369761,258.09692067528,20.0214090781983)) ;
#96596=CARTESIAN_POINT('Ctrl Pts',(31.7372849566914,258.102510036199,20.0235188735263)) ;
#96597=CARTESIAN_POINT('Ctrl Pts',(31.7660644064492,258.112763058849,20.0315488691178)) ;
#96598=CARTESIAN_POINT('Ctrl Pts',(31.7797833584836,258.117595557464,20.0373252655719)) ;
#96599=CARTESIAN_POINT('Ctrl Pts',(31.8050910283457,258.126663582567,20.0534375111736)) ;
#96600=CARTESIAN_POINT('Ctrl Pts',(31.8158319004194,258.130527723509,20.0634821410784)) ;
#96601=CARTESIAN_POINT('Ctrl Pts',(31.8286405478397,258.135110091431,20.0816547245696)) ;
#96602=CARTESIAN_POINT('Ctrl Pts',(31.8325699408238,258.1365240484,20.0892046448113)) ;
#96603=CARTESIAN_POINT('Ctrl Pts',(31.8378194809002,258.138400800961,20.1050586526148)) ;
#96604=CARTESIAN_POINT('Ctrl Pts',(31.8391836130392,258.138878696195,20.1131223643512)) ;
#96605=CARTESIAN_POINT('Ctrl Pts',(31.8391836130392,258.138878696195,20.1213203435596)) ;
#96606=CARTESIAN_POINT('',(30.8701100175112,257.060056991359,20.1213203435596)) ;
#96607=CARTESIAN_POINT('Ctrl Pts',(31.8391836130389,258.138878696195,20.1213203435596)) ;
#96608=CARTESIAN_POINT('Ctrl Pts',(31.8161947094271,258.090742958311,20.1213203435596)) ;
#96609=CARTESIAN_POINT('Ctrl Pts',(31.793311036054,258.042524781297,20.1213203435591)) ;
#96610=CARTESIAN_POINT('Ctrl Pts',(31.7705219542047,257.994277738389,20.1213203435586)) ;
#96611=CARTESIAN_POINT('Ctrl Pts',(31.763219062687,257.978816697759,20.1213203435584)) ;
#96612=CARTESIAN_POINT('Ctrl Pts',(31.7559258446855,257.963352350932,20.1213203435583)) ;
#96613=CARTESIAN_POINT('Ctrl Pts',(31.7486423864986,257.947886769573,20.1213203435582)) ;
#96614=CARTESIAN_POINT('Ctrl Pts',(31.7336364378791,257.916023372641,20.1213203435579)) ;
#96615=CARTESIAN_POINT('Ctrl Pts',(31.7186788666546,257.884169716522,20.1213203435578)) ;
#96616=CARTESIAN_POINT('Ctrl Pts',(31.7037592987293,257.852317706678,20.1213203435577)) ;
#96617=CARTESIAN_POINT('Ctrl Pts',(31.6909614196972,257.824995322347,20.1213203435576)) ;
#96618=CARTESIAN_POINT('Ctrl Pts',(31.6781912970159,257.797673558857,20.1213203435576)) ;
#96619=CARTESIAN_POINT('Ctrl Pts',(31.6654605313248,257.770384692618,20.1213203435575)) ;
#96620=CARTESIAN_POINT('Ctrl Pts',(31.6633499687775,257.765860623882,20.1213203435575)) ;
#96621=CARTESIAN_POINT('Ctrl Pts',(31.6612405375509,257.761337564344,20.1213203435575)) ;
#96622=CARTESIAN_POINT('Ctrl Pts',(31.6591323537695,257.756815795697,20.1213203435575)) ;
#96623=CARTESIAN_POINT('Ctrl Pts',(31.6493305524312,257.735792259531,20.1213203435574)) ;
#96624=CARTESIAN_POINT('Ctrl Pts',(31.6395692606201,257.714825762861,20.1213203435573)) ;
#96625=CARTESIAN_POINT('Ctrl Pts',(31.6298125740882,257.693842295384,20.1213203435572)) ;
#96626=CARTESIAN_POINT('Ctrl Pts',(31.6207074593623,257.67426014748,20.1213203435572)) ;
#96627=CARTESIAN_POINT('Ctrl Pts',(31.6116061277011,257.654662670896,20.1213203435571)) ;
#96628=CARTESIAN_POINT('Ctrl Pts',(31.6024983920955,257.6350301264,20.121320343557)) ;
#96629=CARTESIAN_POINT('Ctrl Pts',(31.5941252568093,257.616981079064,20.1213203435569)) ;
#96630=CARTESIAN_POINT('Ctrl Pts',(31.5857465930023,257.598902102712,20.1213203435568)) ;
#96631=CARTESIAN_POINT('Ctrl Pts',(31.5773733235883,257.580818658925,20.1213203435568)) ;
#96632=CARTESIAN_POINT('Ctrl Pts',(31.5750924224581,257.575892680155,20.1213203435568)) ;
#96633=CARTESIAN_POINT('Ctrl Pts',(31.5728120430202,257.57096663462,20.1213203435567)) ;
#96634=CARTESIAN_POINT('Ctrl Pts',(31.5705326966186,257.566041672035,20.1213203435567)) ;
#96635=CARTESIAN_POINT('Ctrl Pts',(31.5639474099359,257.551812904305,20.1213203435567)) ;
#96636=CARTESIAN_POINT('Ctrl Pts',(31.5573679174951,257.537587063929,20.1213203435566)) ;
#96637=CARTESIAN_POINT('Ctrl Pts',(31.5507742308301,257.523322084297,20.1213203435566)) ;
#96638=CARTESIAN_POINT('Ctrl Pts',(31.5446786159545,257.510134648123,20.1213203435565)) ;
#96639=CARTESIAN_POINT('Ctrl Pts',(31.5385707666793,257.496913509859,20.1213203435565)) ;
#96640=CARTESIAN_POINT('Ctrl Pts',(31.532453652466,257.483666271913,20.1213203435565)) ;
#96641=CARTESIAN_POINT('Ctrl Pts',(31.5303660108531,257.479145269978,20.1213203435565)) ;
#96642=CARTESIAN_POINT('Ctrl Pts',(31.5282774683563,257.474621617872,20.1213203435565)) ;
#96643=CARTESIAN_POINT('Ctrl Pts',(31.5261887405501,257.470096927279,20.1213203435565)) ;
#96644=CARTESIAN_POINT('Ctrl Pts',(31.5252619024114,257.468089171268,20.1213203435565)) ;
#96645=CARTESIAN_POINT('Ctrl Pts',(31.5243348062921,257.466080731128,20.1213203435565)) ;
#96646=CARTESIAN_POINT('Ctrl Pts',(31.5234072657788,257.464071208821,20.1213203435565)) ;
#96647=CARTESIAN_POINT('Ctrl Pts',(31.5206246442389,257.458042641898,20.1213203435565)) ;
#96648=CARTESIAN_POINT('Ctrl Pts',(31.5178386301049,257.452005647303,20.1213203435565)) ;
#96649=CARTESIAN_POINT('Ctrl Pts',(31.5150484732124,257.445958780731,20.1213203435565)) ;
#96650=CARTESIAN_POINT('Ctrl Pts',(31.5132912927696,257.442150594995,20.1213203435565)) ;
#96651=CARTESIAN_POINT('Ctrl Pts',(31.5115322300475,257.438337975969,20.1213203435565)) ;
#96652=CARTESIAN_POINT('Ctrl Pts',(31.509772818656,257.434524303432,20.1213203435565)) ;
#96653=CARTESIAN_POINT('Ctrl Pts',(31.5078072976114,257.430263870844,20.1213203435565)) ;
#96654=CARTESIAN_POINT('Ctrl Pts',(31.5058437201315,257.425992735893,20.1213203435565)) ;
#96655=CARTESIAN_POINT('Ctrl Pts',(31.5038815376229,257.421712469162,20.1213203435565)) ;
#96656=CARTESIAN_POINT('Ctrl Pts',(31.4975523389697,257.407906078415,20.1213203435565)) ;
#96657=CARTESIAN_POINT('Ctrl Pts',(31.4912358139239,257.393993745983,20.1213203435565)) ;
#96658=CARTESIAN_POINT('Ctrl Pts',(31.4848699785717,257.379985562715,20.1213203435566)) ;
#96659=CARTESIAN_POINT('Ctrl Pts',(31.4837555525691,257.377533239835,20.1213203435566)) ;
#96660=CARTESIAN_POINT('Ctrl Pts',(31.4826395531966,257.375078092253,20.1213203435566)) ;
#96661=CARTESIAN_POINT('Ctrl Pts',(31.4815215526911,257.372620316615,20.1213203435566)) ;
#96662=CARTESIAN_POINT('Ctrl Pts',(31.4766434373058,257.361896427766,20.1213203435566)) ;
#96663=CARTESIAN_POINT('Ctrl Pts',(31.4717384967145,257.351142007976,20.1213203435566)) ;
#96664=CARTESIAN_POINT('Ctrl Pts',(31.4667122855711,257.340279417221,20.1213203435566)) ;
#96665=CARTESIAN_POINT('Ctrl Pts',(31.4619026837029,257.329884959985,20.1213203435566)) ;
#96666=CARTESIAN_POINT('Ctrl Pts',(31.456983429614,257.319391751533,20.1213203435566)) ;
#96667=CARTESIAN_POINT('Ctrl Pts',(31.4518530945931,257.308774346739,20.1213203435566)) ;
#96668=CARTESIAN_POINT('Ctrl Pts',(31.4472164096362,257.299178567733,20.1213203435566)) ;
#96669=CARTESIAN_POINT('Ctrl Pts',(31.4424083086682,257.289481950142,20.1213203435566)) ;
#96670=CARTESIAN_POINT('Ctrl Pts',(31.4373224728242,257.279694483374,20.1213203435566)) ;
#96671=CARTESIAN_POINT('Ctrl Pts',(31.4358230654828,257.276808940077,20.1213203435566)) ;
#96672=CARTESIAN_POINT('Ctrl Pts',(31.4342992376485,257.273915674778,20.1213203435566)) ;
#96673=CARTESIAN_POINT('Ctrl Pts',(31.4327474548286,257.271015368647,20.1213203435566)) ;
#96674=CARTESIAN_POINT('Ctrl Pts',(31.4286512948732,257.263359582234,20.1213203435566)) ;
#96675=CARTESIAN_POINT('Ctrl Pts',(31.4243584117938,257.255643973918,20.1213203435566)) ;
#96676=CARTESIAN_POINT('Ctrl Pts',(31.419744467576,257.247826312544,20.1213203435566)) ;
#96677=CARTESIAN_POINT('Ctrl Pts',(31.4157201000424,257.241007603619,20.1213203435566)) ;
#96678=CARTESIAN_POINT('Ctrl Pts',(31.4114518978677,257.234111772635,20.1213203435566)) ;
#96679=CARTESIAN_POINT('Ctrl Pts',(31.4068277629769,257.22712911912,20.1213203435566)) ;
#96680=CARTESIAN_POINT('Ctrl Pts',(31.4035112192784,257.22212098764,20.1213203435566)) ;
#96681=CARTESIAN_POINT('Ctrl Pts',(31.4000098313069,257.217066848291,20.1213203435566)) ;
#96682=CARTESIAN_POINT('Ctrl Pts',(31.3962725453509,257.211973553155,20.1213203435566)) ;
#96683=CARTESIAN_POINT('Ctrl Pts',(31.3908345527168,257.204562479516,20.1213203435566)) ;
#96684=CARTESIAN_POINT('Ctrl Pts',(31.3849071071445,257.197083054429,20.1213203435566)) ;
#96685=CARTESIAN_POINT('Ctrl Pts',(31.3783637344278,257.189642216166,20.1213203435566)) ;
#96686=CARTESIAN_POINT('Ctrl Pts',(31.3741084934393,257.184803341577,20.1213203435566)) ;
#96687=CARTESIAN_POINT('Ctrl Pts',(31.3695918484284,257.179980247687,20.1213203435566)) ;
#96688=CARTESIAN_POINT('Ctrl Pts',(31.3647692135685,257.175195683227,20.1213203435566)) ;
#96689=CARTESIAN_POINT('Ctrl Pts',(31.3624414920458,257.17288633699,20.1213203435566)) ;
#96690=CARTESIAN_POINT('Ctrl Pts',(31.3600437861251,257.170587098048,20.1213203435566)) ;
#96691=CARTESIAN_POINT('Ctrl Pts',(31.3575620270058,257.168292523018,20.1213203435566)) ;
#96692=CARTESIAN_POINT('Ctrl Pts',(31.3550802678865,257.165997947987,20.1213203435566)) ;
#96693=CARTESIAN_POINT('Ctrl Pts',(31.3525136339308,257.163708938113,20.1213203435566)) ;
#96694=CARTESIAN_POINT('Ctrl Pts',(31.3499252983641,257.161483805886,20.1213203435566)) ;
#96695=CARTESIAN_POINT('Ctrl Pts',(31.34180172865,257.154500160876,20.1213203435566)) ;
#96696=CARTESIAN_POINT('Ctrl Pts',(31.3334934711741,257.148157614545,20.1213203435567)) ;
#96697=CARTESIAN_POINT('Ctrl Pts',(31.3250514390484,257.142337795154,20.1213203435567)) ;
#96698=CARTESIAN_POINT('Ctrl Pts',(31.3158472909083,257.135992583594,20.1213203435567)) ;
#96699=CARTESIAN_POINT('Ctrl Pts',(31.3064844393971,257.13026861466,20.1213203435567)) ;
#96700=CARTESIAN_POINT('Ctrl Pts',(31.2970839532443,257.12504942768,20.1213203435567)) ;
#96701=CARTESIAN_POINT('Ctrl Pts',(31.2885502552192,257.120311484887,20.1213203435568)) ;
#96702=CARTESIAN_POINT('Ctrl Pts',(31.2799868778864,257.115990220132,20.1213203435568)) ;
#96703=CARTESIAN_POINT('Ctrl Pts',(31.2715131924955,257.112021656713,20.1213203435568)) ;
#96704=CARTESIAN_POINT('Ctrl Pts',(31.2611099851996,257.107149421551,20.1213203435568)) ;
#96705=CARTESIAN_POINT('Ctrl Pts',(31.2503865049053,257.102794974448,20.1213203435569)) ;
#96706=CARTESIAN_POINT('Ctrl Pts',(31.2397927939429,257.098958254889,20.1213203435569)) ;
#96707=CARTESIAN_POINT('Ctrl Pts',(31.2327938866677,257.096423463773,20.1213203435569)) ;
#96708=CARTESIAN_POINT('Ctrl Pts',(31.225851783864,257.094113215673,20.1213203435569)) ;
#96709=CARTESIAN_POINT('Ctrl Pts',(31.2190923526486,257.092015936192,20.1213203435569)) ;
#96710=CARTESIAN_POINT('Ctrl Pts',(31.2102760763554,257.089280470029,20.121320343557)) ;
#96711=CARTESIAN_POINT('Ctrl Pts',(31.2015479560693,257.086836159472,20.121320343557)) ;
#96712=CARTESIAN_POINT('Ctrl Pts',(31.192961649612,257.084631260979,20.121320343557)) ;
#96713=CARTESIAN_POINT('Ctrl Pts',(31.1840312842957,257.082338010776,20.121320343557)) ;
#96714=CARTESIAN_POINT('Ctrl Pts',(31.1752542408135,257.080303377449,20.121320343557)) ;
#96715=CARTESIAN_POINT('Ctrl Pts',(31.1666337736506,257.078472857046,20.121320343557)) ;
#96716=CARTESIAN_POINT('Ctrl Pts',(31.1578040570914,257.076597903402,20.1213203435571)) ;
#96717=CARTESIAN_POINT('Ctrl Pts',(31.1491383134557,257.074936861673,20.1213203435571)) ;
#96718=CARTESIAN_POINT('Ctrl Pts',(31.1405845422787,257.073439581227,20.1213203435571)) ;
#96719=CARTESIAN_POINT('Ctrl Pts',(31.1317559096289,257.071894188119,20.1213203435571)) ;
#96720=CARTESIAN_POINT('Ctrl Pts',(31.1230463636819,257.070523075047,20.1213203435572)) ;
#96721=CARTESIAN_POINT('Ctrl Pts',(31.1143441789641,257.069283073925,20.1213203435572)) ;
#96722=CARTESIAN_POINT('Ctrl Pts',(31.1090904981052,257.068534460747,20.1213203435573)) ;
#96723=CARTESIAN_POINT('Ctrl Pts',(31.1038384763594,257.067833878059,20.1213203435573)) ;
#96724=CARTESIAN_POINT('Ctrl Pts',(31.0985547216863,257.06717420603,20.1213203435573)) ;
#96725=CARTESIAN_POINT('Ctrl Pts',(31.0822151079867,257.065134219923,20.1213203435575)) ;
#96726=CARTESIAN_POINT('Ctrl Pts',(31.0658113380929,257.063516915152,20.1213203435576)) ;
#96727=CARTESIAN_POINT('Ctrl Pts',(31.0494699256462,257.062255478661,20.1213203435578)) ;
#96728=CARTESIAN_POINT('Ctrl Pts',(31.0329217121231,257.060978078653,20.121320343558)) ;
#96729=CARTESIAN_POINT('Ctrl Pts',(31.0164374106932,257.060065168486,20.1213203435582)) ;
#96730=CARTESIAN_POINT('Ctrl Pts',(31.0000947450752,257.059451949941,20.1213203435585)) ;
#96731=CARTESIAN_POINT('Ctrl Pts',(30.9835705235233,257.058831918954,20.1213203435587)) ;
#96732=CARTESIAN_POINT('Ctrl Pts',(30.9671909481073,257.058517989808,20.1213203435589)) ;
#96733=CARTESIAN_POINT('Ctrl Pts',(30.9509833440119,257.058453340951,20.1213203435591)) ;
#96734=CARTESIAN_POINT('Ctrl Pts',(30.9344197759284,257.058387272226,20.1213203435593)) ;
#96735=CARTESIAN_POINT('Ctrl Pts',(30.9180356893947,257.058581350378,20.1213203435594)) ;
#96736=CARTESIAN_POINT('Ctrl Pts',(30.9018072392188,257.058989232507,20.1213203435595)) ;
#96737=CARTESIAN_POINT('Ctrl Pts',(30.891562852584,257.05924671256,20.1213203435596)) ;
#96738=CARTESIAN_POINT('Ctrl Pts',(30.8813794324915,257.059589694101,20.1213203435596)) ;
#96739=CARTESIAN_POINT('Ctrl Pts',(30.8712408692026,257.060009804349,20.1213203435596)) ;
#96740=CARTESIAN_POINT('Ctrl Pts',(30.8708637790654,257.060025429781,20.1213203435596)) ;
#96741=CARTESIAN_POINT('Ctrl Pts',(30.8704868289408,257.060041158946,20.1213203435596)) ;
#96742=CARTESIAN_POINT('Ctrl Pts',(30.8701100175113,257.060056991359,20.1213203435596)) ;
#96743=CARTESIAN_POINT('Ctrl Pts',(30.7743961481367,257.164166814187,20.0213203435596)) ;
#96744=CARTESIAN_POINT('Ctrl Pts',(30.7746326029829,257.163914930351,20.0213203435596)) ;
#96745=CARTESIAN_POINT('Ctrl Pts',(30.7748690126325,257.163663002226,20.0213212573643)) ;
#96746=CARTESIAN_POINT('Ctrl Pts',(30.7862474765949,257.151533217284,20.0214091930669)) ;
#96747=CARTESIAN_POINT('Ctrl Pts',(30.7973822007925,257.139448779789,20.0235241814884)) ;
#96748=CARTESIAN_POINT('Ctrl Pts',(30.8179379288125,257.116974935591,20.0315745600298)) ;
#96749=CARTESIAN_POINT('Ctrl Pts',(30.8276826449037,257.106246996249,20.0373654819654)) ;
#96750=CARTESIAN_POINT('Ctrl Pts',(30.8457792331966,257.086541872235,20.0535013924982)) ;
#96751=CARTESIAN_POINT('Ctrl Pts',(30.8534645081883,257.078193034956,20.0635493061725)) ;
#96752=CARTESIAN_POINT('Ctrl Pts',(30.862600318185,257.068236069426,20.0817133908593)) ;
#96753=CARTESIAN_POINT('Ctrl Pts',(30.8654074439578,257.065190004858,20.0892538401936)) ;
#96754=CARTESIAN_POINT('Ctrl Pts',(30.8691476327655,257.061117063952,20.1050848833404)) ;
#96755=CARTESIAN_POINT('Ctrl Pts',(30.8701100175112,257.060056991359,20.1131368914135)) ;
#96756=CARTESIAN_POINT('Ctrl Pts',(30.8701100175112,257.060056991359,20.1213203435596)) ;
#96757=CARTESIAN_POINT('Origin',(30.4489043471128,249.417461949796,20.1213203435596)) ;
#96758=CARTESIAN_POINT('',(30.853318115509,256.660409724306,20.1213203435596)) ;
#96759=CARTESIAN_POINT('',(30.5488161932143,249.413263973069,20.1213203435596)) ;
#96760=CARTESIAN_POINT('Ctrl Pts',(30.8533181205427,256.660409843506,20.1213203435596)) ;
#96761=CARTESIAN_POINT('Ctrl Pts',(30.8533181205427,256.660409843506,20.1131416452177)) ;
#96762=CARTESIAN_POINT('Ctrl Pts',(30.852270661312,256.659427382356,20.1050923261438)) ;
#96763=CARTESIAN_POINT('Ctrl Pts',(30.848206446685,256.6556792969,20.0892708055417)) ;
#96764=CARTESIAN_POINT('Ctrl Pts',(30.8451552021593,256.652881747536,20.0817291561053)) ;
#96765=CARTESIAN_POINT('Ctrl Pts',(30.8352215948528,256.643740521483,20.0635661934299)) ;
#96766=CARTESIAN_POINT('Ctrl Pts',(30.8268708481235,256.636074154367,20.0535155318311)) ;
#96767=CARTESIAN_POINT('Ctrl Pts',(30.8071303445457,256.617958965926,20.0373366241602)) ;
#96768=CARTESIAN_POINT('Ctrl Pts',(30.7964637143612,256.608111454119,20.0315189424004)) ;
#96769=CARTESIAN_POINT('Ctrl Pts',(30.7739733916521,256.587476318765,20.0234653725465)) ;
#96770=CARTESIAN_POINT('Ctrl Pts',(30.7619107901203,256.576402602838,20.0214062385825)) ;
#96771=CARTESIAN_POINT('Ctrl Pts',(30.7497119762593,256.565159924822,20.0213212211531)) ;
#96772=CARTESIAN_POINT('Ctrl Pts',(30.7494601335157,256.564927828289,20.0213203435596)) ;
#96773=CARTESIAN_POINT('Ctrl Pts',(30.7492082877751,256.564695737578,20.0213203435596)) ;
#96774=CARTESIAN_POINT('Origin',(44.5070901774322,252.121399060531,20.1213203435596)) ;
#96775=CARTESIAN_POINT('Origin',(31.2093839453833,258.32222131243,20.1213203435596)) ;
#96776=CARTESIAN_POINT('Origin',(33.9819120129541,260.896418149051,20.1213203435596)) ;
#96777=CARTESIAN_POINT('Origin',(32.8217003142836,259.81920153961,20.1213203435596)) ;
#96778=CARTESIAN_POINT('Origin',(32.319849148055,249.82847140953,20.1213203435596)) ;
#96779=CARTESIAN_POINT('Origin',(32.7113239146176,257.621855202687,20.1213203435596)) ;
#96780=CARTESIAN_POINT('Origin',(44.9147880370394,251.931286426383,20.1213203435596)) ;
#96781=CARTESIAN_POINT('Ctrl Pts',(32.2494313841384,257.837239226894,20.0213203435596)) ;
#96782=CARTESIAN_POINT('Ctrl Pts',(32.2493153942693,257.837560219903,20.0213203435596)) ;
#96783=CARTESIAN_POINT('Ctrl Pts',(32.2491993914172,257.83788121024,20.0213212212867)) ;
#96784=CARTESIAN_POINT('Ctrl Pts',(32.2435730092924,257.853448270305,20.021406349793)) ;
#96785=CARTESIAN_POINT('Ctrl Pts',(32.2380346526045,257.868835513893,20.0234710123247)) ;
#96786=CARTESIAN_POINT('Ctrl Pts',(32.2277406393474,257.897506337361,20.0315483482936)) ;
#96787=CARTESIAN_POINT('Ctrl Pts',(32.2228080732768,257.911121026691,20.0373826504411)) ;
#96788=CARTESIAN_POINT('Ctrl Pts',(32.2137969550926,257.936231034257,20.0535836290149)) ;
#96789=CARTESIAN_POINT('Ctrl Pts',(32.2099856311187,257.946839250697,20.0636304094217)) ;
#96790=CARTESIAN_POINT('Ctrl Pts',(32.205442564853,257.959461423177,20.081776839957)) ;
#96791=CARTESIAN_POINT('Ctrl Pts',(32.2040624233514,257.963329996811,20.0893091862125)) ;
#96792=CARTESIAN_POINT('Ctrl Pts',(32.2022100389283,257.968490994962,20.1051145990528)) ;
#96793=CARTESIAN_POINT('Ctrl Pts',(32.201722180204,257.96982418595,20.1131541545092)) ;
#96794=CARTESIAN_POINT('Ctrl Pts',(32.201722180204,257.96982418595,20.1213203435596)) ;
#96795=CARTESIAN_POINT('Ctrl Pts',(30.753406264502,256.66460758368,20.1213203435596)) ;
#96796=CARTESIAN_POINT('Ctrl Pts',(30.7867102132026,256.663208258104,20.1213203435596)) ;
#96797=CARTESIAN_POINT('Ctrl Pts',(30.8200141619031,256.661808932529,20.1213203435596)) ;
#96798=CARTESIAN_POINT('Ctrl Pts',(31.0531097612377,256.652014999784,20.1213203435596)) ;
#96799=CARTESIAN_POINT('Ctrl Pts',(31.3534533862626,256.674660174757,20.1213203435596)) ;
#96800=CARTESIAN_POINT('Ctrl Pts',(31.6605197347822,256.879677823259,20.1213203435596)) ;
#96801=CARTESIAN_POINT('Ctrl Pts',(31.8101800588843,257.116691929027,20.1213203435596)) ;
#96802=CARTESIAN_POINT('Ctrl Pts',(31.9242228131995,257.380707018173,20.1213203435596)) ;
#96803=CARTESIAN_POINT('Ctrl Pts',(32.0570123966128,257.663429119505,20.1213203435596)) ;
#96804=CARTESIAN_POINT('Ctrl Pts',(32.1456747857374,257.852474228961,20.1213203435596)) ;
#96805=CARTESIAN_POINT('Ctrl Pts',(32.2017221802041,257.96982418595,20.1213203435596)) ;
#96806=CARTESIAN_POINT('Ctrl Pts',(30.753406264502,256.66460758368,20.1063603785425)) ;
#96807=CARTESIAN_POINT('Ctrl Pts',(30.7867102132026,256.663208258104,20.1063603785425)) ;
#96808=CARTESIAN_POINT('Ctrl Pts',(30.8200141619031,256.661808932529,20.1063603785425)) ;
#96809=CARTESIAN_POINT('Ctrl Pts',(31.0531097612377,256.652014999784,20.1063603785425)) ;
#96810=CARTESIAN_POINT('Ctrl Pts',(31.3534533862626,256.674660174757,20.1063603785425)) ;
#96811=CARTESIAN_POINT('Ctrl Pts',(31.6605197347822,256.879677823259,20.1063603785425)) ;
#96812=CARTESIAN_POINT('Ctrl Pts',(31.8101800588843,257.116691929027,20.1063603785425)) ;
#96813=CARTESIAN_POINT('Ctrl Pts',(31.9242228131995,257.380707018173,20.1063603785425)) ;
#96814=CARTESIAN_POINT('Ctrl Pts',(32.0570123966128,257.663429119505,20.1063603785425)) ;
#96815=CARTESIAN_POINT('Ctrl Pts',(32.1456747857374,257.852474228961,20.1063603785425)) ;
#96816=CARTESIAN_POINT('Ctrl Pts',(32.2017221802041,257.96982418595,20.1063603785425)) ;
#96817=CARTESIAN_POINT('Ctrl Pts',(30.7531194015905,256.657780246386,20.0764517751007)) ;
#96818=CARTESIAN_POINT('Ctrl Pts',(30.786423350291,256.65638092081,20.0764517751007)) ;
#96819=CARTESIAN_POINT('Ctrl Pts',(30.8197272989916,256.654981595234,20.0764517751007)) ;
#96820=CARTESIAN_POINT('Ctrl Pts',(31.0536921529186,256.64482049014,20.0764517751007)) ;
#96821=CARTESIAN_POINT('Ctrl Pts',(31.3553494356536,256.667797230937,20.0764517751007)) ;
#96822=CARTESIAN_POINT('Ctrl Pts',(31.66580693853,256.874741802429,20.0764517751007)) ;
#96823=CARTESIAN_POINT('Ctrl Pts',(31.8165721794156,257.113917383899,20.0764517751007)) ;
#96824=CARTESIAN_POINT('Ctrl Pts',(31.9305266534185,257.377866256042,20.0764517751007)) ;
#96825=CARTESIAN_POINT('Ctrl Pts',(32.0632111374223,257.660448052357,20.0764517751007)) ;
#96826=CARTESIAN_POINT('Ctrl Pts',(32.1520275174255,257.849713728641,20.0764517751007)) ;
#96827=CARTESIAN_POINT('Ctrl Pts',(32.2078883528472,257.96687916646,20.0764517751007)) ;
#96828=CARTESIAN_POINT('Ctrl Pts',(30.7519150570582,256.629116846515,20.0404585252547)) ;
#96829=CARTESIAN_POINT('Ctrl Pts',(30.7852190057587,256.62771752094,20.0404585252546)) ;
#96830=CARTESIAN_POINT('Ctrl Pts',(30.8185229544592,256.626318195364,20.0404585252547)) ;
#96831=CARTESIAN_POINT('Ctrl Pts',(31.0547005508067,256.616146526555,20.0404585252547)) ;
#96832=CARTESIAN_POINT('Ctrl Pts',(31.3629325847851,256.638409046288,20.0404585252546)) ;
#96833=CARTESIAN_POINT('Ctrl Pts',(31.6873976939643,256.854298178497,20.0404585252547)) ;
#96834=CARTESIAN_POINT('Ctrl Pts',(31.8430521064208,257.10234330074,20.0404585252546)) ;
#96835=CARTESIAN_POINT('Ctrl Pts',(31.9565799920417,257.365847966563,20.0404585252547)) ;
#96836=CARTESIAN_POINT('Ctrl Pts',(32.0892804342346,257.64827986717,20.0404585252547)) ;
#96837=CARTESIAN_POINT('Ctrl Pts',(32.17787741575,257.83732196866,20.0404585252547)) ;
#96838=CARTESIAN_POINT('Ctrl Pts',(32.2337759667908,257.954515009303,20.0404585252547)) ;
#96839=CARTESIAN_POINT('Ctrl Pts',(30.7504644798715,256.594593109473,20.0238261114369)) ;
#96840=CARTESIAN_POINT('Ctrl Pts',(30.7837684285721,256.593193783897,20.0238261114369)) ;
#96841=CARTESIAN_POINT('Ctrl Pts',(30.8170723772726,256.591794458321,20.023826111437)) ;
#96842=CARTESIAN_POINT('Ctrl Pts',(31.0559072718364,256.581618428455,20.0238261114369)) ;
#96843=CARTESIAN_POINT('Ctrl Pts',(31.3720640767969,256.603009197133,20.0238261114369)) ;
#96844=CARTESIAN_POINT('Ctrl Pts',(31.7133994447527,256.829676306926,20.0238261114369)) ;
#96845=CARTESIAN_POINT('Ctrl Pts',(31.8749440054121,257.088403260065,20.0238261114369)) ;
#96846=CARTESIAN_POINT('Ctrl Pts',(31.9879577794308,257.351371992096,20.0238261114369)) ;
#96847=CARTESIAN_POINT('Ctrl Pts',(32.1206799398744,257.63362574903,20.0238261114369)) ;
#96848=CARTESIAN_POINT('Ctrl Pts',(32.2090079362795,257.822392285682,20.0238261114369)) ;
#96849=CARTESIAN_POINT('Ctrl Pts',(32.2649563982988,257.939622954894,20.0238261114369)) ;
#96850=CARTESIAN_POINT('Ctrl Pts',(30.7495222957,256.572169126191,20.0213203435596)) ;
#96851=CARTESIAN_POINT('Ctrl Pts',(30.7828262444005,256.570769800615,20.0213203435596)) ;
#96852=CARTESIAN_POINT('Ctrl Pts',(30.8161301931011,256.569370475039,20.0213203435597)) ;
#96853=CARTESIAN_POINT('Ctrl Pts',(31.0567131604158,256.559168067985,20.0213203435596)) ;
#96854=CARTESIAN_POINT('Ctrl Pts',(31.3780009959797,256.580025005874,20.0213203435596)) ;
#96855=CARTESIAN_POINT('Ctrl Pts',(31.7302975263905,256.81367952226,20.0213203435596)) ;
#96856=CARTESIAN_POINT('Ctrl Pts',(31.8956640270926,257.079347730437,20.0213203435596)) ;
#96857=CARTESIAN_POINT('Ctrl Pts',(32.0083447340676,257.341970916896,20.0213203435596)) ;
#96858=CARTESIAN_POINT('Ctrl Pts',(32.1410739697034,257.624102211558,20.0213203435596)) ;
#96859=CARTESIAN_POINT('Ctrl Pts',(32.2292405707272,257.812707441946,20.0213203435596)) ;
#96860=CARTESIAN_POINT('Ctrl Pts',(32.285208825607,257.929950213537,20.0213203435596)) ;
#96861=CARTESIAN_POINT('Ctrl Pts',(30.7492082877751,256.564695737578,20.0213203435596)) ;
#96862=CARTESIAN_POINT('Ctrl Pts',(30.7825122364757,256.563296412003,20.0213203435596)) ;
#96863=CARTESIAN_POINT('Ctrl Pts',(30.8158161851762,256.561897086427,20.0213203435597)) ;
#96864=CARTESIAN_POINT('Ctrl Pts',(31.0569053558616,256.55176728934,20.0213203435596)) ;
#96865=CARTESIAN_POINT('Ctrl Pts',(31.3799595822748,256.57233432435,20.0213203435596)) ;
#96866=CARTESIAN_POINT('Ctrl Pts',(31.735897005124,256.808363024752,20.0213203435596)) ;
#96867=CARTESIAN_POINT('Ctrl Pts',(31.9025505811396,257.076333688533,20.0213203435596)) ;
#96868=CARTESIAN_POINT('Ctrl Pts',(32.0151173093266,257.33883287554,20.0213203435596)) ;
#96869=CARTESIAN_POINT('Ctrl Pts',(32.1478732124172,257.62094670617,20.0213203435596)) ;
#96870=CARTESIAN_POINT('Ctrl Pts',(32.2359399838344,257.809437053091,20.0213203435596)) ;
#96871=CARTESIAN_POINT('Ctrl Pts',(32.2919584854562,257.926726515311,20.0213203435596)) ;
#96872=CARTESIAN_POINT('Ctrl Pts',(30.8533181204414,256.66040984351,20.1213203435596)) ;
#96873=CARTESIAN_POINT('Ctrl Pts',(31.0538433767003,256.652070516101,20.1213203435596)) ;
#96874=CARTESIAN_POINT('Ctrl Pts',(31.3537346899415,256.674847991556,20.1213203435596)) ;
#96875=CARTESIAN_POINT('Ctrl Pts',(31.6605197347822,256.879677823259,20.1213203435596)) ;
#96876=CARTESIAN_POINT('Ctrl Pts',(31.8101800588843,257.116691929027,20.1213203435596)) ;
#96877=CARTESIAN_POINT('Ctrl Pts',(31.9242228131995,257.380707018173,20.1213203435596)) ;
#96878=CARTESIAN_POINT('Ctrl Pts',(32.0570123966128,257.663429119505,20.1213203435596)) ;
#96879=CARTESIAN_POINT('Ctrl Pts',(32.1456747857374,257.852474228961,20.1213203435596)) ;
#96880=CARTESIAN_POINT('Ctrl Pts',(32.2017221802041,257.96982418595,20.1213203435596)) ;
#96881=CARTESIAN_POINT('Ctrl Pts',(30.8533181106036,256.660409606953,20.0213203435596)) ;
#96882=CARTESIAN_POINT('Ctrl Pts',(30.8533181106036,256.660409606953,20.3813203435596)) ;
#96883=CARTESIAN_POINT('Ctrl Pts',(31.2255082708192,256.644771364927,20.0213203435596)) ;
#96884=CARTESIAN_POINT('Ctrl Pts',(31.2255082708192,256.644771364927,20.3813203435596)) ;
#96885=CARTESIAN_POINT('Ctrl Pts',(31.4869115990368,256.735802916448,20.0213203435596)) ;
#96886=CARTESIAN_POINT('Ctrl Pts',(31.4869115990368,256.735802916448,20.3813203435596)) ;
#96887=CARTESIAN_POINT('Ctrl Pts',(31.6392361795028,256.887658160472,20.0213203435596)) ;
#96888=CARTESIAN_POINT('Ctrl Pts',(31.6392361795028,256.887658160472,20.3813203435596)) ;
#96889=CARTESIAN_POINT('Ctrl Pts',(31.8202190831926,257.068083426833,20.0213203435596)) ;
#96890=CARTESIAN_POINT('Ctrl Pts',(31.8202190831926,257.068083426833,20.3813203435596)) ;
#96891=CARTESIAN_POINT('Ctrl Pts',(31.8533149361085,257.224893291544,20.0213203435596)) ;
#96892=CARTESIAN_POINT('Ctrl Pts',(31.8533149361085,257.224893291544,20.3813203435596)) ;
#96893=CARTESIAN_POINT('Ctrl Pts',(31.9557184877316,257.447246089354,20.0213203435596)) ;
#96894=CARTESIAN_POINT('Ctrl Pts',(31.9557184877316,257.447246089354,20.3813203435596)) ;
#96895=CARTESIAN_POINT('Ctrl Pts',(32.0253094429367,257.598351625704,20.0213203435596)) ;
#96896=CARTESIAN_POINT('Ctrl Pts',(32.0253094429367,257.598351625704,20.3813203435596)) ;
#96897=CARTESIAN_POINT('Ctrl Pts',(32.1145256312286,257.787255283878,20.0213203435596)) ;
#96898=CARTESIAN_POINT('Ctrl Pts',(32.1145256312286,257.787255283878,20.3813203435596)) ;
#96899=CARTESIAN_POINT('Ctrl Pts',(32.201722180204,257.969824185949,20.0213203435596)) ;
#96900=CARTESIAN_POINT('Ctrl Pts',(32.201722180204,257.969824185949,20.3813203435596)) ;
#96901=CARTESIAN_POINT('',(30.8533181106036,256.660409606953,20.0213203435596)) ;
#96902=CARTESIAN_POINT('Origin',(30.8701100175113,257.060056991358,20.0213203435596)) ;
#96903=CARTESIAN_POINT('',(30.8701100175112,257.060056991359,20.0213203435596)) ;
#96904=CARTESIAN_POINT('Ctrl Pts',(31.8391836130389,258.138878696195,20.0213203435596)) ;
#96905=CARTESIAN_POINT('Ctrl Pts',(31.8391836130389,258.138878696195,20.3813203435596)) ;
#96906=CARTESIAN_POINT('Ctrl Pts',(31.7162037244466,257.881374998661,20.0213203435596)) ;
#96907=CARTESIAN_POINT('Ctrl Pts',(31.7162037244466,257.881374998661,20.3813203435596)) ;
#96908=CARTESIAN_POINT('Ctrl Pts',(31.5892548552809,257.6068083194,20.0213203435596)) ;
#96909=CARTESIAN_POINT('Ctrl Pts',(31.5892548552809,257.6068083194,20.3813203435596)) ;
#96910=CARTESIAN_POINT('Ctrl Pts',(31.509772818656,257.434524303432,20.0213203435596)) ;
#96911=CARTESIAN_POINT('Ctrl Pts',(31.509772818656,257.434524303432,20.3813203435596)) ;
#96912=CARTESIAN_POINT('Ctrl Pts',(31.4282577248589,257.257833464625,20.0213203435596)) ;
#96913=CARTESIAN_POINT('Ctrl Pts',(31.4282577248589,257.257833464625,20.3813203435596)) ;
#96914=CARTESIAN_POINT('Ctrl Pts',(31.4006948106297,257.172522539205,20.0213203435596)) ;
#96915=CARTESIAN_POINT('Ctrl Pts',(31.4006948106297,257.172522539205,20.3813203435596)) ;
#96916=CARTESIAN_POINT('Ctrl Pts',(31.2715131924955,257.112021656713,20.0213203435596)) ;
#96917=CARTESIAN_POINT('Ctrl Pts',(31.2715131924955,257.112021656713,20.3813203435596)) ;
#96918=CARTESIAN_POINT('Ctrl Pts',(31.1997685794864,257.078420804952,20.0213203435596)) ;
#96919=CARTESIAN_POINT('Ctrl Pts',(31.1997685794864,257.078420804952,20.3813203435596)) ;
#96920=CARTESIAN_POINT('Ctrl Pts',(31.0748905561884,257.051452767045,20.0213203435596)) ;
#96921=CARTESIAN_POINT('Ctrl Pts',(31.0748905561884,257.051452767045,20.3813203435596)) ;
#96922=CARTESIAN_POINT('Ctrl Pts',(30.8701100175112,257.060056991359,20.0213203435596)) ;
#96923=CARTESIAN_POINT('Ctrl Pts',(30.8701100175112,257.060056991359,20.3813203435596)) ;
#96924=CARTESIAN_POINT('Ctrl Pts',(29.5759712687709,255.502885024398,20.1213203435596)) ;
#96925=CARTESIAN_POINT('Ctrl Pts',(29.6096896012297,255.570241420972,20.1213203435596)) ;
#96926=CARTESIAN_POINT('Ctrl Pts',(29.7111240387136,255.772053704706,20.1213203435596)) ;
#96927=CARTESIAN_POINT('Ctrl Pts',(29.8202483669958,256.007253286122,20.1213203435596)) ;
#96928=CARTESIAN_POINT('Ctrl Pts',(29.8999342879726,256.197254367133,20.1213203435596)) ;
#96929=CARTESIAN_POINT('Ctrl Pts',(29.9295469120274,256.267285941343,20.1213203435596)) ;
#96930=CARTESIAN_POINT('Ctrl Pts',(29.9544466269417,256.322163872416,20.1213203435596)) ;
#96931=CARTESIAN_POINT('Ctrl Pts',(29.981825823837,256.378579501238,20.1213203435596)) ;
#96932=CARTESIAN_POINT('Ctrl Pts',(30.030187806939,256.446752104601,20.1213203435596)) ;
#96933=CARTESIAN_POINT('Ctrl Pts',(30.0935892844406,256.495791347758,20.1213203435596)) ;
#96934=CARTESIAN_POINT('Ctrl Pts',(30.2113796608321,256.560201882538,20.1213203435596)) ;
#96935=CARTESIAN_POINT('Ctrl Pts',(30.3858069793213,256.614439322451,20.1213203435596)) ;
#96936=CARTESIAN_POINT('Ctrl Pts',(30.5388867945401,256.6452934669,20.1213203435596)) ;
#96937=CARTESIAN_POINT('Ctrl Pts',(30.6483865150998,256.663405993051,20.1213203435596)) ;
#96938=CARTESIAN_POINT('Ctrl Pts',(30.6812729811269,256.668845796667,20.1213203435596)) ;
#96939=CARTESIAN_POINT('Ctrl Pts',(30.7141594471539,256.674285600284,20.1213203435596)) ;
#96940=CARTESIAN_POINT('Ctrl Pts',(29.5759712687709,255.502885024398,20.1063603785425)) ;
#96941=CARTESIAN_POINT('Ctrl Pts',(29.6096896012297,255.570241420972,20.1063603785425)) ;
#96942=CARTESIAN_POINT('Ctrl Pts',(29.7111240387136,255.772053704706,20.1063603785425)) ;
#96943=CARTESIAN_POINT('Ctrl Pts',(29.8202483669958,256.007253286122,20.1063603785425)) ;
#96944=CARTESIAN_POINT('Ctrl Pts',(29.8999342879726,256.197254367133,20.1063603785425)) ;
#96945=CARTESIAN_POINT('Ctrl Pts',(29.9295469120274,256.267285941343,20.1063603785425)) ;
#96946=CARTESIAN_POINT('Ctrl Pts',(29.9544466269417,256.322163872416,20.1063603785425)) ;
#96947=CARTESIAN_POINT('Ctrl Pts',(29.981825823837,256.378579501238,20.1063603785425)) ;
#96948=CARTESIAN_POINT('Ctrl Pts',(30.030187806939,256.446752104601,20.1063603785425)) ;
#96949=CARTESIAN_POINT('Ctrl Pts',(30.0935892844406,256.495791347758,20.1063603785425)) ;
#96950=CARTESIAN_POINT('Ctrl Pts',(30.2113796608321,256.560201882538,20.1063603785425)) ;
#96951=CARTESIAN_POINT('Ctrl Pts',(30.3858069793213,256.614439322451,20.1063603785425)) ;
#96952=CARTESIAN_POINT('Ctrl Pts',(30.5388867945401,256.6452934669,20.1063603785425)) ;
#96953=CARTESIAN_POINT('Ctrl Pts',(30.6483865150998,256.663405993051,20.1063603785425)) ;
#96954=CARTESIAN_POINT('Ctrl Pts',(30.6812729811269,256.668845796667,20.1063603785425)) ;
#96955=CARTESIAN_POINT('Ctrl Pts',(30.7141594471539,256.674285600284,20.1063603785425)) ;
#96956=CARTESIAN_POINT('Ctrl Pts',(29.5820931728356,255.499820424641,20.0764990745067)) ;
#96957=CARTESIAN_POINT('Ctrl Pts',(29.6157879144431,255.567133304607,20.0764990745067)) ;
#96958=CARTESIAN_POINT('Ctrl Pts',(29.7171758868717,255.768968124513,20.0764990745067)) ;
#96959=CARTESIAN_POINT('Ctrl Pts',(29.8264197782412,256.004440884627,20.0764990745067)) ;
#96960=CARTESIAN_POINT('Ctrl Pts',(29.9060885809734,256.194470121105,20.0764990745067)) ;
#96961=CARTESIAN_POINT('Ctrl Pts',(29.9356887118595,256.264457942251,20.0764990745067)) ;
#96962=CARTESIAN_POINT('Ctrl Pts',(29.9605274326313,256.319158916676,20.0764990745067)) ;
#96963=CARTESIAN_POINT('Ctrl Pts',(29.9877640220894,256.375182355551,20.0764990745067)) ;
#96964=CARTESIAN_POINT('Ctrl Pts',(30.0351997933448,256.44195523641,20.0764990745067)) ;
#96965=CARTESIAN_POINT('Ctrl Pts',(30.09745915079,256.490158379369,20.0764990745067)) ;
#96966=CARTESIAN_POINT('Ctrl Pts',(30.2138634005463,256.553814059384,20.0764990745067)) ;
#96967=CARTESIAN_POINT('Ctrl Pts',(30.3874884736995,256.607807329319,20.0764990745067)) ;
#96968=CARTESIAN_POINT('Ctrl Pts',(30.5401558482827,256.638579125182,20.0764990745067)) ;
#96969=CARTESIAN_POINT('Ctrl Pts',(30.6495037630039,256.656651643477,20.0764990745067)) ;
#96970=CARTESIAN_POINT('Ctrl Pts',(30.6823902290309,256.662091447093,20.0764990745067)) ;
#96971=CARTESIAN_POINT('Ctrl Pts',(30.7152766950579,256.66753125071,20.0764990745067)) ;
#96972=CARTESIAN_POINT('Ctrl Pts',(29.6120092577916,255.484844556725,20.0344442939593)) ;
#96973=CARTESIAN_POINT('Ctrl Pts',(29.6457436600241,255.55223306503,20.0344442939593)) ;
#96974=CARTESIAN_POINT('Ctrl Pts',(29.7471844945767,255.754197572988,20.0344442939593)) ;
#96975=CARTESIAN_POINT('Ctrl Pts',(29.8570682054636,255.990988132927,20.0344442939593)) ;
#96976=CARTESIAN_POINT('Ctrl Pts',(29.9369263762561,256.181564104702,20.0344442939593)) ;
#96977=CARTESIAN_POINT('Ctrl Pts',(29.9664278986104,256.251202813136,20.0344442939593)) ;
#96978=CARTESIAN_POINT('Ctrl Pts',(29.9906663597142,256.304833928402,20.0344442939593)) ;
#96979=CARTESIAN_POINT('Ctrl Pts',(30.0172467190228,256.358916591612,20.0344442939593)) ;
#96980=CARTESIAN_POINT('Ctrl Pts',(30.0594700010607,256.41830695162,20.0344442939593)) ;
#96981=CARTESIAN_POINT('Ctrl Pts',(30.1154245125015,256.461746853186,20.0344442939593)) ;
#96982=CARTESIAN_POINT('Ctrl Pts',(30.2256762972524,256.522325166701,20.0344442939593)) ;
#96983=CARTESIAN_POINT('Ctrl Pts',(30.3954814694958,256.57530322983,20.0344442939593)) ;
#96984=CARTESIAN_POINT('Ctrl Pts',(30.5463544154014,256.605679815488,20.0344442939593)) ;
#96985=CARTESIAN_POINT('Ctrl Pts',(30.6549634505227,256.623644968832,20.0344442939593)) ;
#96986=CARTESIAN_POINT('Ctrl Pts',(30.6878499165497,256.629084772448,20.0344442939593)) ;
#96987=CARTESIAN_POINT('Ctrl Pts',(30.7207363825767,256.634524576065,20.0344442939593)) ;
#96988=CARTESIAN_POINT('Ctrl Pts',(29.6453265506804,255.46816605824,20.0213203435596)) ;
#96989=CARTESIAN_POINT('Ctrl Pts',(29.6790557391669,255.535546911685,20.0213203435596)) ;
#96990=CARTESIAN_POINT('Ctrl Pts',(29.7804662281711,255.737649617999,20.0213203435596)) ;
#96991=CARTESIAN_POINT('Ctrl Pts',(29.8910447966664,255.975913266732,20.0213203435596)) ;
#96992=CARTESIAN_POINT('Ctrl Pts',(29.9710268478646,256.16696772935,20.0213203435596)) ;
#96993=CARTESIAN_POINT('Ctrl Pts',(30.0004305211738,256.236260757865,20.0213203435596)) ;
#96994=CARTESIAN_POINT('Ctrl Pts',(30.0240967948258,256.288765755951,20.0213203435596)) ;
#96995=CARTESIAN_POINT('Ctrl Pts',(30.0499333589383,256.340694722479,20.0213203435596)) ;
#96996=CARTESIAN_POINT('Ctrl Pts',(30.0865702872101,256.392036123077,20.0213203435596)) ;
#96997=CARTESIAN_POINT('Ctrl Pts',(30.1357337756256,256.430387158868,20.0213203435596)) ;
#96998=CARTESIAN_POINT('Ctrl Pts',(30.2389356351689,256.487343368006,20.0213203435596)) ;
#96999=CARTESIAN_POINT('Ctrl Pts',(30.4044545988853,256.539134076114,20.0213203435596)) ;
#97000=CARTESIAN_POINT('Ctrl Pts',(30.5532586492272,256.569068223099,20.0213203435596)) ;
#97001=CARTESIAN_POINT('Ctrl Pts',(30.6610438587183,256.586885712129,20.0213203435597)) ;
#97002=CARTESIAN_POINT('Ctrl Pts',(30.6939303247453,256.592325515745,20.0213203435596)) ;
#97003=CARTESIAN_POINT('Ctrl Pts',(30.7268167907724,256.597765319362,20.0213203435596)) ;
#97004=CARTESIAN_POINT('Ctrl Pts',(29.6653926650914,255.458121044681,20.0213203435596)) ;
#97005=CARTESIAN_POINT('Ctrl Pts',(29.6991510606097,255.525557472002,20.0213203435596)) ;
#97006=CARTESIAN_POINT('Ctrl Pts',(29.8006017126181,255.727747494973,20.0213203435596)) ;
#97007=CARTESIAN_POINT('Ctrl Pts',(29.9116103717487,255.966894765232,20.0213203435596)) ;
#97008=CARTESIAN_POINT('Ctrl Pts',(29.9917240307883,256.158322827055,20.0213203435596)) ;
#97009=CARTESIAN_POINT('Ctrl Pts',(30.0210609313549,256.227379414746,20.0213203435596)) ;
#97010=CARTESIAN_POINT('Ctrl Pts',(30.0443195024724,256.279163360013,20.0213203435596)) ;
#97011=CARTESIAN_POINT('Ctrl Pts',(30.0697165858412,256.329790150052,20.0213203435596)) ;
#97012=CARTESIAN_POINT('Ctrl Pts',(30.102845715951,256.376170629923,20.0213203435596)) ;
#97013=CARTESIAN_POINT('Ctrl Pts',(30.1477680849333,256.411315348599,20.0213203435596)) ;
#97014=CARTESIAN_POINT('Ctrl Pts',(30.2468536416027,256.46621770294,20.0213203435596)) ;
#97015=CARTESIAN_POINT('Ctrl Pts',(30.4098121082759,256.517330456645,20.0213203435596)) ;
#97016=CARTESIAN_POINT('Ctrl Pts',(30.5574162678237,256.546999638827,20.0213203435596)) ;
#97017=CARTESIAN_POINT('Ctrl Pts',(30.6647059259495,256.564746594971,20.0213203435597)) ;
#97018=CARTESIAN_POINT('Ctrl Pts',(30.6975923919765,256.570186398587,20.0213203435596)) ;
#97019=CARTESIAN_POINT('Ctrl Pts',(30.7304788580035,256.575626202204,20.0213203435596)) ;
#97020=CARTESIAN_POINT('Ctrl Pts',(29.7113866401971,255.550077591566,20.0213203435596)) ;
#97021=CARTESIAN_POINT('Ctrl Pts',(29.7110571373176,255.549958798757,20.0213203435596)) ;
#97022=CARTESIAN_POINT('Ctrl Pts',(29.7107276113308,255.549840065814,20.0213212580779)) ;
#97023=CARTESIAN_POINT('Ctrl Pts',(29.694928578155,255.544150689885,20.0214088991967)) ;
#97024=CARTESIAN_POINT('Ctrl Pts',(29.6792649744873,255.538667136519,20.0235081059122)) ;
#97025=CARTESIAN_POINT('Ctrl Pts',(29.650188463837,255.528611542996,20.0314970318247)) ;
#97026=CARTESIAN_POINT('Ctrl Pts',(29.6363171942346,255.523870388381,20.0372432193757)) ;
#97027=CARTESIAN_POINT('Ctrl Pts',(29.6106557248686,255.514948318743,20.0533121285624)) ;
#97028=CARTESIAN_POINT('Ctrl Pts',(29.5997479208537,255.511139096753,20.0633496625201)) ;
#97029=CARTESIAN_POINT('Ctrl Pts',(29.5867225388609,255.506615978723,20.0815270572468)) ;
#97030=CARTESIAN_POINT('Ctrl Pts',(29.5827146684804,255.505215912772,20.08909649826)) ;
#97031=CARTESIAN_POINT('Ctrl Pts',(29.5773629195699,255.50335835714,20.1050033356937)) ;
#97032=CARTESIAN_POINT('Ctrl Pts',(29.5759712687709,255.502885024398,20.1130919745432)) ;
#97033=CARTESIAN_POINT('Ctrl Pts',(29.5759712687709,255.502885024398,20.1213203435596)) ;
#97034=CARTESIAN_POINT('Ctrl Pts',(30.7304788580025,256.575626202204,20.0213203435596)) ;
#97035=CARTESIAN_POINT('Ctrl Pts',(30.7301957245571,256.575824538007,20.0213203435596)) ;
#97036=CARTESIAN_POINT('Ctrl Pts',(30.7299126263369,256.576022926472,20.021321258476)) ;
#97037=CARTESIAN_POINT('Ctrl Pts',(30.7162932839813,256.585570725375,20.0214092548886)) ;
#97038=CARTESIAN_POINT('Ctrl Pts',(30.7029218650816,256.595123932586,20.0235245925657)) ;
#97039=CARTESIAN_POINT('Ctrl Pts',(30.6782054645625,256.612919481131,20.0315757241732)) ;
#97040=CARTESIAN_POINT('Ctrl Pts',(30.6664740137926,256.621427535467,20.0373664729568)) ;
#97041=CARTESIAN_POINT('Ctrl Pts',(30.6447342707739,256.637012105662,20.0535001884872)) ;
#97042=CARTESIAN_POINT('Ctrl Pts',(30.6355028892112,256.643611871642,20.0635480166157)) ;
#97043=CARTESIAN_POINT('Ctrl Pts',(30.6245226322433,256.6514906015,20.0817172500721)) ;
#97044=CARTESIAN_POINT('Ctrl Pts',(30.6211521485668,256.653899078661,20.0892580265995)) ;
#97045=CARTESIAN_POINT('Ctrl Pts',(30.6166589348149,256.657123518393,20.1050867998701)) ;
#97046=CARTESIAN_POINT('Ctrl Pts',(30.6155000490728,256.657966189434,20.1131378012872)) ;
#97047=CARTESIAN_POINT('Ctrl Pts',(30.6155000490728,256.657966189434,20.1213203435596)) ;
#97048=CARTESIAN_POINT('Origin',(43.2063774077619,249.25726004992,20.1213203435596)) ;
#97049=CARTESIAN_POINT('Origin',(30.2066640303894,255.319125951608,20.1213203435596)) ;
#97050=CARTESIAN_POINT('Origin',(28.3509795345864,248.977232647076,20.1213203435596)) ;
#97051=CARTESIAN_POINT('',(28.7971429244132,255.86605864576,20.1213203435596)) ;
#97052=CARTESIAN_POINT('Origin',(28.704724061155,256.019492061351,20.1213203435596)) ;
#97053=CARTESIAN_POINT('',(28.7065616828874,254.062789469896,20.1213203435596)) ;
#97054=CARTESIAN_POINT('',(28.4508536117473,248.972215804318,20.1213203435596)) ;
#97055=CARTESIAN_POINT('Origin',(28.594347661489,253.822145724429,20.1213203435596)) ;
#97056=CARTESIAN_POINT('Origin',(42.7981704029692,249.447610102367,20.1213203435596)) ;
#97057=CARTESIAN_POINT('',(42.7559085767951,249.356979323663,20.1213203435596)) ;
#97058=CARTESIAN_POINT('Ctrl Pts',(29.1672120667081,255.803830362557,20.0213203435596)) ;
#97059=CARTESIAN_POINT('Ctrl Pts',(29.1673235517997,255.803511486707,20.0213203435596)) ;
#97060=CARTESIAN_POINT('Ctrl Pts',(29.1674350651738,255.803192616964,20.0213212211779)) ;
#97061=CARTESIAN_POINT('Ctrl Pts',(29.172875934703,255.78763807154,20.02140682762)) ;
#97062=CARTESIAN_POINT('Ctrl Pts',(29.178235369087,255.772301108476,20.0234957973127)) ;
#97063=CARTESIAN_POINT('Ctrl Pts',(29.1881961388463,255.743729511578,20.0316145116046)) ;
#97064=CARTESIAN_POINT('Ctrl Pts',(29.1929424011081,255.730156724038,20.0375089738243)) ;
#97065=CARTESIAN_POINT('Ctrl Pts',(29.2020451864744,255.704209432607,20.0544007578192)) ;
#97066=CARTESIAN_POINT('Ctrl Pts',(29.2055656625208,255.69409678375,20.0647127777204)) ;
#97067=CARTESIAN_POINT('Ctrl Pts',(29.2097099600077,255.682260454704,20.0818702576819)) ;
#97068=CARTESIAN_POINT('Ctrl Pts',(29.2110458674259,255.678427653878,20.0893909150032)) ;
#97069=CARTESIAN_POINT('Ctrl Pts',(29.2128367240668,255.673316457768,20.105158929986)) ;
#97070=CARTESIAN_POINT('Ctrl Pts',(29.2133075051976,255.671997914687,20.1131782970793)) ;
#97071=CARTESIAN_POINT('Ctrl Pts',(29.2133075051976,255.671997914687,20.1213203435596)) ;
#97072=CARTESIAN_POINT('Origin',(32.5650931541241,257.50884617869,20.1213203435596)) ;
#97073=CARTESIAN_POINT('',(32.4970522102795,257.582129396146,20.1213203435596)) ;
#97074=CARTESIAN_POINT('Ctrl Pts',(30.6488818037555,257.068923192604,20.1213203435596)) ;
#97075=CARTESIAN_POINT('Ctrl Pts',(30.6159953377285,257.063483388987,20.1213203435596)) ;
#97076=CARTESIAN_POINT('Ctrl Pts',(30.5831088717014,257.058043585371,20.1213203435596)) ;
#97077=CARTESIAN_POINT('Ctrl Pts',(30.35235925836,257.019874918049,20.1213203435596)) ;
#97078=CARTESIAN_POINT('Ctrl Pts',(30.0562477831581,256.952359843337,20.1213203435596)) ;
#97079=CARTESIAN_POINT('Ctrl Pts',(29.7424371293616,256.748815981268,20.1213203435596)) ;
#97080=CARTESIAN_POINT('Ctrl Pts',(29.5940323940009,256.523626711091,20.1213203435596)) ;
#97081=CARTESIAN_POINT('Ctrl Pts',(29.493524415239,256.258021637289,20.1213203435596)) ;
#97082=CARTESIAN_POINT('Ctrl Pts',(29.3619731302367,255.972670333182,20.1213203435596)) ;
#97083=CARTESIAN_POINT('Ctrl Pts',(29.2709280858246,255.787069709302,20.1213203435596)) ;
#97084=CARTESIAN_POINT('Ctrl Pts',(29.2133075051975,255.671997914687,20.1213203435596)) ;
#97085=CARTESIAN_POINT('Ctrl Pts',(30.6488818037555,257.068923192604,20.1063603785425)) ;
#97086=CARTESIAN_POINT('Ctrl Pts',(30.6159953377285,257.063483388987,20.1063603785425)) ;
#97087=CARTESIAN_POINT('Ctrl Pts',(30.5831088717014,257.058043585371,20.1063603785425)) ;
#97088=CARTESIAN_POINT('Ctrl Pts',(30.35235925836,257.019874918049,20.1063603785425)) ;
#97089=CARTESIAN_POINT('Ctrl Pts',(30.0562477831581,256.952359843337,20.1063603785425)) ;
#97090=CARTESIAN_POINT('Ctrl Pts',(29.7424371293616,256.748815981268,20.1063603785425)) ;
#97091=CARTESIAN_POINT('Ctrl Pts',(29.5940323940009,256.523626711091,20.1063603785425)) ;
#97092=CARTESIAN_POINT('Ctrl Pts',(29.493524415239,256.258021637289,20.1063603785425)) ;
#97093=CARTESIAN_POINT('Ctrl Pts',(29.3619731302367,255.972670333182,20.1063603785425)) ;
#97094=CARTESIAN_POINT('Ctrl Pts',(29.2709280858246,255.787069709302,20.1063603785425)) ;
#97095=CARTESIAN_POINT('Ctrl Pts',(29.2133075051975,255.671997914687,20.1063603785425)) ;
#97096=CARTESIAN_POINT('Ctrl Pts',(30.6479033156902,257.074838666173,20.0802089331821)) ;
#97097=CARTESIAN_POINT('Ctrl Pts',(30.6150168496632,257.069398862557,20.0802089331821)) ;
#97098=CARTESIAN_POINT('Ctrl Pts',(30.5821303836361,257.06395905894,20.0802089331821)) ;
#97099=CARTESIAN_POINT('Ctrl Pts',(30.3513532542168,257.026024900111,20.0802089331821)) ;
#97100=CARTESIAN_POINT('Ctrl Pts',(30.0541250166344,256.958485975665,20.0802089331821)) ;
#97101=CARTESIAN_POINT('Ctrl Pts',(29.7381084482561,256.753746292952,20.0802089331821)) ;
#97102=CARTESIAN_POINT('Ctrl Pts',(29.5884325466772,256.526156268995,20.0802089331821)) ;
#97103=CARTESIAN_POINT('Ctrl Pts',(29.4880187414454,256.260571687147,20.0802089331821)) ;
#97104=CARTESIAN_POINT('Ctrl Pts',(29.3567315627788,255.975220870925,20.0802089331821)) ;
#97105=CARTESIAN_POINT('Ctrl Pts',(29.2652966109379,255.79035111116,20.0802089331821)) ;
#97106=CARTESIAN_POINT('Ctrl Pts',(29.2079462293641,255.674682498059,20.0802089331821)) ;
#97107=CARTESIAN_POINT('Ctrl Pts',(30.6439632681149,257.098658320313,20.046158428686)) ;
#97108=CARTESIAN_POINT('Ctrl Pts',(30.6110768020878,257.093218516696,20.046158428686)) ;
#97109=CARTESIAN_POINT('Ctrl Pts',(30.5781903360608,257.087778713079,20.046158428686)) ;
#97110=CARTESIAN_POINT('Ctrl Pts',(30.346034219779,257.049493628584,20.046158428686)) ;
#97111=CARTESIAN_POINT('Ctrl Pts',(30.0466036859445,256.982025168442,20.046158428686)) ;
#97112=CARTESIAN_POINT('Ctrl Pts',(29.7209071767827,256.771897391692,20.046158428686)) ;
#97113=CARTESIAN_POINT('Ctrl Pts',(29.5657738058475,256.535373232231,20.046158428686)) ;
#97114=CARTESIAN_POINT('Ctrl Pts',(29.4658953017976,256.269858985514,20.046158428686)) ;
#97115=CARTESIAN_POINT('Ctrl Pts',(29.3348931712675,255.985906642723,20.046158428686)) ;
#97116=CARTESIAN_POINT('Ctrl Pts',(29.2438344960392,255.800828730593,20.046158428686)) ;
#97117=CARTESIAN_POINT('Ctrl Pts',(29.1863581460773,255.685492426746,20.046158428686)) ;
#97118=CARTESIAN_POINT('Ctrl Pts',(30.6397271501173,257.124267875443,20.0298289990098)) ;
#97119=CARTESIAN_POINT('Ctrl Pts',(30.6068406840902,257.118828071826,20.0298289990098)) ;
#97120=CARTESIAN_POINT('Ctrl Pts',(30.5739542180632,257.113388268209,20.0298289990098)) ;
#97121=CARTESIAN_POINT('Ctrl Pts',(30.3405240702817,257.074938910687,20.0298289990098)) ;
#97122=CARTESIAN_POINT('Ctrl Pts',(30.0383483709799,257.007518825832,20.0298289990098)) ;
#97123=CARTESIAN_POINT('Ctrl Pts',(29.7023756891282,256.791692300423,20.0298289990098)) ;
#97124=CARTESIAN_POINT('Ctrl Pts',(29.5414304926382,256.545442119708,20.0298289990098)) ;
#97125=CARTESIAN_POINT('Ctrl Pts',(29.4421018414893,256.280005496473,20.0298289990098)) ;
#97126=CARTESIAN_POINT('Ctrl Pts',(29.3115342048088,255.997327031355,20.0298289990098)) ;
#97127=CARTESIAN_POINT('Ctrl Pts',(29.2205599742109,255.812543583895,20.0298289990098)) ;
#97128=CARTESIAN_POINT('Ctrl Pts',(29.1631478506694,255.697114655307,20.0298289990098)) ;
#97129=CARTESIAN_POINT('Ctrl Pts',(30.636200901783,257.145585896132,20.0236265255013)) ;
#97130=CARTESIAN_POINT('Ctrl Pts',(30.603314435756,257.140146092516,20.0236265255013)) ;
#97131=CARTESIAN_POINT('Ctrl Pts',(30.5704279697289,257.134706288899,20.0236265255013)) ;
#97132=CARTESIAN_POINT('Ctrl Pts',(30.3357835140935,257.095963136756,20.0236265255013)) ;
#97133=CARTESIAN_POINT('Ctrl Pts',(30.0316008933358,257.028603509364,20.0236265255013)) ;
#97134=CARTESIAN_POINT('Ctrl Pts',(29.6869773794647,256.807963737247,20.0236265255013)) ;
#97135=CARTESIAN_POINT('Ctrl Pts',(29.5211531836893,256.553706245957,20.0236265255013)) ;
#97136=CARTESIAN_POINT('Ctrl Pts',(29.4223011707526,256.288332761635,20.0236265255013)) ;
#97137=CARTESIAN_POINT('Ctrl Pts',(29.2920008308411,256.006884035643,20.0236265255013)) ;
#97138=CARTESIAN_POINT('Ctrl Pts',(29.2013328910854,255.821963624557,20.0236265255013)) ;
#97139=CARTESIAN_POINT('Ctrl Pts',(29.1438270325134,255.706789282908,20.0236265255013)) ;
#97140=CARTESIAN_POINT('Ctrl Pts',(30.6343935863363,257.156512065941,20.0217377892707)) ;
#97141=CARTESIAN_POINT('Ctrl Pts',(30.6015071203092,257.151072262324,20.0217377892707)) ;
#97142=CARTESIAN_POINT('Ctrl Pts',(30.5686206542822,257.145632458708,20.0217377892707)) ;
#97143=CARTESIAN_POINT('Ctrl Pts',(30.3333675899215,257.106752783705,20.0217377892707)) ;
#97144=CARTESIAN_POINT('Ctrl Pts',(30.0281314560414,257.039422335769,20.0217377892707)) ;
#97145=CARTESIAN_POINT('Ctrl Pts',(29.6790827674713,256.816321837849,20.0217377892707)) ;
#97146=CARTESIAN_POINT('Ctrl Pts',(29.510761605924,256.557952389036,20.0217377892707)) ;
#97147=CARTESIAN_POINT('Ctrl Pts',(29.4121521913412,256.292611397608,20.0217377892707)) ;
#97148=CARTESIAN_POINT('Ctrl Pts',(29.2819972974163,256.011777796768,20.0217377892707)) ;
#97149=CARTESIAN_POINT('Ctrl Pts',(29.191465219267,255.826821384756,20.0217377892707)) ;
#97150=CARTESIAN_POINT('Ctrl Pts',(29.1339244931038,255.711747840063,20.0217377892707)) ;
#97151=CARTESIAN_POINT('Ctrl Pts',(30.6331727374444,257.163892737824,20.0213203435597)) ;
#97152=CARTESIAN_POINT('Ctrl Pts',(30.6002862714174,257.158452934208,20.0213203435597)) ;
#97153=CARTESIAN_POINT('Ctrl Pts',(30.5673998053903,257.153013130591,20.0213203435597)) ;
#97154=CARTESIAN_POINT('Ctrl Pts',(30.3317495219155,257.114055428562,20.0213203435596)) ;
#97155=CARTESIAN_POINT('Ctrl Pts',(30.0257765890063,257.04674286674,20.0213203435596)) ;
#97156=CARTESIAN_POINT('Ctrl Pts',(29.6737474166104,256.821986417431,20.0213203435596)) ;
#97157=CARTESIAN_POINT('Ctrl Pts',(29.5037432587571,256.560831292509,20.0213203435596)) ;
#97158=CARTESIAN_POINT('Ctrl Pts',(29.4052960096356,256.295512383638,20.0213203435596)) ;
#97159=CARTESIAN_POINT('Ctrl Pts',(29.2752478960571,256.015078997478,20.0213203435596)) ;
#97160=CARTESIAN_POINT('Ctrl Pts',(29.1847862627121,255.830132800747,20.0213203435596)) ;
#97161=CARTESIAN_POINT('Ctrl Pts',(29.1272352876938,255.715097365469,20.0213203435596)) ;
#97162=CARTESIAN_POINT('Ctrl Pts',(30.6325623929059,257.167582590684,20.0213203435597)) ;
#97163=CARTESIAN_POINT('Ctrl Pts',(30.5996759268789,257.162142787068,20.0213203435597)) ;
#97164=CARTESIAN_POINT('Ctrl Pts',(30.5667894608518,257.156702983451,20.0213203435597)) ;
#97165=CARTESIAN_POINT('Ctrl Pts',(30.3309225628221,257.117687857779,20.0213203435596)) ;
#97166=CARTESIAN_POINT('Ctrl Pts',(30.0246139021395,257.050386605117,20.0213203435596)) ;
#97167=CARTESIAN_POINT('Ctrl Pts',(29.6710833447946,256.82479414277,20.0213203435596)) ;
#97168=CARTESIAN_POINT('Ctrl Pts',(29.5002329804407,256.562256782507,20.0213203435596)) ;
#97169=CARTESIAN_POINT('Ctrl Pts',(29.4018690227886,256.296948740307,20.0213203435596)) ;
#97170=CARTESIAN_POINT('Ctrl Pts',(29.2718632248773,256.016735290733,20.0213203435596)) ;
#97171=CARTESIAN_POINT('Ctrl Pts',(29.1814644817151,255.831749398905,20.0213203435596)) ;
#97172=CARTESIAN_POINT('Ctrl Pts',(29.1238911228127,255.716771908939,20.0213203435596)) ;
#97173=CARTESIAN_POINT('Ctrl Pts',(30.6325623929049,257.167582590684,20.0213203435597)) ;
#97174=CARTESIAN_POINT('Ctrl Pts',(30.632363372354,257.167303914202,20.0213203435597)) ;
#97175=CARTESIAN_POINT('Ctrl Pts',(30.6321643395558,257.167025244098,20.0213212207922)) ;
#97176=CARTESIAN_POINT('Ctrl Pts',(30.6224905315818,257.153481996673,20.0214065029112)) ;
#97177=CARTESIAN_POINT('Ctrl Pts',(30.6129575908717,257.140181501842,20.0234788659747)) ;
#97178=CARTESIAN_POINT('Ctrl Pts',(30.5951908320103,257.115407134294,20.0315134132315)) ;
#97179=CARTESIAN_POINT('Ctrl Pts',(30.5867361809595,257.103625687996,20.0373513069104)) ;
#97180=CARTESIAN_POINT('Ctrl Pts',(30.5706299595814,257.081105304138,20.0540392142044)) ;
#97181=CARTESIAN_POINT('Ctrl Pts',(30.5642378623769,257.072204164288,20.0642748433054)) ;
#97182=CARTESIAN_POINT('Ctrl Pts',(30.5567091101513,257.061696581791,20.081623449277)) ;
#97183=CARTESIAN_POINT('Ctrl Pts',(30.5542798478843,257.058313743444,20.0891865612042)) ;
#97184=CARTESIAN_POINT('Ctrl Pts',(30.5510510049725,257.053787395618,20.1050494520494)) ;
#97185=CARTESIAN_POINT('Ctrl Pts',(30.550222414244,257.052603729947,20.1131190766524)) ;
#97186=CARTESIAN_POINT('Ctrl Pts',(30.550222414244,257.052603729947,20.1213203435596)) ;
#97187=CARTESIAN_POINT('Origin',(32.3250488694829,246.935614134431,20.1213203435596)) ;
#97188=CARTESIAN_POINT('Origin',(28.7065616828874,254.062789469896,20.0213203435596)) ;
#97189=CARTESIAN_POINT('',(28.7065616828874,254.062789469896,20.0213203435596)) ;
#97190=CARTESIAN_POINT('Origin',(28.7971429244132,255.86605864576,20.0213203435596)) ;
#97191=CARTESIAN_POINT('',(28.7971429244132,255.86605864576,20.0213203435596)) ;
#97192=CARTESIAN_POINT('Origin',(58.2408539117876,252.51941903599,20.1213203435596)) ;
#97193=CARTESIAN_POINT('',(66.856524993511,256.02214694455,20.0213203435596)) ;
#97194=CARTESIAN_POINT('',(64.8184058153773,255.19354324572,20.0213203435596)) ;
#97195=CARTESIAN_POINT('',(58.2408539117876,252.51941903599,20.0213203435596)) ;
#97196=CARTESIAN_POINT('Origin',(64.8184058153773,255.19354324572,20.1213203435596)) ;
#97197=CARTESIAN_POINT('',(66.5910039984262,256.02214694455,20.1213203435596)) ;
#97198=CARTESIAN_POINT('',(58.2031921065628,252.61205589921,20.1213203435596)) ;
#97199=CARTESIAN_POINT('Origin',(66.856524993511,256.02214694455,20.1213203435596)) ;
#97200=CARTESIAN_POINT('Origin',(64.4170577015585,257.013919968902,20.1213203435596)) ;
#97201=CARTESIAN_POINT('',(64.9184058153773,256.70214694455,20.1213203435596)) ;
#97202=CARTESIAN_POINT('',(64.3793958963336,256.921283105682,20.1213203435596)) ;
#97203=CARTESIAN_POINT('',(64.8184058153773,256.85075064338,20.0213203435596)) ;
#97204=CARTESIAN_POINT('Origin',(64.8184058153773,256.85075064338,20.1213203435596)) ;
#97205=CARTESIAN_POINT('',(64.4170577015585,257.013919968902,20.0213203435596)) ;
#97206=CARTESIAN_POINT('Origin',(64.8184058153773,248.269379137783,20.1213203435596)) ;
#97207=CARTESIAN_POINT('',(64.8184058153773,255.72214694455,20.0213203435596)) ;
#97208=CARTESIAN_POINT('',(64.8184058153773,248.269379137783,20.0213203435596)) ;
#97209=CARTESIAN_POINT('Origin',(64.8184058153773,255.72214694455,20.1213203435596)) ;
#97210=CARTESIAN_POINT('Origin',(59.2625927064781,255.72214694455,20.1213203435596)) ;
#97211=CARTESIAN_POINT('',(63.2110039984262,255.72214694455,20.0213203435596)) ;
#97212=CARTESIAN_POINT('',(59.2625927064781,255.72214694455,20.0213203435596)) ;
#97213=CARTESIAN_POINT('Origin',(63.2110039984262,255.72214694455,20.1213203435596)) ;
#97214=CARTESIAN_POINT('Origin',(63.2110039984262,248.469379137783,20.1213203435596)) ;
#97215=CARTESIAN_POINT('',(63.2110039984262,256.32214694455,20.0213203435596)) ;
#97216=CARTESIAN_POINT('',(63.2110039984262,248.469379137783,20.0213203435596)) ;
#97217=CARTESIAN_POINT('Origin',(63.2110039984262,256.32214694455,20.1213203435596)) ;
#97218=CARTESIAN_POINT('Origin',(60.0662936149535,256.32214694455,20.1213203435596)) ;
#97219=CARTESIAN_POINT('',(64.8184058153773,256.32214694455,20.0213203435596)) ;
#97220=CARTESIAN_POINT('',(60.0662936149535,256.32214694455,20.0213203435596)) ;
#97221=CARTESIAN_POINT('Origin',(64.8184058153773,256.32214694455,20.1213203435596)) ;
#97222=CARTESIAN_POINT('Origin',(64.8184058153773,248.709379137783,20.1213203435596)) ;
#97223=CARTESIAN_POINT('',(64.9184058153773,248.709379137783,20.1213203435596)) ;
#97224=CARTESIAN_POINT('',(64.8184058153773,248.709379137783,20.0213203435596)) ;
#97225=CARTESIAN_POINT('Origin',(64.9184058153773,256.70214694455,20.0213203435596)) ;
#97226=CARTESIAN_POINT('',(64.9184058153773,256.70214694455,20.0213203435596)) ;
#97227=CARTESIAN_POINT('Origin',(66.5910039984262,256.02214694455,20.0213203435596)) ;
#97228=CARTESIAN_POINT('',(66.5910039984262,256.02214694455,20.0213203435596)) ;
#97229=CARTESIAN_POINT('Origin',(64.9184058153773,255.34214694455,20.0213203435596)) ;
#97230=CARTESIAN_POINT('Origin',(55.2141814145299,240.716611331017,20.0213203435596)) ;
#97231=CARTESIAN_POINT('',(68.6350889359327,257.,20.0213203435596)) ;
#97232=CARTESIAN_POINT('',(68.6350889359328,261.466666666667,20.0213203435596)) ;
#97233=CARTESIAN_POINT('',(68.6350889359325,252.258305665508,20.0213203435596)) ;
#97234=CARTESIAN_POINT('',(68.65,256.631336165532,20.0213203435596)) ;
#97235=CARTESIAN_POINT('Origin',(73.2,257.,20.0213203435596)) ;
#97236=CARTESIAN_POINT('',(68.65,255.5,20.0213203435596)) ;
#97237=CARTESIAN_POINT('',(68.65,248.108305665508,20.0213203435596)) ;
#97238=CARTESIAN_POINT('Origin',(73.2,255.5,20.0213203435596)) ;
#97239=CARTESIAN_POINT('',(55.75,255.5,20.0213203435596)) ;
#97240=CARTESIAN_POINT('Origin',(51.2,255.5,20.0213203435596)) ;
#97241=CARTESIAN_POINT('',(55.75,256.631336165532,20.0213203435596)) ;
#97242=CARTESIAN_POINT('',(55.75,248.684378986433,20.0213203435596)) ;
#97243=CARTESIAN_POINT('',(55.7649110640674,257.,20.0213203435596)) ;
#97244=CARTESIAN_POINT('Origin',(51.2,257.,20.0213203435596)) ;
#97245=CARTESIAN_POINT('',(55.7649110640674,248.858305665508,20.0213203435596)) ;
#97246=CARTESIAN_POINT('',(56.2695111541429,261.559687576257,20.0213203435596)) ;
#97247=CARTESIAN_POINT('Ctrl Pts',(56.2695111541429,261.559687576257,20.0213203435596)) ;
#97248=CARTESIAN_POINT('Ctrl Pts',(56.2620293235127,261.559687576257,20.0213203435596)) ;
#97249=CARTESIAN_POINT('Ctrl Pts',(56.2545427899591,261.559686365099,20.0213203435619)) ;
#97250=CARTESIAN_POINT('Ctrl Pts',(56.2469607049508,261.559621906612,20.0213203435607)) ;
#97251=CARTESIAN_POINT('Ctrl Pts',(56.2429395471374,261.559587721062,20.02132034356)) ;
#97252=CARTESIAN_POINT('Ctrl Pts',(56.2388941346124,261.559536451947,20.0213203435599)) ;
#97253=CARTESIAN_POINT('Ctrl Pts',(56.2348134639309,261.559459472082,20.0213203435598)) ;
#97254=CARTESIAN_POINT('Ctrl Pts',(56.2307620197578,261.559383043561,20.0213203435597)) ;
#97255=CARTESIAN_POINT('Ctrl Pts',(56.2266758214071,261.559281270923,20.0213203435597)) ;
#97256=CARTESIAN_POINT('Ctrl Pts',(56.2225540991302,261.559148465343,20.0213203435599)) ;
#97257=CARTESIAN_POINT('Ctrl Pts',(56.2136298089806,261.55886091673,20.0213203435605)) ;
#97258=CARTESIAN_POINT('Ctrl Pts',(56.2045275984428,261.558424861714,20.0213203435596)) ;
#97259=CARTESIAN_POINT('Ctrl Pts',(56.1952509539508,261.557785784382,20.0213203435596)) ;
#97260=CARTESIAN_POINT('Ctrl Pts',(56.184797181305,261.557065613512,20.0213203435597)) ;
#97261=CARTESIAN_POINT('Ctrl Pts',(56.1741226379547,261.55608811322,20.0213203435597)) ;
#97262=CARTESIAN_POINT('Ctrl Pts',(56.1632977864506,261.554797675761,20.0213203435596)) ;
#97263=CARTESIAN_POINT('Ctrl Pts',(56.1471254853081,261.552869765418,20.0213203435596)) ;
#97264=CARTESIAN_POINT('Ctrl Pts',(56.1306227005856,261.550241630897,20.0213203435595)) ;
#97265=CARTESIAN_POINT('Ctrl Pts',(56.1141385164753,261.546788423019,20.0213203435597)) ;
#97266=CARTESIAN_POINT('Ctrl Pts',(56.1033359290827,261.544525430829,20.0213203435598)) ;
#97267=CARTESIAN_POINT('Ctrl Pts',(56.0925439545573,261.541909763607,20.0213203435596)) ;
#97268=CARTESIAN_POINT('Ctrl Pts',(56.0818401088614,261.538912650206,20.0213203435596)) ;
#97269=CARTESIAN_POINT('Ctrl Pts',(56.0716896860479,261.536070497106,20.0213203435596)) ;
#97270=CARTESIAN_POINT('Ctrl Pts',(56.0616200212418,261.532885652269,20.02132034356)) ;
#97271=CARTESIAN_POINT('Ctrl Pts',(56.051650953882,261.52933162481,20.0213203435597)) ;
#97272=CARTESIAN_POINT('Ctrl Pts',(56.048894385141,261.528348892861,20.0213203435597)) ;
#97273=CARTESIAN_POINT('Ctrl Pts',(56.0461448965502,261.527337901265,20.0213203435597)) ;
#97274=CARTESIAN_POINT('Ctrl Pts',(56.0434023233072,261.526297906278,20.0213203435596)) ;
#97275=CARTESIAN_POINT('Ctrl Pts',(56.0358527224709,261.523435066775,20.0213203435596)) ;
#97276=CARTESIAN_POINT('Ctrl Pts',(56.0283554905343,261.52035255579,20.0213203435597)) ;
#97277=CARTESIAN_POINT('Ctrl Pts',(56.0209014644149,261.517041751319,20.0213203435596)) ;
#97278=CARTESIAN_POINT('Ctrl Pts',(56.0157914271727,261.514772060567,20.0213203435596)) ;
#97279=CARTESIAN_POINT('Ctrl Pts',(56.0107040385674,261.512396296763,20.0213203435596)) ;
#97280=CARTESIAN_POINT('Ctrl Pts',(56.0056387442236,261.509913017798,20.0213203435596)) ;
#97281=CARTESIAN_POINT('Ctrl Pts',(56.0005924317678,261.507439044772,20.0213203435596)) ;
#97282=CARTESIAN_POINT('Ctrl Pts',(55.995568049491,261.504858361603,20.0213203435597)) ;
#97283=CARTESIAN_POINT('Ctrl Pts',(55.9905731854363,261.502174888351,20.0213203435597)) ;
#97284=CARTESIAN_POINT('Ctrl Pts',(55.9832419391146,261.498236201893,20.0213203435597)) ;
#97285=CARTESIAN_POINT('Ctrl Pts',(55.9759714235957,261.49407441593,20.0213203435596)) ;
#97286=CARTESIAN_POINT('Ctrl Pts',(55.9687841103927,261.489701274464,20.0213203435596)) ;
#97287=CARTESIAN_POINT('Ctrl Pts',(55.9642788487677,261.486960035023,20.0213203435596)) ;
#97288=CARTESIAN_POINT('Ctrl Pts',(55.9598062775265,261.484135753404,20.0213203435596)) ;
#97289=CARTESIAN_POINT('Ctrl Pts',(55.9553742025499,261.481233192763,20.0213203435596)) ;
#97290=CARTESIAN_POINT('Ctrl Pts',(55.947918042932,261.47635016268,20.0213203435596)) ;
#97291=CARTESIAN_POINT('Ctrl Pts',(55.9405757308991,261.471244857424,20.0213203435596)) ;
#97292=CARTESIAN_POINT('Ctrl Pts',(55.933384073417,261.465939267956,20.0213203435596)) ;
#97293=CARTESIAN_POINT('Ctrl Pts',(55.9219179108755,261.45748019557,20.0213203435596)) ;
#97294=CARTESIAN_POINT('Ctrl Pts',(55.9108347324416,261.44851198663,20.0213203435596)) ;
#97295=CARTESIAN_POINT('Ctrl Pts',(55.9002853073786,261.439128427997,20.0213203435596)) ;
#97296=CARTESIAN_POINT('',(68.6263598493594,261.559687576257,20.0213203435596)) ;
#97297=CARTESIAN_POINT('',(55.2268638269143,261.559687576257,20.0213203435596)) ;
#97298=CARTESIAN_POINT('Origin',(68.1350889359328,261.466666666667,20.0213203435596)) ;
#97299=CARTESIAN_POINT('',(63.,254.92214694455,20.0213203435596)) ;
#97300=CARTESIAN_POINT('',(62.4,254.92214694455,20.0213203435596)) ;
#97301=CARTESIAN_POINT('',(58.8570907072643,254.92214694455,20.0213203435596)) ;
#97302=CARTESIAN_POINT('',(63.,257.12214694455,20.0213203435596)) ;
#97303=CARTESIAN_POINT('',(63.,247.869379137783,20.0213203435596)) ;
#97304=CARTESIAN_POINT('',(62.4,257.12214694455,20.0213203435596)) ;
#97305=CARTESIAN_POINT('',(59.057090707265,257.12214694455,20.0213203435596)) ;
#97306=CARTESIAN_POINT('',(62.4,248.869379137783,20.0213203435596)) ;
#97307=CARTESIAN_POINT('',(62.1889960015738,256.32214694455,20.0213203435596)) ;
#97308=CARTESIAN_POINT('',(62.1889960015738,255.72214694455,20.0213203435596)) ;
#97309=CARTESIAN_POINT('',(62.188996001574,248.269379137783,20.0213203435596)) ;
#97310=CARTESIAN_POINT('',(60.5815941846227,256.32214694455,20.0213203435596)) ;
#97311=CARTESIAN_POINT('',(58.651588708052,256.32214694455,20.0213203435596)) ;
#97312=CARTESIAN_POINT('',(60.5815941846227,256.85075064338,20.0213203435596)) ;
#97313=CARTESIAN_POINT('',(60.5815941846227,248.469379137783,20.0213203435596)) ;
#97314=CARTESIAN_POINT('',(58.5434750064891,256.02214694455,20.0213203435596)) ;
#97315=CARTESIAN_POINT('',(55.3952199758442,254.742214057778,20.0213203435596)) ;
#97316=CARTESIAN_POINT('',(60.5815941846227,255.19354324572,20.0213203435596)) ;
#97317=CARTESIAN_POINT('',(59.8988255825664,255.471124947113,20.0213203435596)) ;
#97318=CARTESIAN_POINT('',(60.5815941846227,255.72214694455,20.0213203435596)) ;
#97319=CARTESIAN_POINT('',(60.5815941846227,248.029379137783,20.0213203435596)) ;
#97320=CARTESIAN_POINT('',(57.8478877995763,255.72214694455,20.0213203435596)) ;
#97321=CARTESIAN_POINT('Origin',(58.8570907072643,254.92214694455,20.1213203435596)) ;
#97322=CARTESIAN_POINT('Origin',(62.4,254.92214694455,20.1213203435596)) ;
#97323=CARTESIAN_POINT('Origin',(63.,254.92214694455,20.1213203435596)) ;
#97324=CARTESIAN_POINT('Origin',(62.4,248.869379137783,20.1213203435596)) ;
#97325=CARTESIAN_POINT('Origin',(62.4,257.12214694455,20.1213203435596)) ;
#97326=CARTESIAN_POINT('Origin',(59.057090707265,257.12214694455,20.1213203435596)) ;
#97327=CARTESIAN_POINT('',(62.9,257.02214694455,20.1213203435596)) ;
#97328=CARTESIAN_POINT('',(59.057090707265,257.02214694455,20.1213203435596)) ;
#97329=CARTESIAN_POINT('Origin',(63.,257.12214694455,20.1213203435596)) ;
#97330=CARTESIAN_POINT('Origin',(63.,247.869379137783,20.1213203435596)) ;
#97331=CARTESIAN_POINT('',(62.9,247.869379137783,20.1213203435596)) ;
#97332=CARTESIAN_POINT('Origin',(62.9,255.02214694455,20.0213203435596)) ;
#97333=CARTESIAN_POINT('',(62.9,257.02214694455,20.0213203435596)) ;
#97334=CARTESIAN_POINT('Origin',(62.188996001574,248.269379137783,20.1213203435596)) ;
#97335=CARTESIAN_POINT('',(62.0889960015738,255.82214694455,20.1213203435596)) ;
#97336=CARTESIAN_POINT('Origin',(62.1889960015738,255.72214694455,20.1213203435596)) ;
#97337=CARTESIAN_POINT('',(62.0889960015738,256.22214694455,20.1213203435596)) ;
#97338=CARTESIAN_POINT('',(62.088996001574,248.269379137783,20.1213203435596)) ;
#97339=CARTESIAN_POINT('Origin',(62.1889960015738,256.32214694455,20.1213203435596)) ;
#97340=CARTESIAN_POINT('Origin',(57.8478877995763,255.72214694455,20.1213203435596)) ;
#97341=CARTESIAN_POINT('Origin',(60.5815941846227,255.72214694455,20.1213203435596)) ;
#97342=CARTESIAN_POINT('',(57.8478877995763,255.82214694455,20.1213203435596)) ;
#97343=CARTESIAN_POINT('Origin',(60.5815941846227,248.029379137783,20.1213203435596)) ;
#97344=CARTESIAN_POINT('Origin',(60.5815941846227,255.19354324572,20.1213203435596)) ;
#97345=CARTESIAN_POINT('Origin',(59.8988255825664,255.471124947113,20.1213203435596)) ;
#97346=CARTESIAN_POINT('Origin',(58.5434750064891,256.02214694455,20.1213203435596)) ;
#97347=CARTESIAN_POINT('Origin',(55.3952199758442,254.742214057778,20.1213203435596)) ;
#97348=CARTESIAN_POINT('Origin',(60.5815941846227,256.85075064338,20.1213203435596)) ;
#97349=CARTESIAN_POINT('Origin',(60.5815941846227,248.469379137783,20.1213203435596)) ;
#97350=CARTESIAN_POINT('Origin',(60.5815941846227,256.32214694455,20.1213203435596)) ;
#97351=CARTESIAN_POINT('Origin',(58.651588708052,256.32214694455,20.1213203435596)) ;
#97352=CARTESIAN_POINT('',(58.651588708052,256.22214694455,20.1213203435596)) ;
#97353=CARTESIAN_POINT('Origin',(62.0889960015738,256.22214694455,20.0213203435596)) ;
#97354=CARTESIAN_POINT('',(62.0889960015738,256.22214694455,20.0213203435596)) ;
#97355=CARTESIAN_POINT('Origin',(62.0889960015738,255.82214694455,20.0213203435596)) ;
#97356=CARTESIAN_POINT('',(62.0889960015738,255.82214694455,20.0213203435596)) ;
#97357=CARTESIAN_POINT('Origin',(64.9712721217948,249.52834685842,18.1213203435596)) ;
#97358=CARTESIAN_POINT('Origin',(74.8283628290596,249.52834685842,18.1213203435596)) ;
#97359=CARTESIAN_POINT('Origin',(74.2283628290596,249.52834685842,18.1213203435596)) ;
#97360=CARTESIAN_POINT('Origin',(74.8283628290596,247.98917342921,18.1213203435596)) ;
#97361=CARTESIAN_POINT('',(74.7283628290596,246.92834685842,18.1213203435596)) ;
#97362=CARTESIAN_POINT('Origin',(74.8283628290596,246.82834685842,18.1213203435596)) ;
#97363=CARTESIAN_POINT('',(74.7283628290596,247.98917342921,18.1213203435596)) ;
#97364=CARTESIAN_POINT('Origin',(74.2283628290596,249.23917342921,18.1213203435596)) ;
#97365=CARTESIAN_POINT('Origin',(74.2283628290596,246.82834685842,18.1213203435596)) ;
#97366=CARTESIAN_POINT('Origin',(64.7712721217948,246.82834685842,18.1213203435596)) ;
#97367=CARTESIAN_POINT('',(64.7712721217948,246.92834685842,18.1213203435596)) ;
#97368=CARTESIAN_POINT('Origin',(77.0348658990794,248.670975591968,18.1213203435596)) ;
#97369=CARTESIAN_POINT('',(76.9348658990794,248.291951183936,18.1213203435596)) ;
#97370=CARTESIAN_POINT('',(76.9348658990794,249.302824616567,18.1213203435596)) ;
#97371=CARTESIAN_POINT('',(76.9348658990794,248.670975591968,18.1213203435596)) ;
#97372=CARTESIAN_POINT('Origin',(77.0348658990794,249.302824616567,18.1213203435596)) ;
#97373=CARTESIAN_POINT('Origin',(77.0348658990794,248.391951183936,18.1213203435596)) ;
#97374=CARTESIAN_POINT('Origin',(66.3218485782223,248.391951183936,18.1213203435596)) ;
#97375=CARTESIAN_POINT('Origin',(77.578119440745,248.391951183936,18.1213203435596)) ;
#97376=CARTESIAN_POINT('',(66.3218485782223,248.291951183936,18.1213203435596)) ;
#97377=CARTESIAN_POINT('Origin',(75.7388649854292,243.867931095515,18.1213203435596)) ;
#97378=CARTESIAN_POINT('Origin',(76.7495157419148,246.353832005802,18.1213203435596)) ;
#97379=CARTESIAN_POINT('Origin',(74.3655697550003,252.217631603154,18.1213203435596)) ;
#97380=CARTESIAN_POINT('Origin',(75.9209120430846,248.391951183936,18.1213203435596)) ;
#97381=CARTESIAN_POINT('Origin',(65.8745236568046,248.391951183936,18.1213203435596)) ;
#97382=CARTESIAN_POINT('Origin',(76.4348658990794,248.391951183936,18.1213203435596)) ;
#97383=CARTESIAN_POINT('Origin',(68.1060880979734,244.423124592531,18.1213203435596)) ;
#97384=CARTESIAN_POINT('Origin',(76.1283346412558,249.472090948443,18.1213203435596)) ;
#97385=CARTESIAN_POINT('Origin',(75.2544545302692,248.922096472997,18.1213203435596)) ;
#97386=CARTESIAN_POINT('Origin',(76.2348658990794,249.302824616567,18.1213203435596)) ;
#97387=CARTESIAN_POINT('Origin',(76.4348658990794,249.302824616567,18.1213203435596)) ;
#97388=CARTESIAN_POINT('Origin',(76.4348658990794,249.176412308284,18.1213203435596)) ;
#97389=CARTESIAN_POINT('Origin',(76.2348658990794,249.302824616567,18.1213203435596)) ;
#97390=CARTESIAN_POINT('',(75.8620064966968,249.895256778131,18.1213203435596)) ;
#97391=CARTESIAN_POINT('Origin',(75.8087408677849,249.979889944069,18.1213203435596)) ;
#97392=CARTESIAN_POINT('Origin',(76.2348658990794,249.302824616567,18.1213203435596)) ;
#97393=CARTESIAN_POINT('Origin',(68.223434379996,245.20592082588,18.1213203435596)) ;
#97394=CARTESIAN_POINT('',(74.9881263857102,249.345262302685,18.1213203435596)) ;
#97395=CARTESIAN_POINT('Origin',(74.9348607567984,249.429895468622,18.1213203435596)) ;
#97396=CARTESIAN_POINT('',(68.2767000089078,245.121287659942,18.1213203435596)) ;
#97397=CARTESIAN_POINT('Origin',(75.8620064966968,249.895256778131,18.0213203435596)) ;
#97398=CARTESIAN_POINT('',(74.9881263857102,249.345262302685,18.0213203435596)) ;
#97399=CARTESIAN_POINT('',(75.8620064966968,249.895256778131,18.0213203435596)) ;
#97400=CARTESIAN_POINT('Origin',(76.2348658990794,249.302824616567,18.0213203435596)) ;
#97401=CARTESIAN_POINT('',(76.9348658990794,249.302824616567,18.0213203435596)) ;
#97402=CARTESIAN_POINT('Origin',(76.9348658990794,248.291951183936,18.0213203435596)) ;
#97403=CARTESIAN_POINT('',(76.9348658990794,248.291951183936,18.0213203435596)) ;
#97404=CARTESIAN_POINT('Origin',(77.4295157419147,248.291951183936,18.0213203435596)) ;
#97405=CARTESIAN_POINT('Origin',(71.0478693800126,252.145540430945,18.1213203435596)) ;
#97406=CARTESIAN_POINT('',(74.0601316280705,247.171652088685,18.1213203435596)) ;
#97407=CARTESIAN_POINT('Origin',(74.19803042292,247.140284551659,18.1213203435596)) ;
#97408=CARTESIAN_POINT('',(73.8470691124233,247.510184752435,18.1213203435596)) ;
#97409=CARTESIAN_POINT('',(70.963236214075,252.092274802033,18.1213203435596)) ;
#97410=CARTESIAN_POINT('Origin',(73.8784366494491,247.648083547285,18.1213203435596)) ;
#97411=CARTESIAN_POINT('Origin',(72.0133921147013,248.637481603717,18.1213203435596)) ;
#97412=CARTESIAN_POINT('',(72.1133921147013,247.214089774802,18.1213203435596)) ;
#97413=CARTESIAN_POINT('',(72.1133921147013,248.637481603717,18.1213203435596)) ;
#97414=CARTESIAN_POINT('Origin',(72.0133921147013,247.214089774802,18.1213203435596)) ;
#97415=CARTESIAN_POINT('Origin',(72.0133921147013,248.124963207434,18.1213203435596)) ;
#97416=CARTESIAN_POINT('Origin',(63.416461843198,248.124963207434,18.1213203435596)) ;
#97417=CARTESIAN_POINT('Origin',(71.4701385730357,248.124963207434,18.1213203435596)) ;
#97418=CARTESIAN_POINT('Origin',(70.8466068278818,246.591260172113,18.1213203435596)) ;
#97419=CARTESIAN_POINT('Origin',(72.2987422718658,250.163082385568,18.1213203435596)) ;
#97420=CARTESIAN_POINT('Origin',(71.6675838322311,251.715544825786,18.1213203435596)) ;
#97421=CARTESIAN_POINT('Origin',(73.1273459706961,248.124963207434,18.1213203435596)) ;
#97422=CARTESIAN_POINT('Origin',(63.8637867646156,248.124963207434,18.1213203435596)) ;
#97423=CARTESIAN_POINT('Origin',(72.6133921147013,248.124963207434,18.1213203435596)) ;
#97424=CARTESIAN_POINT('Origin',(72.8133921147013,247.214089774802,18.1213203435596)) ;
#97425=CARTESIAN_POINT('',(73.1862515170839,246.621657613239,18.1213203435596)) ;
#97426=CARTESIAN_POINT('Origin',(73.2395171459957,246.537024447301,18.1213203435596)) ;
#97427=CARTESIAN_POINT('Origin',(72.8133921147013,247.214089774802,18.1213203435596)) ;
#97428=CARTESIAN_POINT('Origin',(67.3503775087141,242.830572927334,18.1213203435596)) ;
#97429=CARTESIAN_POINT('',(67.2971118798023,242.915206093271,18.1213203435596)) ;
#97430=CARTESIAN_POINT('Origin',(67.4677237907363,243.613369160683,18.1213203435596)) ;
#97431=CARTESIAN_POINT('',(67.5209894196481,243.528735994745,18.1213203435596)) ;
#97432=CARTESIAN_POINT('Origin',(72.9199233725249,247.044823442927,18.1213203435596)) ;
#97433=CARTESIAN_POINT('Origin',(72.8133921147013,247.214089774802,18.1213203435596)) ;
#97434=CARTESIAN_POINT('Origin',(72.6133921147013,247.214089774802,18.1213203435596)) ;
#97435=CARTESIAN_POINT('Origin',(72.6133921147013,248.132044887401,18.1213203435596)) ;
#97436=CARTESIAN_POINT('Origin',(73.8470691124233,247.510184752435,18.0213203435596)) ;
#97437=CARTESIAN_POINT('',(73.8470691124233,247.510184752435,18.0213203435596)) ;
#97438=CARTESIAN_POINT('Origin',(74.0601316280705,247.171652088685,18.0213203435596)) ;
#97439=CARTESIAN_POINT('',(74.0601316280705,247.171652088685,18.0213203435596)) ;
#97440=CARTESIAN_POINT('Origin',(73.1862515170839,246.621657613239,18.0213203435596)) ;
#97441=CARTESIAN_POINT('',(73.1862515170839,246.621657613239,18.0213203435596)) ;
#97442=CARTESIAN_POINT('Origin',(72.8133921147013,247.214089774802,18.0213203435596)) ;
#97443=CARTESIAN_POINT('',(72.1133921147013,247.214089774802,18.0213203435596)) ;
#97444=CARTESIAN_POINT('Origin',(72.1133921147013,248.224963207434,18.0213203435596)) ;
#97445=CARTESIAN_POINT('Origin',(74.9881263857102,249.345262302685,18.0213203435596)) ;
#97446=CARTESIAN_POINT('Origin',(74.7283628290596,246.92834685842,18.0213203435596)) ;
#97447=CARTESIAN_POINT('',(74.7283628290596,246.92834685842,18.0213203435596)) ;
#97448=CARTESIAN_POINT('Origin',(74.3283628290596,246.92834685842,18.0213203435596)) ;
#97449=CARTESIAN_POINT('Origin',(62.9,257.02214694455,20.0213203435596)) ;
#97450=CARTESIAN_POINT('Origin',(29.2133075051975,255.671997914687,20.0213203435596)) ;
#97451=CARTESIAN_POINT('Origin',(60.4815941846227,255.82214694455,20.0213203435596)) ;
#97452=CARTESIAN_POINT('Origin',(75.8499999999999,228.11847800166,30.7213203435596)) ;
#97453=CARTESIAN_POINT('',(70.4999999999999,220.262610236549,30.7213203435596)) ;
#97454=CARTESIAN_POINT('',(73.9975476984278,220.262610236549,30.7213203435596)) ;
#97455=CARTESIAN_POINT('',(70.4999999999999,220.305309236677,30.7213203435596)) ;
#97456=CARTESIAN_POINT('Origin',(55.2141814145299,240.716611331017,20.0213203435596)) ;
#97457=CARTESIAN_POINT('',(77.1300306216516,253.207106781187,20.0213203435596)) ;
#97458=CARTESIAN_POINT('',(52.2356360608974,253.207106781187,20.0213203435596)) ;
#97459=CARTESIAN_POINT('',(77.75,255.5,20.0213203435596)) ;
#97460=CARTESIAN_POINT('Origin',(73.2,255.5,20.0213203435596)) ;
#97461=CARTESIAN_POINT('',(77.75,256.631336165532,20.0213203435596)) ;
#97462=CARTESIAN_POINT('',(77.75,248.684378986433,20.0213203435596)) ;
#97463=CARTESIAN_POINT('',(77.7,257.767080845051,20.0213203435596)) ;
#97464=CARTESIAN_POINT('Origin',(73.2,257.,20.0213203435596)) ;
#97465=CARTESIAN_POINT('',(77.7,261.8,20.0213203435596)) ;
#97466=CARTESIAN_POINT('',(77.7,249.220072841596,20.0213203435596)) ;
#97467=CARTESIAN_POINT('',(66.207090707265,261.8,20.0213203435596)) ;
#97468=CARTESIAN_POINT('Origin',(26.7,263.8,30.7213203435596)) ;
#97469=CARTESIAN_POINT('',(26.7,245.5,30.7213203435596)) ;
#97470=CARTESIAN_POINT('Origin',(59.9573593128807,226.261195155516,30.7213203435596)) ;
#97471=CARTESIAN_POINT('',(56.9573593128807,226.261195155516,30.7213203435596)) ;
#97472=CARTESIAN_POINT('',(56.9573593128807,226.261195155516,30.7213203435596)) ;
#97473=CARTESIAN_POINT('Origin',(59.9573593128807,226.261195155516,30.7213203435596)) ;
#97474=CARTESIAN_POINT('Origin',(56.9573593128808,244.4,30.7213203435596)) ;
#97475=CARTESIAN_POINT('',(56.9573593128808,244.4,30.7213203435596)) ;
#97476=CARTESIAN_POINT('',(56.9573593128808,244.4,30.7213203435596)) ;
#97477=CARTESIAN_POINT('',(56.9573593128808,244.4,30.7213203435596)) ;
#97478=CARTESIAN_POINT('Origin',(55.3573593128808,244.4,30.7213203435596)) ;
#97479=CARTESIAN_POINT('',(55.3573593128808,246.,30.7213203435596)) ;
#97480=CARTESIAN_POINT('',(55.3573593128808,246.,30.7213203435596)) ;
#97481=CARTESIAN_POINT('Origin',(55.3573593128808,244.4,30.7213203435596)) ;
#97482=CARTESIAN_POINT('Origin',(47.2,246.,30.7213203435596)) ;
#97483=CARTESIAN_POINT('',(47.2,246.,30.7213203435596)) ;
#97484=CARTESIAN_POINT('',(47.2,246.,30.7213203435596)) ;
#97485=CARTESIAN_POINT('',(47.2,246.,30.7213203435596)) ;
#97486=CARTESIAN_POINT('Origin',(47.2,248.9,30.7213203435596)) ;
#97487=CARTESIAN_POINT('',(47.2,248.9,30.7213203435596)) ;
#97488=CARTESIAN_POINT('',(47.2,248.9,30.7213203435596)) ;
#97489=CARTESIAN_POINT('',(47.2,248.9,30.7213203435596)) ;
#97490=CARTESIAN_POINT('Origin',(46.3,248.9,30.7213203435596)) ;
#97491=CARTESIAN_POINT('',(46.3,248.9,30.7213203435596)) ;
#97492=CARTESIAN_POINT('',(46.3,248.9,30.7213203435596)) ;
#97493=CARTESIAN_POINT('',(47.2,248.9,30.7213203435596)) ;
#97494=CARTESIAN_POINT('Origin',(53.5411791018402,233.961738491187,30.7213203435596)) ;
#97495=CARTESIAN_POINT('',(46.3,245.6,30.7213203435596)) ;
#97496=CARTESIAN_POINT('',(46.3,245.6,30.7213203435596)) ;
#97497=CARTESIAN_POINT('Origin',(46.8000000000001,245.6,30.7213203435596)) ;
#97498=CARTESIAN_POINT('Origin',(46.8000000000001,245.6,29.5213203435596)) ;
#97499=CARTESIAN_POINT('',(46.3,245.6,20.0213203435596)) ;
#97500=CARTESIAN_POINT('',(46.3,245.6,29.5213203435596)) ;
#97501=CARTESIAN_POINT('Origin',(46.8000000000001,245.6,20.0213203435596)) ;
#97502=CARTESIAN_POINT('Origin',(46.3,245.6,29.5213203435596)) ;
#97503=CARTESIAN_POINT('',(46.3,248.9,20.0213203435596)) ;
#97504=CARTESIAN_POINT('',(46.3,248.9,29.5213203435596)) ;
#97505=CARTESIAN_POINT('',(46.3,245.6,20.0213203435596)) ;
#97506=CARTESIAN_POINT('Origin',(33.8,245.5,30.7213203435596)) ;
#97507=CARTESIAN_POINT('',(33.8,245.5,30.7213203435596)) ;
#97508=CARTESIAN_POINT('Origin',(26.7,245.5,30.7213203435596)) ;
#97509=CARTESIAN_POINT('Origin',(34.1,248.9,29.5213203435596)) ;
#97510=CARTESIAN_POINT('',(34.1,245.6,20.0213203435596)) ;
#97511=CARTESIAN_POINT('',(34.1,245.6,29.5213203435596)) ;
#97512=CARTESIAN_POINT('',(34.1,248.9,20.0213203435596)) ;
#97513=CARTESIAN_POINT('',(34.1,248.9,20.0213203435596)) ;
#97514=CARTESIAN_POINT('',(34.1,248.9,29.5213203435596)) ;
#97515=CARTESIAN_POINT('Origin',(75.4283628290596,245.483789937202,16.0213203435596)) ;
#97516=CARTESIAN_POINT('',(75.4283628290596,246.,18.5213203435596)) ;
#97517=CARTESIAN_POINT('',(75.4283628290596,246.,18.5213203435596)) ;
#97518=CARTESIAN_POINT('',(75.4283628290596,246.,16.0213203435596)) ;
#97519=CARTESIAN_POINT('Origin',(75.4283628290596,246.,16.0213203435596)) ;
#97520=CARTESIAN_POINT('',(73.6283628290596,246.,18.5213203435596)) ;
#97521=CARTESIAN_POINT('',(73.6283628290596,246.,18.5213203435596)) ;
#97522=CARTESIAN_POINT('',(73.6283628290596,246.,16.0213203435596)) ;
#97523=CARTESIAN_POINT('Origin',(73.6283628290596,246.,16.0213203435596)) ;
#97524=CARTESIAN_POINT('',(73.6283628290596,244.8,18.5213203435596)) ;
#97525=CARTESIAN_POINT('Origin',(74.5283628290597,239.625,18.5213203435596)) ;
#97526=CARTESIAN_POINT('Origin',(41.7,245.1,19.2213203435596)) ;
#97527=CARTESIAN_POINT('',(55.3573593128808,245.1,20.0213203435596)) ;
#97528=CARTESIAN_POINT('',(38.7,245.1,22.2213203435596)) ;
#97529=CARTESIAN_POINT('',(38.7,245.1,19.2213203435596)) ;
#97530=CARTESIAN_POINT('',(41.7,245.1,22.2213203435596)) ;
#97531=CARTESIAN_POINT('',(55.3573593128808,245.1,22.2213203435596)) ;
#97532=CARTESIAN_POINT('',(41.7,245.1,19.2213203435596)) ;
#97533=CARTESIAN_POINT('Origin',(40.2,242.9,19.2213203435596)) ;
#97534=CARTESIAN_POINT('',(41.7000000000001,242.9,22.2213203435596)) ;
#97535=CARTESIAN_POINT('',(41.7000000000001,242.9,19.2213203435596)) ;
#97536=CARTESIAN_POINT('',(38.7000000000001,242.9,22.2213203435596)) ;
#97537=CARTESIAN_POINT('Origin',(40.2,242.9,22.2213203435596)) ;
#97538=CARTESIAN_POINT('',(38.7000000000001,242.9,19.2213203435596)) ;
#97539=CARTESIAN_POINT('Origin',(38.7,245.1,19.2213203435596)) ;
#97540=CARTESIAN_POINT('',(38.7000000000001,242.9,22.2213203435596)) ;
#97541=CARTESIAN_POINT('Origin',(41.7000000000001,242.9,19.2213203435596)) ;
#97542=CARTESIAN_POINT('',(41.7,246.9,22.2213203435596)) ;
#97543=CARTESIAN_POINT('Origin',(40.2,243.25,22.2213203435596)) ;
#97544=CARTESIAN_POINT('Origin',(59.7722678973651,244.793417527584,18.0213203435596)) ;
#97545=CARTESIAN_POINT('',(59.4894251848905,244.51057481511,24.0213203435596)) ;
#97546=CARTESIAN_POINT('',(59.4894251848905,244.51057481511,18.0213203435596)) ;
#97547=CARTESIAN_POINT('Origin',(59.7722678973651,244.793417527584,24.0213203435596)) ;
#97548=CARTESIAN_POINT('Origin',(68.4464305354851,241.4,17.0213203435596)) ;
#97549=CARTESIAN_POINT('Origin',(66.25,251.8,23.0213203435596)) ;
#97550=CARTESIAN_POINT('Origin',(66.25,251.8,23.0213203435596)) ;
#97551=CARTESIAN_POINT('',(58.5931591083782,252.048885472713,23.0213203435596)) ;
#97552=CARTESIAN_POINT('Origin',(62.7,247.5,24.0213203435596)) ;
#97553=CARTESIAN_POINT('',(59.35,244.65,24.0213203435596)) ;
#97554=CARTESIAN_POINT('',(58.3716948501153,251.81856264412,24.0213203435596)) ;
#97555=CARTESIAN_POINT('',(65.7,242.,24.0213203435596)) ;
#97556=CARTESIAN_POINT('Origin',(59.1,244.9,24.0213203435596)) ;
#97557=CARTESIAN_POINT('Origin',(43.7,259.4,24.7713203435596)) ;
#97558=CARTESIAN_POINT('',(43.7,259.,25.7213203435596)) ;
#97559=CARTESIAN_POINT('',(43.7,259.,24.7713203435596)) ;
#97560=CARTESIAN_POINT('Origin',(43.7,259.4,25.7213203435596)) ;
#97561=CARTESIAN_POINT('Origin',(45.7,259.,20.0213203435596)) ;
#97562=CARTESIAN_POINT('',(34.7,259.,25.7213203435596)) ;
#97563=CARTESIAN_POINT('Origin',(36.7,259.4,24.7713203435596)) ;
#97564=CARTESIAN_POINT('',(36.7,259.,24.7713203435596)) ;
#97565=CARTESIAN_POINT('Origin',(58.45,251.9,24.0213203435596)) ;
#97566=CARTESIAN_POINT('Origin',(62.9568347953872,216.946231446812,18.0213203435596)) ;
#97567=CARTESIAN_POINT('',(62.9568347953872,216.946231446812,18.0213203435596)) ;
#97568=CARTESIAN_POINT('Origin',(65.3568347953872,216.946231446812,18.0213203435596)) ;
#97569=CARTESIAN_POINT('Origin',(65.7,242.,24.0213203435596)) ;
#97570=CARTESIAN_POINT('Origin',(67.55,249.825,18.7713203435596)) ;
#97571=CARTESIAN_POINT('Origin',(77.7,249.220072841596,20.5213203435596)) ;
#97572=CARTESIAN_POINT('',(77.2,257.723534352175,20.5213203435596)) ;
#97573=CARTESIAN_POINT('Ctrl Pts',(77.7,257.767080845051,20.0213203435596)) ;
#97574=CARTESIAN_POINT('Ctrl Pts',(77.6987927240906,257.766978684289,20.0213203435596)) ;
#97575=CARTESIAN_POINT('Ctrl Pts',(77.6975854537437,257.766876503587,20.021324716105)) ;
#97576=CARTESIAN_POINT('Ctrl Pts',(77.6963782127139,257.766774304936,20.0213334610748)) ;
#97577=CARTESIAN_POINT('Ctrl Pts',(77.6298579761241,257.761143052947,20.0218153180106)) ;
#97578=CARTESIAN_POINT('Ctrl Pts',(77.5640846778152,257.755510562374,20.0355676249654)) ;
#97579=CARTESIAN_POINT('Ctrl Pts',(77.5029237754161,257.75021874678,20.0617978068938)) ;
#97580=CARTESIAN_POINT('Ctrl Pts',(77.4431171654848,257.74504410843,20.0874471710707)) ;
#97581=CARTESIAN_POINT('Ctrl Pts',(77.3888531038272,257.740294173789,20.1245427545607)) ;
#97582=CARTESIAN_POINT('Ctrl Pts',(77.3432091028781,257.736270106201,20.171034380765)) ;
#97583=CARTESIAN_POINT('Ctrl Pts',(77.297752578747,257.73226256695,20.2173350486404)) ;
#97584=CARTESIAN_POINT('Ctrl Pts',(77.2617111099311,257.729052975728,20.2720740981487)) ;
#97585=CARTESIAN_POINT('Ctrl Pts',(77.2371396870212,257.726858660253,20.3322163227955)) ;
#97586=CARTESIAN_POINT('Ctrl Pts',(77.2126212406766,257.724669075773,20.3922288793925)) ;
#97587=CARTESIAN_POINT('Ctrl Pts',(77.2,257.723534352175,20.4564568635466)) ;
#97588=CARTESIAN_POINT('Ctrl Pts',(77.2,257.723534352175,20.5213203435596)) ;
#97589=CARTESIAN_POINT('',(77.2,261.559687576257,20.5213203435596)) ;
#97590=CARTESIAN_POINT('',(77.2,249.220072841596,20.5213203435596)) ;
#97591=CARTESIAN_POINT('Origin',(77.7,261.559687576257,20.5213203435596)) ;
#97592=CARTESIAN_POINT('Origin',(68.6263598493594,261.559687576257,20.5213203435596)) ;
#97593=CARTESIAN_POINT('',(69.117630762786,261.652708485847,20.5213203435596)) ;
#97594=CARTESIAN_POINT('Origin',(68.6263598493594,261.559687576257,20.5213203435596)) ;
#97595=CARTESIAN_POINT('',(68.6263598493594,261.950121980978,20.2089728197824)) ;
#97596=CARTESIAN_POINT('Origin',(68.6263598493594,261.559687576257,20.5213203435596)) ;
#97597=CARTESIAN_POINT('Origin',(68.6263598493594,261.559687576257,20.5213203435596)) ;
#97598=CARTESIAN_POINT('Origin',(73.2,257.,20.5213203435596)) ;
#97599=CARTESIAN_POINT('',(77.25,256.652146641849,20.5213203435596)) ;
#97600=CARTESIAN_POINT('Ctrl Pts',(77.75,256.631336165532,20.0213203435596)) ;
#97601=CARTESIAN_POINT('Ctrl Pts',(77.7485328081134,256.63139550792,20.0213203435596)) ;
#97602=CARTESIAN_POINT('Ctrl Pts',(77.7470656238674,256.631454864325,20.0213268015157)) ;
#97603=CARTESIAN_POINT('Ctrl Pts',(77.7455984898958,256.631514233046,20.0213397172261)) ;
#97604=CARTESIAN_POINT('Ctrl Pts',(77.6796694448428,256.634182103317,20.0219201144309)) ;
#97605=CARTESIAN_POINT('Ctrl Pts',(77.6144986337877,256.636849380763,20.0355352673941)) ;
#97606=CARTESIAN_POINT('Ctrl Pts',(77.5538469838264,256.639357070684,20.0614029659297)) ;
#97607=CARTESIAN_POINT('Ctrl Pts',(77.4939656651802,256.641832910654,20.0869421210828)) ;
#97608=CARTESIAN_POINT('Ctrl Pts',(77.4396362683022,256.644105318551,20.1239355278407)) ;
#97609=CARTESIAN_POINT('Ctrl Pts',(77.3939221201998,256.646031042763,20.1703095979733)) ;
#97610=CARTESIAN_POINT('Ctrl Pts',(77.3482511109358,256.647954949736,20.2166399065224)) ;
#97611=CARTESIAN_POINT('Ctrl Pts',(77.3120515823072,256.64949525193,20.2714483566738)) ;
#97612=CARTESIAN_POINT('Ctrl Pts',(77.2873671506917,256.65054853451,20.3316605250927)) ;
#97613=CARTESIAN_POINT('Ctrl Pts',(77.2626949528298,256.651601295077,20.3918428519969)) ;
#97614=CARTESIAN_POINT('Ctrl Pts',(77.25,256.652146641849,20.4562688621889)) ;
#97615=CARTESIAN_POINT('Ctrl Pts',(77.25,256.652146641849,20.5213203435596)) ;
#97616=CARTESIAN_POINT('Origin',(73.2,257.,20.5213203435596)) ;
#97617=CARTESIAN_POINT('Ctrl Pts',(55.5095145719656,261.79455482774,20.2277364888237)) ;
#97618=CARTESIAN_POINT('Ctrl Pts',(55.5340602178732,261.756752943059,20.1881500276994)) ;
#97619=CARTESIAN_POINT('Ctrl Pts',(55.5890667713761,261.688545713664,20.1225709708889)) ;
#97620=CARTESIAN_POINT('Ctrl Pts',(55.735413453564,261.557876251656,20.0417117307531)) ;
#97621=CARTESIAN_POINT('Ctrl Pts',(55.8502255851785,261.475529765423,20.0213203435596)) ;
#97622=CARTESIAN_POINT('Ctrl Pts',(55.9002853073786,261.439128427997,20.0213203435596)) ;
#97623=CARTESIAN_POINT('Ctrl Pts',(55.5235850209285,261.795524155342,20.2176307773862)) ;
#97624=CARTESIAN_POINT('Ctrl Pts',(55.5482267599533,261.758752662429,20.1800147865656)) ;
#97625=CARTESIAN_POINT('Ctrl Pts',(55.6035725767284,261.691952725752,20.1174091581561)) ;
#97626=CARTESIAN_POINT('Ctrl Pts',(55.7504527952051,261.564081963617,20.0401902813788)) ;
#97627=CARTESIAN_POINT('Ctrl Pts',(55.8622446715528,261.484225598423,20.0213203435596)) ;
#97628=CARTESIAN_POINT('Ctrl Pts',(55.9108349616358,261.448512190495,20.0213203435596)) ;
#97629=CARTESIAN_POINT('Ctrl Pts',(55.5532287114159,261.797064527402,20.1984257565318)) ;
#97630=CARTESIAN_POINT('Ctrl Pts',(55.5780804509168,261.762295810682,20.1644899997044)) ;
#97631=CARTESIAN_POINT('Ctrl Pts',(55.6342304168334,261.698178708499,20.1074661938862)) ;
#97632=CARTESIAN_POINT('Ctrl Pts',(55.7819183628387,261.575867031561,20.0373124202088)) ;
#97633=CARTESIAN_POINT('Ctrl Pts',(55.8872841120386,261.500839109789,20.0213203435596)) ;
#97634=CARTESIAN_POINT('Ctrl Pts',(55.9330008011269,261.466448157126,20.0213203435596)) ;
#97635=CARTESIAN_POINT('Ctrl Pts',(55.6031763483208,261.79822250744,20.1723029608032)) ;
#97636=CARTESIAN_POINT('Ctrl Pts',(55.6283903853712,261.766259990504,20.1432509083838)) ;
#97637=CARTESIAN_POINT('Ctrl Pts',(55.6861581265256,261.705670081893,20.0935677319834)) ;
#97638=CARTESIAN_POINT('Ctrl Pts',(55.8330482728718,261.591606059386,20.0335654961594)) ;
#97639=CARTESIAN_POINT('Ctrl Pts',(55.9272521877398,261.523003776658,20.0213203435596)) ;
#97640=CARTESIAN_POINT('Ctrl Pts',(55.9685491941045,261.490298772052,20.0213203435596)) ;
#97641=CARTESIAN_POINT('Ctrl Pts',(55.6599047282381,261.79814256388,20.1486416834275)) ;
#97642=CARTESIAN_POINT('Ctrl Pts',(55.6855379524164,261.768683922706,20.123848253105)) ;
#97643=CARTESIAN_POINT('Ctrl Pts',(55.7449568036994,261.711182780251,20.0807219288465)) ;
#97644=CARTESIAN_POINT('Ctrl Pts',(55.887500553162,261.605190989655,20.0304664474941)) ;
#97645=CARTESIAN_POINT('Ctrl Pts',(55.9689294097052,261.541942710494,20.0213203435596)) ;
#97646=CARTESIAN_POINT('Ctrl Pts',(56.0055078009848,261.510563832554,20.0213203435596)) ;
#97647=CARTESIAN_POINT('Ctrl Pts',(55.7252078119995,261.796555096217,20.1272203634637)) ;
#97648=CARTESIAN_POINT('Ctrl Pts',(55.751115773334,261.769255478328,20.1061252686703)) ;
#97649=CARTESIAN_POINT('Ctrl Pts',(55.8113298661455,261.714598172442,20.0691496430748)) ;
#97650=CARTESIAN_POINT('Ctrl Pts',(55.9442663460163,261.616377934868,20.0280919148922)) ;
#97651=CARTESIAN_POINT('Ctrl Pts',(56.0117059172473,261.557294041147,20.0213203435596)) ;
#97652=CARTESIAN_POINT('Ctrl Pts',(56.0432529317468,261.526923260636,20.0213203435596)) ;
#97653=CARTESIAN_POINT('Ctrl Pts',(55.8010086453308,261.793278462298,20.1080994112902)) ;
#97654=CARTESIAN_POINT('Ctrl Pts',(55.8264732881332,261.767898003963,20.0903515933129)) ;
#97655=CARTESIAN_POINT('Ctrl Pts',(55.88546498208,261.715868557646,20.0591653394807)) ;
#97656=CARTESIAN_POINT('Ctrl Pts',(56.0021591954208,261.625132679932,20.0265188148335)) ;
#97657=CARTESIAN_POINT('Ctrl Pts',(56.0555340297016,261.569069711917,20.0213203435596)) ;
#97658=CARTESIAN_POINT('Ctrl Pts',(56.081895506616,261.539529506758,20.0213203435596)) ;
#97659=CARTESIAN_POINT('Ctrl Pts',(55.8886521902875,261.788562905801,20.0918367827122)) ;
#97660=CARTESIAN_POINT('Ctrl Pts',(55.9122449680893,261.764902435925,20.077124846578)) ;
#97661=CARTESIAN_POINT('Ctrl Pts',(55.966266526308,261.715404406956,20.0512640137083)) ;
#97662=CARTESIAN_POINT('Ctrl Pts',(56.060051810839,261.631716223329,20.0257337627999)) ;
#97663=CARTESIAN_POINT('Ctrl Pts',(56.1003810935014,261.577565074392,20.0213203435596)) ;
#97664=CARTESIAN_POINT('Ctrl Pts',(56.1213725159607,261.548761013242,20.0213203435596)) ;
#97665=CARTESIAN_POINT('Ctrl Pts',(55.9864294144668,261.783244910011,20.0795560745166)) ;
#97666=CARTESIAN_POINT('Ctrl Pts',(56.0059208588127,261.761024223606,20.0673697854514)) ;
#97667=CARTESIAN_POINT('Ctrl Pts',(56.0496683079691,261.713900171691,20.0459122043803)) ;
#97668=CARTESIAN_POINT('Ctrl Pts',(56.1161262096349,261.636127836261,20.0255537625844)) ;
#97669=CARTESIAN_POINT('Ctrl Pts',(56.145213082859,261.582971518512,20.0213203435596)) ;
#97670=CARTESIAN_POINT('Ctrl Pts',(56.1607380593261,261.554911951281,20.0213203435596)) ;
#97671=CARTESIAN_POINT('Ctrl Pts',(56.0870864420511,261.778692438248,20.0723692404909)) ;
#97672=CARTESIAN_POINT('Ctrl Pts',(56.100316035454,261.75738417469,20.0617919516248)) ;
#97673=CARTESIAN_POINT('Ctrl Pts',(56.1294240269605,261.712066783038,20.0432182833585)) ;
#97674=CARTESIAN_POINT('Ctrl Pts',(56.1690343411742,261.638107172439,20.0256017416873)) ;
#97675=CARTESIAN_POINT('Ctrl Pts',(56.1887559131447,261.58555790289,20.0213203435596)) ;
#97676=CARTESIAN_POINT('Ctrl Pts',(56.1988987568555,261.558363227878,20.0213203435596)) ;
#97677=CARTESIAN_POINT('Ctrl Pts',(56.1809390611363,261.776355954665,20.0702679342639)) ;
#97678=CARTESIAN_POINT('Ctrl Pts',(56.1874552820846,261.755032522864,20.0600771865253)) ;
#97679=CARTESIAN_POINT('Ctrl Pts',(56.2013267910678,261.710037910159,20.0423497842736)) ;
#97680=CARTESIAN_POINT('Ctrl Pts',(56.2195156636653,261.637327921928,20.0254466687852)) ;
#97681=CARTESIAN_POINT('Ctrl Pts',(56.2301181856568,261.585806509747,20.0213203435596)) ;
#97682=CARTESIAN_POINT('Ctrl Pts',(56.2351113333668,261.559674193744,20.0213203435596)) ;
#97683=CARTESIAN_POINT('Ctrl Pts',(56.2391336395509,261.776281941501,20.0706687254062)) ;
#97684=CARTESIAN_POINT('Ctrl Pts',(56.2414470866218,261.754222015824,20.0600661769919)) ;
#97685=CARTESIAN_POINT('Ctrl Pts',(56.2461461230855,261.708290875557,20.0419846645419)) ;
#97686=CARTESIAN_POINT('Ctrl Pts',(56.2528435308144,261.635323465912,20.0251686372497)) ;
#97687=CARTESIAN_POINT('Ctrl Pts',(56.2563772874478,261.584992844062,20.0213203435596)) ;
#97688=CARTESIAN_POINT('Ctrl Pts',(56.2580619020738,261.559687576257,20.0213203435596)) ;
#97689=CARTESIAN_POINT('Ctrl Pts',(56.2695111541429,261.776281941501,20.0706687254062)) ;
#97690=CARTESIAN_POINT('Ctrl Pts',(56.2695111541429,261.753848118778,20.0598864727815)) ;
#97691=CARTESIAN_POINT('Ctrl Pts',(56.2695111541429,261.707367453737,20.0416786272431)) ;
#97692=CARTESIAN_POINT('Ctrl Pts',(56.2695111541429,261.634358610927,20.0250444537314)) ;
#97693=CARTESIAN_POINT('Ctrl Pts',(56.2695111541429,261.584578003606,20.0213203435596)) ;
#97694=CARTESIAN_POINT('Ctrl Pts',(56.2695111541429,261.559687576257,20.0213203435596)) ;
#97695=CARTESIAN_POINT('Origin',(56.2695111541429,261.559687576257,20.5213203435596)) ;
#97696=CARTESIAN_POINT('Origin',(55.2268638269143,261.559687576257,20.5213203435596)) ;
#97697=CARTESIAN_POINT('',(55.2268638269143,261.950121980978,20.2089728197824)) ;
#97698=CARTESIAN_POINT('Ctrl Pts',(77.1300306216516,253.207106781187,20.0213203435596)) ;
#97699=CARTESIAN_POINT('Ctrl Pts',(76.9727816340446,253.072343999508,20.0213203435596)) ;
#97700=CARTESIAN_POINT('Ctrl Pts',(76.7853404806882,252.94731363725,19.9686339808095)) ;
#97701=CARTESIAN_POINT('Ctrl Pts',(76.6208916966195,252.853553390593,19.8748737341529)) ;
#97702=CARTESIAN_POINT('Ctrl Pts',(77.0169669281593,253.273071401074,20.0213203435596)) ;
#97703=CARTESIAN_POINT('Ctrl Pts',(76.8741225322589,253.140600606275,20.0395012945359)) ;
#97704=CARTESIAN_POINT('Ctrl Pts',(76.6994917884722,252.999180185916,20.0023959135144)) ;
#97705=CARTESIAN_POINT('Ctrl Pts',(76.543994900258,252.887271264403,19.9085916079623)) ;
#97706=CARTESIAN_POINT('Ctrl Pts',(76.7919007678944,253.404381490571,20.1298498989989)) ;
#97707=CARTESIAN_POINT('Ctrl Pts',(76.6768979485241,253.246681150455,20.1631107893611)) ;
#97708=CARTESIAN_POINT('Ctrl Pts',(76.5281740570552,253.06465267538,20.1270179596422)) ;
#97709=CARTESIAN_POINT('Ctrl Pts',(76.3903553725496,252.918990684446,20.0116085736344)) ;
#97710=CARTESIAN_POINT('Ctrl Pts',(76.6981591247668,253.459073068968,20.3904206496601)) ;
#97711=CARTESIAN_POINT('Ctrl Pts',(76.5739302623505,253.245411894379,20.4018503552973)) ;
#97712=CARTESIAN_POINT('Ctrl Pts',(76.41949641419,253.033434868643,20.3194987016572)) ;
#97713=CARTESIAN_POINT('Ctrl Pts',(76.2808206834693,252.870551298285,20.1561059751854)) ;
#97714=CARTESIAN_POINT('Ctrl Pts',(76.6981591247668,253.459073068968,20.5213203435596)) ;
#97715=CARTESIAN_POINT('Ctrl Pts',(76.5581902456883,253.219165699387,20.5213203435596)) ;
#97716=CARTESIAN_POINT('Ctrl Pts',(76.3913470212719,252.996584175367,20.4159476180594)) ;
#97717=CARTESIAN_POINT('Ctrl Pts',(76.2449695321558,252.82967032967,20.2284271247462)) ;
#97718=CARTESIAN_POINT('',(76.2449695321558,252.82967032967,20.2284271247462)) ;
#97719=CARTESIAN_POINT('',(76.6981591247668,253.459073068968,20.5213203435596)) ;
#97720=CARTESIAN_POINT('Ctrl Pts',(76.2449695321558,252.82967032967,20.2284271247462)) ;
#97721=CARTESIAN_POINT('Ctrl Pts',(76.3913470212719,252.996584175367,20.4159476180594)) ;
#97722=CARTESIAN_POINT('Ctrl Pts',(76.5581902456883,253.219165699387,20.5213203435596)) ;
#97723=CARTESIAN_POINT('Ctrl Pts',(76.6981591247668,253.459073068968,20.5213203435596)) ;
#97724=CARTESIAN_POINT('Origin',(77.1300306216516,253.207106781187,20.5213203435596)) ;
#97725=CARTESIAN_POINT('Ctrl Pts',(77.1300306216516,253.207106781187,20.0213203435596)) ;
#97726=CARTESIAN_POINT('Ctrl Pts',(76.9727816340446,253.072343999508,20.0213203435596)) ;
#97727=CARTESIAN_POINT('Ctrl Pts',(76.7853404806882,252.94731363725,19.9686339808095)) ;
#97728=CARTESIAN_POINT('Ctrl Pts',(76.6208916966195,252.853553390593,19.8748737341529)) ;
#97729=CARTESIAN_POINT('Origin',(76.6208916966195,252.5,20.2284271247462)) ;
#97730=CARTESIAN_POINT('Origin',(73.2,255.5,20.5213203435596)) ;
#97731=CARTESIAN_POINT('',(77.25,255.5,20.5213203435596)) ;
#97732=CARTESIAN_POINT('Origin',(77.75,255.5,20.5213203435596)) ;
#97733=CARTESIAN_POINT('Origin',(73.2,255.5,20.5213203435596)) ;
#97734=CARTESIAN_POINT('Origin',(77.75,248.684378986433,20.5213203435596)) ;
#97735=CARTESIAN_POINT('',(77.25,248.684378986433,20.5213203435596)) ;
#97736=CARTESIAN_POINT('Origin',(52.2356360608974,253.207106781187,19.5213203435596)) ;
#97737=CARTESIAN_POINT('Origin',(46.6263598493593,261.559687576257,20.5213203435596)) ;
#97738=CARTESIAN_POINT('',(47.1176307627859,261.652708485847,20.5213203435596)) ;
#97739=CARTESIAN_POINT('Origin',(46.6263598493593,261.559687576257,20.5213203435596)) ;
#97740=CARTESIAN_POINT('Origin',(46.6263598493593,261.559687576257,20.5213203435596)) ;
#97741=CARTESIAN_POINT('Ctrl Pts',(46.6262992790349,261.950068411826,20.2089058667418)) ;
#97742=CARTESIAN_POINT('Ctrl Pts',(46.6121566500185,262.024832042591,20.3023601782468)) ;
#97743=CARTESIAN_POINT('Ctrl Pts',(46.580666198832,262.09625764165,20.3916424900841)) ;
#97744=CARTESIAN_POINT('Ctrl Pts',(46.5350110422629,262.157126340136,20.4677282733508)) ;
#97745=CARTESIAN_POINT('Ctrl Pts',(46.7442583096226,261.958793642181,20.2197842338569)) ;
#97746=CARTESIAN_POINT('Ctrl Pts',(46.7189281932969,262.039807921917,20.3214382905633)) ;
#97747=CARTESIAN_POINT('Ctrl Pts',(46.675218628264,262.116429910146,20.4166884625079)) ;
#97748=CARTESIAN_POINT('Ctrl Pts',(46.6167573320855,262.181064672294,20.4976354561752)) ;
#97749=CARTESIAN_POINT('Ctrl Pts',(46.979430861431,261.907070818778,20.2967667810524)) ;
#97750=CARTESIAN_POINT('Ctrl Pts',(46.9323308081948,262.013112885638,20.4047147907279)) ;
#97751=CARTESIAN_POINT('Ctrl Pts',(46.8639746536185,262.109285954832,20.5046230523416)) ;
#97752=CARTESIAN_POINT('Ctrl Pts',(46.7800765251102,262.189709099368,20.588731540056)) ;
#97753=CARTESIAN_POINT('Ctrl Pts',(47.1005251724555,261.743097807743,20.4462783497206)) ;
#97754=CARTESIAN_POINT('Ctrl Pts',(47.0598088706616,261.88150309857,20.5446866530911)) ;
#97755=CARTESIAN_POINT('Ctrl Pts',(46.9899272559849,262.009912469407,20.6374702762036)) ;
#97756=CARTESIAN_POINT('Ctrl Pts',(46.8967323918744,262.117798129565,20.7162682354584)) ;
#97757=CARTESIAN_POINT('Ctrl Pts',(47.1176490922737,261.65261165586,20.5212598248177)) ;
#97758=CARTESIAN_POINT('Ctrl Pts',(47.0893506066563,261.802146309377,20.6147189832657)) ;
#97759=CARTESIAN_POINT('Ctrl Pts',(47.0263552568488,261.945003652573,20.7040048227633)) ;
#97760=CARTESIAN_POINT('Ctrl Pts',(46.9350298022437,262.066745503355,20.780093479502)) ;
#97761=CARTESIAN_POINT('',(46.9350889359326,262.066666666667,20.7800442065721)) ;
#97762=CARTESIAN_POINT('Origin',(46.5350889359327,261.766666666667,20.7800442065721)) ;
#97763=CARTESIAN_POINT('Origin',(46.1350889359327,261.466666666667,20.4050442065721)) ;
#97764=CARTESIAN_POINT('Origin',(44.3686862542563,264.655203575568,24.3907153426993)) ;
#97765=CARTESIAN_POINT('',(44.7686862542563,264.955203575568,24.3907153426993)) ;
#97766=CARTESIAN_POINT('Origin',(51.2,257.,20.5213203435596)) ;
#97767=CARTESIAN_POINT('',(55.25,256.652146641849,20.5213203435596)) ;
#97768=CARTESIAN_POINT('',(55.2649110640674,257.,20.5213203435596)) ;
#97769=CARTESIAN_POINT('Origin',(51.2,257.,20.5213203435596)) ;
#97770=CARTESIAN_POINT('Origin',(55.7649110640674,257.,20.5213203435596)) ;
#97771=CARTESIAN_POINT('Ctrl Pts',(55.75,256.631336165532,20.0213203435596)) ;
#97772=CARTESIAN_POINT('Ctrl Pts',(55.7485328081134,256.63139550792,20.0213203435596)) ;
#97773=CARTESIAN_POINT('Ctrl Pts',(55.7470656238674,256.631454864325,20.0213268015157)) ;
#97774=CARTESIAN_POINT('Ctrl Pts',(55.7455984898958,256.631514233046,20.0213397172261)) ;
#97775=CARTESIAN_POINT('Ctrl Pts',(55.6796694448428,256.634182103317,20.0219201144309)) ;
#97776=CARTESIAN_POINT('Ctrl Pts',(55.6144986337877,256.636849380763,20.0355352673941)) ;
#97777=CARTESIAN_POINT('Ctrl Pts',(55.5538469838264,256.639357070684,20.0614029659297)) ;
#97778=CARTESIAN_POINT('Ctrl Pts',(55.4939656651802,256.641832910654,20.0869421210828)) ;
#97779=CARTESIAN_POINT('Ctrl Pts',(55.4396362683022,256.644105318551,20.1239355278407)) ;
#97780=CARTESIAN_POINT('Ctrl Pts',(55.3939221201998,256.646031042763,20.1703095979733)) ;
#97781=CARTESIAN_POINT('Ctrl Pts',(55.3482511109358,256.647954949736,20.2166399065224)) ;
#97782=CARTESIAN_POINT('Ctrl Pts',(55.3120515823072,256.64949525193,20.2714483566738)) ;
#97783=CARTESIAN_POINT('Ctrl Pts',(55.2873671506917,256.65054853451,20.3316605250927)) ;
#97784=CARTESIAN_POINT('Ctrl Pts',(55.2626949528298,256.651601295077,20.3918428519969)) ;
#97785=CARTESIAN_POINT('Ctrl Pts',(55.25,256.652146641849,20.4562688621889)) ;
#97786=CARTESIAN_POINT('Ctrl Pts',(55.25,256.652146641849,20.5213203435596)) ;
#97787=CARTESIAN_POINT('Ctrl Pts',(69.7791083033805,252.853553390593,19.8748737341529)) ;
#97788=CARTESIAN_POINT('Ctrl Pts',(69.6146576393448,252.947314709111,19.9686350526701)) ;
#97789=CARTESIAN_POINT('Ctrl Pts',(69.4272201636148,253.072342458909,20.0213203435596)) ;
#97790=CARTESIAN_POINT('Ctrl Pts',(69.2699693783484,253.207106781187,20.0213203435596)) ;
#97791=CARTESIAN_POINT('Ctrl Pts',(69.8560050997421,252.887271264403,19.9085916079623)) ;
#97792=CARTESIAN_POINT('Ctrl Pts',(69.7005064338981,252.999181465251,20.0023969858787)) ;
#97793=CARTESIAN_POINT('Ctrl Pts',(69.5258791007283,253.140599091878,20.0395015023792)) ;
#97794=CARTESIAN_POINT('Ctrl Pts',(69.3830330718407,253.273071401074,20.0213203435596)) ;
#97795=CARTESIAN_POINT('Ctrl Pts',(70.0096447013339,252.918990818726,20.0116085041473)) ;
#97796=CARTESIAN_POINT('Ctrl Pts',(69.8718244412945,253.064654474858,20.1270192095074)) ;
#97797=CARTESIAN_POINT('Ctrl Pts',(69.7231037922912,253.246679596241,20.1631106762666)) ;
#97798=CARTESIAN_POINT('Ctrl Pts',(69.6080996582165,253.404381739176,20.1298494056682)) ;
#97799=CARTESIAN_POINT('Ctrl Pts',(70.1191793165307,252.870551298284,20.1561059751854)) ;
#97800=CARTESIAN_POINT('Ctrl Pts',(69.9805020004785,253.033436730717,20.3195005695518)) ;
#97801=CARTESIAN_POINT('Ctrl Pts',(69.8260711578255,253.245409451819,20.4018504859609)) ;
#97802=CARTESIAN_POINT('Ctrl Pts',(69.7018408752332,253.459073068968,20.3904206496601)) ;
#97803=CARTESIAN_POINT('Ctrl Pts',(70.1550304678442,252.82967032967,20.2284271247462)) ;
#97804=CARTESIAN_POINT('Ctrl Pts',(70.0086513053506,252.996586083515,20.415949761781)) ;
#97805=CARTESIAN_POINT('Ctrl Pts',(69.8418113544264,253.219162956782,20.5213203435596)) ;
#97806=CARTESIAN_POINT('Ctrl Pts',(69.7018408752332,253.459073068968,20.5213203435597)) ;
#97807=CARTESIAN_POINT('',(69.7018408752332,253.459073068968,20.5213203435596)) ;
#97808=CARTESIAN_POINT('Origin',(69.2699693783484,253.207106781187,20.5213203435596)) ;
#97809=CARTESIAN_POINT('',(70.1550304678442,252.82967032967,20.2284271247462)) ;
#97810=CARTESIAN_POINT('Ctrl Pts',(69.7018408752332,253.459073068968,20.5213203435597)) ;
#97811=CARTESIAN_POINT('Ctrl Pts',(69.8418113544264,253.219162956782,20.5213203435596)) ;
#97812=CARTESIAN_POINT('Ctrl Pts',(70.0086513053506,252.996586083515,20.415949761781)) ;
#97813=CARTESIAN_POINT('Ctrl Pts',(70.1550304678442,252.82967032967,20.2284271247462)) ;
#97814=CARTESIAN_POINT('Origin',(69.7791083033806,252.5,20.2284271247462)) ;
#97815=CARTESIAN_POINT('Origin',(68.65,248.108305665508,20.5213203435596)) ;
#97816=CARTESIAN_POINT('',(69.15,256.652146641849,20.5213203435596)) ;
#97817=CARTESIAN_POINT('',(69.15,255.5,20.5213203435596)) ;
#97818=CARTESIAN_POINT('',(69.15,248.108305665508,20.5213203435596)) ;
#97819=CARTESIAN_POINT('Origin',(68.65,255.5,20.5213203435596)) ;
#97820=CARTESIAN_POINT('Ctrl Pts',(68.65,256.631336165532,20.0213203435596)) ;
#97821=CARTESIAN_POINT('Ctrl Pts',(68.6514671918867,256.63139550792,20.0213203435596)) ;
#97822=CARTESIAN_POINT('Ctrl Pts',(68.6529343761326,256.631454864325,20.0213268015157)) ;
#97823=CARTESIAN_POINT('Ctrl Pts',(68.6544015101042,256.631514233046,20.0213397172261)) ;
#97824=CARTESIAN_POINT('Ctrl Pts',(68.7203305551572,256.634182103317,20.0219201144309)) ;
#97825=CARTESIAN_POINT('Ctrl Pts',(68.7855013662124,256.636849380763,20.0355352673941)) ;
#97826=CARTESIAN_POINT('Ctrl Pts',(68.8461530161737,256.639357070684,20.0614029659297)) ;
#97827=CARTESIAN_POINT('Ctrl Pts',(68.9060343348199,256.641832910654,20.0869421210828)) ;
#97828=CARTESIAN_POINT('Ctrl Pts',(68.9603637316979,256.644105318551,20.1239355278407)) ;
#97829=CARTESIAN_POINT('Ctrl Pts',(69.0060778798002,256.646031042763,20.1703095979734)) ;
#97830=CARTESIAN_POINT('Ctrl Pts',(69.0517488890642,256.647954949736,20.2166399065224)) ;
#97831=CARTESIAN_POINT('Ctrl Pts',(69.0879484176928,256.64949525193,20.2714483566738)) ;
#97832=CARTESIAN_POINT('Ctrl Pts',(69.1126328493083,256.65054853451,20.3316605250927)) ;
#97833=CARTESIAN_POINT('Ctrl Pts',(69.1373050471702,256.651601295077,20.3918428519969)) ;
#97834=CARTESIAN_POINT('Ctrl Pts',(69.15,256.652146641849,20.4562688621889)) ;
#97835=CARTESIAN_POINT('Ctrl Pts',(69.15,256.652146641849,20.5213203435596)) ;
#97836=CARTESIAN_POINT('Origin',(73.2,255.5,20.5213203435596)) ;
#97837=CARTESIAN_POINT('Origin',(73.2,255.5,20.5213203435596)) ;
#97838=CARTESIAN_POINT('Ctrl Pts',(70.1355962910396,252.851973368904,20.2591799537788)) ;
#97839=CARTESIAN_POINT('Ctrl Pts',(70.7856774065376,252.099086619409,19.4120576663318)) ;
#97840=CARTESIAN_POINT('Ctrl Pts',(72.3423540954159,251.274930902987,18.4845162963506)) ;
#97841=CARTESIAN_POINT('Ctrl Pts',(74.7133620656512,251.567894939807,18.8142426993568)) ;
#97842=CARTESIAN_POINT('Ctrl Pts',(75.8285852540374,252.347451852855,19.6915099002701)) ;
#97843=CARTESIAN_POINT('Ctrl Pts',(76.264406030056,252.851970687799,20.2591769318912)) ;
#97844=CARTESIAN_POINT('Ctrl Pts',(70.0947889951709,252.900719289552,20.1752138941917)) ;
#97845=CARTESIAN_POINT('Ctrl Pts',(70.7436999646066,252.124445761866,19.333077491043)) ;
#97846=CARTESIAN_POINT('Ctrl Pts',(72.3252162682866,251.268385211843,18.4095866632333)) ;
#97847=CARTESIAN_POINT('Ctrl Pts',(74.7427882755993,251.573002122969,18.7379343247678)) ;
#97848=CARTESIAN_POINT('Ctrl Pts',(75.8701660286286,252.380531879248,19.6108864310171)) ;
#97849=CARTESIAN_POINT('Ctrl Pts',(76.3052135920791,252.900716378702,20.1752108539644)) ;
#97850=CARTESIAN_POINT('Ctrl Pts',(69.9783224959303,252.946276054393,20.0291514232781)) ;
#97851=CARTESIAN_POINT('Ctrl Pts',(70.6482383333472,252.129634870077,19.1954195941612)) ;
#97852=CARTESIAN_POINT('Ctrl Pts',(72.2905009969719,251.229483751751,18.278969793691)) ;
#97853=CARTESIAN_POINT('Ctrl Pts',(74.8036092356417,251.549747804448,18.6049119908004)) ;
#97854=CARTESIAN_POINT('Ctrl Pts',(75.9725494008639,252.399037878032,19.4704581943099)) ;
#97855=CARTESIAN_POINT('Ctrl Pts',(76.4216801989973,252.946272993645,20.0291483590762)) ;
#97856=CARTESIAN_POINT('Ctrl Pts',(69.8218648241276,252.909543105076,19.9308614440711)) ;
#97857=CARTESIAN_POINT('Ctrl Pts',(70.5341758458511,252.069082299954,19.0904632296569)) ;
#97858=CARTESIAN_POINT('Ctrl Pts',(72.2520280195758,251.147401176394,18.1687895568493)) ;
#97859=CARTESIAN_POINT('Ctrl Pts',(74.8723377634464,251.475110145404,18.4964972590599)) ;
#97860=CARTESIAN_POINT('Ctrl Pts',(76.1005933035414,252.346338454721,19.3676988212773)) ;
#97861=CARTESIAN_POINT('Ctrl Pts',(76.5781378198995,252.909540071613,19.930858408753)) ;
#97862=CARTESIAN_POINT('Ctrl Pts',(69.7553711163591,252.880849873491,19.9021702170509)) ;
#97863=CARTESIAN_POINT('Ctrl Pts',(70.4856634311088,252.033932725798,19.0552530693574)) ;
#97864=CARTESIAN_POINT('Ctrl Pts',(72.2356775436909,251.106558080618,18.1278784241775)) ;
#97865=CARTESIAN_POINT('Ctrl Pts',(74.9015612406156,251.436227730249,18.4575480738079)) ;
#97866=CARTESIAN_POINT('Ctrl Pts',(76.155035835944,252.313317347784,19.3346376913431)) ;
#97867=CARTESIAN_POINT('Ctrl Pts',(76.644631503471,252.880846850851,19.9021671944111)) ;
#97868=CARTESIAN_POINT('Origin',(73.2,255.5,23.2284271247462)) ;
#97869=CARTESIAN_POINT('Ctrl Pts',(55.1300306216516,253.207106781187,20.0213203435596)) ;
#97870=CARTESIAN_POINT('Ctrl Pts',(54.9727816340446,253.072343999508,20.0213203435596)) ;
#97871=CARTESIAN_POINT('Ctrl Pts',(54.7853404806882,252.94731363725,19.9686339808095)) ;
#97872=CARTESIAN_POINT('Ctrl Pts',(54.6208916966195,252.853553390593,19.8748737341529)) ;
#97873=CARTESIAN_POINT('Ctrl Pts',(55.0169669281593,253.273071401074,20.0213203435596)) ;
#97874=CARTESIAN_POINT('Ctrl Pts',(54.8741225322591,253.140600606275,20.0395012945359)) ;
#97875=CARTESIAN_POINT('Ctrl Pts',(54.6994917884722,252.999180185916,20.0023959135144)) ;
#97876=CARTESIAN_POINT('Ctrl Pts',(54.543994900258,252.887271264403,19.9085916079623)) ;
#97877=CARTESIAN_POINT('Ctrl Pts',(54.7918993697755,253.404382306274,20.1298482803242)) ;
#97878=CARTESIAN_POINT('Ctrl Pts',(54.6768965504056,253.246681966159,20.1631091706864)) ;
#97879=CARTESIAN_POINT('Ctrl Pts',(54.5281738146352,253.064653115969,20.1270177316471)) ;
#97880=CARTESIAN_POINT('Ctrl Pts',(54.3903551301296,252.918991125035,20.0116083456393)) ;
#97881=CARTESIAN_POINT('Ctrl Pts',(54.6981591247668,253.459073068968,20.3904206496601)) ;
#97882=CARTESIAN_POINT('Ctrl Pts',(54.573930262351,253.24541189438,20.4018503552973)) ;
#97883=CARTESIAN_POINT('Ctrl Pts',(54.41949641419,253.033434868643,20.3194987016572)) ;
#97884=CARTESIAN_POINT('Ctrl Pts',(54.2808206834693,252.870551298285,20.1561059751854)) ;
#97885=CARTESIAN_POINT('Ctrl Pts',(54.6981591247668,253.459073068968,20.5213203435596)) ;
#97886=CARTESIAN_POINT('Ctrl Pts',(54.5581902456889,253.219165699388,20.5213203435596)) ;
#97887=CARTESIAN_POINT('Ctrl Pts',(54.3913470212719,252.996584175367,20.4159476180594)) ;
#97888=CARTESIAN_POINT('Ctrl Pts',(54.2449695321558,252.82967032967,20.2284271247462)) ;
#97889=CARTESIAN_POINT('',(54.2449695321558,252.82967032967,20.2284271247462)) ;
#97890=CARTESIAN_POINT('',(54.6981591247668,253.459073068968,20.5213203435596)) ;
#97891=CARTESIAN_POINT('Ctrl Pts',(54.2449695321558,252.82967032967,20.2284271247462)) ;
#97892=CARTESIAN_POINT('Ctrl Pts',(54.3913470212719,252.996584175367,20.4159476180594)) ;
#97893=CARTESIAN_POINT('Ctrl Pts',(54.5581902456889,253.219165699388,20.5213203435596)) ;
#97894=CARTESIAN_POINT('Ctrl Pts',(54.6981591247668,253.459073068968,20.5213203435596)) ;
#97895=CARTESIAN_POINT('Origin',(55.1300306216516,253.207106781187,20.5213203435596)) ;
#97896=CARTESIAN_POINT('Origin',(54.6208916966195,252.5,20.2284271247462)) ;
#97897=CARTESIAN_POINT('Origin',(51.2,255.5,20.5213203435596)) ;
#97898=CARTESIAN_POINT('',(55.25,255.5,20.5213203435596)) ;
#97899=CARTESIAN_POINT('Origin',(55.75,255.5,20.5213203435596)) ;
#97900=CARTESIAN_POINT('Origin',(51.2,255.5,20.5213203435596)) ;
#97901=CARTESIAN_POINT('Origin',(55.75,248.684378986433,20.5213203435596)) ;
#97902=CARTESIAN_POINT('',(55.25,248.684378986433,20.5213203435596)) ;
#97903=CARTESIAN_POINT('Ctrl Pts',(47.7791083033805,252.853553390593,19.8748737341529)) ;
#97904=CARTESIAN_POINT('Ctrl Pts',(47.6146576398327,252.947314708832,19.968635052392)) ;
#97905=CARTESIAN_POINT('Ctrl Pts',(47.4272201631483,253.072342459309,20.0213203435596)) ;
#97906=CARTESIAN_POINT('Ctrl Pts',(47.2699693783484,253.207106781187,20.0213203435596)) ;
#97907=CARTESIAN_POINT('Ctrl Pts',(47.8560050997421,252.887271264403,19.9085916079623)) ;
#97908=CARTESIAN_POINT('Ctrl Pts',(47.7005064343595,252.999181464919,20.0023969856004)) ;
#97909=CARTESIAN_POINT('Ctrl Pts',(47.5258791003045,253.140599092271,20.0395015023253)) ;
#97910=CARTESIAN_POINT('Ctrl Pts',(47.3830330718407,253.273071401074,20.0213203435596)) ;
#97911=CARTESIAN_POINT('Ctrl Pts',(48.0096449535698,252.918991277155,20.0116082669203)) ;
#97912=CARTESIAN_POINT('Ctrl Pts',(47.8718246939395,253.064654932855,20.1270189719378)) ;
#97913=CARTESIAN_POINT('Ctrl Pts',(47.7231052466809,253.246680445441,20.1631089919506)) ;
#97914=CARTESIAN_POINT('Ctrl Pts',(47.6081011129474,253.404382587908,20.1298477214509)) ;
#97915=CARTESIAN_POINT('Ctrl Pts',(48.1191793165307,252.870551298284,20.1561059751854)) ;
#97916=CARTESIAN_POINT('Ctrl Pts',(47.9805020008901,253.033436730234,20.3195005690668)) ;
#97917=CARTESIAN_POINT('Ctrl Pts',(47.8260711574569,253.245409452453,20.401850485927)) ;
#97918=CARTESIAN_POINT('Ctrl Pts',(47.7018408752332,253.459073068968,20.3904206496601)) ;
#97919=CARTESIAN_POINT('Ctrl Pts',(48.1550304678442,252.82967032967,20.2284271247462)) ;
#97920=CARTESIAN_POINT('Ctrl Pts',(48.0086513057851,252.996586083019,20.4159497612244)) ;
#97921=CARTESIAN_POINT('Ctrl Pts',(47.8418113540112,253.219162957494,20.5213203435596)) ;
#97922=CARTESIAN_POINT('Ctrl Pts',(47.7018408752332,253.459073068968,20.5213203435597)) ;
#97923=CARTESIAN_POINT('',(47.7018408752332,253.459073068968,20.5213203435596)) ;
#97924=CARTESIAN_POINT('Origin',(47.2699693783484,253.207106781187,20.5213203435596)) ;
#97925=CARTESIAN_POINT('',(48.1550304678442,252.82967032967,20.2284271247462)) ;
#97926=CARTESIAN_POINT('Ctrl Pts',(47.7018408752332,253.459073068968,20.5213203435597)) ;
#97927=CARTESIAN_POINT('Ctrl Pts',(47.8418113540112,253.219162957494,20.5213203435596)) ;
#97928=CARTESIAN_POINT('Ctrl Pts',(48.0086513057851,252.996586083019,20.4159497612244)) ;
#97929=CARTESIAN_POINT('Ctrl Pts',(48.1550304678442,252.82967032967,20.2284271247462)) ;
#97930=CARTESIAN_POINT('Origin',(47.7791083033805,252.5,20.2284271247462)) ;
#97931=CARTESIAN_POINT('Origin',(46.65,248.108305665508,20.5213203435596)) ;
#97932=CARTESIAN_POINT('',(47.15,256.652146641849,20.5213203435596)) ;
#97933=CARTESIAN_POINT('',(47.15,255.5,20.5213203435596)) ;
#97934=CARTESIAN_POINT('',(47.15,248.108305665508,20.5213203435596)) ;
#97935=CARTESIAN_POINT('Origin',(46.65,255.5,20.5213203435596)) ;
#97936=CARTESIAN_POINT('Ctrl Pts',(46.65,256.631336165532,20.0213203435596)) ;
#97937=CARTESIAN_POINT('Ctrl Pts',(46.6514671918867,256.63139550792,20.0213203435596)) ;
#97938=CARTESIAN_POINT('Ctrl Pts',(46.6529343761326,256.631454864325,20.0213268015157)) ;
#97939=CARTESIAN_POINT('Ctrl Pts',(46.6544015101042,256.631514233046,20.0213397172261)) ;
#97940=CARTESIAN_POINT('Ctrl Pts',(46.7203305551572,256.634182103317,20.0219201144309)) ;
#97941=CARTESIAN_POINT('Ctrl Pts',(46.7855013662124,256.636849380763,20.0355352673941)) ;
#97942=CARTESIAN_POINT('Ctrl Pts',(46.8461530161737,256.639357070684,20.0614029659297)) ;
#97943=CARTESIAN_POINT('Ctrl Pts',(46.9060343348199,256.641832910654,20.0869421210828)) ;
#97944=CARTESIAN_POINT('Ctrl Pts',(46.9603637316979,256.644105318551,20.1239355278407)) ;
#97945=CARTESIAN_POINT('Ctrl Pts',(47.0060778798002,256.646031042763,20.1703095979734)) ;
#97946=CARTESIAN_POINT('Ctrl Pts',(47.0517488890642,256.647954949736,20.2166399065224)) ;
#97947=CARTESIAN_POINT('Ctrl Pts',(47.0879484176928,256.64949525193,20.2714483566738)) ;
#97948=CARTESIAN_POINT('Ctrl Pts',(47.1126328493083,256.65054853451,20.3316605250927)) ;
#97949=CARTESIAN_POINT('Ctrl Pts',(47.1373050471702,256.651601295077,20.3918428519969)) ;
#97950=CARTESIAN_POINT('Ctrl Pts',(47.15,256.652146641849,20.4562688621889)) ;
#97951=CARTESIAN_POINT('Ctrl Pts',(47.15,256.652146641849,20.5213203435596)) ;
#97952=CARTESIAN_POINT('Origin',(51.2,255.5,20.5213203435596)) ;
#97953=CARTESIAN_POINT('Origin',(51.2,255.5,20.5213203435596)) ;
#97954=CARTESIAN_POINT('Ctrl Pts',(48.1355790860796,252.851993235277,20.2592073869394)) ;
#97955=CARTESIAN_POINT('Ctrl Pts',(48.7856610521171,252.099095428559,19.4120715145791)) ;
#97956=CARTESIAN_POINT('Ctrl Pts',(50.342337689149,251.274913578509,18.4844993376728)) ;
#97957=CARTESIAN_POINT('Ctrl Pts',(52.7133682967689,251.567886823659,18.8142366178283)) ;
#97958=CARTESIAN_POINT('Ctrl Pts',(53.8285998534377,252.347462033393,19.6915256689909)) ;
#97959=CARTESIAN_POINT('Ctrl Pts',(54.2644232365963,252.851990549191,20.2592043594362)) ;
#97960=CARTESIAN_POINT('Ctrl Pts',(48.0947719613241,252.900740969046,20.1752401619291)) ;
#97961=CARTESIAN_POINT('Ctrl Pts',(48.7436831353515,252.124455787674,19.3330903436158)) ;
#97962=CARTESIAN_POINT('Ctrl Pts',(50.3251986179094,251.268368342706,18.4095681618135)) ;
#97963=CARTESIAN_POINT('Ctrl Pts',(52.7427942699489,251.572994887056,18.7379268805199)) ;
#97964=CARTESIAN_POINT('Ctrl Pts',(53.8701809022354,252.380543404302,19.6109011660618)) ;
#97965=CARTESIAN_POINT('Ctrl Pts',(54.3052306275292,252.900738052886,20.1752371160155)) ;
#97966=CARTESIAN_POINT('Ctrl Pts',(47.9783044652226,252.946300082069,20.029175924824)) ;
#97967=CARTESIAN_POINT('Ctrl Pts',(48.6482204122624,252.129646231424,19.1954309996876)) ;
#97968=CARTESIAN_POINT('Ctrl Pts',(50.2904824667079,251.229464286701,18.2789505158584)) ;
#97969=CARTESIAN_POINT('Ctrl Pts',(52.803616289905,251.549739273436,18.6049035944158)) ;
#97970=CARTESIAN_POINT('Ctrl Pts',(53.9725652609706,252.39905095601,19.4704714029658)) ;
#97971=CARTESIAN_POINT('Ctrl Pts',(54.4216982315916,252.946297015605,20.029172854931)) ;
#97972=CARTESIAN_POINT('Ctrl Pts',(47.8218443356631,252.909567273718,19.9308856107869)) ;
#97973=CARTESIAN_POINT('Ctrl Pts',(48.5341561059935,252.069093188583,19.0904741258717)) ;
#97974=CARTESIAN_POINT('Ctrl Pts',(50.2520089559848,251.147381593048,18.168769389023)) ;
#97975=CARTESIAN_POINT('Ctrl Pts',(52.8723457948022,251.475101351358,18.4964880562147)) ;
#97976=CARTESIAN_POINT('Ctrl Pts',(54.100611059619,252.346351184295,19.3677115571897)) ;
#97977=CARTESIAN_POINT('Ctrl Pts',(54.5781583101924,252.90956423463,19.9308825698009)) ;
#97978=CARTESIAN_POINT('Ctrl Pts',(47.7553501107488,252.880874227796,19.9021945713554)) ;
#97979=CARTESIAN_POINT('Ctrl Pts',(48.4856433188052,252.033943681986,19.0552640255452)) ;
#97980=CARTESIAN_POINT('Ctrl Pts',(50.2356583566825,251.106538354053,18.1278586976125)) ;
#97981=CARTESIAN_POINT('Ctrl Pts',(52.9015694301209,251.436218838326,18.4575391818863)) ;
#97982=CARTESIAN_POINT('Ctrl Pts',(54.1550539561438,252.313330163616,19.3346505071756)) ;
#97983=CARTESIAN_POINT('Ctrl Pts',(54.6446525108684,252.880871199536,19.9021915430963)) ;
#97984=CARTESIAN_POINT('Origin',(51.2,255.5,23.2284271247462)) ;
#97985=CARTESIAN_POINT('Origin',(46.6350889359327,252.258305665508,20.5213203435596)) ;
#97986=CARTESIAN_POINT('',(47.1350889359327,261.466666666667,20.5213203435596)) ;
#97987=CARTESIAN_POINT('Origin',(46.6350889359327,261.466666666667,20.5213203435596)) ;
#97988=CARTESIAN_POINT('',(47.1350889359327,257.,20.5213203435596)) ;
#97989=CARTESIAN_POINT('',(47.1350889359327,252.258305665508,20.5213203435596)) ;
#97990=CARTESIAN_POINT('Origin',(46.6350889359327,257.,20.5213203435596)) ;
#97991=CARTESIAN_POINT('Origin',(51.2,257.,20.5213203435596)) ;
#97992=CARTESIAN_POINT('Origin',(51.2,257.,20.5213203435596)) ;
#97993=CARTESIAN_POINT('Ctrl Pts',(46.6350889359327,261.46666666666,20.0213203435596)) ;
#97994=CARTESIAN_POINT('Ctrl Pts',(46.6350889359326,261.51358669041,20.0213203435594)) ;
#97995=CARTESIAN_POINT('Ctrl Pts',(46.6263598493585,261.559687576261,20.0213203435597)) ;
#97996=CARTESIAN_POINT('Ctrl Pts',(47.135088935933,261.46666666666,20.0213203435596)) ;
#97997=CARTESIAN_POINT('Ctrl Pts',(47.1350889359328,261.560506714154,20.0213203435591)) ;
#97998=CARTESIAN_POINT('Ctrl Pts',(47.1176307627857,261.65270848585,20.0213203435596)) ;
#97999=CARTESIAN_POINT('Ctrl Pts',(47.1350889359328,261.466666666663,20.5213203435598)) ;
#98000=CARTESIAN_POINT('Ctrl Pts',(47.1350889359326,261.560506714153,20.5213203435594)) ;
#98001=CARTESIAN_POINT('Ctrl Pts',(47.117630762786,261.652708485847,20.5213203435599)) ;
#98002=CARTESIAN_POINT('Origin',(46.1350889359327,261.466666666667,20.5213203435596)) ;
#98003=CARTESIAN_POINT('Origin',(55.7649110640674,248.858305665508,20.5213203435596)) ;
#98004=CARTESIAN_POINT('',(55.2649110640674,248.858305665508,20.5213203435596)) ;
#98005=CARTESIAN_POINT('Origin',(68.6350889359325,252.258305665508,20.5213203435596)) ;
#98006=CARTESIAN_POINT('',(69.1350889359328,261.466666666667,20.5213203435596)) ;
#98007=CARTESIAN_POINT('Origin',(68.6350889359328,261.466666666667,20.5213203435596)) ;
#98008=CARTESIAN_POINT('',(69.1350889359327,257.,20.5213203435596)) ;
#98009=CARTESIAN_POINT('',(69.1350889359325,252.258305665508,20.5213203435596)) ;
#98010=CARTESIAN_POINT('Origin',(68.6350889359327,257.,20.5213203435596)) ;
#98011=CARTESIAN_POINT('Origin',(73.2,257.,20.5213203435596)) ;
#98012=CARTESIAN_POINT('Origin',(73.2,257.,20.5213203435596)) ;
#98013=CARTESIAN_POINT('Origin',(57.665166384558,263.475191490368,22.9157002361986)) ;
#98014=CARTESIAN_POINT('',(57.2649110640674,263.8,22.8217108732387)) ;
#98015=CARTESIAN_POINT('',(57.5776651911054,263.8,22.5213203435596)) ;
#98016=CARTESIAN_POINT('Origin',(58.0982443974007,263.8,23.3217108732387)) ;
#98017=CARTESIAN_POINT('',(55.9649110640674,262.590434404722,21.0093633494615)) ;
#98018=CARTESIAN_POINT('',(57.665166384558,263.865625895089,22.6033527124214)) ;
#98019=CARTESIAN_POINT('',(55.6649110640674,262.6,21.3217108732387)) ;
#98020=CARTESIAN_POINT('Origin',(55.9649110640674,262.2,21.3217108732387)) ;
#98021=CARTESIAN_POINT('',(57.365166384558,263.875191490368,22.9157002361986)) ;
#98022=CARTESIAN_POINT('Ctrl Pts',(55.9650977189936,262.590464694559,21.0094012321746)) ;
#98023=CARTESIAN_POINT('Ctrl Pts',(55.8927140481104,262.53619262041,20.9415612709441)) ;
#98024=CARTESIAN_POINT('Ctrl Pts',(55.8355197652987,262.461874531184,20.848663071755)) ;
#98025=CARTESIAN_POINT('Ctrl Pts',(55.8015907112375,262.378001899972,20.7438227615689)) ;
#98026=CARTESIAN_POINT('Ctrl Pts',(55.9077153029172,262.620351120509,21.0467320017693)) ;
#98027=CARTESIAN_POINT('Ctrl Pts',(55.8195025091066,262.563096995791,20.9750736401434)) ;
#98028=CARTESIAN_POINT('Ctrl Pts',(55.7469181715793,262.484205180484,20.8768444382602)) ;
#98029=CARTESIAN_POINT('Ctrl Pts',(55.6986544996547,262.394288534095,20.7641242532738)) ;
#98030=CARTESIAN_POINT('Ctrl Pts',(55.7930388940241,262.653447436406,21.1426403859049)) ;
#98031=CARTESIAN_POINT('Ctrl Pts',(55.6732458887353,262.583510286414,21.0686846092405)) ;
#98032=CARTESIAN_POINT('Ctrl Pts',(55.5698160988869,262.486660039231,20.9668129965483)) ;
#98033=CARTESIAN_POINT('Ctrl Pts',(55.4933050272729,262.371949383066,20.8484878936816)) ;
#98034=CARTESIAN_POINT('Ctrl Pts',(55.700947067087,262.62701282797,21.26207073822)) ;
#98035=CARTESIAN_POINT('Ctrl Pts',(55.5611083984992,262.53238639435,21.1921713125216)) ;
#98036=CARTESIAN_POINT('Ctrl Pts',(55.445503826815,262.401589921389,21.0962896327055)) ;
#98037=CARTESIAN_POINT('Ctrl Pts',(55.3681023539349,262.2496543881,20.9868645016167)) ;
#98038=CARTESIAN_POINT('Ctrl Pts',(55.6651117444407,262.600150470022,21.3218049170024)) ;
#98039=CARTESIAN_POINT('Ctrl Pts',(55.5202967823214,262.49159734544,21.2539592141385)) ;
#98040=CARTESIAN_POINT('Ctrl Pts',(55.4058619171326,262.342947400721,21.1610529986893)) ;
#98041=CARTESIAN_POINT('Ctrl Pts',(55.337960684994,262.175183945868,21.0562008394061)) ;
#98042=CARTESIAN_POINT('Origin',(56.2649110640674,261.8,20.8217108732387)) ;
#98043=CARTESIAN_POINT('Origin',(56.2649110640674,262.190434404722,20.5093633494615)) ;
#98044=CARTESIAN_POINT('Ctrl Pts',(68.6350889359328,261.466666666666,20.0213203435596)) ;
#98045=CARTESIAN_POINT('Ctrl Pts',(68.6350889359328,261.513586690411,20.0213203435595)) ;
#98046=CARTESIAN_POINT('Ctrl Pts',(68.6263598493592,261.559687576258,20.0213203435596)) ;
#98047=CARTESIAN_POINT('Ctrl Pts',(69.1350889359329,261.466666666666,20.0213203435596)) ;
#98048=CARTESIAN_POINT('Ctrl Pts',(69.1350889359329,261.560506714156,20.0213203435594)) ;
#98049=CARTESIAN_POINT('Ctrl Pts',(69.1176307627859,261.652708485848,20.0213203435596)) ;
#98050=CARTESIAN_POINT('Ctrl Pts',(69.1350889359328,261.466666666667,20.5213203435597)) ;
#98051=CARTESIAN_POINT('Ctrl Pts',(69.1350889359328,261.560506714155,20.5213203435595)) ;
#98052=CARTESIAN_POINT('Ctrl Pts',(69.117630762786,261.652708485847,20.5213203435597)) ;
#98053=CARTESIAN_POINT('Origin',(68.1350889359328,261.466666666667,20.5213203435596)) ;
#98054=CARTESIAN_POINT('Ctrl Pts',(68.6262992790349,261.950068411825,20.2089058667418)) ;
#98055=CARTESIAN_POINT('Ctrl Pts',(68.6121566500185,262.024832042591,20.3023601782468)) ;
#98056=CARTESIAN_POINT('Ctrl Pts',(68.580666198832,262.09625764165,20.391642490084)) ;
#98057=CARTESIAN_POINT('Ctrl Pts',(68.5350110422629,262.157126340135,20.4677282733507)) ;
#98058=CARTESIAN_POINT('Ctrl Pts',(68.7442583098237,261.958793642379,20.2197842337291)) ;
#98059=CARTESIAN_POINT('Ctrl Pts',(68.718928193498,262.039807922115,20.3214382904355)) ;
#98060=CARTESIAN_POINT('Ctrl Pts',(68.675218628314,262.116429910232,20.4166884624688)) ;
#98061=CARTESIAN_POINT('Ctrl Pts',(68.6167573321357,262.181064672381,20.497635456136)) ;
#98062=CARTESIAN_POINT('Ctrl Pts',(68.9794298419464,261.907069815511,20.2967674292355)) ;
#98063=CARTESIAN_POINT('Ctrl Pts',(68.9323297883792,262.013111882128,20.4047154391056)) ;
#98064=CARTESIAN_POINT('Ctrl Pts',(68.8639744001522,262.109285517,20.5046232503294)) ;
#98065=CARTESIAN_POINT('Ctrl Pts',(68.780076271313,262.189708661292,20.5887317382383)) ;
#98066=CARTESIAN_POINT('Ctrl Pts',(69.1005251724556,261.743097807743,20.4462783497206)) ;
#98067=CARTESIAN_POINT('Ctrl Pts',(69.0598088706616,261.88150309857,20.544686653091)) ;
#98068=CARTESIAN_POINT('Ctrl Pts',(68.9899272559851,262.009912469407,20.6374702762036)) ;
#98069=CARTESIAN_POINT('Ctrl Pts',(68.8967323918745,262.117798129565,20.7162682354583)) ;
#98070=CARTESIAN_POINT('Ctrl Pts',(69.1176490922737,261.65261165586,20.5212598248177)) ;
#98071=CARTESIAN_POINT('Ctrl Pts',(69.0893506066564,261.802146309377,20.6147189832657)) ;
#98072=CARTESIAN_POINT('Ctrl Pts',(69.0263552568489,261.945003652573,20.7040048227633)) ;
#98073=CARTESIAN_POINT('Ctrl Pts',(68.9350298022437,262.066745503355,20.7800934795019)) ;
#98074=CARTESIAN_POINT('',(68.5350889359328,262.157101071388,20.4676966827948)) ;
#98075=CARTESIAN_POINT('',(68.9350889359328,262.066666666667,20.780044206572)) ;
#98076=CARTESIAN_POINT('Origin',(68.5350889359328,261.766666666667,20.780044206572)) ;
#98077=CARTESIAN_POINT('Origin',(68.1350889359328,261.466666666667,20.405044206572)) ;
#98078=CARTESIAN_POINT('Origin',(68.1350889359328,261.857101071388,20.0926966827948)) ;
#98079=CARTESIAN_POINT('Origin',(65.6921072521396,265.557308911724,25.5183470128943)) ;
#98080=CARTESIAN_POINT('',(67.3029147394739,263.8,22.5213203435596)) ;
#98081=CARTESIAN_POINT('',(67.6350889359328,263.8,22.9467108732387)) ;
#98082=CARTESIAN_POINT('Origin',(67.0100889359328,263.8,23.3217108732387)) ;
#98083=CARTESIAN_POINT('',(66.0921072521396,265.857308911724,25.5183470128943)) ;
#98084=CARTESIAN_POINT('',(65.6921072521396,265.947743316446,25.205999489117)) ;
#98085=CARTESIAN_POINT('Origin',(77.3541022134511,261.790576660088,20.8099316983491)) ;
#98086=CARTESIAN_POINT('',(77.9,262.590434404722,21.0093633494615)) ;
#98087=CARTESIAN_POINT('',(77.3541022134511,262.18101106481,20.4975841745719)) ;
#98088=CARTESIAN_POINT('',(77.6,262.6,21.3217108732387)) ;
#98089=CARTESIAN_POINT('Origin',(77.9,262.2,21.3217108732387)) ;
#98090=CARTESIAN_POINT('',(77.0541022134511,262.190576660088,20.8099316983491)) ;
#98091=CARTESIAN_POINT('Ctrl Pts',(77.9013408131542,262.590650840007,21.0096349450888)) ;
#98092=CARTESIAN_POINT('Ctrl Pts',(77.7773296632107,262.497850078956,20.8936360832999)) ;
#98093=CARTESIAN_POINT('Ctrl Pts',(77.7008997254075,262.344523367308,20.7019653495671)) ;
#98094=CARTESIAN_POINT('Ctrl Pts',(77.7014183412461,262.189532131413,20.5082389714827)) ;
#98095=CARTESIAN_POINT('Ctrl Pts',(77.8439164601299,262.620738304929,21.0470483108589)) ;
#98096=CARTESIAN_POINT('Ctrl Pts',(77.6926768304702,262.522860915164,20.9244672749778)) ;
#98097=CARTESIAN_POINT('Ctrl Pts',(77.5898523574372,262.360080698584,20.722059188087)) ;
#98098=CARTESIAN_POINT('Ctrl Pts',(77.5699237452358,262.189749951308,20.5078746887228)) ;
#98099=CARTESIAN_POINT('Ctrl Pts',(77.7292852020685,262.654121976102,21.1430750184117)) ;
#98100=CARTESIAN_POINT('Ctrl Pts',(77.5237875914152,262.53454414738,21.0165447946381)) ;
#98101=CARTESIAN_POINT('Ctrl Pts',(77.3673899123099,262.334900270471,20.8066567599894)) ;
#98102=CARTESIAN_POINT('Ctrl Pts',(77.3083819928147,262.104716141742,20.5755253312968)) ;
#98103=CARTESIAN_POINT('Ctrl Pts',(77.6372360358209,262.62782351523,21.2626696196308)) ;
#98104=CARTESIAN_POINT('Ctrl Pts',(77.397228569769,262.465950156281,21.1430850537563)) ;
#98105=CARTESIAN_POINT('Ctrl Pts',(77.2317300815822,262.195301292123,20.9454483332071)) ;
#98106=CARTESIAN_POINT('Ctrl Pts',(77.19981303009,261.900502715367,20.7387374087547)) ;
#98107=CARTESIAN_POINT('Ctrl Pts',(77.6014435723759,262.601080513305,21.3223861940545)) ;
#98108=CARTESIAN_POINT('Ctrl Pts',(77.3528342375612,262.415369091606,21.2063165554919)) ;
#98109=CARTESIAN_POINT('Ctrl Pts',(77.1994052692525,262.108511154987,21.0145303451059)) ;
#98110=CARTESIAN_POINT('Ctrl Pts',(77.2000017327813,261.798196834116,20.820583894561)) ;
#98111=CARTESIAN_POINT('',(77.7,262.190434404721,20.5093633494615)) ;
#98112=CARTESIAN_POINT('',(77.2,261.8,20.8217108732387)) ;
#98113=CARTESIAN_POINT('Origin',(77.7,261.8,20.8217108732387)) ;
#98114=CARTESIAN_POINT('Origin',(78.2,261.8,20.8217108732387)) ;
#98115=CARTESIAN_POINT('Origin',(78.2,262.190434404721,20.5093633494615)) ;
#98116=CARTESIAN_POINT('Origin',(77.7,263.431230834727,22.8607494166478)) ;
#98117=CARTESIAN_POINT('',(77.2,263.431230834727,22.8607494166478)) ;
#98118=CARTESIAN_POINT('',(77.7,263.821665239449,22.5484018928706)) ;
#98119=CARTESIAN_POINT('Origin',(47.15,255.5,30.7213203435596)) ;
#98120=CARTESIAN_POINT('',(47.15,256.652146641849,29.5213203435596)) ;
#98121=CARTESIAN_POINT('',(47.15,255.5,30.7213203435596)) ;
#98122=CARTESIAN_POINT('Origin',(51.2,257.,29.5213203435596)) ;
#98123=CARTESIAN_POINT('',(47.1350889359327,257.,29.5213203435596)) ;
#98124=CARTESIAN_POINT('Origin',(47.1350889359327,263.8,29.5213203435596)) ;
#98125=CARTESIAN_POINT('',(47.1350889359327,261.466666666667,29.5213203435596)) ;
#98126=CARTESIAN_POINT('Origin',(46.1350889359327,261.466666666667,29.5213203435596)) ;
#98127=CARTESIAN_POINT('',(46.9350889359326,262.066666666667,29.5213203435596)) ;
#98128=CARTESIAN_POINT('Origin',(46.3850889359327,262.8,29.5213203435596)) ;
#98129=CARTESIAN_POINT('Origin',(66.207090707265,262.8,21.2713203435596)) ;
#98130=CARTESIAN_POINT('Origin',(33.6,245.6,29.5213203435596)) ;
#98131=CARTESIAN_POINT('Origin',(33.6,245.6,20.0213203435596)) ;
#98132=CARTESIAN_POINT('Origin',(51.2,257.,29.5213203435596)) ;
#98133=CARTESIAN_POINT('',(55.25,256.652146641849,29.5213203435596)) ;
#98134=CARTESIAN_POINT('',(55.2649110640674,257.,29.5213203435596)) ;
#98135=CARTESIAN_POINT('Origin',(73.2,257.,29.5213203435596)) ;
#98136=CARTESIAN_POINT('',(69.1350889359327,257.,29.5213203435596)) ;
#98137=CARTESIAN_POINT('',(69.15,256.652146641849,29.5213203435596)) ;
#98138=CARTESIAN_POINT('Origin',(74.6,224.285258985103,29.5213203435596)) ;
#98139=CARTESIAN_POINT('',(74.6,224.787496202879,25.7213203435596)) ;
#98140=CARTESIAN_POINT('',(74.6,224.787496202879,30.7213203435596)) ;
#98141=CARTESIAN_POINT('',(74.6000000000001,225.9,25.7213203435596)) ;
#98142=CARTESIAN_POINT('',(74.6000000000001,225.9,29.5213203435596)) ;
#98143=CARTESIAN_POINT('',(74.6,225.892629492551,25.7213203435596)) ;
#98144=CARTESIAN_POINT('Origin',(74.4,225.9,29.5213203435596)) ;
#98145=CARTESIAN_POINT('',(74.4,226.1,25.7213203435596)) ;
#98146=CARTESIAN_POINT('Origin',(74.4,225.9,25.7213203435596)) ;
#98147=CARTESIAN_POINT('',(74.4,226.1,29.5213203435596)) ;
#98148=CARTESIAN_POINT('Origin',(74.4,226.1,29.5213203435596)) ;
#98149=CARTESIAN_POINT('',(74.3,226.1,25.7213203435596)) ;
#98150=CARTESIAN_POINT('',(73.7,226.1,25.7213203435596)) ;
#98151=CARTESIAN_POINT('',(74.3,226.1,29.5213203435596)) ;
#98152=CARTESIAN_POINT('Origin',(74.3,226.1,29.5213203435596)) ;
#98153=CARTESIAN_POINT('',(74.3,231.9,25.7213203435596)) ;
#98154=CARTESIAN_POINT('',(74.3,226.8,25.7213203435596)) ;
#98155=CARTESIAN_POINT('',(74.3,231.9,29.5213203435596)) ;
#98156=CARTESIAN_POINT('Origin',(74.1,231.9,29.5213203435596)) ;
#98157=CARTESIAN_POINT('',(74.1,232.1,25.7213203435596)) ;
#98158=CARTESIAN_POINT('Origin',(74.1,231.9,25.7213203435596)) ;
#98159=CARTESIAN_POINT('',(74.1,232.1,29.5213203435596)) ;
#98160=CARTESIAN_POINT('Origin',(74.1,232.1,29.5213203435596)) ;
#98161=CARTESIAN_POINT('',(71.9,232.1,25.7213203435596)) ;
#98162=CARTESIAN_POINT('',(73.55,232.1,25.7213203435596)) ;
#98163=CARTESIAN_POINT('',(71.9,232.1,29.5213203435596)) ;
#98164=CARTESIAN_POINT('Origin',(71.9,231.9,29.5213203435596)) ;
#98165=CARTESIAN_POINT('',(71.7,231.9,25.7213203435596)) ;
#98166=CARTESIAN_POINT('Origin',(71.9,231.9,25.7213203435596)) ;
#98167=CARTESIAN_POINT('',(71.7,231.9,29.5213203435596)) ;
#98168=CARTESIAN_POINT('Origin',(71.7,231.9,29.5213203435596)) ;
#98169=CARTESIAN_POINT('',(71.7,226.1,25.7213203435596)) ;
#98170=CARTESIAN_POINT('',(71.7,229.7,25.7213203435596)) ;
#98171=CARTESIAN_POINT('',(71.7,226.1,29.5213203435596)) ;
#98172=CARTESIAN_POINT('Origin',(71.7,226.1,29.5213203435596)) ;
#98173=CARTESIAN_POINT('',(71.6,226.1,25.7213203435596)) ;
#98174=CARTESIAN_POINT('',(72.3500000000003,226.1,25.7213203435596)) ;
#98175=CARTESIAN_POINT('',(71.6,226.1,29.5213203435596)) ;
#98176=CARTESIAN_POINT('Ctrl Pts',(46.3,248.9,29.5213203435596)) ;
#98177=CARTESIAN_POINT('Ctrl Pts',(46.3,248.9,18.1213203435596)) ;
#98178=CARTESIAN_POINT('Ctrl Pts',(46.2722901777919,248.927709822208,29.5213203435596)) ;
#98179=CARTESIAN_POINT('Ctrl Pts',(46.2722901777919,248.927709822208,18.1213203435596)) ;
#98180=CARTESIAN_POINT('Ctrl Pts',(46.2384776727796,248.960391271619,29.5213203435596)) ;
#98181=CARTESIAN_POINT('Ctrl Pts',(46.2384776727796,248.960391271619,18.1213203435596)) ;
#98182=CARTESIAN_POINT('Ctrl Pts',(46.1815269526849,248.99104280001,29.5213203435596)) ;
#98183=CARTESIAN_POINT('Ctrl Pts',(46.1815269526849,248.99104280001,18.1213203435596)) ;
#98184=CARTESIAN_POINT('Ctrl Pts',(46.1522826614306,249.,29.5213203435596)) ;
#98185=CARTESIAN_POINT('Ctrl Pts',(46.1522826614306,249.,18.1213203435596)) ;
#98186=CARTESIAN_POINT('Ctrl Pts',(46.1267949192431,249.,29.5213203435596)) ;
#98187=CARTESIAN_POINT('Ctrl Pts',(46.1267949192431,249.,18.1213203435596)) ;
#98188=CARTESIAN_POINT('',(46.1267949192431,249.,20.0213203435596)) ;
#98189=CARTESIAN_POINT('',(46.1267949192431,249.,29.5213203435596)) ;
#98190=CARTESIAN_POINT('Ctrl Pts',(46.3,248.9,20.0213203435596)) ;
#98191=CARTESIAN_POINT('Ctrl Pts',(46.2722901777919,248.927709822208,20.0213203435596)) ;
#98192=CARTESIAN_POINT('Ctrl Pts',(46.2384776727796,248.960391271619,20.0213203435596)) ;
#98193=CARTESIAN_POINT('Ctrl Pts',(46.1815269526849,248.99104280001,20.0213203435596)) ;
#98194=CARTESIAN_POINT('Ctrl Pts',(46.1522826614306,249.,20.0213203435596)) ;
#98195=CARTESIAN_POINT('Ctrl Pts',(46.1267949192431,249.,20.0213203435596)) ;
#98196=CARTESIAN_POINT('Origin',(46.1267949192431,249.,29.5213203435596)) ;
#98197=CARTESIAN_POINT('',(34.2732050807569,249.,20.0213203435596)) ;
#98198=CARTESIAN_POINT('',(34.2732050807569,249.,29.5213203435596)) ;
#98199=CARTESIAN_POINT('',(46.1267949192431,249.,20.0213203435596)) ;
#98200=CARTESIAN_POINT('Ctrl Pts',(34.2732050807569,249.,29.5213203435596)) ;
#98201=CARTESIAN_POINT('Ctrl Pts',(34.2732050807569,249.,18.1213203435596)) ;
#98202=CARTESIAN_POINT('Ctrl Pts',(34.2477173385693,249.,29.5213203435596)) ;
#98203=CARTESIAN_POINT('Ctrl Pts',(34.2477173385693,249.,18.1213203435596)) ;
#98204=CARTESIAN_POINT('Ctrl Pts',(34.2184730473151,248.99104280001,29.5213203435596)) ;
#98205=CARTESIAN_POINT('Ctrl Pts',(34.2184730473151,248.99104280001,18.1213203435596)) ;
#98206=CARTESIAN_POINT('Ctrl Pts',(34.1615223272204,248.960391271619,29.5213203435596)) ;
#98207=CARTESIAN_POINT('Ctrl Pts',(34.1615223272204,248.960391271619,18.1213203435596)) ;
#98208=CARTESIAN_POINT('Ctrl Pts',(34.1277098222081,248.927709822208,29.5213203435596)) ;
#98209=CARTESIAN_POINT('Ctrl Pts',(34.1277098222081,248.927709822208,18.1213203435596)) ;
#98210=CARTESIAN_POINT('Ctrl Pts',(34.1,248.9,29.5213203435596)) ;
#98211=CARTESIAN_POINT('Ctrl Pts',(34.1,248.9,18.1213203435596)) ;
#98212=CARTESIAN_POINT('Ctrl Pts',(34.2732050807569,249.,20.0213203435596)) ;
#98213=CARTESIAN_POINT('Ctrl Pts',(34.2477173385693,249.,20.0213203435596)) ;
#98214=CARTESIAN_POINT('Ctrl Pts',(34.2184730473151,248.99104280001,20.0213203435596)) ;
#98215=CARTESIAN_POINT('Ctrl Pts',(34.1615223272204,248.960391271619,20.0213203435596)) ;
#98216=CARTESIAN_POINT('Ctrl Pts',(34.1277098222081,248.927709822208,20.0213203435596)) ;
#98217=CARTESIAN_POINT('Ctrl Pts',(34.1,248.9,20.0213203435596)) ;
#98218=CARTESIAN_POINT('Origin',(43.1,259.9,29.5213203435596)) ;
#98219=CARTESIAN_POINT('',(43.1,260.1,29.5213203435596)) ;
#98220=CARTESIAN_POINT('Origin',(43.1,260.1,29.5213203435596)) ;
#98221=CARTESIAN_POINT('',(37.3,260.1,29.5213203435596)) ;
#98222=CARTESIAN_POINT('',(42.2,260.1,25.0213203435596)) ;
#98223=CARTESIAN_POINT('Origin',(40.2,260.1,25.0213203435596)) ;
#98224=CARTESIAN_POINT('Origin',(37.3,259.9,29.5213203435596)) ;
#98225=CARTESIAN_POINT('Origin',(30.7,254.8,29.5213203435596)) ;
#98226=CARTESIAN_POINT('',(28.1,254.8,25.7213203435596)) ;
#98227=CARTESIAN_POINT('',(28.1,254.8,29.5213203435596)) ;
#98228=CARTESIAN_POINT('Origin',(30.7,254.8,25.7213203435596)) ;
#98229=CARTESIAN_POINT('Origin',(75.1,252.658578643763,29.5213203435596)) ;
#98230=CARTESIAN_POINT('',(75.1,251.923339546448,25.7213203435596)) ;
#98231=CARTESIAN_POINT('',(75.1,251.923339546448,30.7213203435596)) ;
#98232=CARTESIAN_POINT('',(75.1,249.341421356237,25.7213203435596)) ;
#98233=CARTESIAN_POINT('',(75.1,249.341421356237,29.5213203435596)) ;
#98234=CARTESIAN_POINT('',(75.1,251.829289321881,25.7213203435596)) ;
#98235=CARTESIAN_POINT('Origin',(75.3,249.341421356237,29.5213203435596)) ;
#98236=CARTESIAN_POINT('',(75.1585786437627,249.2,25.7213203435596)) ;
#98237=CARTESIAN_POINT('Origin',(75.3,249.341421356237,25.7213203435596)) ;
#98238=CARTESIAN_POINT('',(75.1585786437627,249.2,29.5213203435596)) ;
#98239=CARTESIAN_POINT('Origin',(75.1585786437627,249.2,29.5213203435596)) ;
#98240=CARTESIAN_POINT('',(75.8999999999999,248.458578643763,25.7213203435596)) ;
#98241=CARTESIAN_POINT('',(75.343933982822,249.014644660941,25.7213203435596)) ;
#98242=CARTESIAN_POINT('',(75.8999999999999,248.458578643763,29.5213203435596)) ;
#98243=CARTESIAN_POINT('Origin',(76.0414213562372,248.6,29.5213203435596)) ;
#98244=CARTESIAN_POINT('',(76.0414213562372,248.4,25.7213203435596)) ;
#98245=CARTESIAN_POINT('Origin',(76.0414213562372,248.6,25.7213203435596)) ;
#98246=CARTESIAN_POINT('',(76.0414213562372,248.4,29.5213203435596)) ;
#98247=CARTESIAN_POINT('Origin',(76.0414213562372,248.4,29.5213203435596)) ;
#98248=CARTESIAN_POINT('',(80.0999999999999,248.4,25.7213203435596)) ;
#98249=CARTESIAN_POINT('',(76.8707106781186,248.4,25.7213203435596)) ;
#98250=CARTESIAN_POINT('',(80.0999999999999,248.4,29.5213203435596)) ;
#98251=CARTESIAN_POINT('Origin',(59.3,248.1,29.5213203435596)) ;
#98252=CARTESIAN_POINT('',(59.5,248.1,25.7213203435596)) ;
#98253=CARTESIAN_POINT('',(59.3,247.9,25.7213203435596)) ;
#98254=CARTESIAN_POINT('Origin',(59.3,248.1,25.7213203435596)) ;
#98255=CARTESIAN_POINT('',(59.3,247.9,29.5213203435596)) ;
#98256=CARTESIAN_POINT('',(59.5,248.1,29.5213203435596)) ;
#98257=CARTESIAN_POINT('Origin',(59.5,248.1,29.5213203435596)) ;
#98258=CARTESIAN_POINT('',(59.5,250.9,25.7213203435596)) ;
#98259=CARTESIAN_POINT('',(59.5,250.3,25.7213203435596)) ;
#98260=CARTESIAN_POINT('',(59.5,250.9,29.5213203435596)) ;
#98261=CARTESIAN_POINT('Origin',(59.3,250.9,29.5213203435596)) ;
#98262=CARTESIAN_POINT('',(59.3,251.1,25.7213203435596)) ;
#98263=CARTESIAN_POINT('Origin',(59.3,250.9,25.7213203435596)) ;
#98264=CARTESIAN_POINT('',(59.3,251.1,29.5213203435596)) ;
#98265=CARTESIAN_POINT('Origin',(59.3,251.1,29.5213203435596)) ;
#98266=CARTESIAN_POINT('',(59.2,251.1,25.7213203435596)) ;
#98267=CARTESIAN_POINT('',(58.5999999999998,251.1,25.7213203435596)) ;
#98268=CARTESIAN_POINT('',(59.2,251.1,29.5213203435596)) ;
#98269=CARTESIAN_POINT('Origin',(59.2,251.1,29.5213203435596)) ;
#98270=CARTESIAN_POINT('',(59.2,256.9,25.7213203435596)) ;
#98271=CARTESIAN_POINT('',(59.2,251.8,25.7213203435596)) ;
#98272=CARTESIAN_POINT('',(59.2,256.9,29.5213203435596)) ;
#98273=CARTESIAN_POINT('Origin',(59.,256.9,29.5213203435596)) ;
#98274=CARTESIAN_POINT('',(59.,257.1,25.7213203435596)) ;
#98275=CARTESIAN_POINT('Origin',(59.,256.9,25.7213203435596)) ;
#98276=CARTESIAN_POINT('',(59.,257.1,29.5213203435596)) ;
#98277=CARTESIAN_POINT('Origin',(59.,257.1,29.5213203435596)) ;
#98278=CARTESIAN_POINT('',(56.8,257.1,25.7213203435596)) ;
#98279=CARTESIAN_POINT('',(58.45,257.1,25.7213203435596)) ;
#98280=CARTESIAN_POINT('',(56.8,257.1,29.5213203435596)) ;
#98281=CARTESIAN_POINT('Origin',(61.5,261.2,29.5213203435596)) ;
#98282=CARTESIAN_POINT('',(59.,261.2,25.7213203435596)) ;
#98283=CARTESIAN_POINT('',(59.,261.2,29.5213203435596)) ;
#98284=CARTESIAN_POINT('Origin',(61.5,261.2,25.7213203435596)) ;
#98285=CARTESIAN_POINT('Origin',(63.0573593128808,238.841421356237,29.5213203435596)) ;
#98286=CARTESIAN_POINT('',(63.0573593128808,242.158578643763,25.7213203435596)) ;
#98287=CARTESIAN_POINT('',(63.0573593128808,238.841421356237,25.7213203435596)) ;
#98288=CARTESIAN_POINT('',(63.0573593128808,239.670710678119,25.7213203435596)) ;
#98289=CARTESIAN_POINT('',(63.0573593128808,238.841421356237,29.5213203435596)) ;
#98290=CARTESIAN_POINT('',(63.0573593128808,242.158578643763,29.5213203435596)) ;
#98291=CARTESIAN_POINT('Origin',(62.8573593128808,242.158578643763,29.5213203435596)) ;
#98292=CARTESIAN_POINT('',(62.9987806691181,242.3,25.7213203435596)) ;
#98293=CARTESIAN_POINT('Origin',(62.8573593128808,242.158578643763,25.7213203435596)) ;
#98294=CARTESIAN_POINT('',(62.9987806691181,242.3,29.5213203435596)) ;
#98295=CARTESIAN_POINT('Origin',(62.9987806691181,242.3,29.5213203435596)) ;
#98296=CARTESIAN_POINT('',(62.2573593128808,243.041421356237,25.7213203435596)) ;
#98297=CARTESIAN_POINT('',(62.8257680045734,242.473012664545,25.7213203435596)) ;
#98298=CARTESIAN_POINT('',(62.2573593128808,243.041421356237,29.5213203435596)) ;
#98299=CARTESIAN_POINT('Origin',(62.1159379566435,242.9,29.5213203435596)) ;
#98300=CARTESIAN_POINT('',(62.1159379566435,243.1,25.7213203435596)) ;
#98301=CARTESIAN_POINT('Origin',(62.1159379566435,242.9,25.7213203435596)) ;
#98302=CARTESIAN_POINT('',(62.1159379566435,243.1,29.5213203435596)) ;
#98303=CARTESIAN_POINT('Origin',(62.1159379566435,243.1,29.5213203435596)) ;
#98304=CARTESIAN_POINT('',(58.0573593128808,243.1,25.7213203435596)) ;
#98305=CARTESIAN_POINT('',(61.3113339837915,243.1,25.7213203435596)) ;
#98306=CARTESIAN_POINT('',(58.0573593128808,243.1,29.5213203435596)) ;
#98307=CARTESIAN_POINT('Ctrl Pts',(58.0573593128808,243.1,29.5213203435596)) ;
#98308=CARTESIAN_POINT('Ctrl Pts',(58.0573593128808,243.1,18.1213203435596)) ;
#98309=CARTESIAN_POINT('Ctrl Pts',(58.0296494906727,243.072290177792,29.5213203435596)) ;
#98310=CARTESIAN_POINT('Ctrl Pts',(58.0296494906727,243.072290177792,18.1213203435596)) ;
#98311=CARTESIAN_POINT('Ctrl Pts',(57.9969680412619,243.03847767278,29.5213203435596)) ;
#98312=CARTESIAN_POINT('Ctrl Pts',(57.9969680412619,243.03847767278,18.1213203435596)) ;
#98313=CARTESIAN_POINT('Ctrl Pts',(57.9663165128705,242.981526952685,29.5213203435596)) ;
#98314=CARTESIAN_POINT('Ctrl Pts',(57.9663165128705,242.981526952685,18.1213203435596)) ;
#98315=CARTESIAN_POINT('Ctrl Pts',(57.9573593128807,242.952282661431,29.5213203435596)) ;
#98316=CARTESIAN_POINT('Ctrl Pts',(57.9573593128807,242.952282661431,18.1213203435596)) ;
#98317=CARTESIAN_POINT('Ctrl Pts',(57.9573593128807,242.926794919243,29.5213203435596)) ;
#98318=CARTESIAN_POINT('Ctrl Pts',(57.9573593128807,242.926794919243,18.1213203435596)) ;
#98319=CARTESIAN_POINT('',(57.9573593128808,242.926794919243,25.7213203435596)) ;
#98320=CARTESIAN_POINT('Ctrl Pts',(57.9573593128807,242.926794919243,25.7213203435596)) ;
#98321=CARTESIAN_POINT('Ctrl Pts',(57.9573593128807,242.952282661431,25.7213203435596)) ;
#98322=CARTESIAN_POINT('Ctrl Pts',(57.9663165128705,242.981526952685,25.7213203435596)) ;
#98323=CARTESIAN_POINT('Ctrl Pts',(57.9969680412619,243.03847767278,25.7213203435596)) ;
#98324=CARTESIAN_POINT('Ctrl Pts',(58.0296494906727,243.072290177792,25.7213203435596)) ;
#98325=CARTESIAN_POINT('Ctrl Pts',(58.0573593128808,243.1,25.7213203435596)) ;
#98326=CARTESIAN_POINT('',(57.9573593128808,242.926794919243,29.5213203435596)) ;
#98327=CARTESIAN_POINT('Origin',(62.5573593128808,227.1,29.5213203435596)) ;
#98328=CARTESIAN_POINT('',(62.7573593128808,227.1,25.7213203435596)) ;
#98329=CARTESIAN_POINT('',(62.5573593128808,226.9,25.7213203435596)) ;
#98330=CARTESIAN_POINT('Origin',(62.5573593128808,227.1,25.7213203435596)) ;
#98331=CARTESIAN_POINT('',(62.5573593128808,226.9,29.5213203435596)) ;
#98332=CARTESIAN_POINT('',(62.7573593128808,227.1,29.5213203435596)) ;
#98333=CARTESIAN_POINT('Origin',(62.7573593128808,227.1,29.5213203435596)) ;
#98334=CARTESIAN_POINT('',(62.7573593128808,229.9,25.7213203435596)) ;
#98335=CARTESIAN_POINT('',(62.7573593128808,229.275314650971,25.7213203435596)) ;
#98336=CARTESIAN_POINT('',(62.7573593128808,229.9,29.5213203435596)) ;
#98337=CARTESIAN_POINT('Origin',(62.5573593128808,229.9,29.5213203435596)) ;
#98338=CARTESIAN_POINT('',(62.5573593128808,230.1,25.7213203435596)) ;
#98339=CARTESIAN_POINT('Origin',(62.5573593128808,229.9,25.7213203435596)) ;
#98340=CARTESIAN_POINT('',(62.5573593128808,230.1,29.5213203435596)) ;
#98341=CARTESIAN_POINT('Origin',(62.5573593128808,230.1,29.5213203435596)) ;
#98342=CARTESIAN_POINT('',(62.4573593128808,230.1,25.7213203435596)) ;
#98343=CARTESIAN_POINT('',(61.8573593128805,230.1,25.7213203435596)) ;
#98344=CARTESIAN_POINT('',(62.4573593128808,230.1,29.5213203435596)) ;
#98345=CARTESIAN_POINT('Origin',(62.4573593128808,230.1,29.5213203435596)) ;
#98346=CARTESIAN_POINT('',(62.4573593128808,230.775314650971,25.7213203435596)) ;
#98347=CARTESIAN_POINT('Origin',(62.2841542321239,236.,29.5213203435596)) ;
#98348=CARTESIAN_POINT('',(60.0305643936376,236.,25.7213203435596)) ;
#98349=CARTESIAN_POINT('',(61.7207567725023,236.,25.7213203435596)) ;
#98350=CARTESIAN_POINT('',(60.0305643936376,236.,29.5213203435596)) ;
#98351=CARTESIAN_POINT('Origin',(76.0414213562372,225.6,29.5213203435596)) ;
#98352=CARTESIAN_POINT('',(76.0414213562372,225.5,25.7213203435596)) ;
#98353=CARTESIAN_POINT('',(75.9707106781185,225.529289321881,25.7213203435596)) ;
#98354=CARTESIAN_POINT('Origin',(76.0414213562372,225.6,25.7213203435596)) ;
#98355=CARTESIAN_POINT('',(75.9707106781185,225.529289321881,29.5213203435596)) ;
#98356=CARTESIAN_POINT('',(76.0414213562372,225.5,29.5213203435596)) ;
#98357=CARTESIAN_POINT('Origin',(76.0414213562372,225.5,29.5213203435596)) ;
#98358=CARTESIAN_POINT('',(80.0999999999999,225.5,25.7213203435596)) ;
#98359=CARTESIAN_POINT('',(76.8707106781186,225.5,25.7213203435596)) ;
#98360=CARTESIAN_POINT('',(80.,225.5,30.7213203435596)) ;
#98361=CARTESIAN_POINT('',(80.0999999999999,225.5,29.5213203435596)) ;
#98362=CARTESIAN_POINT('Origin',(80.0999999999999,225.6,29.5213203435596)) ;
#98363=CARTESIAN_POINT('',(80.1999999999999,225.6,25.7213203435596)) ;
#98364=CARTESIAN_POINT('Origin',(80.0999999999999,225.6,25.7213203435596)) ;
#98365=CARTESIAN_POINT('',(80.1999999999999,225.6,29.5213203435596)) ;
#98366=CARTESIAN_POINT('Origin',(80.1999999999999,225.6,29.5213203435596)) ;
#98367=CARTESIAN_POINT('',(80.2,230.4,25.7213203435596)) ;
#98368=CARTESIAN_POINT('',(80.1999999999999,226.8,25.7213203435596)) ;
#98369=CARTESIAN_POINT('',(80.2,230.4,29.5213203435596)) ;
#98370=CARTESIAN_POINT('Origin',(80.1,230.4,29.5213203435596)) ;
#98371=CARTESIAN_POINT('Origin',(80.1,230.4,25.7213203435596)) ;
#98372=CARTESIAN_POINT('Origin',(67.3,248.1,29.5213203435596)) ;
#98373=CARTESIAN_POINT('',(67.5,248.1,25.7213203435596)) ;
#98374=CARTESIAN_POINT('',(67.3,247.9,25.7213203435596)) ;
#98375=CARTESIAN_POINT('Origin',(67.3,248.1,25.7213203435596)) ;
#98376=CARTESIAN_POINT('',(67.3,247.9,29.5213203435596)) ;
#98377=CARTESIAN_POINT('',(67.5,248.1,29.5213203435596)) ;
#98378=CARTESIAN_POINT('Origin',(67.5,248.1,29.5213203435596)) ;
#98379=CARTESIAN_POINT('',(67.5,250.9,25.7213203435596)) ;
#98380=CARTESIAN_POINT('',(67.5,250.3,25.7213203435596)) ;
#98381=CARTESIAN_POINT('',(67.5,250.9,29.5213203435596)) ;
#98382=CARTESIAN_POINT('Origin',(67.3,250.9,29.5213203435596)) ;
#98383=CARTESIAN_POINT('',(67.3,251.1,25.7213203435596)) ;
#98384=CARTESIAN_POINT('Origin',(67.3,250.9,25.7213203435596)) ;
#98385=CARTESIAN_POINT('',(67.3,251.1,29.5213203435596)) ;
#98386=CARTESIAN_POINT('Origin',(67.3,251.1,29.5213203435596)) ;
#98387=CARTESIAN_POINT('',(67.2,251.1,25.7213203435596)) ;
#98388=CARTESIAN_POINT('',(66.5999999999998,251.1,25.7213203435596)) ;
#98389=CARTESIAN_POINT('',(67.2,251.1,29.5213203435596)) ;
#98390=CARTESIAN_POINT('Origin',(67.2,251.1,29.5213203435596)) ;
#98391=CARTESIAN_POINT('',(67.2,256.9,25.7213203435596)) ;
#98392=CARTESIAN_POINT('',(67.2,251.8,25.7213203435596)) ;
#98393=CARTESIAN_POINT('',(67.2,256.9,29.5213203435596)) ;
#98394=CARTESIAN_POINT('Origin',(67.,256.9,29.5213203435596)) ;
#98395=CARTESIAN_POINT('',(67.,257.1,25.7213203435596)) ;
#98396=CARTESIAN_POINT('Origin',(67.,256.9,25.7213203435596)) ;
#98397=CARTESIAN_POINT('',(67.,257.1,29.5213203435596)) ;
#98398=CARTESIAN_POINT('Origin',(67.,257.1,29.5213203435596)) ;
#98399=CARTESIAN_POINT('',(64.8,257.1,25.7213203435596)) ;
#98400=CARTESIAN_POINT('',(66.45,257.1,25.7213203435596)) ;
#98401=CARTESIAN_POINT('',(64.8,257.1,29.5213203435596)) ;
#98402=CARTESIAN_POINT('Origin',(64.8,256.9,29.5213203435596)) ;
#98403=CARTESIAN_POINT('',(64.6,256.9,25.7213203435596)) ;
#98404=CARTESIAN_POINT('Origin',(64.8,256.9,25.7213203435596)) ;
#98405=CARTESIAN_POINT('',(64.6,256.9,29.5213203435596)) ;
#98406=CARTESIAN_POINT('Origin',(64.6,256.9,29.5213203435596)) ;
#98407=CARTESIAN_POINT('',(64.6,251.1,25.7213203435596)) ;
#98408=CARTESIAN_POINT('',(64.6,254.7,25.7213203435596)) ;
#98409=CARTESIAN_POINT('',(64.6,251.1,29.5213203435596)) ;
#98410=CARTESIAN_POINT('Origin',(64.6,251.1,29.5213203435596)) ;
#98411=CARTESIAN_POINT('',(64.5,251.1,25.7213203435596)) ;
#98412=CARTESIAN_POINT('',(65.2500000000003,251.1,25.7213203435596)) ;
#98413=CARTESIAN_POINT('',(64.5,251.1,29.5213203435596)) ;
#98414=CARTESIAN_POINT('Origin',(64.5,250.9,29.5213203435596)) ;
#98415=CARTESIAN_POINT('',(64.3,250.9,25.7213203435596)) ;
#98416=CARTESIAN_POINT('Origin',(64.5,250.9,25.7213203435596)) ;
#98417=CARTESIAN_POINT('',(64.3,250.9,29.5213203435596)) ;
#98418=CARTESIAN_POINT('Origin',(64.3,250.9,29.5213203435596)) ;
#98419=CARTESIAN_POINT('',(64.3,248.1,25.7213203435596)) ;
#98420=CARTESIAN_POINT('',(64.3,251.7,25.7213203435596)) ;
#98421=CARTESIAN_POINT('',(64.3,248.1,29.5213203435596)) ;
#98422=CARTESIAN_POINT('Origin',(64.5,248.1,29.5213203435596)) ;
#98423=CARTESIAN_POINT('',(64.5,247.9,25.7213203435596)) ;
#98424=CARTESIAN_POINT('Origin',(64.5,248.1,25.7213203435596)) ;
#98425=CARTESIAN_POINT('',(64.5,247.9,29.5213203435596)) ;
#98426=CARTESIAN_POINT('Origin',(64.5,247.9,29.5213203435596)) ;
#98427=CARTESIAN_POINT('',(65.2,247.9,25.7213203435596)) ;
#98428=CARTESIAN_POINT('Origin',(65.9,252.5,25.7213203435596)) ;
#98429=CARTESIAN_POINT('Origin',(57.9573593128808,242.926794919243,29.5213203435596)) ;
#98430=CARTESIAN_POINT('',(57.9573593128808,238.073205080757,25.7213203435596)) ;
#98431=CARTESIAN_POINT('',(57.9573593128808,241.713397459622,25.7213203435596)) ;
#98432=CARTESIAN_POINT('',(57.9573593128808,238.073205080757,29.5213203435596)) ;
#98433=CARTESIAN_POINT('Ctrl Pts',(57.9573593128807,238.073205080757,29.5213203435596)) ;
#98434=CARTESIAN_POINT('Ctrl Pts',(57.9573593128807,238.073205080757,18.1213203435596)) ;
#98435=CARTESIAN_POINT('Ctrl Pts',(57.9573593128807,238.047717338569,29.5213203435596)) ;
#98436=CARTESIAN_POINT('Ctrl Pts',(57.9573593128807,238.047717338569,18.1213203435596)) ;
#98437=CARTESIAN_POINT('Ctrl Pts',(57.9663165128705,238.018473047315,29.5213203435596)) ;
#98438=CARTESIAN_POINT('Ctrl Pts',(57.9663165128705,238.018473047315,18.1213203435596)) ;
#98439=CARTESIAN_POINT('Ctrl Pts',(57.9969680412619,237.96152232722,29.5213203435596)) ;
#98440=CARTESIAN_POINT('Ctrl Pts',(57.9969680412619,237.96152232722,18.1213203435596)) ;
#98441=CARTESIAN_POINT('Ctrl Pts',(58.0296494906727,237.927709822208,29.5213203435596)) ;
#98442=CARTESIAN_POINT('Ctrl Pts',(58.0296494906727,237.927709822208,18.1213203435596)) ;
#98443=CARTESIAN_POINT('Ctrl Pts',(58.0573593128808,237.9,29.5213203435596)) ;
#98444=CARTESIAN_POINT('Ctrl Pts',(58.0573593128808,237.9,18.1213203435596)) ;
#98445=CARTESIAN_POINT('',(58.0573593128808,237.9,25.7213203435596)) ;
#98446=CARTESIAN_POINT('Ctrl Pts',(58.0573593128808,237.9,25.7213203435596)) ;
#98447=CARTESIAN_POINT('Ctrl Pts',(58.0296494906727,237.927709822208,25.7213203435596)) ;
#98448=CARTESIAN_POINT('Ctrl Pts',(57.9969680412619,237.96152232722,25.7213203435596)) ;
#98449=CARTESIAN_POINT('Ctrl Pts',(57.9663165128705,238.018473047315,25.7213203435596)) ;
#98450=CARTESIAN_POINT('Ctrl Pts',(57.9573593128807,238.047717338569,25.7213203435596)) ;
#98451=CARTESIAN_POINT('Ctrl Pts',(57.9573593128807,238.073205080757,25.7213203435596)) ;
#98452=CARTESIAN_POINT('',(58.0573593128808,237.9,29.5213203435596)) ;
#98453=CARTESIAN_POINT('Origin',(58.0573593128808,237.9,29.5213203435596)) ;
#98454=CARTESIAN_POINT('',(62.1159379566435,237.9,25.7213203435596)) ;
#98455=CARTESIAN_POINT('',(59.2820446619101,237.9,25.7213203435596)) ;
#98456=CARTESIAN_POINT('',(62.1159379566435,237.9,29.5213203435596)) ;
#98457=CARTESIAN_POINT('Origin',(62.1159379566435,238.1,29.5213203435596)) ;
#98458=CARTESIAN_POINT('',(62.2573593128808,237.958578643763,25.7213203435596)) ;
#98459=CARTESIAN_POINT('Origin',(62.1159379566435,238.1,25.7213203435596)) ;
#98460=CARTESIAN_POINT('',(62.2573593128808,237.958578643763,29.5213203435596)) ;
#98461=CARTESIAN_POINT('Origin',(62.2573593128808,237.958578643763,29.5213203435596)) ;
#98462=CARTESIAN_POINT('',(62.9987806691181,238.7,25.7213203435596)) ;
#98463=CARTESIAN_POINT('',(62.4550573264548,238.156276657337,25.7213203435596)) ;
#98464=CARTESIAN_POINT('',(62.9987806691181,238.7,29.5213203435596)) ;
#98465=CARTESIAN_POINT('Origin',(62.8573593128808,238.841421356237,29.5213203435596)) ;
#98466=CARTESIAN_POINT('Origin',(62.8573593128808,238.841421356237,25.7213203435596)) ;
#98467=CARTESIAN_POINT('Origin',(60.5067300109395,240.5,25.7213203435596)) ;
#98468=CARTESIAN_POINT('Ctrl Pts',(60.0305643936376,236.,29.5213203435596)) ;
#98469=CARTESIAN_POINT('Ctrl Pts',(60.0305643936376,236.,18.1213203435596)) ;
#98470=CARTESIAN_POINT('Ctrl Pts',(60.0050766514501,236.,29.5213203435596)) ;
#98471=CARTESIAN_POINT('Ctrl Pts',(60.0050766514501,236.,18.1213203435596)) ;
#98472=CARTESIAN_POINT('Ctrl Pts',(59.9758323601959,235.99104280001,29.5213203435596)) ;
#98473=CARTESIAN_POINT('Ctrl Pts',(59.9758323601959,235.99104280001,18.1213203435596)) ;
#98474=CARTESIAN_POINT('Ctrl Pts',(59.9188816401012,235.960391271619,29.5213203435596)) ;
#98475=CARTESIAN_POINT('Ctrl Pts',(59.9188816401012,235.960391271619,18.1213203435596)) ;
#98476=CARTESIAN_POINT('Ctrl Pts',(59.8850691350889,235.927709822208,29.5213203435596)) ;
#98477=CARTESIAN_POINT('Ctrl Pts',(59.8850691350889,235.927709822208,18.1213203435596)) ;
#98478=CARTESIAN_POINT('Ctrl Pts',(59.8573593128808,235.9,29.5213203435596)) ;
#98479=CARTESIAN_POINT('Ctrl Pts',(59.8573593128808,235.9,18.1213203435596)) ;
#98480=CARTESIAN_POINT('',(59.8573593128808,235.9,25.7213203435596)) ;
#98481=CARTESIAN_POINT('Ctrl Pts',(59.8573593128808,235.9,25.7213203435596)) ;
#98482=CARTESIAN_POINT('Ctrl Pts',(59.8850691350889,235.927709822208,25.7213203435596)) ;
#98483=CARTESIAN_POINT('Ctrl Pts',(59.9188816401012,235.960391271619,25.7213203435596)) ;
#98484=CARTESIAN_POINT('Ctrl Pts',(59.9758323601959,235.99104280001,25.7213203435596)) ;
#98485=CARTESIAN_POINT('Ctrl Pts',(60.0050766514501,236.,25.7213203435596)) ;
#98486=CARTESIAN_POINT('Ctrl Pts',(60.0305643936376,236.,25.7213203435596)) ;
#98487=CARTESIAN_POINT('',(59.8573593128808,235.9,29.5213203435596)) ;
#98488=CARTESIAN_POINT('Origin',(59.8573593128808,235.9,29.5213203435596)) ;
#98489=CARTESIAN_POINT('',(59.8573593128808,230.1,25.7213203435596)) ;
#98490=CARTESIAN_POINT('',(59.8573593128808,233.675314650971,25.7213203435596)) ;
#98491=CARTESIAN_POINT('',(59.8573593128808,230.1,29.5213203435596)) ;
#98492=CARTESIAN_POINT('Origin',(59.8573593128808,230.1,29.5213203435596)) ;
#98493=CARTESIAN_POINT('',(59.7573593128808,230.1,25.7213203435596)) ;
#98494=CARTESIAN_POINT('',(60.5073593128808,230.1,25.7213203435596)) ;
#98495=CARTESIAN_POINT('',(59.7573593128808,230.1,29.5213203435596)) ;
#98496=CARTESIAN_POINT('Origin',(59.7573593128808,229.9,29.5213203435596)) ;
#98497=CARTESIAN_POINT('',(59.5573593128808,229.9,25.7213203435596)) ;
#98498=CARTESIAN_POINT('Origin',(59.7573593128808,229.9,25.7213203435596)) ;
#98499=CARTESIAN_POINT('',(59.5573593128808,229.9,29.5213203435596)) ;
#98500=CARTESIAN_POINT('Origin',(59.5573593128808,229.9,29.5213203435596)) ;
#98501=CARTESIAN_POINT('',(59.5573593128807,227.1,25.7213203435596)) ;
#98502=CARTESIAN_POINT('',(59.5573593128808,230.675314650971,25.7213203435596)) ;
#98503=CARTESIAN_POINT('',(59.5573593128807,227.1,29.5213203435596)) ;
#98504=CARTESIAN_POINT('Origin',(59.7573593128808,227.1,29.5213203435596)) ;
#98505=CARTESIAN_POINT('',(59.7573593128808,226.9,25.7213203435596)) ;
#98506=CARTESIAN_POINT('Origin',(59.7573593128808,227.1,25.7213203435596)) ;
#98507=CARTESIAN_POINT('',(59.7573593128808,226.9,29.5213203435596)) ;
#98508=CARTESIAN_POINT('Origin',(59.7573593128808,226.9,29.5213203435596)) ;
#98509=CARTESIAN_POINT('',(60.4573593128807,226.9,25.7213203435596)) ;
#98510=CARTESIAN_POINT('Origin',(61.1573593128807,231.450629301941,25.7213203435596)) ;
#98511=CARTESIAN_POINT('Origin',(80.0999999999999,248.6,29.5213203435596)) ;
#98512=CARTESIAN_POINT('',(80.2999999999999,248.6,25.7213203435596)) ;
#98513=CARTESIAN_POINT('Origin',(80.0999999999999,248.6,25.7213203435596)) ;
#98514=CARTESIAN_POINT('',(80.2999999999999,248.6,29.5213203435596)) ;
#98515=CARTESIAN_POINT('Origin',(80.2999999999999,248.6,29.5213203435596)) ;
#98516=CARTESIAN_POINT('',(80.2999999999999,249.600000000004,25.7213203435596)) ;
#98517=CARTESIAN_POINT('',(80.2999999999999,249.8,25.7213203435596)) ;
#98518=CARTESIAN_POINT('',(80.2999999999999,249.600000000004,29.5213203435596)) ;
#98519=CARTESIAN_POINT('Origin',(80.2999999999999,249.600000000004,29.5213203435596)) ;
#98520=CARTESIAN_POINT('',(80.2,249.600000000004,25.7213203435596)) ;
#98521=CARTESIAN_POINT('',(79.,249.600000000004,25.7213203435596)) ;
#98522=CARTESIAN_POINT('',(80.2,249.600000000004,29.5213203435596)) ;
#98523=CARTESIAN_POINT('Origin',(80.2,249.600000000004,29.5213203435596)) ;
#98524=CARTESIAN_POINT('',(80.2,252.400000000001,25.7213203435596)) ;
#98525=CARTESIAN_POINT('',(80.2,250.300000000002,25.7213203435596)) ;
#98526=CARTESIAN_POINT('',(80.2,252.400000000001,29.5213203435596)) ;
#98527=CARTESIAN_POINT('Origin',(80.2,252.400000000001,29.5213203435596)) ;
#98528=CARTESIAN_POINT('',(80.3,252.400000000001,25.7213203435596)) ;
#98529=CARTESIAN_POINT('',(78.95,252.400000000001,25.7213203435596)) ;
#98530=CARTESIAN_POINT('',(80.3,252.400000000001,29.5213203435596)) ;
#98531=CARTESIAN_POINT('Origin',(80.3,252.400000000001,29.5213203435596)) ;
#98532=CARTESIAN_POINT('',(80.3,253.4,25.7213203435596)) ;
#98533=CARTESIAN_POINT('',(80.3,251.700000000001,25.7213203435596)) ;
#98534=CARTESIAN_POINT('',(80.3,253.4,29.5213203435596)) ;
#98535=CARTESIAN_POINT('Origin',(80.1,253.4,29.5213203435596)) ;
#98536=CARTESIAN_POINT('',(80.1,253.6,25.7213203435596)) ;
#98537=CARTESIAN_POINT('Origin',(80.1,253.4,25.7213203435596)) ;
#98538=CARTESIAN_POINT('',(80.1,253.6,29.5213203435596)) ;
#98539=CARTESIAN_POINT('Origin',(77.7,251.,25.7213203435596)) ;
#98540=CARTESIAN_POINT('',(76.7766604535517,253.6,25.7213203435596)) ;
#98541=CARTESIAN_POINT('Origin',(73.2,255.5,25.7213203435596)) ;
#98542=CARTESIAN_POINT('',(78.9,253.6,25.7213203435596)) ;
#98543=CARTESIAN_POINT('Origin',(56.8,256.9,29.5213203435596)) ;
#98544=CARTESIAN_POINT('',(56.6,256.9,25.7213203435596)) ;
#98545=CARTESIAN_POINT('Origin',(56.8,256.9,25.7213203435596)) ;
#98546=CARTESIAN_POINT('',(56.6,256.9,29.5213203435596)) ;
#98547=CARTESIAN_POINT('Origin',(56.6,256.9,29.5213203435596)) ;
#98548=CARTESIAN_POINT('',(56.6,251.1,25.7213203435596)) ;
#98549=CARTESIAN_POINT('',(56.6,254.7,25.7213203435596)) ;
#98550=CARTESIAN_POINT('',(56.6,251.1,29.5213203435596)) ;
#98551=CARTESIAN_POINT('Origin',(56.6,251.1,29.5213203435596)) ;
#98552=CARTESIAN_POINT('',(56.5,251.1,25.7213203435596)) ;
#98553=CARTESIAN_POINT('',(57.2500000000003,251.1,25.7213203435596)) ;
#98554=CARTESIAN_POINT('',(56.5,251.1,29.5213203435596)) ;
#98555=CARTESIAN_POINT('Origin',(56.5,250.9,29.5213203435596)) ;
#98556=CARTESIAN_POINT('',(56.3,250.9,25.7213203435596)) ;
#98557=CARTESIAN_POINT('Origin',(56.5,250.9,25.7213203435596)) ;
#98558=CARTESIAN_POINT('',(56.3,250.9,29.5213203435596)) ;
#98559=CARTESIAN_POINT('Origin',(56.3,250.9,29.5213203435596)) ;
#98560=CARTESIAN_POINT('',(56.3,248.1,25.7213203435596)) ;
#98561=CARTESIAN_POINT('',(56.3,251.7,25.7213203435596)) ;
#98562=CARTESIAN_POINT('',(56.3,248.1,29.5213203435596)) ;
#98563=CARTESIAN_POINT('Origin',(56.5,248.1,29.5213203435596)) ;
#98564=CARTESIAN_POINT('',(56.5,247.9,25.7213203435596)) ;
#98565=CARTESIAN_POINT('Origin',(56.5,248.1,25.7213203435596)) ;
#98566=CARTESIAN_POINT('',(56.5,247.9,29.5213203435596)) ;
#98567=CARTESIAN_POINT('Origin',(56.5,247.9,29.5213203435596)) ;
#98568=CARTESIAN_POINT('',(57.2,247.9,25.7213203435596)) ;
#98569=CARTESIAN_POINT('Origin',(57.9,252.5,25.7213203435596)) ;
#98570=CARTESIAN_POINT('Origin',(76.0414213562372,230.4,29.5213203435596)) ;
#98571=CARTESIAN_POINT('',(75.9707106781186,230.470710678119,25.7213203435596)) ;
#98572=CARTESIAN_POINT('Origin',(76.0414213562372,230.4,25.7213203435596)) ;
#98573=CARTESIAN_POINT('',(75.9707106781186,230.470710678119,29.5213203435596)) ;
#98574=CARTESIAN_POINT('Origin',(75.9707106781186,230.470710678119,29.5213203435596)) ;
#98575=CARTESIAN_POINT('',(75.2292893218813,229.729289321881,25.7213203435596)) ;
#98576=CARTESIAN_POINT('',(75.7853553390592,230.285355339059,25.7213203435596)) ;
#98577=CARTESIAN_POINT('',(75.2292893218813,229.729289321881,29.5213203435596)) ;
#98578=CARTESIAN_POINT('Origin',(75.3,229.658578643763,29.5213203435596)) ;
#98579=CARTESIAN_POINT('',(75.2,229.658578643763,25.7213203435596)) ;
#98580=CARTESIAN_POINT('Origin',(75.3,229.658578643763,25.7213203435596)) ;
#98581=CARTESIAN_POINT('',(75.2,229.658578643763,29.5213203435596)) ;
#98582=CARTESIAN_POINT('Origin',(75.2,229.658578643763,29.5213203435596)) ;
#98583=CARTESIAN_POINT('',(75.1999999999999,226.341421356237,25.7213203435596)) ;
#98584=CARTESIAN_POINT('',(75.2,228.829289321881,25.7213203435596)) ;
#98585=CARTESIAN_POINT('',(75.1999999999999,226.341421356237,29.5213203435596)) ;
#98586=CARTESIAN_POINT('Origin',(75.2999999999999,226.341421356237,29.5213203435596)) ;
#98587=CARTESIAN_POINT('',(75.2292893218813,226.270710678119,25.7213203435596)) ;
#98588=CARTESIAN_POINT('Origin',(75.2999999999999,226.341421356237,25.7213203435596)) ;
#98589=CARTESIAN_POINT('',(75.2292893218813,226.270710678119,29.5213203435596)) ;
#98590=CARTESIAN_POINT('Origin',(75.2292893218813,226.270710678119,29.5213203435596)) ;
#98591=CARTESIAN_POINT('',(75.4146446609407,226.085355339059,25.7213203435596)) ;
#98592=CARTESIAN_POINT('Origin',(77.7,228.,25.7213203435596)) ;
#98593=CARTESIAN_POINT('Origin',(30.7,254.8,25.7213203435596)) ;
#98594=CARTESIAN_POINT('Origin',(71.6,225.9,29.5213203435596)) ;
#98595=CARTESIAN_POINT('',(71.4,225.9,25.7213203435596)) ;
#98596=CARTESIAN_POINT('Origin',(71.6,225.9,25.7213203435596)) ;
#98597=CARTESIAN_POINT('',(71.4,225.9,29.5213203435596)) ;
#98598=CARTESIAN_POINT('Origin',(71.4,225.9,29.5213203435596)) ;
#98599=CARTESIAN_POINT('',(71.4,223.1,25.7213203435596)) ;
#98600=CARTESIAN_POINT('',(71.4,226.7,25.7213203435596)) ;
#98601=CARTESIAN_POINT('',(71.4,223.1,29.5213203435596)) ;
#98602=CARTESIAN_POINT('Origin',(61.5,261.2,25.7213203435596)) ;
#98603=CARTESIAN_POINT('Origin',(56.2649110640674,263.05,29.5213203435596)) ;
#98604=CARTESIAN_POINT('',(55.6649110640674,262.6,29.5213203435596)) ;
#98605=CARTESIAN_POINT('',(57.2649110640674,263.8,29.5213203435596)) ;
#98606=CARTESIAN_POINT('Origin',(55.2649110640674,263.8,29.5213203435596)) ;
#98607=CARTESIAN_POINT('',(67.6350889359328,263.8,29.5213203435596)) ;
#98608=CARTESIAN_POINT('',(55.2395462392986,263.8,22.5213203435596)) ;
#98609=CARTESIAN_POINT('Origin',(68.3850889359328,262.8,29.5213203435596)) ;
#98610=CARTESIAN_POINT('',(68.9350889359328,262.066666666667,29.5213203435596)) ;
#98611=CARTESIAN_POINT('Origin',(77.2,257.723534352175,29.5213203435596)) ;
#98612=CARTESIAN_POINT('',(77.2,257.723534352175,29.5213203435596)) ;
#98613=CARTESIAN_POINT('',(77.2,261.8,29.5213203435596)) ;
#98614=CARTESIAN_POINT('Origin',(82.9283628290597,247.251297405594,30.7213203435596)) ;
#98615=CARTESIAN_POINT('Origin',(81.1,247.600000000001,30.7213203435596)) ;
#98616=CARTESIAN_POINT('',(81.1,247.600000000001,30.7213203435596)) ;
#98617=CARTESIAN_POINT('Origin',(84.1283628290597,244.301866670644,30.7213203435596)) ;
#98618=CARTESIAN_POINT('',(82.349868392482,246.421393804845,30.7213203435596)) ;
#98619=CARTESIAN_POINT('Origin',(81.9668461709225,246.100000000001,30.7213203435596)) ;
#98620=CARTESIAN_POINT('',(81.9668461709225,246.600000000001,30.7213203435596)) ;
#98621=CARTESIAN_POINT('Origin',(81.9668461709225,246.600000000001,30.7213203435596)) ;
#98622=CARTESIAN_POINT('',(80.6401337790902,246.600000000001,30.7213203435596)) ;
#98623=CARTESIAN_POINT('Origin',(80.6,247.098386676966,30.7213203435596)) ;
#98624=CARTESIAN_POINT('',(81.1,247.098386676966,30.7213203435596)) ;
#98625=CARTESIAN_POINT('Origin',(81.1,247.098386676966,30.7213203435596)) ;
#98626=CARTESIAN_POINT('Origin',(73.,227.5,25.7213203435596)) ;
#98627=CARTESIAN_POINT('',(71.4146847058821,223.024778714675,25.7213203435596)) ;
#98628=CARTESIAN_POINT('Origin',(74.9999999999998,220.305309236676,25.7213203435596)) ;
#98629=CARTESIAN_POINT('Origin',(71.6,223.1,25.7213203435596)) ;
#98630=CARTESIAN_POINT('Origin',(71.6,223.1,29.5213203435596)) ;
#98631=CARTESIAN_POINT('',(71.4146847058821,223.024778714675,30.7213203435596)) ;
#98632=CARTESIAN_POINT('Origin',(80.,230.5,30.7213203435596)) ;
#98633=CARTESIAN_POINT('Origin',(74.9999999999998,220.305309236676,30.7213203435596)) ;
#98634=CARTESIAN_POINT('',(75.,224.805309236676,30.7213203435596)) ;
#98635=CARTESIAN_POINT('Origin',(75.,224.805309236676,30.7213203435596)) ;
#98636=CARTESIAN_POINT('',(80.,224.805309236676,30.7213203435596)) ;
#98637=CARTESIAN_POINT('Origin',(80.,224.805309236676,30.7213203435596)) ;
#98638=CARTESIAN_POINT('Origin',(72.1450953968557,220.262610236549,30.7213203435596)) ;
#98639=CARTESIAN_POINT('',(70.4999999999999,220.262610236549,30.7213203435596)) ;
#98640=CARTESIAN_POINT('Origin',(70.4999999999998,218.133222662034,30.7213203435596)) ;
#98641=CARTESIAN_POINT('Origin',(69.1350889359328,263.8,29.5213203435596)) ;
#98642=CARTESIAN_POINT('',(69.1350889359328,261.466666666667,29.5213203435596)) ;
#98643=CARTESIAN_POINT('Origin',(68.1350889359328,261.466666666667,29.5213203435596)) ;
#98644=CARTESIAN_POINT('Origin',(78.2,263.05,29.5213203435596)) ;
#98645=CARTESIAN_POINT('',(77.6,262.6,29.5213203435596)) ;
#98646=CARTESIAN_POINT('Origin',(78.2,261.8,29.5213203435596)) ;
#98647=CARTESIAN_POINT('Origin',(55.2395462392986,262.8,21.2713203435596)) ;
#98648=CARTESIAN_POINT('Origin',(55.2649110640674,257.,29.5213203435596)) ;
#98649=CARTESIAN_POINT('',(55.2649110640674,261.8,29.5213203435596)) ;
#98650=CARTESIAN_POINT('Origin',(56.2649110640674,261.8,29.5213203435596)) ;
#98651=CARTESIAN_POINT('Origin',(40.2,265.,25.0213203435596)) ;
#98652=CARTESIAN_POINT('',(42.2,265.,25.0213203435596)) ;
#98653=CARTESIAN_POINT('Origin',(80.1,253.6,29.5213203435596)) ;
#98654=CARTESIAN_POINT('',(76.7766604535517,253.6,30.7213203435596)) ;
#98655=CARTESIAN_POINT('Origin',(73.2,257.,29.5213203435596)) ;
#98656=CARTESIAN_POINT('',(77.25,256.652146641849,29.5213203435596)) ;
#98657=CARTESIAN_POINT('Origin',(69.15,255.5,30.7213203435596)) ;
#98658=CARTESIAN_POINT('',(69.15,255.5,30.7213203435596)) ;
#98659=CARTESIAN_POINT('Origin',(73.2,255.5,30.7213203435596)) ;
#98660=CARTESIAN_POINT('',(77.25,255.5,30.7213203435596)) ;
#98661=CARTESIAN_POINT('Origin',(77.25,256.652146641849,30.7213203435596)) ;
#98662=CARTESIAN_POINT('Origin',(55.25,256.652146641849,30.7213203435596)) ;
#98663=CARTESIAN_POINT('',(55.25,255.5,30.7213203435596)) ;
#98664=CARTESIAN_POINT('Origin',(51.2,255.5,30.7213203435596)) ;
#98665=CARTESIAN_POINT('Origin',(44.5,256.,25.7213203435596)) ;
#98666=CARTESIAN_POINT('',(45.7,253.,25.7213203435596)) ;
#98667=CARTESIAN_POINT('',(45.7,259.,25.7213203435596)) ;
#98668=CARTESIAN_POINT('Origin',(45.7,253.,20.0213203435596)) ;
#98669=CARTESIAN_POINT('Origin',(37.1,259.,20.0213203435596)) ;
#98670=CARTESIAN_POINT('Origin',(55.2141814145299,249.05,20.0213203435596)) ;
#98671=CARTESIAN_POINT('Origin',(43.3,253.,20.0213203435596)) ;
#117141=UNCERTAINTY_MEASURE_WITH_UNIT(LENGTH_MEASURE(0.01),#117171,
'DISTANCE_ACCURACY_VALUE',
'Maximum model space distance between geometric entities at asserted c
onnectivities') ;
#117147=UNCERTAINTY_MEASURE_WITH_UNIT(LENGTH_MEASURE(0.01),#117171,
'DISTANCE_ACCURACY_VALUE',
'Maximum model space distance between geometric entities at asserted c
onnectivities') ;
#117164=(
GEOMETRIC_REPRESENTATION_CONTEXT(3)
GLOBAL_UNCERTAINTY_ASSIGNED_CONTEXT((#117141))
GLOBAL_UNIT_ASSIGNED_CONTEXT((#117171,#117173,#117174))
REPRESENTATION_CONTEXT('','3D')
) ;
#117170=(
GEOMETRIC_REPRESENTATION_CONTEXT(3)
GLOBAL_UNCERTAINTY_ASSIGNED_CONTEXT((#117147))
GLOBAL_UNIT_ASSIGNED_CONTEXT((#117171,#117173,#117174))
REPRESENTATION_CONTEXT('','3D')
) ;
#117171=(
LENGTH_UNIT()
NAMED_UNIT(*)
SI_UNIT(.MILLI.,.METRE.)
) ;
#117173=(
NAMED_UNIT(*)
PLANE_ANGLE_UNIT()
SI_UNIT($,.RADIAN.)
) ;
#117174=(
NAMED_UNIT(*)
SI_UNIT($,.STERADIAN.)
SOLID_ANGLE_UNIT()
) ;
#117191=SHAPE_DEFINITION_REPRESENTATION(#117213,#117256) ;
#117213=PRODUCT_DEFINITION_SHAPE('',$,#117279) ;
#117256=SHAPE_REPRESENTATION('',(#52526),#117164) ;
#117262=PRODUCT_DEFINITION_CONTEXT('part definition',#117330,'design') ;
#117279=PRODUCT_DEFINITION('Housing','Housing',#117301,#117262) ;
#117301=PRODUCT_DEFINITION_FORMATION('',$,#117348) ;
#117330=APPLICATION_CONTEXT(
'Core Data for Automotive Mechanical Design Process') ;
#117331=PRODUCT_CONTEXT('part definition',#117330,'mechanical') ;
#117348=PRODUCT('Housing','Housing',$,(#117331)) ;
#117355=PRESENTATION_STYLE_ASSIGNMENT((#117357)) ;
#117357=SURFACE_STYLE_USAGE(.BOTH.,#117359) ;
#117359=SURFACE_SIDE_STYLE('',(#117361)) ;
#117361=SURFACE_STYLE_FILL_AREA(#117363) ;
#117363=FILL_AREA_STYLE('Opaque(160,160,160)',(#117365)) ;
#117365=FILL_AREA_STYLE_COLOUR('Opaque(160,160,160)',#117367) ;
#117367=COLOUR_RGB('Opaque(160,160,160)', 0.09019608, 0.27058824, 0.51372549) ;
ENDSEC;
END-ISO-10303-21;
